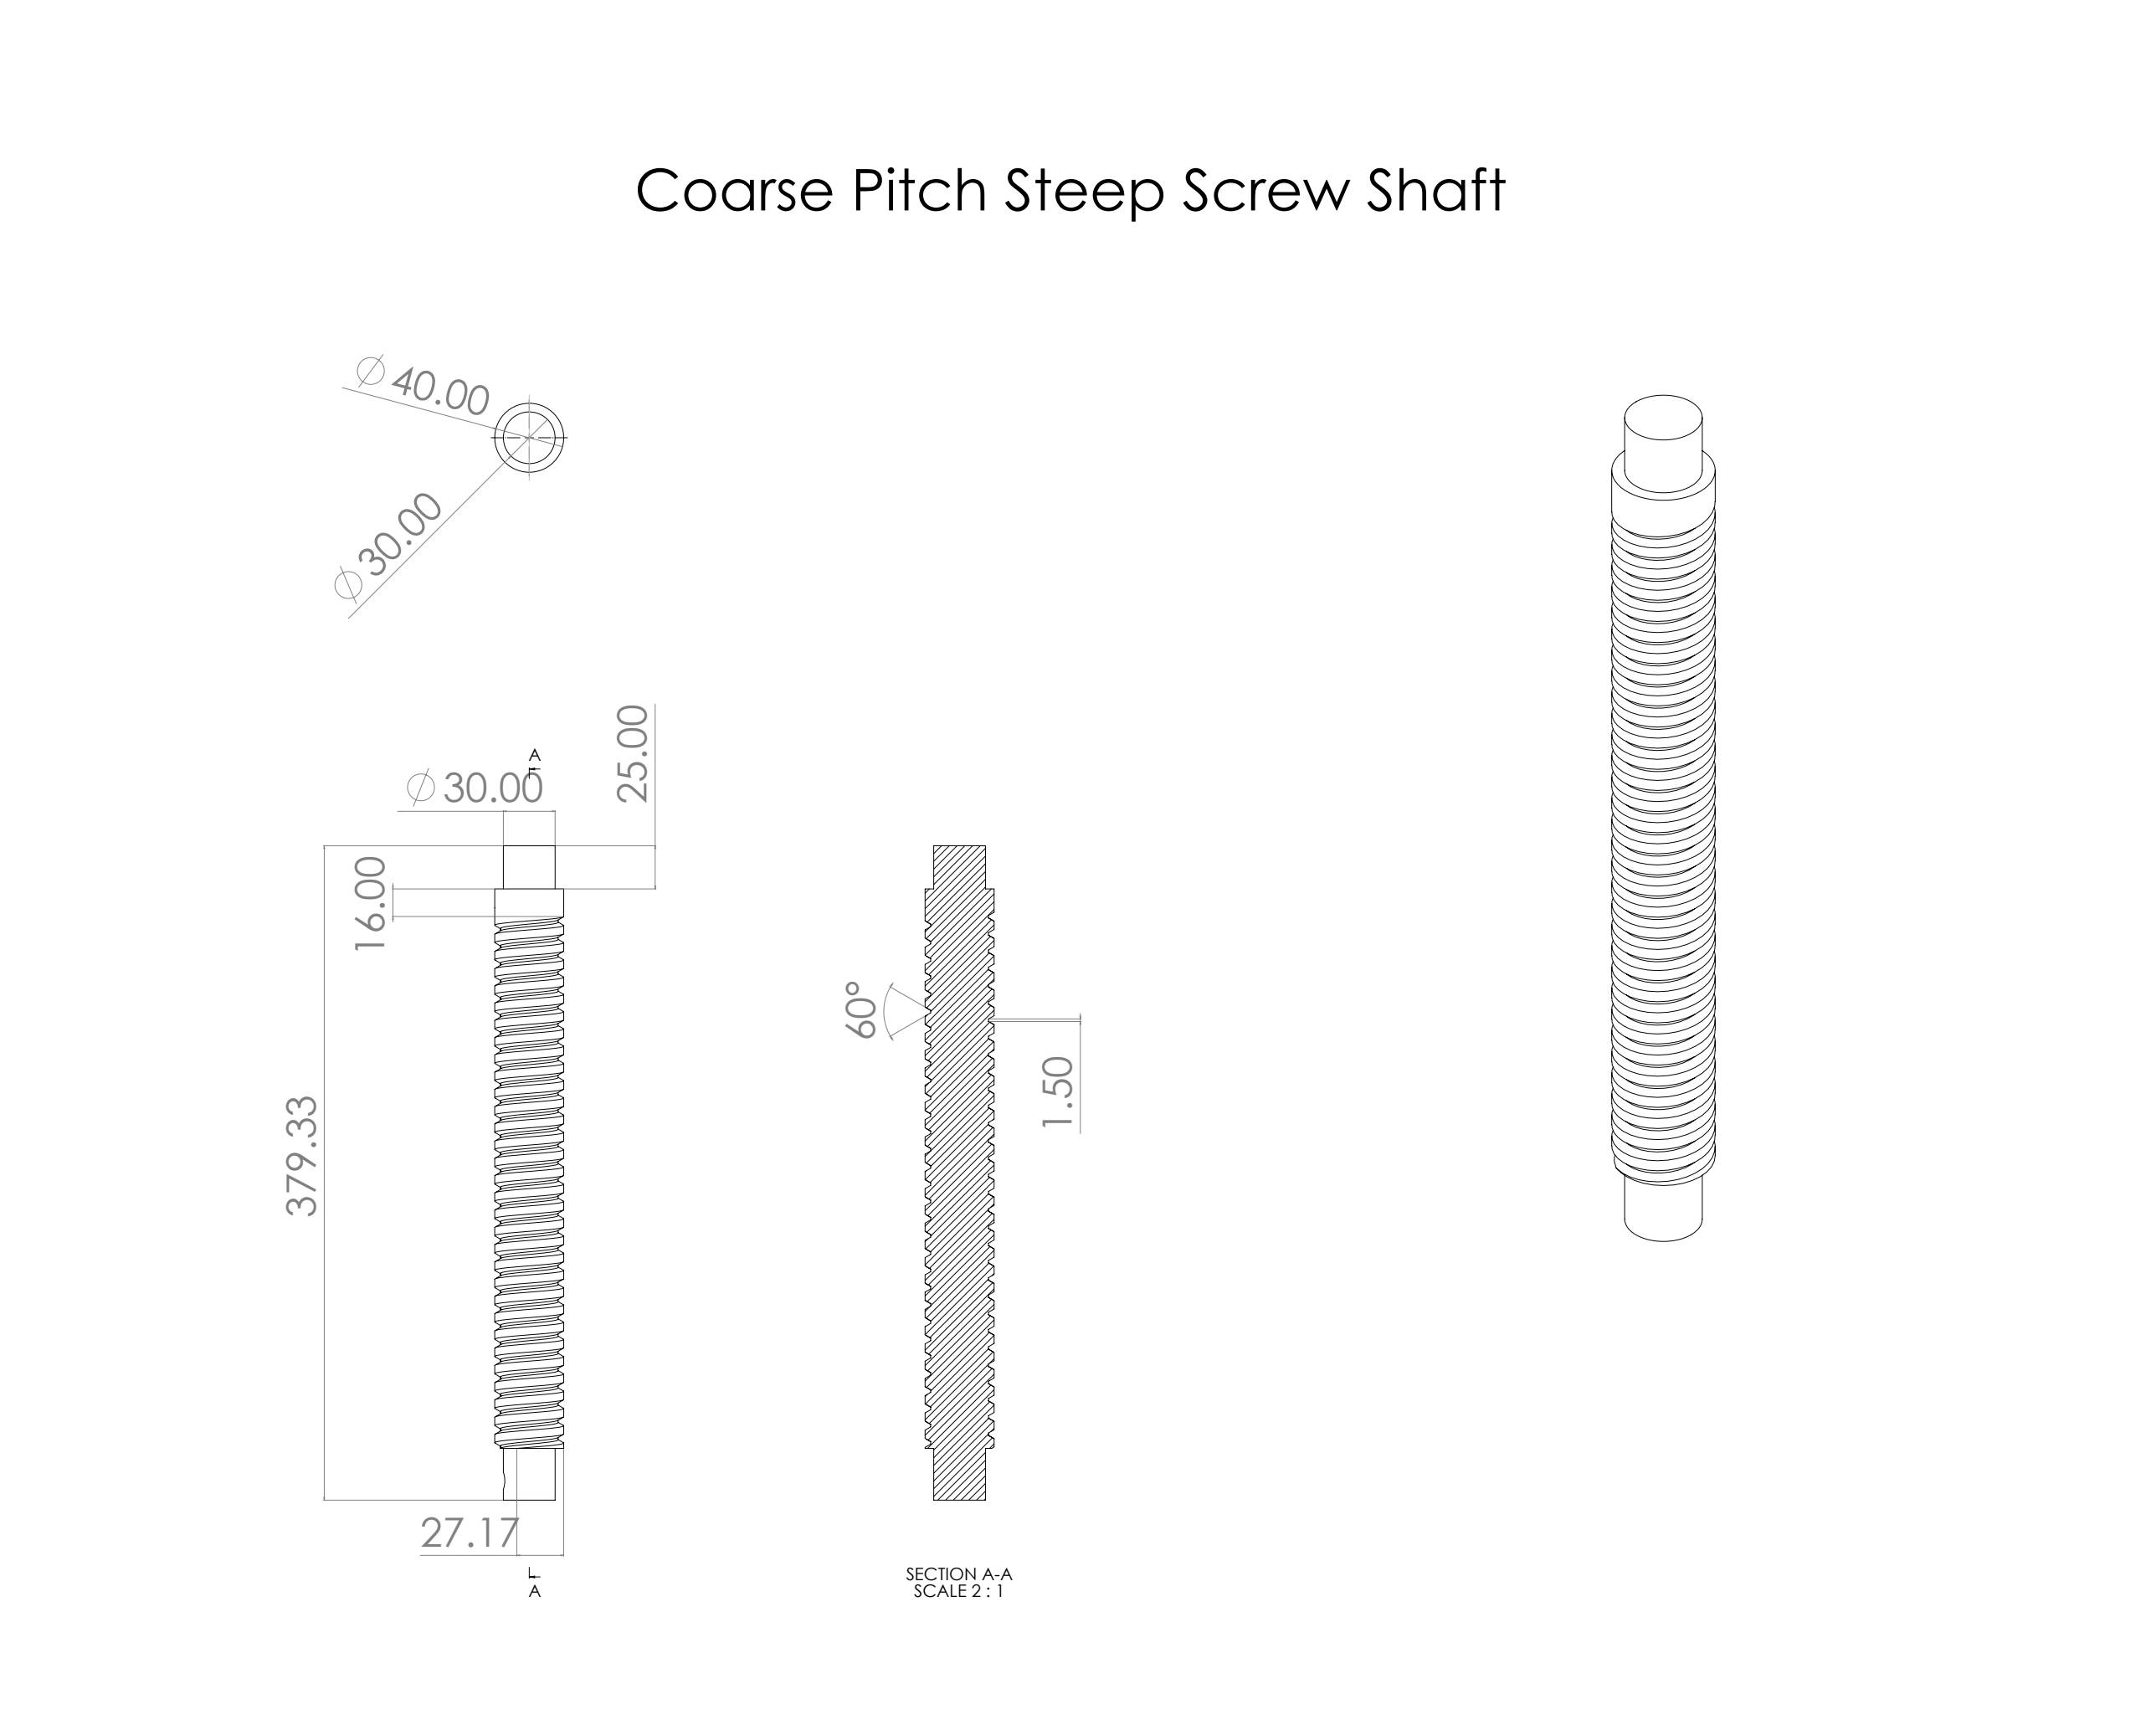
ISO-10303-21;
HEADER;
FILE_DESCRIPTION (('STEP AP214'),
    '1' );
FILE_NAME ('Coarse Pitch Steep Screw Shaft.step',
    '2026-10-24T00:28:05',
    ( '' ),
    ( '' ),
    'SwSTEP 2.0',
    'SolidWorks 2025',
    '' );
FILE_SCHEMA (( 'AUTOMOTIVE_DESIGN' ));
ENDSEC;

DATA;
#1=CARTESIAN_POINT ( 'NONE',  ( -40.53162694259543031, 272.6198905683720568, -11.84573899990672707 ) ) ;
#2=CARTESIAN_POINT ( 'NONE',  ( -13.20868407381886200, 380.9948905683720568, -6.410867750099233042 ) ) ;
#6=CARTESIAN_POINT ( 'NONE',  ( -10.20829729246297646, 267.6198905765655809, -7.653668647301794969 ) ) ;
#7=CARTESIAN_POINT ( 'NONE',  ( -42.88789093042844058, 432.9323905683720000, -9.489475012073736337 ) ) ;
#10=CARTESIAN_POINT ( 'NONE',  ( -47.16347859291445133, 436.6198905601784759, -7.653668647301793193 ) ) ;
#15=CARTESIAN_POINT ( 'NONE',  ( -40.01497788969912506, 298.8073905601784759, 16.95518130045146776 ) ) ;
#17=CARTESIAN_POINT ( 'NONE',  ( -40.53162694259543741, 334.1198905683720568, -11.84573899990672707 ) ) ;
#18=CARTESIAN_POINT ( 'NONE',  ( -48.68588794268872277, 492.3073905765656946, 3.978247347593168115 ) ) ;
#19=CARTESIAN_POINT ( 'NONE',  ( -25.35362745456398059, 366.6823905683720000, 16.75240474999998952 ) ) ;
#20=CARTESIAN_POINT ( 'NONE',  ( -28.68588794268870856, 309.4948905765656377, -19.99999999999999289 ) ) ;
#21=CARTESIAN_POINT ( 'NONE',  ( -11.93348319268872437, 388.5573905683719431, 3.332260488124728859 ) ) ;
#22=CARTESIAN_POINT ( 'NONE',  ( -36.33955658999050087, 300.1198905765656377, -18.47759065022572855 ) ) ;
#24=CARTESIAN_POINT ( 'NONE',  ( -28.68588794268870146, 276.3698905683720000, 16.75240474999999307 ) ) ;
#27=CARTESIAN_POINT ( 'NONE',  ( -16.84014894278199392, 429.1198905683720000, 11.84573899990672530 ) ) ;
#29=CARTESIAN_POINT ( 'NONE',  ( -45.64106924314019409, 498.1823905601784759, 11.32908994701042538 ) ) ;
#31=CARTESIAN_POINT ( 'NONE',  ( -36.33955658999052218, 449.1198905601784759, 18.47759065022572500 ) ) ;
#33=CARTESIAN_POINT ( 'NONE',  ( -35.09675569278794427, 343.4948905683720000, -15.47720386886985544 ) ) ;
#34=CARTESIAN_POINT ( 'NONE',  ( -45.43829269268872650, 483.8698905683720568, 0.000000000000000000 ) ) ;
#36=CARTESIAN_POINT ( 'NONE',  ( -14.54375231895778597, 493.4948905601784759, -14.14213562373094746 ) ) ;
#37=CARTESIAN_POINT ( 'NONE',  ( -11.93348319268871371, 298.8698905683720000, -2.051577885510841163E-15 ) ) ;
#43=ORIENTED_EDGE ( 'NONE', *, *, #17610, .F. ) ;
#44=CYLINDRICAL_SURFACE ( 'NONE', #20879, 19.99999999999999645 ) ;
#46=CARTESIAN_POINT ( 'NONE',  ( -38.17536295476245556, 396.9323905683721136, 14.20200298773971781 ) ) ;
#47=CARTESIAN_POINT ( 'NONE',  ( -42.82802356641967378, 478.4948905601784759, 14.14213562373094923 ) ) ;
#50=CARTESIAN_POINT ( 'NONE',  ( -35.09675569278795848, 415.7448905683720000, 15.47720386886985366 ) ) ;
#52=CARTESIAN_POINT ( 'NONE',  ( -44.16309181155858710, 453.2448905683720000, -6.410867750099231266 ) ) ;
#54=( BOUNDED_CURVE ( )  B_SPLINE_CURVE ( 2, ( #11189, #17470, #6102, #14134, #19307, #19518, #7828, #9666, #17890, #9247, #17790, #20831, #12824, #19413, #5894, #9562, #16180 ),
 .UNSPECIFIED., .F., .T. ) 
 B_SPLINE_CURVE_WITH_KNOTS ( ( 3, 2, 2, 2, 2, 2, 2, 2, 3 ),
 ( 0.5937500000000002220, 0.5957031250000002220, 0.5976562500000002220, 0.5996093750000002220, 0.6015625000000002220, 0.6035156250000002220, 0.6054687500000002220, 0.6074218750000002220, 0.6093750000000002220 ),
 .UNSPECIFIED. ) 
 CURVE ( )  GEOMETRIC_REPRESENTATION_ITEM ( )  RATIONAL_B_SPLINE_CURVE ( ( 0.9999999999999977796, 0.9807852804032326510, 1.000000000000000000, 0.9807852804032304306, 1.000000000000000000, 0.9807852804032304306, 1.000000000000000000, 0.9807852804032304306, 1.000000000000000000, 0.9807852804032304306, 1.000000000000000000, 0.9807852804032304306, 1.000000000000000000, 0.9807852804032304306, 1.000000000000000000, 0.9807852804032282101, 1.000000000000002220 ) ) 
 REPRESENTATION_ITEM ( '' )  );
#56=DIRECTION ( 'NONE',  ( -1.191790137725560488E-16, 1.000000000000000000, -0.000000000000000000 ) ) ;
#57=CARTESIAN_POINT ( 'NONE',  ( -40.01497788969913927, 393.5573905765656377, 16.95518130045146776 ) ) ;
#58=CYLINDRICAL_SURFACE ( 'NONE', #7896, 15.00000000000000000 ) ;
#61=CARTESIAN_POINT ( 'NONE',  ( -47.16347859291445843, 491.3698905765655809, -7.653668647301793193 ) ) ;
#62=CARTESIAN_POINT ( 'NONE',  ( -11.93348319268873858, 500.3698905683720000, -2.051577885510841163E-15 ) ) ;
#65=DIRECTION ( 'NONE',  ( -1.191790137725560488E-16, 1.000000000000000000, -0.000000000000000000 ) ) ;
#67=CARTESIAN_POINT ( 'NONE',  ( -48.68588794268872277, 467.2448905601784759, 0.000000000000000000 ) ) ;
#69=CARTESIAN_POINT ( 'NONE',  ( -11.93348319268872615, 400.3698905683720000, -2.051577885510841163E-15 ) ) ;
#71=CARTESIAN_POINT ( 'NONE',  ( -22.27502019258946930, 222.2448905683720568, -15.47720386886985544 ) ) ;
#72=CARTESIAN_POINT ( 'NONE',  ( -22.27502019258947641, 356.9948905683720000, 15.47720386886985189 ) ) ;
#75=CARTESIAN_POINT ( 'NONE',  ( -44.16309181155859420, 533.2448905683719431, -6.410867750099231266 ) ) ;
#76=ORIENTED_EDGE ( 'NONE', *, *, #1697, .T. ) ;
#77=CARTESIAN_POINT ( 'NONE',  ( -11.93348319268873148, 450.3698905683720000, -2.051577885510841163E-15 ) ) ;
#78=CARTESIAN_POINT ( 'NONE',  ( -11.93348319268874036, 519.1823905683719431, -3.332260488124732856 ) ) ;
#81=CARTESIAN_POINT ( 'NONE',  ( -36.33955658999052218, 429.1198905601784759, 18.47759065022572500 ) ) ;
#82=CARTESIAN_POINT ( 'NONE',  ( -45.43829269268872650, 493.8698905683720568, 0.000000000000000000 ) ) ;
#84=CARTESIAN_POINT ( 'NONE',  ( -13.20868407381887799, 499.4948905683720568, -6.410867750099233042 ) ) ;
#86=CARTESIAN_POINT ( 'NONE',  ( -40.01497788969914637, 440.4323905765656377, -16.95518130045146421 ) ) ;
#88=CARTESIAN_POINT ( 'NONE',  ( -8.685887942688530927, 247.3073905765656093, -3.978247347592740013 ) ) ;
#93=CARTESIAN_POINT ( 'NONE',  ( -28.68588794268870856, 292.8698905683720568, -16.75240474999999307 ) ) ;
#95=CARTESIAN_POINT ( 'NONE',  ( -14.54375231895775400, 260.9948905601784759, 14.14213562373094568 ) ) ;
#98=CARTESIAN_POINT ( 'NONE',  ( -16.84014894278200458, 509.1198905683720568, 11.84573899990672530 ) ) ;
#99=CARTESIAN_POINT ( 'NONE',  ( -32.66413529028187668, 369.4323905601784190, 19.99999999999999289 ) ) ;
#102=CARTESIAN_POINT ( 'NONE',  ( -14.48388495494900852, 469.4323905683720568, 9.489475012073732785 ) ) ;
#103=CARTESIAN_POINT ( 'NONE',  ( -42.88789093042842637, 274.8073905683720000, 9.489475012073736337 ) ) ;
#108=CARTESIAN_POINT ( 'NONE',  ( -10.20829729246297291, 237.6198905765656377, -7.653668647301794969 ) ) ;
#109=CARTESIAN_POINT ( 'NONE',  ( -28.68588794268870501, 309.7448905601785327, 19.99999999999999289 ) ) ;
#110=CARTESIAN_POINT ( 'NONE',  ( -48.68588794268872988, 537.2448905601785327, 0.000000000000000000 ) ) ;
#112=CARTESIAN_POINT ( 'NONE',  ( -44.16309181155856578, 273.2448905683720568, -6.410867750099231266 ) ) ;
#114=CARTESIAN_POINT ( 'NONE',  ( -11.93348319268872260, 350.6823905683720000, -3.332260488124732856 ) ) ;
#115=EDGE_CURVE ( 'NONE', #339, #18802, #16604, .T. ) ;
#118=CARTESIAN_POINT ( 'NONE',  ( -19.19641293061498999, 427.3073905683720568, 14.20200298773971426 ) ) ;
#119=CARTESIAN_POINT ( 'NONE',  ( -14.54375231895778420, 510.9948905601784190, 14.14213562373094568 ) ) ;
#121=CARTESIAN_POINT ( 'NONE',  ( -14.54375231895777354, 420.9948905601784759, 14.14213562373094568 ) ) ;
#125=ORIENTED_EDGE ( 'NONE', *, *, #1712, .T. ) ;
#126=VERTEX_POINT ( 'NONE', #20705 ) ;
#127=CARTESIAN_POINT ( 'NONE',  ( -45.43829269268873361, 525.3698905683720568, 0.000000000000000000 ) ) ;
#128=CARTESIAN_POINT ( 'NONE',  ( -36.33955658999050087, 305.3698905601784759, -18.47759065022572855 ) ) ;
#131=CARTESIAN_POINT ( 'NONE',  ( -35.09675569278794427, 343.4948905683720000, -15.47720386886985544 ) ) ;
#133=CARTESIAN_POINT ( 'NONE',  ( -45.64106924314020119, 481.0573905765656377, -11.32908994701042715 ) ) ;
#134=CARTESIAN_POINT ( 'NONE',  ( -38.17536295476245556, 362.3073905683719431, -14.20200298773971426 ) ) ;
#135=VECTOR ( 'NONE', #18235, 1000.000000000000000 ) ;
#136=CARTESIAN_POINT ( 'NONE',  ( -14.48388495494899963, 377.9323905683720000, 9.489475012073731008 ) ) ;
#137=CARTESIAN_POINT ( 'NONE',  ( -14.54375231895775933, 305.7448905765656377, 14.14213562373094568 ) ) ;
#139=CARTESIAN_POINT ( 'NONE',  ( -32.01814843081343298, 271.6823905683720000, -16.75240474999999307 ) ) ;
#140=CARTESIAN_POINT ( 'NONE',  ( -24.70764059509555821, 440.0573905601785327, 19.99999999999998934 ) ) ;
#141=CARTESIAN_POINT ( 'NONE',  ( -28.68588794268871922, 427.8698905683720568, 16.75240474999999307 ) ) ;
#143=CARTESIAN_POINT ( 'NONE',  ( -48.68588794268881514, 497.5573905601784190, 3.978247347592954952 ) ) ;
#148=CARTESIAN_POINT ( 'NONE',  ( -13.20868407381885845, 340.9948905683720000, -6.410867750099233042 ) ) ;
#149=CARTESIAN_POINT ( 'NONE',  ( -32.01814843081346140, 486.0573905683721136, 16.75240474999999307 ) ) ;
#152=CARTESIAN_POINT ( 'NONE',  ( -28.68588794268872633, 489.7448905601784759, 19.99999999999999289 ) ) ;
#153=CARTESIAN_POINT ( 'NONE',  ( -40.53162694259543031, 312.6198905683720000, -11.84573899990672707 ) ) ;
#159=CARTESIAN_POINT ( 'NONE',  ( -42.88789093042844058, 394.4323905683720000, -9.489475012073734561 ) ) ;
#160=CARTESIAN_POINT ( 'NONE',  ( -14.54375231895777709, 445.7448905765656377, 14.14213562373094568 ) ) ;
#162=CARTESIAN_POINT ( 'NONE',  ( -22.27502019258948351, 416.9948905683720000, 15.47720386886985189 ) ) ;
#163=CARTESIAN_POINT ( 'NONE',  ( -38.17536295476243424, 256.9323905683720568, 14.20200298773971781 ) ) ;
#164=CARTESIAN_POINT ( 'NONE',  ( -38.17536295476246266, 442.3073905683721136, -14.20200298773971426 ) ) ;
#166=CARTESIAN_POINT ( 'NONE',  ( -48.68588794268873698, 573.2448905601785327, 0.000000000000000000 ) ) ;
#167=CARTESIAN_POINT ( 'NONE',  ( -10.20829729246298534, 356.3698905765655809, 7.653668647301790529 ) ) ;
#169=CARTESIAN_POINT ( 'NONE',  ( -14.54375231895777354, 388.2448905765655809, -14.14213562373094746 ) ) ;
#170=CARTESIAN_POINT ( 'NONE',  ( -32.66413529028187668, 429.8073905765656946, -19.99999999999999289 ) ) ;
#172=CARTESIAN_POINT ( 'NONE',  ( -22.27502019258949417, 498.4948905683720568, 15.47720386886985189 ) ) ;
#175=CARTESIAN_POINT ( 'NONE',  ( -40.01497788969915348, 465.6823905601785896, -16.95518130045146421 ) ) ;
#176=CARTESIAN_POINT ( 'NONE',  ( -14.54375231895777354, 420.9948905601784759, 14.14213562373094568 ) ) ;
#177=CARTESIAN_POINT ( 'NONE',  ( -11.93348319268872615, 400.6823905683720568, -3.332260488124732856 ) ) ;
#178=CARTESIAN_POINT ( 'NONE',  ( -47.16347859291445843, 471.3698905765656377, -7.653668647301793193 ) ) ;
#180=CARTESIAN_POINT ( 'NONE',  ( -42.88789093042841927, 236.3073905683720284, 9.489475012073736337 ) ) ;
#181=CARTESIAN_POINT ( 'NONE',  ( -35.09675569278795138, 365.7448905683720568, 15.47720386886985366 ) ) ;
#183=CARTESIAN_POINT ( 'NONE',  ( -16.84014894278200813, 527.6198905683719431, 11.84573899990672530 ) ) ;
#185=CARTESIAN_POINT ( 'NONE',  ( -35.09675569278795848, 447.2448905683720000, 15.47720386886985366 ) ) ;
#186=( BOUNDED_CURVE ( )  B_SPLINE_CURVE ( 2, ( #15683, #18905, #9166, #8954, #869, #19445, #2803, #4526, #19338, #8177, #16322, #1390, #12644, #11113, #16106, #17715, #7966, #3227, #12748, #9388, #20969, #19235, #11001, #14702, #1604, #16006, #4629, #6032, #9702, #21278, #1189, #19652, #11223, #18032, #12856, #14808, #9803, #4832, #1496, #17820, #3012, #6451, #7759, #4419, #17612, #2913, #9493, #16426, #14385, #6138, #1283, #7861, #14489, #21070, #6244, #9596, #16213, #8072, #12959, #19548, #14595, #13067, #11432, #21177, #6349, #4729, #11326, #17920, #3118, #15134, #11654, #3650, #13178, #3748, #8400, #11760, #18356, #8721, #18246, #1830, #8286, #19984, #15026, #16753, #98, #20097, #13397, #18136, #19875, #13290, #2139, #10231, #1940, #6557, #5050, #10021, #3438, #8506, #18566, #6670, #3330, #16531, #19763, #4947, #8608, #16958, #9912, #5164, #20768, #16855, #15231, #1717, #13612, #3545, #11969, #6776, #11547, #10336, #20198, #2039, #10132, #14915, #16646, #425, #315, #209, #6883, #13503, #5266, #5365, #11868, #18461, #6991, #10875, #2352, #10445, #631, #10552, #740, #12189, #5585, #7091, #5797, #13712, #20306, #17173, #18775, #8932, #17275, #12296, #15557, #5689, #9041, #529, #12403, #4292, #955, #17481, #2563, #15766, #15347, #3962, #7306, #7521, #19110, #13933, #20522, #9145, #18884, #2669, #4071, #10655, #14146, #2460, #8827, #20732, #18666, #5476, #12074, #15662, #7197, #848, #13819, #7413, #3856, #5906, #12515, #17067, #2250, #15445, #14039, #18994, #20621, #20410, #4178, #10767, #17382, #21258, #1063, #15874, #16082, #16189, #2989, #18007, #17898, #19213, #1163, #4500, #6326, #4606, #4810, #20842, #11404, #1261, #21154, #7838, #11089, #11198, #9366, #7938, #14466, #4705, #21048, #6114, #17799, #6216, #1367, #7629, #15981, #19314, #3093, #9572, #4396, #13040, #12832, #10978, #14256, #6014, #9675, #9257, #12623, #2886, #17694, #20944, #11301, #17588, #2780, #19421, #7735, #16299, #1472, #14365, #8048, #9470, #12725, #14569, #12940, #19526, #14680, #6424, #19630, #3201, #8878, #8376, #18328, #19739, #20465, #11629, #4923, #9887, #19851, #9993, #77, #14890, #6644, #5242, #13477, #10105, #6534, #10497, #14999, #5139, #185, #5028, #6753, #3518, #9779, #290, #13876, #21366, #18113, #2297, #11520, #13371, #16727, #20070, #15496, #18223, #13265, #3416, #11842, #17118, #1807, #682, #16617, #12244, #7248, #5635, #6859, #19961, #16404, #11738, #1915, #8483, #15106, #18438, #1581, #3625, #3309, #8152, #14780, #16511, #13151, #1690, #8261, #12491, #1034, #12597, #2644, #17455, #9230, #7813, #16062, #12700, #9120, #12805, #10954, #14542, #17564, #6193, #17774, #20919, #12078, #2861, #16165, #19397, #1341, #14443, #4581, #5478, #19189, #20704, #15850, #21024, #4368, #1139, #14229, #9332, #14339, #6086, #19081, #7914, #18967, #15742, #4149, #4264, #7598, #5878, #20817, #5987, #929, #1239, #19291, #4477, #10741, #10851, #11172, #11060, #17355, #2967, #2755, #17668, #9546, #9445, #15953, #2537, #7495, #14118, #7712, #11494, #18091, #8456, #17979, #1556, #8023, #19933, #13346, #3178, #3493, #3067, #1449, #17875, #19608, #13015, #1889, #9972, #16487, #6302, #4784, #9758, #11381, #1669, #18303, #6402, #12913, #16381, #8126, #14759, #8238, #10079, #21343, #19714, #16273, #19503, #4682, #8348, #16700, #9651, #4897, #21128, #3393, #14972, #14655, #5111, #3286, #11711, #6511, #11275, #21236, #13127, #16591, #9860, #14868, #46, #1781, #6618, #13239, #19829, #5004, #11605, #18195, #159, #6730, #10183, #10609, #2089, #16804, #370, #10288, #482, #11919, #13880, #6833, #5532, #13449, #20040, #16909, #5319, #8670, #17014, #12025, #15294, #5425, #8781, #267, #12138, #4015, #687, #17227, #2301, #15501, #2409, #18513, #3700, #7253, #7045, #8563, #8885, #18410, #15081, #5217, #13665, #6939, #11816, #3599, #1995, #15185, #13563, #20252, #20151, #18618, #20471, #2196, #18724, #3804, #5640, #10395, #3912, #10502, #12248, #15397, #578, #7147, #13770, #18831, #20358, #17123, #12673, #798, #12779, #17435, #4345, #4558, #20573, #11145, #1010, #20895, #7576, #10825, #10928, #9098, #7686, #14202, #5740, #7466, #902, #17750, #19268, #17538, #15924, #7364, #15611, #15826, #2729, #6169, #9309, #20678, #4448, #13991, #19372, #2619, #20792, #5958, #8989, #5853, #9199, #17330, #7787, #1217, #12458, #12352, #10710, #18939, #11034, #12573, #19057, #1115, #19167, #14315, #4124, #15718, #4240, #2837, #6063, #2513, #14097, #17643, #9419, #16039, #14419, #21001, #19798, #8322, #17953, #12988, #14629, #4978, #2941, #16137, #8101, #6276, #11577, #18168, #1320, #16565, #19580, #11251, #17848, #7891, #13214, #19686, #1640, #19904, #6591, #3044, #3365, #13100, #3259, #9520, #7997, #9945, #1750, #4760, #14945, #131, #14519, #6704, #21102, #14841, #12890, #19480, #13321, #14731, #11686, #21312, #5085, #4660, #9627, #16246, #1423, #11356, #21214, #6379, #16354, #3151, #9732, #1531, #6484, #4871, #11466, #18064, #9835, #16458, #8213, #17, #5397, #10163, #20334, #15269, #3574, #20126, #20441, #10476, #17097, #3887, #10053, #12106, #20227, #15375, #348, #8856, #18385, #5506, #10261, #18700, #13537, #7227, #8538, #6912, #2277, #3678, #11789, #15477, #239, #13850, #5615, #15161, #16781, #18277, #3465, #6808, #16677, #663, #1863, #8435, #15057, #13425, #12001, #553, #5293, #20017, #5193, #7122, #13748, #1967, #11896, #18489, #16882, #18592, #2066, #3778, #8641, #452, #7018, #13641, #10366, #16991, #2171, #8755, #14394, #4216, #2706, #10798, #14069, #7552, #12325, #10904, #17414, #8964, #10686, #4098, #14177, #9176, #4321, #10579, #18913, #879, #6042, #20767, #770, #16015, #2596, #7335, #18806, #17202, #20877, #7768, #15587, #15801, #12223, #15903, #7662, #3988, #2381, #988, #13968, #14290, #12651, #20551, #4428, #7443, #5717, #17305, #2488, #1094, #5935, #9071, #5824, #15692, #20654, #17621, #12550, #19144, #12434, #19030, #19245, #11012, #17515, #2812, #9396, #9287, #1197, #20978, #18040, #19347, #4535, #7976, #17828, #1400, #8081, #3126, #18145, #9501, #16115, #11121, #16223, #9922, #3022, #1292, #4738, #6146, #9812, #5558, #2921, #19772, #11335, #3340, #12967, #14925, #16541, #4957, #14603, #14498, #21081, #17726, #16435, #1506, #12758, #21186, #6253, #7869, #11557, #17929, #21287, #12864, #1726, #6357, #19454, #4637, #19557, #9711, #11231, #8298, #9604, #3236, #16331, #14711, #6460, #13076, #19662, #4841, #11440, #1614, #8187, #14817, #6568, #13188, #8833, #5484, #13298, #8729, #1947, #19884, #11768, #20104, #18675, #3657, #15034, #3863, #1841, #11664, #19993, #18363, #8619, #15243, #20207, #11977, #10345, #2148, #4740, #16225, #12969, #3024, #11558, #1616, #8188, #18255, #1402, #3342, #14818, #6255, #9923, #14606, #19456, #4864, #9813, #3446, #16542, #4639, #21188, #11337, #6462, #13078, #16117, #9713, #16333, #9606, #6679, #13299, #19665, #19885, #6359, #11442, #18043, #1727, #3237, #16436, #6569, #13189, #19773, #5061, #11665, #15143, #11981, #7207, #16760, #6787, #3554, #8837, #5172, #432, #2151, #6999, #538, #8732, #5596, #13725, #10143, #5487, #20209, #10348, #12200, #18470, #11769, #1948, #5274, #16865, #6892, #325, #13512, #12086, #20315, #16971, #13405, #17076, #15245, #18787, #13621, #10456, #641, #19994, #16656, #7104, #20421, #2259, #10030, #18678, #15457, #1842, #2048, #8516, #20105, #3866, #8622, #5375, #3658, #18575, #3758, #15357, #11878, #13829, #8410, #18364, #15035, #10241, #218, #4081, #859, #7423, #20532, #20855, #10886, #17493, #6129, #10667, #12635, #2684, #2363, #6025, #17286, #10561, #1177, #19121, #15673, #7645, #17184, #7748, #12414, #15780, #968, #12737, #14050, #5807, #12305, #2793, #17601, #20633, #14377, #7316 ),
 .UNSPECIFIED., .F., .T. ) 
 B_SPLINE_CURVE_WITH_KNOTS ( ( 3, 2, 2, 2, 2, 2, 2, 2, 2, 2, 2, 2, 2, 2, 2, 2, 2, 2, 2, 2, 2, 2, 2, 2, 2, 2, 2, 2, 2, 2, 2, 2, 2, 2, 2, 2, 2, 2, 2, 2, 2, 2, 2, 2, 2, 2, 2, 2, 2, 2, 2, 2, 2, 2, 2, 2, 2, 2, 2, 2, 2, 2, 2, 2, 2, 2, 2, 2, 2, 2, 2, 2, 2, 2, 2, 2, 2, 2, 2, 2, 2, 2, 2, 2, 2, 2, 2, 2, 2, 2, 2, 2, 2, 2, 2, 2, 2, 2, 2, 2, 2, 2, 2, 2, 2, 2, 2, 2, 2, 2, 2, 2, 2, 2, 2, 2, 2, 2, 2, 2, 2, 2, 2, 2, 2, 2, 2, 2, 2, 2, 2, 2, 2, 2, 2, 2, 2, 2, 2, 2, 2, 2, 2, 2, 2, 2, 2, 2, 2, 2, 2, 2, 2, 2, 2, 2, 2, 2, 2, 2, 2, 2, 2, 2, 2, 2, 2, 2, 2, 2, 2, 2, 2, 2, 2, 2, 2, 2, 2, 2, 2, 2, 2, 2, 2, 2, 2, 2, 2, 2, 2, 2, 2, 2, 2, 2, 2, 2, 2, 2, 2, 2, 2, 2, 2, 2, 2, 2, 2, 2, 2, 2, 2, 2, 2, 2, 2, 2, 2, 2, 2, 2, 2, 2, 2, 2, 2, 2, 2, 2, 2, 2, 2, 2, 2, 2, 2, 2, 2, 2, 2, 2, 2, 2, 2, 2, 2, 2, 2, 2, 2, 2, 2, 2, 2, 2, 2, 2, 2, 2, 2, 2, 2, 2, 2, 2, 2, 2, 2, 2, 2, 2, 2, 2, 2, 2, 2, 2, 2, 2, 2, 2, 2, 2, 2, 2, 2, 2, 2, 2, 2, 2, 2, 2, 2, 2, 2, 2, 2, 2, 2, 2, 2, 2, 2, 2, 2, 2, 2, 2, 2, 2, 2, 2, 2, 2, 2, 2, 2, 2, 2, 2, 2, 2, 2, 2, 2, 2, 2, 2, 2, 2, 2, 2, 2, 2, 2, 2, 2, 2, 2, 2, 2, 2, 2, 2, 2, 2, 2, 2, 2, 2, 2, 2, 2, 2, 2, 2, 2, 2, 2, 2, 2, 2, 2, 2, 2, 2, 2, 2, 2, 2, 2, 2, 2, 2, 2, 2, 2, 2, 2, 2, 2, 2, 2, 2, 2, 2, 2, 2, 2, 2, 2, 2, 2, 2, 2, 2, 2, 2, 2, 2, 2, 2, 2, 2, 2, 2, 2, 2, 2, 2, 2, 2, 2, 2, 2, 2, 2, 2, 2, 2, 2, 2, 2, 2, 2, 2, 2, 2, 2, 2, 2, 2, 2, 2, 2, 2, 2, 2, 2, 2, 2, 2, 2, 2, 2, 2, 2, 2, 2, 2, 2, 2, 2, 2, 2, 2, 2, 2, 2, 2, 2, 2, 2, 2, 2, 2, 2, 2, 2, 2, 2, 2, 2, 2, 2, 2, 2, 2, 2, 2, 2, 2, 2, 2, 2, 2, 2, 2, 2, 2, 2, 2, 2, 2, 2, 2, 2, 3 ),
 ( 0.000000000000000000, 0.001953125000000000000, 0.003906250000000000000, 0.005859374999999999133, 0.007812500000000000000, 0.009765625000000000000, 0.01171874999999999827, 0.01367187500000000000, 0.01562500000000000000, 0.01757812500000000000, 0.01953125000000000000, 0.02148437500000000000, 0.02343749999999999653, 0.02539062500000000000, 0.02734375000000000000, 0.02929687500000000000, 0.03125000000000000000, 0.03320312500000000000, 0.03515625000000000000, 0.03710937500000000000, 0.03906250000000000000, 0.04101562500000000000, 0.04296875000000000000, 0.04492187500000000000, 0.04687499999999999306, 0.04882812500000000000, 0.05078125000000000000, 0.05273437500000000000, 0.05468750000000000000, 0.05664062500000000000, 0.05859375000000000000, 0.06054687500000000000, 0.06250000000000000000, 0.06445312500000000000, 0.06640625000000000000, 0.06835937500000000000, 0.07031250000000000000, 0.07226562500000000000, 0.07421875000000000000, 0.07617187500000000000, 0.07812500000000000000, 0.08007812500000000000, 0.08203125000000000000, 0.08398437500000000000, 0.08593750000000000000, 0.08789062500000000000, 0.08984375000000000000, 0.09179687500000000000, 0.09374999999999998612, 0.09570312500000000000, 0.09765625000000000000, 0.09960937500000000000, 0.1015625000000000000, 0.1035156250000000000, 0.1054687500000000000, 0.1074218750000000000, 0.1093750000000000000, 0.1113281250000000000, 0.1132812500000000000, 0.1152343750000000000, 0.1171875000000000000, 0.1191406250000000000, 0.1210937500000000000, 0.1230468750000000000, 0.1250000000000000000, 0.1269531250000000000, 0.1289062500000000000, 0.1308593750000000000, 0.1328125000000000000, 0.1347656250000000000, 0.1367187500000000000, 0.1386718750000000000, 0.1406250000000000000, 0.1425781250000000000, 0.1445312500000000000, 0.1464843750000000000, 0.1484375000000000000, 0.1503906250000000000, 0.1523437500000000000, 0.1542968750000000000, 0.1562500000000000000, 0.1582031250000000000, 0.1601562500000000000, 0.1621093750000000000, 0.1640625000000000000, 0.1660156250000000000, 0.1679687500000000000, 0.1699218750000000000, 0.1718750000000000000, 0.1738281250000000000, 0.1757812500000000000, 0.1777343750000000000, 0.1796875000000000000, 0.1816406250000000000, 0.1835937500000000000, 0.1855468750000000000, 0.1874999999999999722, 0.1894531250000000000, 0.1914062500000000000, 0.1933593750000000000, 0.1953125000000000000, 0.1972656250000000000, 0.1992187500000000000, 0.2011718750000000000, 0.2031250000000000000, 0.2050781250000000000, 0.2070312500000000000, 0.2089843750000000000, 0.2109375000000000000, 0.2128906250000000000, 0.2148437500000000000, 0.2167968750000000000, 0.2187500000000000000, 0.2207031250000000000, 0.2226562500000000000, 0.2246093750000000000, 0.2265625000000000000, 0.2285156250000000000, 0.2304687500000000000, 0.2324218750000000000, 0.2343750000000000000, 0.2363281250000000000, 0.2382812500000000000, 0.2402343750000000000, 0.2421875000000000000, 0.2441406250000000000, 0.2460937500000000000, 0.2480468750000000000, 0.2500000000000000000, 0.2519531250000000000, 0.2539062500000000000, 0.2558593750000000000, 0.2578125000000000000, 0.2597656250000000000, 0.2617187500000000000, 0.2636718750000000000, 0.2656250000000000000, 0.2675781250000000000, 0.2695312500000000000, 0.2714843750000000000, 0.2734375000000000000, 0.2753906250000000000, 0.2773437500000000000, 0.2792968750000000000, 0.2812500000000000000, 0.2832031250000000000, 0.2851562500000000000, 0.2871093750000000000, 0.2890625000000000000, 0.2910156250000000000, 0.2929687500000000000, 0.2949218750000000000, 0.2968750000000000000, 0.2988281250000000000, 0.3007812500000000000, 0.3027343750000000000, 0.3046875000000000000, 0.3066406250000000000, 0.3085937500000000000, 0.3105468750000000000, 0.3125000000000000000, 0.3144531249999999445, 0.3164062500000000000, 0.3183593750000000000, 0.3203125000000000000, 0.3222656250000000000, 0.3242187500000000000, 0.3261718750000000000, 0.3281250000000000000, 0.3300781250000000000, 0.3320312500000000000, 0.3339843750000000000, 0.3359375000000000000, 0.3378906250000000000, 0.3398437500000000000, 0.3417968750000000000, 0.3437500000000000000, 0.3457031250000000000, 0.3476562500000000000, 0.3496093750000000000, 0.3515625000000000000, 0.3535156250000000000, 0.3554687500000000000, 0.3574218750000000000, 0.3593750000000000000, 0.3613281250000000000, 0.3632812500000000000, 0.3652343750000000000, 0.3671875000000000000, 0.3691406250000000000, 0.3710937500000000000, 0.3730468750000000000, 0.3749999999999999445, 0.3769531250000000000, 0.3789062500000000000, 0.3808593750000000000, 0.3828125000000000000, 0.3847656250000000000, 0.3867187500000000000, 0.3886718750000000000, 0.3906250000000000000, 0.3925781250000000000, 0.3945312500000000000, 0.3964843750000000000, 0.3984375000000000000, 0.4003906250000000000, 0.4023437500000000000, 0.4042968750000000000, 0.4062500000000000000, 0.4082031250000000000, 0.4101562500000000000, 0.4121093750000000000, 0.4140625000000000000, 0.4160156250000000000, 0.4179687500000000000, 0.4199218750000000000, 0.4218750000000000000, 0.4238281250000000000, 0.4257812500000000000, 0.4277343750000000000, 0.4296875000000000000, 0.4316406250000000000, 0.4335937500000000000, 0.4355468750000000555, 0.4375000000000000000, 0.4394531250000000000, 0.4414062500000000000, 0.4433593750000000000, 0.4453125000000000000, 0.4472656250000000000, 0.4492187500000000000, 0.4511718750000000000, 0.4531250000000000000, 0.4550781250000000000, 0.4570312500000000000, 0.4589843750000000000, 0.4609375000000000000, 0.4628906250000000000, 0.4648437500000000000, 0.4667968750000000000, 0.4687500000000000000, 0.4707031250000000000, 0.4726562500000000000, 0.4746093750000000000, 0.4765625000000000000, 0.4785156250000000000, 0.4804687500000000000, 0.4824218750000000000, 0.4843750000000000000, 0.4863281250000000000, 0.4882812500000000000, 0.4902343750000000000, 0.4921875000000000000, 0.4941406250000000000, 0.4960937500000000000, 0.4980468750000000000, 0.5000000000000000000, 0.5019531250000000000, 0.5039062500000000000, 0.5058593750000000000, 0.5078125000000000000, 0.5097656250000000000, 0.5117187500000000000, 0.5136718750000000000, 0.5156250000000000000, 0.5175781250000000000, 0.5195312500000000000, 0.5214843750000000000, 0.5234375000000000000, 0.5253906250000000000, 0.5273437500000000000, 0.5292968750000000000, 0.5312500000000000000, 0.5332031250000000000, 0.5351562500000000000, 0.5371093750000000000, 0.5390625000000000000, 0.5410156250000000000, 0.5429687500000000000, 0.5449218750000000000, 0.5468750000000000000, 0.5488281250000000000, 0.5507812500000000000, 0.5527343750000000000, 0.5546875000000000000, 0.5566406250000000000, 0.5585937500000000000, 0.5605468750000001110, 0.5625000000000000000, 0.5644531250000000000, 0.5664062500000000000, 0.5683593750000000000, 0.5703125000000000000, 0.5722656250000000000, 0.5742187500000000000, 0.5761718750000000000, 0.5781250000000000000, 0.5800781250000000000, 0.5820312500000000000, 0.5839843750000000000, 0.5859375000000000000, 0.5878906250000000000, 0.5898437500000000000, 0.5917968750000000000, 0.5937500000000000000, 0.5957031250000000000, 0.5976562500000000000, 0.5996093750000000000, 0.6015625000000000000, 0.6035156250000000000, 0.6054687500000000000, 0.6074218750000000000, 0.6093750000000000000, 0.6113281250000000000, 0.6132812500000000000, 0.6152343750000000000, 0.6171875000000000000, 0.6191406250000000000, 0.6210937500000000000, 0.6230468750000000000, 0.6250000000000000000, 0.6269531250000000000, 0.6289062499999998890, 0.6308593750000000000, 0.6328125000000000000, 0.6347656250000000000, 0.6367187500000000000, 0.6386718750000000000, 0.6406250000000000000, 0.6425781250000000000, 0.6445312500000000000, 0.6464843750000000000, 0.6484375000000000000, 0.6503906250000000000, 0.6523437500000000000, 0.6542968750000000000, 0.6562500000000000000, 0.6582031250000000000, 0.6601562500000000000, 0.6621093750000000000, 0.6640625000000000000, 0.6660156250000000000, 0.6679687500000000000, 0.6699218750000000000, 0.6718750000000000000, 0.6738281250000000000, 0.6757812500000000000, 0.6777343750000000000, 0.6796875000000000000, 0.6816406250000001110, 0.6835937500000000000, 0.6855468750000000000, 0.6875000000000000000, 0.6894531250000000000, 0.6914062500000000000, 0.6933593750000000000, 0.6953125000000000000, 0.6972656250000000000, 0.6992187500000000000, 0.7011718750000000000, 0.7031250000000000000, 0.7050781250000000000, 0.7070312500000000000, 0.7089843750000000000, 0.7109375000000000000, 0.7128906250000000000, 0.7148437500000000000, 0.7167968750000000000, 0.7187500000000000000, 0.7207031250000000000, 0.7226562500000000000, 0.7246093750000000000, 0.7265625000000000000, 0.7285156250000000000, 0.7304687500000000000, 0.7324218750000000000, 0.7343750000000000000, 0.7363281250000000000, 0.7382812500000000000, 0.7402343750000000000, 0.7421875000000000000, 0.7441406250000000000, 0.7460937500000000000, 0.7480468750000000000, 0.7499999999999998890, 0.7519531250000000000, 0.7539062500000000000, 0.7558593750000000000, 0.7578125000000000000, 0.7597656250000000000, 0.7617187500000000000, 0.7636718750000000000, 0.7656250000000000000, 0.7675781250000000000, 0.7695312500000000000, 0.7714843750000000000, 0.7734375000000000000, 0.7753906250000000000, 0.7773437500000000000, 0.7792968750000000000, 0.7812500000000000000, 0.7832031250000000000, 0.7851562500000000000, 0.7871093750000000000, 0.7890625000000000000, 0.7910156250000000000, 0.7929687500000000000, 0.7949218750000000000, 0.7968750000000000000, 0.7988281250000000000, 0.8007812500000000000, 0.8027343750000000000, 0.8046875000000000000, 0.8066406250000000000, 0.8085937500000000000, 0.8105468750000000000, 0.8125000000000000000, 0.8144531250000000000, 0.8164062500000000000, 0.8183593749999998890, 0.8203125000000000000, 0.8222656250000000000, 0.8242187500000000000, 0.8261718750000000000, 0.8281250000000000000, 0.8300781250000000000, 0.8320312500000000000, 0.8339843750000000000, 0.8359375000000000000, 0.8378906250000000000, 0.8398437500000000000, 0.8417968750000000000, 0.8437500000000000000, 0.8457031250000000000, 0.8476562500000000000, 0.8496093750000000000, 0.8515625000000000000, 0.8535156250000000000, 0.8554687500000000000, 0.8574218750000000000, 0.8593750000000000000, 0.8613281250000000000, 0.8632812500000000000, 0.8652343750000000000, 0.8671875000000000000, 0.8691406250000000000, 0.8710937500000001110, 0.8730468750000000000, 0.8750000000000000000, 0.8769531250000000000, 0.8789062500000000000, 0.8808593750000000000, 0.8828125000000000000, 0.8847656250000000000, 0.8867187500000000000, 0.8886718750000000000, 0.8906250000000000000, 0.8925781250000000000, 0.8945312500000000000, 0.8964843750000000000, 0.8984375000000000000, 0.9003906250000000000, 0.9023437500000000000, 0.9042968750000000000, 0.9062500000000000000, 0.9082031250000000000, 0.9101562500000000000, 0.9121093750000000000, 0.9140625000000000000, 0.9160156250000000000, 0.9179687500000000000, 0.9199218750000000000, 0.9218750000000000000, 0.9238281250000000000, 0.9257812500000000000, 0.9277343750000000000, 0.9296875000000000000, 0.9316406250000000000, 0.9335937500000000000, 0.9355468750000000000, 0.9375000000000000000, 0.9394531249999998890, 0.9414062500000000000, 0.9433593750000000000, 0.9453125000000000000, 0.9472656250000000000, 0.9492187500000000000, 0.9511718750000000000, 0.9531250000000000000, 0.9550781250000000000, 0.9570312500000000000, 0.9589843750000000000, 0.9609375000000000000, 0.9628906250000000000, 0.9648437500000000000, 0.9667968750000000000, 0.9687500000000000000, 0.9707031250000000000, 0.9726562500000000000, 0.9733142789544542151 ),
 .UNSPECIFIED. ) 
 CURVE ( )  GEOMETRIC_REPRESENTATION_ITEM ( )  RATIONAL_B_SPLINE_CURVE ( ( 1.000000000000000000, 0.9807852804032304306, 1.000000000000000000, 0.9807852804032304306, 1.000000000000000000, 0.9807852804032304306, 1.000000000000000000, 0.9807852804032304306, 1.000000000000000000, 0.9807852804032304306, 1.000000000000000000, 0.9807852804032304306, 1.000000000000000000, 0.9807852804032304306, 1.000000000000000000, 0.9807852804032304306, 1.000000000000000000, 0.9807852804032304306, 1.000000000000000000, 0.9807852804032304306, 1.000000000000000000, 0.9807852804032304306, 1.000000000000000000, 0.9807852804032304306, 1.000000000000000000, 0.9807852804032304306, 1.000000000000000000, 0.9807852804032304306, 1.000000000000000000, 0.9807852804032304306, 1.000000000000000000, 0.9807852804032304306, 1.000000000000000000, 0.9807852804032304306, 1.000000000000000000, 0.9807852804032304306, 1.000000000000000000, 0.9807852804032304306, 1.000000000000000000, 0.9807852804032304306, 1.000000000000000000, 0.9807852804032304306, 1.000000000000000000, 0.9807852804032304306, 1.000000000000000000, 0.9807852804032304306, 1.000000000000000000, 0.9807852804032304306, 1.000000000000000000, 0.9807852804032304306, 1.000000000000000000, 0.9807852804032304306, 1.000000000000000000, 0.9807852804032304306, 1.000000000000000000, 0.9807852804032304306, 1.000000000000000000, 0.9807852804032304306, 1.000000000000000000, 0.9807852804032304306, 1.000000000000000000, 0.9807852804032304306, 1.000000000000000000, 0.9807852804032304306, 1.000000000000000000, 0.9807852804032304306, 1.000000000000000000, 0.9807852804032304306, 1.000000000000000000, 0.9807852804032304306, 1.000000000000000000, 0.9807852804032304306, 1.000000000000000000, 0.9807852804032304306, 1.000000000000000000, 0.9807852804032304306, 1.000000000000000000, 0.9807852804032304306, 1.000000000000000000, 0.9807852804032304306, 1.000000000000000000, 0.9807852804032304306, 1.000000000000000000, 0.9807852804032304306, 1.000000000000000000, 0.9807852804032304306, 1.000000000000000000, 0.9807852804032304306, 1.000000000000000000, 0.9807852804032304306, 1.000000000000000000, 0.9807852804032304306, 1.000000000000000000, 0.9807852804032304306, 1.000000000000000000, 0.9807852804032304306, 1.000000000000000000, 0.9807852804032304306, 1.000000000000000000, 0.9807852804032304306, 1.000000000000000000, 0.9807852804032304306, 1.000000000000000000, 0.9807852804032304306, 1.000000000000000000, 0.9807852804032304306, 1.000000000000000000, 0.9807852804032304306, 1.000000000000000000, 0.9807852804032304306, 1.000000000000000000, 0.9807852804032304306, 1.000000000000000000, 0.9807852804032304306, 1.000000000000000000, 0.9807852804032304306, 1.000000000000000000, 0.9807852804032304306, 1.000000000000000000, 0.9807852804032304306, 1.000000000000000000, 0.9807852804032304306, 1.000000000000000000, 0.9807852804032304306, 1.000000000000000000, 0.9807852804032304306, 1.000000000000000000, 0.9807852804032304306, 1.000000000000000000, 0.9807852804032304306, 1.000000000000000000, 0.9807852804032304306, 1.000000000000000000, 0.9807852804032304306, 1.000000000000000000, 0.9807852804032304306, 1.000000000000000000, 0.9807852804032304306, 1.000000000000000000, 0.9807852804032304306, 1.000000000000000000, 0.9807852804032304306, 1.000000000000000000, 0.9807852804032304306, 1.000000000000000000, 0.9807852804032304306, 1.000000000000000000, 0.9807852804032304306, 1.000000000000000000, 0.9807852804032304306, 1.000000000000000000, 0.9807852804032304306, 1.000000000000000000, 0.9807852804032304306, 1.000000000000000000, 0.9807852804032304306, 1.000000000000000000, 0.9807852804032304306, 1.000000000000000000, 0.9807852804032304306, 1.000000000000000000, 0.9807852804032304306, 1.000000000000000000, 0.9807852804032304306, 1.000000000000000000, 0.9807852804032304306, 1.000000000000000000, 0.9807852804032304306, 1.000000000000000000, 0.9807852804032304306, 1.000000000000000000, 0.9807852804032304306, 1.000000000000000000, 0.9807852804032304306, 1.000000000000000000, 0.9807852804032304306, 1.000000000000000000, 0.9807852804032304306, 1.000000000000000000, 0.9807852804032304306, 1.000000000000000000, 0.9807852804032304306, 1.000000000000000000, 0.9807852804032304306, 1.000000000000000000, 0.9807852804032304306, 1.000000000000000000, 0.9807852804032304306, 1.000000000000000000, 0.9807852804032304306, 1.000000000000000000, 0.9807852804032304306, 1.000000000000000000, 0.9807852804032304306, 1.000000000000000000, 0.9807852804032304306, 1.000000000000000000, 0.9807852804032304306, 1.000000000000000000, 0.9807852804032304306, 1.000000000000000000, 0.9807852804032304306, 1.000000000000000000, 0.9807852804032304306, 1.000000000000000000, 0.9807852804032304306, 1.000000000000000000, 0.9807852804032304306, 1.000000000000000000, 0.9807852804032304306, 1.000000000000000000, 0.9807852804032304306, 1.000000000000000000, 0.9807852804032304306, 1.000000000000000000, 0.9807852804032304306, 1.000000000000000000, 0.9807852804032304306, 1.000000000000000000, 0.9807852804032304306, 1.000000000000000000, 0.9807852804032304306, 1.000000000000000000, 0.9807852804032304306, 1.000000000000000000, 0.9807852804032304306, 1.000000000000000000, 0.9807852804032304306, 1.000000000000000000, 0.9807852804032304306, 1.000000000000000000, 0.9807852804032304306, 1.000000000000000000, 0.9807852804032304306, 1.000000000000000000, 0.9807852804032304306, 1.000000000000000000, 0.9807852804032304306, 1.000000000000000000, 0.9807852804032304306, 1.000000000000000000, 0.9807852804032304306, 1.000000000000000000, 0.9807852804032304306, 1.000000000000000000, 0.9807852804032304306, 1.000000000000000000, 0.9807852804032304306, 1.000000000000000000, 0.9807852804032304306, 1.000000000000000000, 0.9807852804032304306, 1.000000000000000000, 0.9807852804032304306, 1.000000000000000000, 0.9807852804032304306, 1.000000000000000000, 0.9807852804032304306, 1.000000000000000000, 0.9807852804032304306, 1.000000000000000000, 0.9807852804032304306, 1.000000000000000000, 0.9807852804032304306, 1.000000000000000000, 0.9807852804032304306, 1.000000000000000000, 0.9807852804032304306, 1.000000000000000000, 0.9807852804032304306, 1.000000000000000000, 0.9807852804032304306, 1.000000000000000000, 0.9807852804032304306, 1.000000000000000000, 0.9807852804032304306, 1.000000000000000000, 0.9807852804032304306, 1.000000000000000000, 0.9807852804032304306, 1.000000000000000000, 0.9807852804032304306, 1.000000000000000000, 0.9807852804032304306, 1.000000000000000000, 0.9807852804032304306, 1.000000000000000000, 0.9807852804032304306, 1.000000000000000000, 0.9807852804032304306, 1.000000000000000000, 0.9807852804032304306, 1.000000000000000000, 0.9807852804032304306, 1.000000000000000000, 0.9807852804032304306, 1.000000000000000000, 0.9807852804032304306, 1.000000000000000000, 0.9807852804032304306, 1.000000000000000000, 0.9807852804032304306, 1.000000000000000000, 0.9807852804032304306, 1.000000000000000000, 0.9807852804032304306, 1.000000000000000000, 0.9807852804032304306, 1.000000000000000000, 0.9807852804032304306, 1.000000000000000000, 0.9807852804032304306, 1.000000000000000000, 0.9807852804032304306, 1.000000000000000000, 0.9807852804032304306, 1.000000000000000000, 0.9807852804032304306, 1.000000000000000000, 0.9807852804032304306, 1.000000000000000000, 0.9807852804032304306, 1.000000000000000000, 0.9807852804032304306, 1.000000000000000000, 0.9807852804032304306, 1.000000000000000000, 0.9807852804032304306, 1.000000000000000000, 0.9807852804032304306, 1.000000000000000000, 0.9807852804032304306, 1.000000000000000000, 0.9807852804032304306, 1.000000000000000000, 0.9807852804032304306, 1.000000000000000000, 0.9807852804032304306, 1.000000000000000000, 0.9807852804032304306, 1.000000000000000000, 0.9807852804032304306, 1.000000000000000000, 0.9807852804032304306, 1.000000000000000000, 0.9807852804032304306, 1.000000000000000000, 0.9807852804032304306, 1.000000000000000000, 0.9807852804032304306, 1.000000000000000000, 0.9807852804032304306, 1.000000000000000000, 0.9807852804032304306, 1.000000000000000000, 0.9807852804032304306, 1.000000000000000000, 0.9807852804032304306, 1.000000000000000000, 0.9807852804032304306, 1.000000000000000000, 0.9807852804032304306, 1.000000000000000000, 0.9807852804032304306, 1.000000000000000000, 0.9807852804032304306, 1.000000000000000000, 0.9807852804032304306, 1.000000000000000000, 0.9807852804032304306, 1.000000000000000000, 0.9807852804032304306, 1.000000000000000000, 0.9807852804032304306, 1.000000000000000000, 0.9807852804032304306, 1.000000000000000000, 0.9807852804032304306, 1.000000000000000000, 0.9807852804032304306, 1.000000000000000000, 0.9807852804032304306, 1.000000000000000000, 0.9807852804032304306, 1.000000000000000000, 0.9807852804032304306, 1.000000000000000000, 0.9807852804032304306, 1.000000000000000000, 0.9807852804032304306, 1.000000000000000000, 0.9807852804032304306, 1.000000000000000000, 0.9807852804032304306, 1.000000000000000000, 0.9807852804032304306, 1.000000000000000000, 0.9807852804032304306, 1.000000000000000000, 0.9807852804032304306, 1.000000000000000000, 0.9807852804032304306, 1.000000000000000000, 0.9807852804032304306, 1.000000000000000000, 0.9807852804032304306, 1.000000000000000000, 0.9807852804032304306, 1.000000000000000000, 0.9807852804032304306, 1.000000000000000000, 0.9807852804032304306, 1.000000000000000000, 0.9807852804032304306, 1.000000000000000000, 0.9807852804032304306, 1.000000000000000000, 0.9807852804032304306, 1.000000000000000000, 0.9807852804032304306, 1.000000000000000000, 0.9807852804032304306, 1.000000000000000000, 0.9807852804032304306, 1.000000000000000000, 0.9807852804032304306, 1.000000000000000000, 0.9807852804032304306, 1.000000000000000000, 0.9807852804032304306, 1.000000000000000000, 0.9807852804032304306, 1.000000000000000000, 0.9807852804032304306, 1.000000000000000000, 0.9807852804032304306, 1.000000000000000000, 0.9807852804032304306, 1.000000000000000000, 0.9807852804032304306, 1.000000000000000000, 0.9807852804032304306, 1.000000000000000000, 0.9807852804032304306, 1.000000000000000000, 0.9807852804032304306, 1.000000000000000000, 0.9807852804032304306, 1.000000000000000000, 0.9807852804032304306, 1.000000000000000000, 0.9807852804032304306, 1.000000000000000000, 0.9807852804032304306, 1.000000000000000000, 0.9807852804032304306, 1.000000000000000000, 0.9807852804032304306, 1.000000000000000000, 0.9807852804032304306, 1.000000000000000000, 0.9807852804032304306, 1.000000000000000000, 0.9807852804032304306, 1.000000000000000000, 0.9807852804032304306, 1.000000000000000000, 0.9807852804032304306, 1.000000000000000000, 0.9807852804032304306, 1.000000000000000000, 0.9807852804032304306, 1.000000000000000000, 0.9807852804032304306, 1.000000000000000000, 0.9807852804032304306, 1.000000000000000000, 0.9807852804032304306, 1.000000000000000000, 0.9807852804032304306, 1.000000000000000000, 0.9807852804032304306, 1.000000000000000000, 0.9807852804032304306, 1.000000000000000000, 0.9807852804032304306, 1.000000000000000000, 0.9807852804032304306, 1.000000000000000000, 0.9807852804032304306, 1.000000000000000000, 0.9807852804032304306, 1.000000000000000000, 0.9807852804032304306, 1.000000000000000000, 0.9807852804032304306, 1.000000000000000000, 0.9807852804032304306, 1.000000000000000000, 0.9807852804032304306, 1.000000000000000000, 0.9807852804032304306, 1.000000000000000000, 0.9807852804032304306, 1.000000000000000000, 0.9807852804032304306, 1.000000000000000000, 0.9807852804032304306, 1.000000000000000000, 0.9807852804032304306, 1.000000000000000000, 0.9807852804032304306, 1.000000000000000000, 0.9807852804032304306, 1.000000000000000000, 0.9807852804032304306, 1.000000000000000000, 0.9807852804032304306, 1.000000000000000000, 0.9807852804032304306, 1.000000000000000000, 0.9807852804032304306, 1.000000000000000000, 0.9807852804032304306, 1.000000000000000000, 0.9807852804032304306, 1.000000000000000000, 0.9807852804032304306, 1.000000000000000000, 0.9807852804032304306, 1.000000000000000000, 0.9807852804032304306, 1.000000000000000000, 0.9807852804032304306, 1.000000000000000000, 0.9807852804032304306, 1.000000000000000000, 0.9807852804032304306, 1.000000000000000000, 0.9807852804032304306, 1.000000000000000000, 0.9807852804032304306, 1.000000000000000000, 0.9807852804032304306, 1.000000000000000000, 0.9807852804032304306, 1.000000000000000000, 0.9807852804032304306, 1.000000000000000000, 0.9807852804032304306, 1.000000000000000000, 0.9807852804032304306, 1.000000000000000000, 0.9807852804032304306, 1.000000000000000000, 0.9807852804032304306, 1.000000000000000000, 0.9807852804032304306, 1.000000000000000000, 0.9807852804032304306, 1.000000000000000000, 0.9807852804032304306, 1.000000000000000000, 0.9807852804032304306, 1.000000000000000000, 0.9807852804032304306, 1.000000000000000000, 0.9807852804032304306, 1.000000000000000000, 0.9807852804032304306, 1.000000000000000000, 0.9807852804032304306, 1.000000000000000000, 0.9807852804032304306, 1.000000000000000000, 0.9807852804032304306, 1.000000000000000000, 0.9807852804032304306, 1.000000000000000000, 0.9807852804032304306, 1.000000000000000000, 0.9807852804032304306, 1.000000000000000000, 0.9807852804032304306, 1.000000000000000000, 0.9807852804032304306, 1.000000000000000000, 0.9807852804032304306, 1.000000000000000000, 0.9807852804032304306, 1.000000000000000000, 0.9807852804032304306, 1.000000000000000000, 0.9807852804032304306, 1.000000000000000000, 0.9807852804032304306, 1.000000000000000000, 0.9807852804032304306, 1.000000000000000000, 0.9807852804032304306, 1.000000000000000000, 0.9807852804032304306, 1.000000000000000000, 0.9807852804032304306, 1.000000000000000000, 0.9807852804032304306, 1.000000000000000000, 0.9807852804032304306, 1.000000000000000000, 0.9807852804032304306, 1.000000000000000000, 0.9807852804032304306, 1.000000000000000000, 0.9807852804032304306, 1.000000000000000000, 0.9807852804032304306, 1.000000000000000000, 0.9807852804032304306, 1.000000000000000000, 0.9807852804032304306, 1.000000000000000000, 0.9807852804032304306, 1.000000000000000000, 0.9807852804032304306, 1.000000000000000000, 0.9807852804032304306, 1.000000000000000000, 0.9807852804032304306, 1.000000000000000000, 0.9807852804032304306, 1.000000000000000000, 0.9807852804032304306, 1.000000000000000000, 0.9807852804032304306, 1.000000000000000000, 0.9807852804032304306, 1.000000000000000000, 0.9807852804032304306, 1.000000000000000000, 0.9807852804032304306, 1.000000000000000000, 0.9807852804032304306, 1.000000000000000000, 0.9807852804032304306, 1.000000000000000000, 0.9807852804032304306, 1.000000000000000000, 0.9807852804032304306, 1.000000000000000000, 0.9807852804032304306, 1.000000000000000000, 0.9807852804032304306, 1.000000000000000000, 0.9807852804032304306, 1.000000000000000000, 0.9807852804032304306, 1.000000000000000000, 0.9807852804032304306, 1.000000000000000000, 0.9807852804032304306, 1.000000000000000000, 0.9807852804032304306, 1.000000000000000000, 0.9807852804032304306, 1.000000000000000000, 0.9807852804032304306, 1.000000000000000000, 0.9807852804032304306, 1.000000000000000000, 0.9807852804032304306, 1.000000000000000000, 0.9807852804032304306, 1.000000000000000000, 0.9807852804032304306, 1.000000000000000000, 0.9807852804032304306, 1.000000000000000000, 0.9807852804032304306, 1.000000000000000000, 0.9807852804032304306, 1.000000000000000000, 0.9807852804032304306, 1.000000000000000000, 0.9807852804032304306, 1.000000000000000000, 0.9807852804032304306, 1.000000000000000000, 0.9807852804032304306, 1.000000000000000000, 0.9807852804032304306, 1.000000000000000000, 0.9807852804032304306, 1.000000000000000000, 0.9807852804032304306, 1.000000000000000000, 0.9807852804032304306, 1.000000000000000000, 0.9807852804032304306, 1.000000000000000000, 0.9807852804032304306, 1.000000000000000000, 0.9807852804032304306, 1.000000000000000000, 0.9807852804032304306, 1.000000000000000000, 0.9807852804032304306, 1.000000000000000000, 0.9807852804032304306, 1.000000000000000000, 0.9807852804032304306, 1.000000000000000000, 0.9807852804032304306, 1.000000000000000000, 0.9807852804032304306, 1.000000000000000000, 0.9807852804032304306, 1.000000000000000000, 0.9807852804032304306, 1.000000000000000000, 0.9807852804032304306, 1.000000000000000000, 0.9807852804032304306, 1.000000000000000000, 0.9807852804032304306, 1.000000000000000000, 0.9807852804032304306, 1.000000000000000000, 0.9807852804032304306, 1.000000000000000000, 0.9807852804032304306, 1.000000000000000000, 0.9807852804032304306, 1.000000000000000000, 0.9807852804032304306, 1.000000000000000000, 0.9807852804032304306, 1.000000000000000000, 0.9807852804032304306, 1.000000000000000000, 0.9807852804032304306, 1.000000000000000000, 0.9807852804032304306, 1.000000000000000000, 0.9807852804032304306, 1.000000000000000000, 0.9807852804032304306, 1.000000000000000000, 0.9807852804032304306, 1.000000000000000000, 0.9807852804032304306, 1.000000000000000000, 0.9807852804032304306, 1.000000000000000000, 0.9807852804032304306, 1.000000000000000000, 0.9807852804032304306, 1.000000000000000000, 0.9807852804032304306, 1.000000000000000000, 0.9807852804032304306, 1.000000000000000000, 0.9807852804032304306, 1.000000000000000000, 0.9807852804032304306, 1.000000000000000000, 0.9807852804032304306, 1.000000000000000000, 0.9807852804032304306, 1.000000000000000000, 0.9807852804032304306, 1.000000000000000000, 0.9807852804032304306, 1.000000000000000000, 0.9807852804032304306, 1.000000000000000000, 0.9807852804032304306, 1.000000000000000000, 0.9807852804032304306, 1.000000000000000000, 0.9807852804032304306, 1.000000000000000000, 0.9807852804032304306, 1.000000000000000000, 0.9807852804032304306, 1.000000000000000000, 0.9807852804032304306, 1.000000000000000000, 0.9807852804032304306, 1.000000000000000000, 0.9807852804032304306, 1.000000000000000000, 0.9807852804032304306, 1.000000000000000000, 0.9807852804032304306, 1.000000000000000000, 0.9807852804032304306, 1.000000000000000000, 0.9807852804032304306, 1.000000000000000000, 0.9807852804032304306, 1.000000000000000000, 0.9807852804032304306, 1.000000000000000000, 0.9807852804032304306, 1.000000000000000000, 0.9807852804032304306, 1.000000000000000000, 0.9807852804032304306, 1.000000000000000000, 0.9807852804032304306, 1.000000000000000000, 0.9807852804032304306, 1.000000000000000000, 0.9807852804032304306, 1.000000000000000000, 0.9807852804032304306, 1.000000000000000000, 0.9807852804032304306, 1.000000000000000000, 0.9807852804032304306, 1.000000000000000000, 0.9807852804032304306, 1.000000000000000000, 0.9807852804032304306, 1.000000000000000000, 0.9807852804032304306, 1.000000000000000000, 0.9807852804032304306, 1.000000000000000000, 0.9807852804032304306, 1.000000000000000000, 0.9807852804032304306, 1.000000000000000000, 0.9807852804032304306, 1.000000000000000000, 0.9807852804032304306, 1.000000000000000000, 0.9807852804032304306, 1.000000000000000000, 0.9807852804032304306, 1.000000000000000000, 0.9807852804032304306, 1.000000000000000000, 0.9807852804032304306, 1.000000000000000000, 0.9807852804032304306, 1.000000000000000000, 0.9807852804032304306, 1.000000000000000000, 0.9807852804032304306, 1.000000000000000000, 0.9807852804032304306, 1.000000000000000000, 0.9807852804032304306, 1.000000000000000000, 0.9807852804032304306, 1.000000000000000000, 0.9807852804032304306, 1.000000000000000000, 0.9807852804032304306, 1.000000000000000000, 0.9807852804032304306, 1.000000000000000000, 0.9807852804032304306, 1.000000000000000000, 0.9807852804032304306, 1.000000000000000000, 0.9807852804032304306, 1.000000000000000000, 0.9807852804032304306, 1.000000000000000000, 0.9807852804032304306, 1.000000000000000000, 0.9807852804032304306, 1.000000000000000000, 0.9807852804032304306, 1.000000000000000000, 0.9807852804032304306, 1.000000000000000000, 0.9807852804032304306, 1.000000000000000000, 0.9807852804032304306, 1.000000000000000000, 0.9807852804032304306, 1.000000000000000000, 0.9807852804032304306, 1.000000000000000000, 0.9807852804032304306, 1.000000000000000000, 0.9807852804032304306, 1.000000000000000000, 0.9807852804032304306, 1.000000000000000000, 0.9807852804032304306, 1.000000000000000000, 0.9807852804032304306, 1.000000000000000000, 0.9807852804032304306, 1.000000000000000000, 0.9807852804032304306, 1.000000000000000000, 0.9807852804032304306, 1.000000000000000000, 0.9807852804032304306, 1.000000000000000000, 0.9807852804032304306, 1.000000000000000000, 0.9807852804032304306, 1.000000000000000000, 0.9807852804032304306, 1.000000000000000000, 0.9807852804032304306, 1.000000000000000000, 0.9807852804032304306, 1.000000000000000000, 0.9807852804032304306, 1.000000000000000000, 0.9807852804032304306, 1.000000000000000000, 0.9807852804032304306, 1.000000000000000000, 0.9807852804032304306, 1.000000000000000000, 0.9807852804032304306, 1.000000000000000000, 0.9807852804032304306, 1.000000000000000000, 0.9807852804032304306, 1.000000000000000000, 0.9807852804032304306, 1.000000000000000000, 0.9807852804032304306, 1.000000000000000000, 0.9807852804032304306, 1.000000000000000000, 0.9807852804032304306, 1.000000000000000000, 0.9807852804032304306, 1.000000000000000000, 0.9807852804032304306, 1.000000000000000000, 0.9807852804032304306, 1.000000000000000000, 0.9807852804032304306, 1.000000000000000000, 0.9807852804032304306, 1.000000000000000000, 0.9807852804032304306, 1.000000000000000000, 0.9807852804032304306, 1.000000000000000000, 0.9807852804032304306, 1.000000000000000000, 0.9807852804032304306, 1.000000000000000000, 0.9807852804032304306, 1.000000000000000000, 0.9807852804032304306, 1.000000000000000000, 0.9807852804032304306, 1.000000000000000000, 0.9807852804032304306, 1.000000000000000000, 0.9807852804032304306, 1.000000000000000000, 0.9807852804032304306, 1.000000000000000000, 0.9807852804032304306, 1.000000000000000000, 0.9807852804032304306, 1.000000000000000000, 0.9807852804032304306, 1.000000000000000000, 0.9807852804032304306, 1.000000000000000000, 0.9807852804032304306, 1.000000000000000000, 0.9807852804032304306, 1.000000000000000000, 0.9807852804032304306, 1.000000000000000000, 0.9807852804032304306, 1.000000000000000000, 0.9807852804032304306, 1.000000000000000000, 0.9807852804032304306, 1.000000000000000000, 0.9807852804032304306, 1.000000000000000000, 0.9807852804032304306, 1.000000000000000000, 0.9807852804032304306, 1.000000000000000000, 0.9807852804032304306, 1.000000000000000000, 0.9807852804032304306, 1.000000000000000000, 0.9935263529746467537, 0.9914147894652987070 ) ) 
 REPRESENTATION_ITEM ( '' )  );
#187=CARTESIAN_POINT ( 'NONE',  ( -35.09675569278796559, 521.9948905683720568, -15.47720386886985544 ) ) ;
#189=CARTESIAN_POINT ( 'NONE',  ( -28.68588794268874054, 573.2448905601785327, 0.000000000000000000 ) ) ;
#190=CARTESIAN_POINT ( 'NONE',  ( -45.43829269268871940, 484.1823905683720000, 3.332260488124734632 ) ) ;
#192=CARTESIAN_POINT ( 'NONE',  ( -22.27502019258949417, 496.9948905683720568, 15.47720386886985189 ) ) ;
#194=CARTESIAN_POINT ( 'NONE',  ( -28.68588794268871922, 414.4948905765656377, 19.99999999999999289 ) ) ;
#196=CARTESIAN_POINT ( 'NONE',  ( -28.68588794268870856, 329.7448905601784759, 19.99999999999999289 ) ) ;
#201=CARTESIAN_POINT ( 'NONE',  ( -43.20715004130836689, 201.8397834041948613, -3.766744768033091884 ) ) ;
#202=CARTESIAN_POINT ( 'NONE',  ( -19.19641293061497933, 291.9323905683720568, -14.20200298773971603 ) ) ;
#203=CARTESIAN_POINT ( 'NONE',  ( -36.33955658999053639, 529.1198905601785327, 18.47759065022572500 ) ) ;
#205=CARTESIAN_POINT ( 'NONE',  ( -8.685887942688710339, 262.2448905601784759, -2.449293598294705724E-15 ) ) ;
#207=CARTESIAN_POINT ( 'NONE',  ( -13.20868407381885135, 280.9948905683720000, -6.410867750099233042 ) ) ;
#208=CARTESIAN_POINT ( 'NONE',  ( -28.68588794268873698, 534.7448905601785327, -19.99999999999999289 ) ) ;
#209=CARTESIAN_POINT ( 'NONE',  ( -42.88789093042844769, 496.3073905683721136, 9.489475012073734561 ) ) ;
#213=CARTESIAN_POINT ( 'NONE',  ( -28.68588794268872988, 462.8698905683720000, -16.75240474999999307 ) ) ;
#215=CARTESIAN_POINT ( 'NONE',  ( -14.48388495494898720, 267.9323905683720568, 9.489475012073732785 ) ) ;
#217=CARTESIAN_POINT ( 'NONE',  ( -8.685887942688742314, 573.2448905601785327, 2.449293598294706119E-15 ) ) ;
#218=CARTESIAN_POINT ( 'NONE',  ( -38.17536295476244135, 233.8073905683720284, -14.20200298773971426 ) ) ;
#220=CARTESIAN_POINT ( 'NONE',  ( -48.68588794268869435, 251.6823905765656093, -3.978247347593158345 ) ) ;
#221=CARTESIAN_POINT ( 'NONE',  ( -21.03221929538690205, 310.3698905601784759, 18.47759065022572500 ) ) ;
#222=CARTESIAN_POINT ( 'NONE',  ( -28.68588794268870146, 234.7448905601785043, -19.99999999999999289 ) ) ;
#223=CARTESIAN_POINT ( 'NONE',  ( -8.685887942688726326, 412.2448905601784759, -2.449293598294705724E-15 ) ) ;
#224=CARTESIAN_POINT ( 'NONE',  ( -11.93348319268870839, 258.8698905683720000, -2.051577885510841163E-15 ) ) ;
#225=CARTESIAN_POINT ( 'NONE',  ( -40.53162694259543741, 354.1198905683720568, -11.84573899990672707 ) ) ;
#226=CARTESIAN_POINT ( 'NONE',  ( -48.68588794268865882, 506.9323905601784759, -3.978247347593317773 ) ) ;
#228=CARTESIAN_POINT ( 'NONE',  ( -25.35362745456398770, 416.6823905683720568, 16.75240474999998952 ) ) ;
#231=CARTESIAN_POINT ( 'NONE',  ( -36.33955658999051508, 415.3698905601784759, -18.47759065022572855 ) ) ;
#232=VERTEX_POINT ( 'NONE', #18752 ) ;
#233=ORIENTED_EDGE ( 'NONE', *, *, #12800, .T. ) ;
#235=CARTESIAN_POINT ( 'NONE',  ( -25.35362745456401257, 532.5573905683720568, -16.75240474999999307 ) ) ;
#236=CARTESIAN_POINT ( 'NONE',  ( -28.68588794268870856, 304.7448905601785327, -19.99999999999999289 ) ) ;
#237=CARTESIAN_POINT ( 'NONE',  ( -43.60140439023966508, 209.8858117899327169, -1.618481238659646326 ) ) ;
#238=ORIENTED_EDGE ( 'NONE', *, *, #8071, .F. ) ;
#239=CARTESIAN_POINT ( 'NONE',  ( -45.43829269268870519, 325.0573905683719431, -3.332260488124726638 ) ) ;
#240=ORIENTED_EDGE ( 'NONE', *, *, #13467, .F. ) ;
#241=CARTESIAN_POINT ( 'NONE',  ( -38.17536295476245556, 372.3073905683721136, -14.20200298773971426 ) ) ;
#242=CARTESIAN_POINT ( 'NONE',  ( -40.53162694259543741, 372.6198905683720000, -11.84573899990672707 ) ) ;
#244=CARTESIAN_POINT ( 'NONE',  ( -11.73070664223723902, 296.0573905765655809, 11.32908994701042005 ) ) ;
#246=CARTESIAN_POINT ( 'NONE',  ( -45.43829269268869808, 263.5573905683720000, -3.332260488124726638 ) ) ;
#247=CARTESIAN_POINT ( 'NONE',  ( -47.16347859291445133, 437.8698905601784759, 7.653668647301805628 ) ) ;
#248=EDGE_CURVE ( 'NONE', #20201, #15177, #9669, .T. ) ;
#249=CARTESIAN_POINT ( 'NONE',  ( -16.84014894278199392, 419.1198905683720000, 11.84573899990672530 ) ) ;
#252=LINE ( 'NONE', #16791, #13736 ) ;
#253=CARTESIAN_POINT ( 'NONE',  ( -24.70764059509557597, 514.4323905601785327, -19.99999999999999289 ) ) ;
#254=CARTESIAN_POINT ( 'NONE',  ( -28.68588794268874054, 573.2448905601785327, 0.000000000000000000 ) ) ;
#255=CARTESIAN_POINT ( 'NONE',  ( -17.35679799567829917, 450.6823905601784759, 16.95518130045146421 ) ) ;
#256=CARTESIAN_POINT ( 'NONE',  ( -11.93348319268871727, 320.0573905683720000, 3.332260488124728415 ) ) ;
#257=CARTESIAN_POINT ( 'NONE',  ( -42.88789093042844769, 492.9323905683720568, -9.489475012073736337 ) ) ;
#259=CARTESIAN_POINT ( 'NONE',  ( -40.01497788969914637, 458.8073905601784759, 16.95518130045146776 ) ) ;
#260=CARTESIAN_POINT ( 'NONE',  ( -16.84014894278198327, 300.1198905683720000, -11.84573899990672707 ) ) ;
#263=CARTESIAN_POINT ( 'NONE',  ( -48.68588794268870856, 341.9948905765656377, 0.000000000000000000 ) ) ;
#267=CARTESIAN_POINT ( 'NONE',  ( -35.09675569278795138, 387.2448905683720000, 15.47720386886985366 ) ) ;
#268=FACE_OUTER_BOUND ( 'NONE', #16614, .T. ) ;
#269=CARTESIAN_POINT ( 'NONE',  ( -28.68588794268871922, 416.3698905683720568, 16.75240474999999307 ) ) ;
#270=CARTESIAN_POINT ( 'NONE',  ( -45.43829269268869808, 255.3698905683720000, 0.000000000000000000 ) ) ;
#271=CARTESIAN_POINT ( 'NONE',  ( -35.09675569278795848, 425.7448905683720000, 15.47720386886985366 ) ) ;
#273=LINE ( 'NONE', #3605, #8631 ) ;
#274=CARTESIAN_POINT ( 'NONE',  ( -21.03221929538690915, 365.1198905765656377, 18.47759065022572500 ) ) ;
#277=CARTESIAN_POINT ( 'NONE',  ( -45.43829269268871229, 334.1823905683720000, 3.332260488124734632 ) ) ;
#279=CARTESIAN_POINT ( 'NONE',  ( -16.84014894278200458, 481.6198905683720000, -11.84573899990672707 ) ) ;
#282=CARTESIAN_POINT ( 'NONE',  ( -21.03221929538692692, 520.3698905601785327, 18.47759065022572500 ) ) ;
#283=CARTESIAN_POINT ( 'NONE',  ( -35.09675569278795848, 397.2448905683720568, 15.47720386886985366 ) ) ;
#284=CARTESIAN_POINT ( 'NONE',  ( -48.68588794268886488, 262.3073905765655240, 3.978247347592742678 ) ) ;
#285=CARTESIAN_POINT ( 'NONE',  ( -19.19641293061496512, 228.8073905683720284, 14.20200298773971426 ) ) ;
#286=CARTESIAN_POINT ( 'NONE',  ( -13.20868407381886200, 369.4948905683720568, -6.410867750099233042 ) ) ;
#288=CARTESIAN_POINT ( 'NONE',  ( -11.93348319268874214, 529.1823905683719431, -3.332260488124732856 ) ) ;
#290=CARTESIAN_POINT ( 'NONE',  ( -45.43829269268871940, 445.6823905683720000, 3.332260488124734632 ) ) ;
#291=CARTESIAN_POINT ( 'NONE',  ( -19.19641293061500065, 527.3073905683720568, 14.20200298773971426 ) ) ;
#293=CARTESIAN_POINT ( 'NONE',  ( -42.82802356641968089, 530.7448905765656946, -14.14213562373094746 ) ) ;
#294=CARTESIAN_POINT ( 'NONE',  ( -28.68588794268872988, 481.3698905683720568, -16.75240474999999307 ) ) ;
#295=ORIENTED_EDGE ( 'NONE', *, *, #7360, .T. ) ;
#296=CARTESIAN_POINT ( 'NONE',  ( -35.09675569278797269, 505.7448905683720000, 15.47720386886985366 ) ) ;
#298=CARTESIAN_POINT ( 'NONE',  ( -45.64106924314019409, 422.9323905765656377, 11.32908994701042715 ) ) ;
#301=CARTESIAN_POINT ( 'NONE',  ( -11.73070664223723547, 247.9323905765656377, -11.32908994701042538 ) ) ;
#302=CARTESIAN_POINT ( 'NONE',  ( -36.33955658999052218, 485.3698905601784759, -18.47759065022572855 ) ) ;
#306=CARTESIAN_POINT ( 'NONE',  ( -10.48919683876846420, 223.9102039777117170, -8.480601754011892979 ) ) ;
#307=CARTESIAN_POINT ( 'NONE',  ( -28.68588794268870146, 287.8698905683720568, 16.75240474999999307 ) ) ;
#308=LINE ( 'NONE', #5261, #20260 ) ;
#309=CARTESIAN_POINT ( 'NONE',  ( -42.82802356641965247, 278.4948905601785327, 14.14213562373094923 ) ) ;
#311=( BOUNDED_CURVE ( )  B_SPLINE_CURVE ( 2, ( #7202, #2045, #13619, #18362, #8409, #6891, #16759, #18573, #15242, #5273, #3755, #1946, #8514, #15141, #15354, #8617, #13511 ),
 .UNSPECIFIED., .F., .T. ) 
 B_SPLINE_CURVE_WITH_KNOTS ( ( 3, 2, 2, 2, 2, 2, 2, 2, 3 ),
 ( 0.6093750000000002220, 0.6113281250000002220, 0.6132812500000002220, 0.6152343750000002220, 0.6171875000000002220, 0.6191406250000002220, 0.6210937500000002220, 0.6230468750000002220, 0.6250000000000002220 ),
 .UNSPECIFIED. ) 
 CURVE ( )  GEOMETRIC_REPRESENTATION_ITEM ( )  RATIONAL_B_SPLINE_CURVE ( ( 0.9999999999999977796, 0.9807852804032326510, 1.000000000000000000, 0.9807852804032304306, 1.000000000000000000, 0.9807852804032304306, 1.000000000000000000, 0.9807852804032304306, 1.000000000000000000, 0.9807852804032304306, 1.000000000000000000, 0.9807852804032304306, 1.000000000000000000, 0.9807852804032304306, 1.000000000000000000, 0.9807852804032282101, 1.000000000000002220 ) ) 
 REPRESENTATION_ITEM ( '' )  );
#312=CARTESIAN_POINT ( 'NONE',  ( -42.88789093042842637, 294.4323905683720568, -9.489475012073736337 ) ) ;
#313=VERTEX_POINT ( 'NONE', #1450 ) ;
#314=CARTESIAN_POINT ( 'NONE',  ( -24.70764059509553690, 270.0573905601784759, 19.99999999999998934 ) ) ;
#315=CARTESIAN_POINT ( 'NONE',  ( -40.53162694259545162, 496.6198905683720000, 11.84573899990672885 ) ) ;
#316=ADVANCED_FACE ( 'NONE', ( #2968 ), #17876, .T. ) ;
#318=CARTESIAN_POINT ( 'NONE',  ( -38.17536295476246266, 466.9323905683720568, 14.20200298773971781 ) ) ;
#320=CARTESIAN_POINT ( 'NONE',  ( -11.93348319268871194, 268.5573905683720568, 3.332260488124728415 ) ) ;
#322=CARTESIAN_POINT ( 'NONE',  ( -48.68588794268873698, 573.2448905601785327, 0.000000000000000000 ) ) ;
#325=CARTESIAN_POINT ( 'NONE',  ( -45.43829269268869808, 245.3698905683720568, 0.000000000000000000 ) ) ;
#326=CARTESIAN_POINT ( 'NONE',  ( -32.66413529028186247, 239.8073905765656377, -19.99999999999999289 ) ) ;
#327=CARTESIAN_POINT ( 'NONE',  ( -17.35679799567828141, 310.6823905601784759, 16.95518130045146421 ) ) ;
#328=CARTESIAN_POINT ( 'NONE',  ( -45.64106924314017277, 226.3073905601784759, -11.32908994701042715 ) ) ;
#329=CARTESIAN_POINT ( 'NONE',  ( -11.93348319268871194, 268.5573905683720568, 3.332260488124728415 ) ) ;
#330=CARTESIAN_POINT ( 'NONE',  ( -32.01814843081344719, 367.5573905683721136, 16.75240474999999307 ) ) ;
#331=EDGE_CURVE ( 'NONE', #9067, #11943, #8433, .T. ) ;
#334=CARTESIAN_POINT ( 'NONE',  ( -42.88789093042844058, 412.9323905683720000, -9.489475012073736337 ) ) ;
#337=CARTESIAN_POINT ( 'NONE',  ( -10.20829729246299067, 402.8698905601784759, -7.653668647301794969 ) ) ;
#339=VERTEX_POINT ( 'NONE', #6303 ) ;
#343=CARTESIAN_POINT ( 'NONE',  ( -35.09675569278796559, 533.4948905683720568, -15.47720386886985544 ) ) ;
#345=CARTESIAN_POINT ( 'NONE',  ( -17.35679799567828852, 283.8073905601784190, -16.95518130045146421 ) ) ;
#348=CARTESIAN_POINT ( 'NONE',  ( -14.48388495494899431, 329.4323905683720568, 9.489475012073731008 ) ) ;
#349=VERTEX_POINT ( 'NONE', #11382 ) ;
#350=CARTESIAN_POINT ( 'NONE',  ( -28.68588794268871212, 366.3698905683720568, 16.75240474999999307 ) ) ;
#351=CARTESIAN_POINT ( 'NONE',  ( -19.19641293061498288, 360.4323905683720000, -14.20200298773971603 ) ) ;
#353=CARTESIAN_POINT ( 'NONE',  ( -28.68588794268870501, 294.4948905765656377, 19.99999999999999289 ) ) ;
#354=FACE_OUTER_BOUND ( 'NONE', #1771, .T. ) ;
#355=CARTESIAN_POINT ( 'NONE',  ( -19.19641293061496512, 257.3073905683720568, 14.20200298773971426 ) ) ;
#356=CARTESIAN_POINT ( 'NONE',  ( -8.685887942688868435, 466.6823905765656377, 3.978247347593479866 ) ) ;
#357=CARTESIAN_POINT ( 'NONE',  ( -45.43829269268871229, 415.0573905683721136, -3.332260488124726194 ) ) ;
#358=DIRECTION ( 'NONE',  ( -1.000000000000000000, 0.000000000000000000, 0.000000000000000000 ) ) ;
#360=CARTESIAN_POINT ( 'NONE',  ( -48.68588794268887199, 272.3073905765655809, 3.978247347592742678 ) ) ;
#361=CARTESIAN_POINT ( 'NONE',  ( -14.54375231895777176, 410.9948905601785327, 14.14213562373094568 ) ) ;
#362=CARTESIAN_POINT ( 'NONE',  ( -22.27502019258948351, 332.2448905683720568, -15.47720386886985544 ) ) ;
#363=CARTESIAN_POINT ( 'NONE',  ( -32.01814843081346140, 466.0573905683720000, 16.75240474999999307 ) ) ;
#365=CARTESIAN_POINT ( 'NONE',  ( -8.685887942688736985, 471.9323905601784759, 3.978247347593161010 ) ) ;
#366=CARTESIAN_POINT ( 'NONE',  ( -19.19641293061497578, 297.3073905683720568, 14.20200298773971426 ) ) ;
#368=VERTEX_POINT ( 'NONE', #4369 ) ;
#369=CARTESIAN_POINT ( 'NONE',  ( -10.20829729246298356, 341.6198905601784759, 7.653668647301790529 ) ) ;
#370=CARTESIAN_POINT ( 'NONE',  ( -25.35362745456399480, 392.5573905683720000, -16.75240474999999307 ) ) ;
#371=CARTESIAN_POINT ( 'NONE',  ( -11.73070664223725679, 446.0573905765656377, 11.32908994701042005 ) ) ;
#372=CARTESIAN_POINT ( 'NONE',  ( -42.88789093042844058, 432.9323905683720000, -9.489475012073736337 ) ) ;
#373=CARTESIAN_POINT ( 'NONE',  ( -16.84014894278197616, 251.6198905683720284, -11.84573899990672707 ) ) ;
#374=CARTESIAN_POINT ( 'NONE',  ( -35.09675569278795138, 421.9948905683720000, -15.47720386886985544 ) ) ;
#378=CARTESIAN_POINT ( 'NONE',  ( -48.68588794268870856, 361.9948905765655809, 0.000000000000000000 ) ) ;
#380=CARTESIAN_POINT ( 'NONE',  ( -8.685887942688742314, 573.2448905601785327, 2.449293598294706119E-15 ) ) ;
#381=CARTESIAN_POINT ( 'NONE',  ( -44.16309181155856578, 334.4948905683720568, 6.410867750099241924 ) ) ;
#382=DIRECTION ( 'NONE',  ( -1.191790137725560488E-16, 1.000000000000000000, -0.000000000000000000 ) ) ;
#383=CARTESIAN_POINT ( 'NONE',  ( -38.17536295476246266, 486.9323905683721136, 14.20200298773971781 ) ) ;
#384=ADVANCED_FACE ( 'NONE', ( #21025 ), #9547, .F. ) ;
#388=EDGE_CURVE ( 'NONE', #12297, #573, #12170, .T. ) ;
#391=CARTESIAN_POINT ( 'NONE',  ( -45.43829269268871229, 385.3698905683720568, 0.000000000000000000 ) ) ;
#394=CARTESIAN_POINT ( 'NONE',  ( -8.685887942688742314, 532.2448905601784190, -2.449293598294705724E-15 ) ) ;
#395=CARTESIAN_POINT ( 'NONE',  ( -11.93348319268872260, 368.8698905683720000, -2.051577885510841163E-15 ) ) ;
#397=CARTESIAN_POINT ( 'NONE',  ( -38.17536295476246977, 525.4323905683720568, 14.20200298773971781 ) ) ;
#398=ORIENTED_EDGE ( 'NONE', *, *, #15446, .F. ) ;
#400=CARTESIAN_POINT ( 'NONE',  ( -25.35362745456400191, 526.6823905683720568, 16.75240474999998952 ) ) ;
#401=EDGE_CURVE ( 'NONE', #17928, #21047, #11338, .T. ) ;
#403=CARTESIAN_POINT ( 'NONE',  ( -40.01497788969913927, 428.8073905601784759, 16.95518130045146776 ) ) ;
#404=CARTESIAN_POINT ( 'NONE',  ( -16.84014894278200103, 487.6198905683720000, 11.84573899990672530 ) ) ;
#406=CARTESIAN_POINT ( 'NONE',  ( -42.88789093042844769, 492.9323905683719431, -9.489475012073734561 ) ) ;
#408=VECTOR ( 'NONE', #5128, 1000.000000000000000 ) ;
#409=CARTESIAN_POINT ( 'NONE',  ( -21.03221929538693047, 418.8698905765655809, -18.47759065022572855 ) ) ;
#410=CARTESIAN_POINT ( 'NONE',  ( -11.73070664223726034, 476.0573905765656377, 11.32908994701042005 ) ) ;
#417=CARTESIAN_POINT ( 'NONE',  ( -32.01814843081344009, 293.1823905683720568, -16.75240474999999307 ) ) ;
#419=CARTESIAN_POINT ( 'NONE',  ( -25.35362745456400191, 452.5573905683720568, -16.75240474999999307 ) ) ;
#420=CARTESIAN_POINT ( 'NONE',  ( -40.01497788969913927, 413.5573905765656377, 16.95518130045146776 ) ) ;
#421=CARTESIAN_POINT ( 'NONE',  ( -25.35362745456398059, 272.5573905683721136, -16.75240474999999307 ) ) ;
#422=ORIENTED_EDGE ( 'NONE', *, *, #2699, .T. ) ;
#425=CARTESIAN_POINT ( 'NONE',  ( -38.17536295476246266, 496.9323905683720568, 14.20200298773971781 ) ) ;
#427=CARTESIAN_POINT ( 'NONE',  ( -22.27502019258948707, 458.4948905683720568, 15.47720386886985189 ) ) ;
#429=CARTESIAN_POINT ( 'NONE',  ( -13.20868407381884779, 258.2448905683720000, 6.410867750099229490 ) ) ;
#432=CARTESIAN_POINT ( 'NONE',  ( -13.20868407381884779, 250.9948905683720284, -6.410867750099233042 ) ) ;
#434=DIRECTION ( 'NONE',  ( -1.191790137725560488E-16, 1.000000000000000000, -0.000000000000000000 ) ) ;
#435=CARTESIAN_POINT ( 'NONE',  ( -11.93348319268871016, 259.1823905683720000, -3.332260488124732856 ) ) ;
#436=CARTESIAN_POINT ( 'NONE',  ( -22.27502019258948707, 362.2448905683720000, -15.47720386886985544 ) ) ;
#437=ADVANCED_FACE ( 'NONE', ( #268 ), #19715, .T. ) ;
#439=CARTESIAN_POINT ( 'NONE',  ( -25.35362745456398770, 406.6823905683720000, 16.75240474999998952 ) ) ;
#441=CARTESIAN_POINT ( 'NONE',  ( -36.33955658999053639, 509.1198905601784759, 18.47759065022572500 ) ) ;
#442=CARTESIAN_POINT ( 'NONE',  ( -45.64106924314019409, 416.3073905601784759, -11.32908994701042715 ) ) ;
#447=CARTESIAN_POINT ( 'NONE',  ( -32.01814843081346851, 527.5573905683720568, 16.75240474999999307 ) ) ;
#448=CARTESIAN_POINT ( 'NONE',  ( -42.82802356641965247, 295.9948905601784759, -14.14213562373094746 ) ) ;
#449=CARTESIAN_POINT ( 'NONE',  ( -47.16347859291443712, 321.3698905765656377, -7.653668647301793193 ) ) ;
#452=CARTESIAN_POINT ( 'NONE',  ( -44.16309181155855867, 315.9948905683720568, 6.410867750099241924 ) ) ;
#453=EDGE_CURVE ( 'NONE', #17091, #12371, #14396, .T. ) ;
#455=CARTESIAN_POINT ( 'NONE',  ( -11.93348319268872260, 339.1823905683720568, -3.332260488124732856 ) ) ;
#456=CARTESIAN_POINT ( 'NONE',  ( -25.35362745456399125, 371.0573905683719431, -16.75240474999999307 ) ) ;
#457=CARTESIAN_POINT ( 'NONE',  ( -36.33955658999050797, 293.8698905765656377, 18.47759065022572500 ) ) ;
#459=CARTESIAN_POINT ( 'NONE',  ( -40.53162694259543031, 272.6198905683720568, -11.84573899990672707 ) ) ;
#460=CARTESIAN_POINT ( 'NONE',  ( -28.68588794268872633, 464.4948905765656377, 19.99999999999999289 ) ) ;
#461=VECTOR ( 'NONE', #11102, 1000.000000000000000 ) ;
#462=CARTESIAN_POINT ( 'NONE',  ( -22.27502019258948351, 418.4948905683720000, 15.47720386886985189 ) ) ;
#465=CARTESIAN_POINT ( 'NONE',  ( -10.20829729246299600, 447.6198905765656377, -7.653668647301794969 ) ) ;
#467=CARTESIAN_POINT ( 'NONE',  ( -16.84014894278198327, 329.1198905683720568, 11.84573899990672530 ) ) ;
#468=CARTESIAN_POINT ( 'NONE',  ( -14.48388495494900852, 467.9323905683721136, 9.489475012073732785 ) ) ;
#470=CARTESIAN_POINT ( 'NONE',  ( -36.33955658999052218, 465.3698905601784759, -18.47759065022572855 ) ) ;
#471=CARTESIAN_POINT ( 'NONE',  ( -13.20868407381885135, 289.4948905683720000, -6.410867750099233042 ) ) ;
#474=CARTESIAN_POINT ( 'NONE',  ( -28.68588794268871212, 344.4948905765656377, 19.99999999999999289 ) ) ;
#477=CARTESIAN_POINT ( 'NONE',  ( -47.16347859291444422, 346.6198905601784190, -7.653668647301793193 ) ) ;
#480=CARTESIAN_POINT ( 'NONE',  ( -25.35362745456398414, 301.0573905683720568, -16.75240474999999307 ) ) ;
#482=CARTESIAN_POINT ( 'NONE',  ( -19.19641293061498644, 391.9323905683720568, -14.20200298773971603 ) ) ;
#484=CARTESIAN_POINT ( 'NONE',  ( -38.17536295476245556, 425.4323905683720000, 14.20200298773971781 ) ) ;
#485=CARTESIAN_POINT ( 'NONE',  ( -40.53162694259542320, 256.6198905683720568, 11.84573899990672885 ) ) ;
#486=CARTESIAN_POINT ( 'NONE',  ( -16.84014894278199392, 417.6198905683720000, 11.84573899990672530 ) ) ;
#488=CARTESIAN_POINT ( 'NONE',  ( -48.68588794268870856, 362.3073905765656377, 3.978247347593168115 ) ) ;
#489=LINE ( 'NONE', #7156, #6873 ) ;
#490=CARTESIAN_POINT ( 'NONE',  ( -19.19641293061497933, 320.4323905683720000, -14.20200298773971603 ) ) ;
#491=CARTESIAN_POINT ( 'NONE',  ( -14.48388495494901385, 481.3073905683720000, -9.489475012073736337 ) ) ;
#497=CARTESIAN_POINT ( 'NONE',  ( -44.16309181155857289, 395.9948905683720568, 6.410867750099241924 ) ) ;
#499=( BOUNDED_CURVE ( )  B_SPLINE_CURVE ( 2, ( #11343, #1515, #13084, #19671, #3244, #5381, #19892, #3874, #13412, #10462, #3766, #13307, #2053, #18372, #16664, #5070, #11672 ),
 .UNSPECIFIED., .F., .T. ) 
 B_SPLINE_CURVE_WITH_KNOTS ( ( 3, 2, 2, 2, 2, 2, 2, 2, 3 ),
 ( 0.7968750000000002220, 0.7988281250000002220, 0.8007812500000002220, 0.8027343750000002220, 0.8046875000000002220, 0.8066406250000002220, 0.8085937500000002220, 0.8105468750000002220, 0.8125000000000002220 ),
 .UNSPECIFIED. ) 
 CURVE ( )  GEOMETRIC_REPRESENTATION_ITEM ( )  RATIONAL_B_SPLINE_CURVE ( ( 0.9999999999999977796, 0.9807852804032326510, 1.000000000000000000, 0.9807852804032304306, 1.000000000000000000, 0.9807852804032304306, 1.000000000000000000, 0.9807852804032304306, 1.000000000000000000, 0.9807852804032304306, 1.000000000000000000, 0.9807852804032304306, 1.000000000000000000, 0.9807852804032304306, 1.000000000000000000, 0.9807852804032282101, 1.000000000000002220 ) ) 
 REPRESENTATION_ITEM ( '' )  );
#500=CARTESIAN_POINT ( 'NONE',  ( -17.35679799567831694, 533.8073905601784190, -16.95518130045146421 ) ) ;
#501=CARTESIAN_POINT ( 'NONE',  ( -28.68588794268871212, 346.3698905683720568, 16.75240474999999307 ) ) ;
#502=VERTEX_POINT ( 'NONE', #1782 ) ;
#503=CARTESIAN_POINT ( 'NONE',  ( -35.09675569278797269, 525.7448905683720568, 15.47720386886985366 ) ) ;
#505=CARTESIAN_POINT ( 'NONE',  ( -44.16309181155859420, 513.2448905683719431, -6.410867750099231266 ) ) ;
#506=ORIENTED_EDGE ( 'NONE', *, *, #5396, .F. ) ;
#507=CARTESIAN_POINT ( 'NONE',  ( -45.64106924314018698, 428.1823905601784190, 11.32908994701042538 ) ) ;
#508=CARTESIAN_POINT ( 'NONE',  ( -40.53162694259545162, 475.1198905683720000, 11.84573899990672885 ) ) ;
#510=CARTESIAN_POINT ( 'NONE',  ( -45.43829269268872650, 494.1823905683720000, 3.332260488124734632 ) ) ;
#511=CARTESIAN_POINT ( 'NONE',  ( -14.54375231895778242, 490.9948905601784759, 14.14213562373094568 ) ) ;
#513=CARTESIAN_POINT ( 'NONE',  ( -32.66413529028188378, 424.1823905765656377, 19.99999999999999289 ) ) ;
#515=CARTESIAN_POINT ( 'NONE',  ( -28.68588794268870501, 299.7448905601784759, 19.99999999999999289 ) ) ;
#516=CARTESIAN_POINT ( 'NONE',  ( -14.54375231895778064, 438.2448905765656377, -14.14213562373094746 ) ) ;
#520=EDGE_CURVE ( 'NONE', #232, #14361, #20193, .T. ) ;
#521=CARTESIAN_POINT ( 'NONE',  ( -42.88789093042842637, 294.4323905683720568, -9.489475012073736337 ) ) ;
#523=CARTESIAN_POINT ( 'NONE',  ( -48.68588794268871567, 437.2448905601785327, 0.000000000000000000 ) ) ;
#524=CARTESIAN_POINT ( 'NONE',  ( -38.17536295476246977, 453.8073905683720568, -14.20200298773971426 ) ) ;
#526=CARTESIAN_POINT ( 'NONE',  ( -11.93348319268871194, 270.6823905683719431, -3.332260488124732856 ) ) ;
#528=CARTESIAN_POINT ( 'NONE',  ( -48.68588794268886488, 267.5573905601783622, 3.978247347592742678 ) ) ;
#529=CARTESIAN_POINT ( 'NONE',  ( -32.01814843081345430, 487.5573905683720568, 16.75240474999999307 ) ) ;
#531=CARTESIAN_POINT ( 'NONE',  ( -22.27502019258949773, 462.2448905683720568, -15.47720386886985544 ) ) ;
#532=CARTESIAN_POINT ( 'NONE',  ( -28.68588794268874054, 573.2448905601785327, 0.000000000000000000 ) ) ;
#533=CARTESIAN_POINT ( 'NONE',  ( -40.53162694259542320, 252.6198905683720284, -11.84573899990672707 ) ) ;
#535=DIRECTION ( 'NONE',  ( -1.000000000000000000, 0.000000000000000000, 0.000000000000000000 ) ) ;
#536=CARTESIAN_POINT ( 'NONE',  ( -17.35679799567830628, 485.4323905765656946, 16.95518130045146421 ) ) ;
#537=CARTESIAN_POINT ( 'NONE',  ( -24.70764059509555111, 390.0573905601784759, 19.99999999999998934 ) ) ;
#538=CARTESIAN_POINT ( 'NONE',  ( -11.93348319268870661, 250.0573905683720000, 3.332260488124728859 ) ) ;
#539=CARTESIAN_POINT ( 'NONE',  ( -42.82802356641966668, 420.7448905765656377, -14.14213562373094746 ) ) ;
#540=CARTESIAN_POINT ( 'NONE',  ( -1.592577856902392952, 222.3338630624045607, -7.432224998792205994 ) ) ;
#541=CARTESIAN_POINT ( 'NONE',  ( -14.48388495494898365, 237.9323905683720000, 9.489475012073732785 ) ) ;
#542=CARTESIAN_POINT ( 'NONE',  ( -35.09675569278794427, 353.4948905683720000, -15.47720386886985544 ) ) ;
#544=CARTESIAN_POINT ( 'NONE',  ( -13.20868407381886378, 398.2448905683720568, 6.410867750099229490 ) ) ;
#545=CARTESIAN_POINT ( 'NONE',  ( -11.73070664223725501, 413.1823905601784190, -11.32908994701042715 ) ) ;
#550=CARTESIAN_POINT ( 'NONE',  ( -38.17536295476247687, 523.8073905683720568, -14.20200298773971426 ) ) ;
#551=CARTESIAN_POINT ( 'NONE',  ( -28.68588794268870146, 279.7448905601784759, 19.99999999999999289 ) ) ;
#552=CARTESIAN_POINT ( 'NONE',  ( -28.68588794268871212, 319.4948905765656377, -19.99999999999999289 ) ) ;
#553=CARTESIAN_POINT ( 'NONE',  ( -11.93348319268871549, 320.3698905683720568, -2.051577885510841163E-15 ) ) ;
#555=CARTESIAN_POINT ( 'NONE',  ( -40.53162694259543741, 352.6198905683720000, -11.84573899990672707 ) ) ;
#556=CARTESIAN_POINT ( 'NONE',  ( -22.27502019258947641, 356.9948905683720000, 15.47720386886985189 ) ) ;
#557=EDGE_CURVE ( 'NONE', #10903, #18972, #18791, .T. ) ;
#558=CARTESIAN_POINT ( 'NONE',  ( -36.33955658999050797, 273.8698905765656377, 18.47759065022572500 ) ) ;
#559=CARTESIAN_POINT ( 'NONE',  ( -48.68588794268873698, 573.2448905601785327, 0.000000000000000000 ) ) ;
#561=CARTESIAN_POINT ( 'NONE',  ( -40.53162694259542320, 262.6198905683720568, -11.84573899990672707 ) ) ;
#562=CARTESIAN_POINT ( 'NONE',  ( -43.20748696942036560, 201.8382954020867999, 3.765466433758052123 ) ) ;
#563=CARTESIAN_POINT ( 'NONE',  ( -13.20868407381886378, 409.7448905683720000, 6.410867750099229490 ) ) ;
#564=CARTESIAN_POINT ( 'NONE',  ( -48.68588794268854514, 336.9323905601784190, -3.978247347593583783 ) ) ;
#565=CARTESIAN_POINT ( 'NONE',  ( -36.33955658999050797, 355.3698905601784759, -18.47759065022572855 ) ) ;
#567=CARTESIAN_POINT ( 'NONE',  ( -44.16309181155856578, 324.7448905683720000, -6.410867750099231266 ) ) ;
#568=CARTESIAN_POINT ( 'NONE',  ( -11.93348319268873325, 459.1823905683720000, -3.332260488124732856 ) ) ;
#569=ORIENTED_EDGE ( 'NONE', *, *, #6635, .T. ) ;
#570=CARTESIAN_POINT ( 'NONE',  ( -45.64106924314020119, 468.1823905601785327, 11.32908994701042715 ) ) ;
#571=CARTESIAN_POINT ( 'NONE',  ( -22.27502019258947996, 290.7448905683720568, -15.47720386886985544 ) ) ;
#573=VERTEX_POINT ( 'NONE', #9099 ) ;
#575=CARTESIAN_POINT ( 'NONE',  ( -45.64106924314018698, 346.3073905601784759, -11.32908994701042715 ) ) ;
#576=CARTESIAN_POINT ( 'NONE',  ( -19.19641293061497933, 310.4323905683720568, -14.20200298773971603 ) ) ;
#578=CARTESIAN_POINT ( 'NONE',  ( -45.43829269268871229, 375.6823905683720000, 3.332260488124734632 ) ) ;
#580=CARTESIAN_POINT ( 'NONE',  ( -24.70764059509552979, 230.0573905601784759, 19.99999999999998934 ) ) ;
#582=CARTESIAN_POINT ( 'NONE',  ( -10.20829729246300666, 527.6198905765656946, -7.653668647301794969 ) ) ;
#583=CARTESIAN_POINT ( 'NONE',  ( -22.27502019258949062, 400.7448905683720568, -15.47720386886985544 ) ) ;
#584=CARTESIAN_POINT ( 'NONE',  ( -44.16309181155855867, 254.7448905683720284, -6.410867750099231266 ) ) ;
#585=CARTESIAN_POINT ( 'NONE',  ( -38.17536295476246266, 432.3073905683720000, -14.20200298773971426 ) ) ;
#587=CARTESIAN_POINT ( 'NONE',  ( -45.64106924314018698, 342.9323905765655809, 11.32908994701042715 ) ) ;
#589=CARTESIAN_POINT ( 'NONE',  ( -11.93348319268871727, 328.8698905683720000, -2.051577885510841163E-15 ) ) ;
#591=CARTESIAN_POINT ( 'NONE',  ( -44.16309181155857999, 485.9948905683720568, 6.410867750099241924 ) ) ;
#594=CARTESIAN_POINT ( 'NONE',  ( -28.68588794268869435, 224.4948905765656377, 19.99999999999999289 ) ) ;
#597=CARTESIAN_POINT ( 'NONE',  ( -32.01814843081344719, 387.5573905683719431, 16.75240474999999307 ) ) ;
#599=CARTESIAN_POINT ( 'NONE',  ( -40.01497788969915348, 518.8073905601785327, 16.95518130045146776 ) ) ;
#600=CARTESIAN_POINT ( 'NONE',  ( -11.93348319268872260, 339.1823905683720568, -3.332260488124732856 ) ) ;
#603=CARTESIAN_POINT ( 'NONE',  ( -11.93348319268873858, 508.5573905683720000, 3.332260488124728415 ) ) ;
#605=CARTESIAN_POINT ( 'NONE',  ( -43.23114467231988556, 223.9102039777116033, -8.415129624329841462 ) ) ;
#609=CARTESIAN_POINT ( 'NONE',  ( -45.43829269268871940, 473.5573905683720000, -3.332260488124726194 ) ) ;
#611=CARTESIAN_POINT ( 'NONE',  ( -28.68588794268872633, 486.3698905683720568, 16.75240474999999307 ) ) ;
#612=CARTESIAN_POINT ( 'NONE',  ( -24.70764059509553334, 244.8073905765656377, 19.99999999999998934 ) ) ;
#614=CARTESIAN_POINT ( 'NONE',  ( -21.03221929538691626, 415.1198905765656377, 18.47759065022572500 ) ) ;
#620=CARTESIAN_POINT ( 'NONE',  ( -32.66413529028185536, 259.8073905765655809, -19.99999999999999289 ) ) ;
#623=( BOUNDED_CURVE ( )  B_SPLINE_CURVE ( 2, ( #14337, #9648, #9329, #17771, #1236, #2749, #13124, #7910, #16269, #7808, #4893, #11168, #14440, #21020, #2962, #16160, #6190 ),
 .UNSPECIFIED., .F., .T. ) 
 B_SPLINE_CURVE_WITH_KNOTS ( ( 3, 2, 2, 2, 2, 2, 2, 2, 3 ),
 ( 0.03125000000000002776, 0.03320312500000007633, 0.03515625000000012490, 0.03710937500000016653, 0.03906250000000021511, 0.04101562500000026368, 0.04296875000000030531, 0.04492187500000035388, 0.04687500000000040246 ),
 .UNSPECIFIED. ) 
 CURVE ( )  GEOMETRIC_REPRESENTATION_ITEM ( )  RATIONAL_B_SPLINE_CURVE ( ( 0.9999999999999997780, 0.9807852804032306526, 1.000000000000000000, 0.9807852804032304306, 1.000000000000000000, 0.9807852804032304306, 1.000000000000000000, 0.9807852804032304306, 1.000000000000000000, 0.9807852804032304306, 1.000000000000000000, 0.9807852804032304306, 1.000000000000000000, 0.9807852804032304306, 1.000000000000000000, 0.9807852804032264338, 1.000000000000003997 ) ) 
 REPRESENTATION_ITEM ( '' )  );
#624=CARTESIAN_POINT ( 'NONE',  ( -25.35362745456398059, 272.5573905683721136, -16.75240474999999307 ) ) ;
#625=CARTESIAN_POINT ( 'NONE',  ( -24.70764059509555466, 404.8073905765656946, 19.99999999999998934 ) ) ;
#626=CARTESIAN_POINT ( 'NONE',  ( -32.01814843081346140, 453.1823905683720568, -16.75240474999999307 ) ) ;
#627=CARTESIAN_POINT ( 'NONE',  ( -45.64106924314018698, 401.0573905765655809, -11.32908994701042538 ) ) ;
#628=CARTESIAN_POINT ( 'NONE',  ( -22.27502019258947641, 262.2448905683720000, -15.47720386886985544 ) ) ;
#629=VERTEX_POINT ( 'NONE', #10503 ) ;
#630=CARTESIAN_POINT ( 'NONE',  ( -10.20829729246297646, 271.6198905601784759, 7.653668647301790529 ) ) ;
#631=CARTESIAN_POINT ( 'NONE',  ( -28.68588794268873343, 492.8698905683720568, -16.75240474999999307 ) ) ;
#634=CARTESIAN_POINT ( 'NONE',  ( -13.20868407381884779, 268.2448905683720568, 6.410867750099229490 ) ) ;
#635=EDGE_CURVE ( 'NONE', #15132, #11572, #2303, .T. ) ;
#638=CARTESIAN_POINT ( 'NONE',  ( -17.35679799567831338, 488.5573905765656377, -16.95518130045146421 ) ) ;
#640=CARTESIAN_POINT ( 'NONE',  ( -29.83144594096557967, 223.9102039777117170, -18.35382411513653267 ) ) ;
#641=CARTESIAN_POINT ( 'NONE',  ( -19.19641293061496867, 241.9323905683720000, -14.20200298773971603 ) ) ;
#642=CARTESIAN_POINT ( 'NONE',  ( -19.19641293061500420, 521.9323905683720568, -14.20200298773971603 ) ) ;
#643=CARTESIAN_POINT ( 'NONE',  ( -17.35679799567829207, 375.4323905765655809, 16.95518130045146421 ) ) ;
#644=CARTESIAN_POINT ( 'NONE',  ( -25.35362745456396638, 256.6823905683720000, 16.75240474999998952 ) ) ;
#645=CARTESIAN_POINT ( 'NONE',  ( -25.35362745456398770, 342.5573905683720568, -16.75240474999999307 ) ) ;
#646=EDGE_CURVE ( 'NONE', #8266, #13560, #21015, .T. ) ;
#650=CARTESIAN_POINT ( 'NONE',  ( -38.17536295476245556, 405.4323905683721136, 14.20200298773971781 ) ) ;
#652=CARTESIAN_POINT ( 'NONE',  ( -11.73070664223725146, 411.3073905601784759, 11.32908994701042005 ) ) ;
#654=ORIENTED_EDGE ( 'NONE', *, *, #11731, .T. ) ;
#658=CARTESIAN_POINT ( 'NONE',  ( -35.09675569278795848, 503.4948905683720568, -15.47720386886985544 ) ) ;
#659=CARTESIAN_POINT ( 'NONE',  ( -10.20829729246297646, 291.6198905601784759, 7.653668647301790529 ) ) ;
#660=CARTESIAN_POINT ( 'NONE',  ( -43.68588794268869435, 210.1437886375728965, 2.161863591991830530E-19 ) ) ;
#662=EDGE_CURVE ( 'NONE', #19239, #10847, #8186, .T. ) ;
#663=CARTESIAN_POINT ( 'NONE',  ( -22.27502019258948351, 322.2448905683720000, -15.47720386886985544 ) ) ;
#664=CARTESIAN_POINT ( 'NONE',  ( -44.16309181155857289, 343.2448905683720000, -6.410867750099231266 ) ) ;
#665=CARTESIAN_POINT ( 'NONE',  ( -42.88789093042843348, 364.8073905683720568, 9.489475012073734561 ) ) ;
#666=CARTESIAN_POINT ( 'NONE',  ( -48.68588794268870146, 292.3073905765656377, 3.978247347593168115 ) ) ;
#667=CARTESIAN_POINT ( 'NONE',  ( -24.70764059509557597, 499.1823905765655809, -19.99999999999999289 ) ) ;
#668=CARTESIAN_POINT ( 'NONE',  ( -11.93348319268870661, 248.8698905683720000, -2.051577885510841163E-15 ) ) ;
#670=CARTESIAN_POINT ( 'NONE',  ( -14.48388495494900496, 409.4323905683720000, 9.489475012073732785 ) ) ;
#672=CARTESIAN_POINT ( 'NONE',  ( -40.01497788969913927, 335.6823905601785327, -16.95518130045146421 ) ) ;
#675=CARTESIAN_POINT ( 'NONE',  ( -44.16309181155857289, 334.7448905683720568, -6.410867750099231266 ) ) ;
#676=CARTESIAN_POINT ( 'NONE',  ( -38.17536295476246266, 455.4323905683720000, 14.20200298773971781 ) ) ;
#677=ORIENTED_EDGE ( 'NONE', *, *, #8682, .F. ) ;
#678=CARTESIAN_POINT ( 'NONE',  ( -28.68588794268872633, 469.7448905601784759, 19.99999999999999289 ) ) ;
#679=CARTESIAN_POINT ( 'NONE',  ( -35.09675569278793716, 281.9948905683720000, -15.47720386886985544 ) ) ;
#681=CARTESIAN_POINT ( 'NONE',  ( -45.64106924314017988, 338.1823905601784759, 11.32908994701042538 ) ) ;
#682=CARTESIAN_POINT ( 'NONE',  ( -11.93348319268872970, 440.6823905683721136, -3.332260488124732856 ) ) ;
#683=VERTEX_POINT ( 'NONE', #12675 ) ;
#685=CARTESIAN_POINT ( 'NONE',  ( -22.27502019258947996, 290.7448905683720568, -15.47720386886985544 ) ) ;
#687=CARTESIAN_POINT ( 'NONE',  ( -42.88789093042843348, 386.3073905683720000, 9.489475012073734561 ) ) ;
#688=CARTESIAN_POINT ( 'NONE',  ( -21.03221929538692336, 374.1198905601785327, -18.47759065022572855 ) ) ;
#689=CARTESIAN_POINT ( 'NONE',  ( -11.73070664223726922, 517.9323905765655809, -11.32908994701042715 ) ) ;
#690=CARTESIAN_POINT ( 'NONE',  ( -11.93348319268872615, 398.5573905683720568, 3.332260488124728415 ) ) ;
#691=CARTESIAN_POINT ( 'NONE',  ( -11.93348319268870839, 240.0573905683720000, 3.332260488124728415 ) ) ;
#692=CARTESIAN_POINT ( 'NONE',  ( -25.35362745456398770, 426.6823905683720568, 16.75240474999998952 ) ) ;
#693=CARTESIAN_POINT ( 'NONE',  ( -14.54375231895776466, 345.7448905765655809, 14.14213562373094568 ) ) ;
#695=CARTESIAN_POINT ( 'NONE',  ( -25.35362745456397704, 316.6823905683720000, 16.75240474999998952 ) ) ;
#696=DIRECTION ( 'NONE',  ( 1.000000000000000000, 0.000000000000000000, 0.000000000000000000 ) ) ;
#697=CARTESIAN_POINT ( 'NONE',  ( -45.43829269268872650, 485.3698905683720568, 0.000000000000000000 ) ) ;
#699=DIRECTION ( 'NONE',  ( -1.191790137725560488E-16, 1.000000000000000000, -0.000000000000000000 ) ) ;
#701=ADVANCED_FACE ( 'NONE', ( #5959 ), #6064, .T. ) ;
#702=CARTESIAN_POINT ( 'NONE',  ( -22.27502019258947996, 378.4948905683720000, 15.47720386886985189 ) ) ;
#704=CARTESIAN_POINT ( 'NONE',  ( -48.68588794268872988, 517.5573905601784190, 3.978247347593168115 ) ) ;
#705=CARTESIAN_POINT ( 'NONE',  ( -32.01814843081344719, 336.0573905683721136, 16.75240474999999307 ) ) ;
#707=CARTESIAN_POINT ( 'NONE',  ( -28.68588794268873343, 511.3698905683720000, -16.75240474999999307 ) ) ;
#709=CARTESIAN_POINT ( 'NONE',  ( -42.53266943217990104, 223.9102039777116602, -9.520562566242684710 ) ) ;
#712=CARTESIAN_POINT ( 'NONE',  ( -45.64106924314020119, 521.0573905765656946, -11.32908994701042538 ) ) ;
#713=CARTESIAN_POINT ( 'NONE',  ( -25.35362745456399480, 466.6823905683720000, 16.75240474999998952 ) ) ;
#715=CARTESIAN_POINT ( 'NONE',  ( -11.93348319268873503, 478.5573905683721136, 3.332260488124728859 ) ) ;
#716=CARTESIAN_POINT ( 'NONE',  ( -28.68588794268869790, 249.7448905601784475, 19.99999999999999289 ) ) ;
#719=CARTESIAN_POINT ( 'NONE',  ( -48.68588794268871567, 402.3073905765655809, 3.978247347593168115 ) ) ;
#720=CARTESIAN_POINT ( 'NONE',  ( -11.73070664223724258, 297.9323905765655809, -11.32908994701042538 ) ) ;
#724=AXIS2_PLACEMENT_3D ( 'NONE', #8934, #10982, #3964 ) ;
#725=CARTESIAN_POINT ( 'NONE',  ( -45.64106924314016567, 261.0573905765656377, -11.32908994701042538 ) ) ;
#726=CARTESIAN_POINT ( 'NONE',  ( -14.54375231895775222, 240.9948905601784759, 14.14213562373094568 ) ) ;
#729=CARTESIAN_POINT ( 'NONE',  ( -28.68588794268870501, 282.8698905683720568, -16.75240474999999307 ) ) ;
#731=CARTESIAN_POINT ( 'NONE',  ( -40.01497788969912506, 255.6823905601785043, -16.95518130045146421 ) ) ;
#732=CARTESIAN_POINT ( 'NONE',  ( -21.03221929538691626, 405.1198905765656377, 18.47759065022572500 ) ) ;
#734=CARTESIAN_POINT ( 'NONE',  ( -16.84014894278200103, 451.6198905683720568, -11.84573899990672707 ) ) ;
#735=CARTESIAN_POINT ( 'NONE',  ( -24.70764059509555466, 329.1823905765656377, -19.99999999999999289 ) ) ;
#736=CARTESIAN_POINT ( 'NONE',  ( -14.48388495494898720, 261.3073905683720568, -9.489475012073736337 ) ) ;
#737=ORIENTED_EDGE ( 'NONE', *, *, #646, .T. ) ;
#738=CARTESIAN_POINT ( 'NONE',  ( -14.54375231895775755, 248.2448905765656377, -14.14213562373094746 ) ) ;
#740=CARTESIAN_POINT ( 'NONE',  ( -22.27502019258950128, 492.2448905683720000, -15.47720386886985544 ) ) ;
#745=CARTESIAN_POINT ( 'NONE',  ( -38.17536295476244135, 242.3073905683720284, -14.20200298773971426 ) ) ;
#746=ORIENTED_EDGE ( 'NONE', *, *, #17623, .T. ) ;
#747=CARTESIAN_POINT ( 'NONE',  ( -48.68588794268873698, 573.2448905601785327, 0.000000000000000000 ) ) ;
#748=CARTESIAN_POINT ( 'NONE',  ( -11.73070664223725856, 456.0573905765655809, 11.32908994701042005 ) ) ;
#749=CARTESIAN_POINT ( 'NONE',  ( -48.68588794268870146, 327.2448905601785327, 0.000000000000000000 ) ) ;
#752=( BOUNDED_CURVE ( )  B_SPLINE_CURVE ( 2, ( #12930, #11188, #17789, #4383, #17577, #16290, #7615, #7827, #20932, #11078, #9665, #14457, #2981, #9461, #1357, #7929, #14560 ),
 .UNSPECIFIED., .F., .T. ) 
 B_SPLINE_CURVE_WITH_KNOTS ( ( 3, 2, 2, 2, 2, 2, 2, 2, 3 ),
 ( 0.8750000000000002220, 0.8769531250000002220, 0.8789062500000002220, 0.8808593750000002220, 0.8828125000000002220, 0.8847656250000002220, 0.8867187500000002220, 0.8886718750000002220, 0.8906250000000002220 ),
 .UNSPECIFIED. ) 
 CURVE ( )  GEOMETRIC_REPRESENTATION_ITEM ( )  RATIONAL_B_SPLINE_CURVE ( ( 0.9999999999999977796, 0.9807852804032326510, 1.000000000000000000, 0.9807852804032304306, 1.000000000000000000, 0.9807852804032304306, 1.000000000000000000, 0.9807852804032304306, 1.000000000000000000, 0.9807852804032304306, 1.000000000000000000, 0.9807852804032304306, 1.000000000000000000, 0.9807852804032304306, 1.000000000000000000, 0.9807852804032282101, 1.000000000000002220 ) ) 
 REPRESENTATION_ITEM ( '' )  );
#753=CARTESIAN_POINT ( 'NONE',  ( -13.20868407381887799, 519.7448905683720568, 6.410867750099229490 ) ) ;
#755=CARTESIAN_POINT ( 'NONE',  ( -38.17536295476243424, 255.4323905683720284, 14.20200298773971781 ) ) ;
#756=CARTESIAN_POINT ( 'NONE',  ( -44.16309181155856578, 335.9948905683720000, 6.410867750099241924 ) ) ;
#757=CARTESIAN_POINT ( 'NONE',  ( -42.82802356641965247, 318.4948905601784759, 14.14213562373094923 ) ) ;
#758=AXIS2_PLACEMENT_3D ( 'NONE', #6274, #19685, #17847 ) ;
#759=CARTESIAN_POINT ( 'NONE',  ( -28.68588794268870501, 304.4948905765656377, 19.99999999999999289 ) ) ;
#760=CARTESIAN_POINT ( 'NONE',  ( -14.48388495494900496, 399.8073905683720568, -9.489475012073736337 ) ) ;
#761=CARTESIAN_POINT ( 'NONE',  ( -48.68588794268887199, 322.3073905765654672, 3.978247347592742678 ) ) ;
#762=CARTESIAN_POINT ( 'NONE',  ( -40.01497788969913216, 388.8073905601784759, 16.95518130045146776 ) ) ;
#767=CARTESIAN_POINT ( 'NONE',  ( -40.53162694259545162, 504.1198905683720568, -11.84573899990672707 ) ) ;
#770=CARTESIAN_POINT ( 'NONE',  ( -32.01814843081344009, 307.5573905683719431, 16.75240474999999307 ) ) ;
#773=CARTESIAN_POINT ( 'NONE',  ( -45.43829269268870519, 344.1823905683719431, 3.332260488124734632 ) ) ;
#776=CARTESIAN_POINT ( 'NONE',  ( -40.53162694259543741, 345.1198905683720568, 11.84573899990672885 ) ) ;
#778=CARTESIAN_POINT ( 'NONE',  ( -24.70764059509555111, 279.1823905765656377, -19.99999999999999289 ) ) ;
#780=CARTESIAN_POINT ( 'NONE',  ( -25.35362745456397704, 251.0573905683720000, -16.75240474999999307 ) ) ;
#781=CARTESIAN_POINT ( 'NONE',  ( -36.33955658999052929, 463.8698905765656377, 18.47759065022572500 ) ) ;
#782=CARTESIAN_POINT ( 'NONE',  ( -25.35362745456399480, 402.5573905683720000, -16.75240474999999307 ) ) ;
#784=CARTESIAN_POINT ( 'NONE',  ( -8.685887942688632180, 352.5573905601784759, -3.978247347592952732 ) ) ;
#786=CARTESIAN_POINT ( 'NONE',  ( -28.68588794268873343, 509.4948905765655809, -19.99999999999999289 ) ) ;
#787=ADVANCED_FACE ( 'NONE', ( #19771 ), #9521, .T. ) ;
#788=CARTESIAN_POINT ( 'NONE',  ( -44.16309181155857999, 454.4948905683720568, 6.410867750099241924 ) ) ;
#789=ORIENTED_EDGE ( 'NONE', *, *, #4805, .T. ) ;
#791=CARTESIAN_POINT ( 'NONE',  ( -32.66413529028188378, 449.4323905601785327, 19.99999999999999289 ) ) ;
#792=CARTESIAN_POINT ( 'NONE',  ( -22.27502019258946930, 286.9948905683720000, 15.47720386886985189 ) ) ;
#797=CARTESIAN_POINT ( 'NONE',  ( -38.17536295476244135, 305.4323905683720000, 14.20200298773971781 ) ) ;
#798=CARTESIAN_POINT ( 'NONE',  ( -35.09675569278794427, 373.4948905683720568, -15.47720386886985544 ) ) ;
#799=CARTESIAN_POINT ( 'NONE',  ( -36.33955658999050797, 375.3698905601784759, -18.47759065022572855 ) ) ;
#800=CARTESIAN_POINT ( 'NONE',  ( -10.20829729246300488, 516.3698905765656946, 7.653668647301790529 ) ) ;
#801=CARTESIAN_POINT ( 'NONE',  ( -25.35362745456399836, 411.0573905683720568, -16.75240474999999307 ) ) ;
#802=CARTESIAN_POINT ( 'NONE',  ( -11.93348319268870839, 240.6823905683720284, -3.332260488124732856 ) ) ;
#804=CARTESIAN_POINT ( 'NONE',  ( -32.01814843081344719, 411.6823905683720000, -16.75240474999999307 ) ) ;
#805=CARTESIAN_POINT ( 'NONE',  ( -47.16347859291444422, 351.3698905765655809, -7.653668647301793193 ) ) ;
#807=CARTESIAN_POINT ( 'NONE',  ( -16.84014894278197971, 297.6198905683720000, 11.84573899990672530 ) ) ;
#808=CARTESIAN_POINT ( 'NONE',  ( 0.000000000000000000, 0.000000000000000000, 0.000000000000000000 ) ) ;
#809=CARTESIAN_POINT ( 'NONE',  ( -11.93348319268873325, 460.0573905683720568, 3.332260488124728415 ) ) ;
#810=CARTESIAN_POINT ( 'NONE',  ( -28.68588794268874054, 573.2448905601785327, 0.000000000000000000 ) ) ;
#812=CARTESIAN_POINT ( 'NONE',  ( -14.54375231895775045, 225.7448905765656093, 14.14213562373094568 ) ) ;
#813=CARTESIAN_POINT ( 'NONE',  ( -32.01814843081344719, 367.5573905683721136, 16.75240474999999307 ) ) ;
#816=CARTESIAN_POINT ( 'NONE',  ( -42.82802356641968089, 535.9948905601785327, -14.14213562373094746 ) ) ;
#817=CARTESIAN_POINT ( 'NONE',  ( -16.84014894278198327, 337.6198905683720000, 11.84573899990672530 ) ) ;
#819=CARTESIAN_POINT ( 'NONE',  ( -44.16309181155859420, 513.2448905683719431, -6.410867750099231266 ) ) ;
#821=CARTESIAN_POINT ( 'NONE',  ( -42.82802356641965957, 355.9948905601784759, -14.14213562373094746 ) ) ;
#822=CARTESIAN_POINT ( 'NONE',  ( -45.30451366577094063, 223.9102039777116033, -2.213613569785925606 ) ) ;
#825=CARTESIAN_POINT ( 'NONE',  ( -8.685887942688422569, 517.3073905765655809, -3.978247347592394068 ) ) ;
#826=CARTESIAN_POINT ( 'NONE',  ( -25.35362745456400191, 461.0573905683721136, -16.75240474999999307 ) ) ;
#828=CARTESIAN_POINT ( 'NONE',  ( -35.09675569278796559, 465.7448905683720568, 15.47720386886985366 ) ) ;
#829=CARTESIAN_POINT ( 'NONE',  ( -21.03221929538689849, 245.1198905765656377, 18.47759065022572500 ) ) ;
#831=CARTESIAN_POINT ( 'NONE',  ( -36.33955658999051508, 410.1198905765656377, -18.47759065022572855 ) ) ;
#833=DIRECTION ( 'NONE',  ( -1.000000000000000000, 0.000000000000000000, 0.000000000000000000 ) ) ;
#837=CARTESIAN_POINT ( 'NONE',  ( -48.68588794268869435, 261.9948905765655809, 0.000000000000000000 ) ) ;
#838=CARTESIAN_POINT ( 'NONE',  ( -24.70764059509553334, 240.0573905601785043, 19.99999999999998934 ) ) ;
#841=CARTESIAN_POINT ( 'NONE',  ( -42.88789093042842637, 284.4323905683720000, -9.489475012073736337 ) ) ;
#842=CARTESIAN_POINT ( 'NONE',  ( -28.68588794268872633, 452.8698905683720000, -16.75240474999999307 ) ) ;
#843=CARTESIAN_POINT ( 'NONE',  ( -28.68588794268871212, 329.4948905765656377, -19.99999999999999289 ) ) ;
#844=CARTESIAN_POINT ( 'NONE',  ( -45.43829269268869098, 265.0573905683720568, -3.332260488124726194 ) ) ;
#846=LINE ( 'NONE', #7519, #3923 ) ;
#848=CARTESIAN_POINT ( 'NONE',  ( -19.19641293061499354, 478.8073905683720568, 14.20200298773971426 ) ) ;
#850=ORIENTED_EDGE ( 'NONE', *, *, #4862, .F. ) ;
#852=CARTESIAN_POINT ( 'NONE',  ( -22.27502019258946220, 236.9948905683720284, 15.47720386886985189 ) ) ;
#853=ORIENTED_EDGE ( 'NONE', *, *, #17633, .T. ) ;
#856=CARTESIAN_POINT ( 'NONE',  ( -10.20829729246299777, 466.3698905765656377, 7.653668647301790529 ) ) ;
#859=CARTESIAN_POINT ( 'NONE',  ( -32.01814843081343298, 233.1823905683720284, -16.75240474999999307 ) ) ;
#860=CARTESIAN_POINT ( 'NONE',  ( -13.20868407381887977, 520.9948905683720568, -6.410867750099233042 ) ) ;
#863=CARTESIAN_POINT ( 'NONE',  ( -13.20868407381884779, 239.4948905683720284, -6.410867750099233042 ) ) ;
#864=CARTESIAN_POINT ( 'NONE',  ( -11.93348319268871727, 330.3698905683720000, -2.051577885510841163E-15 ) ) ;
#867=EDGE_CURVE ( 'NONE', #17801, #4217, #13526, .T. ) ;
#868=CARTESIAN_POINT ( 'NONE',  ( -32.01814843081345430, 391.6823905683720568, -16.75240474999999307 ) ) ;
#869=CARTESIAN_POINT ( 'NONE',  ( -40.53162694259545873, 534.1198905683720568, -11.84573899990672707 ) ) ;
#870=CARTESIAN_POINT ( 'NONE',  ( -42.82802356641965957, 385.9948905601784759, -14.14213562373094746 ) ) ;
#875=CARTESIAN_POINT ( 'NONE',  ( -22.27502019258949417, 508.4948905683720568, 15.47720386886985189 ) ) ;
#876=CARTESIAN_POINT ( 'NONE',  ( -48.68588794268879383, 292.3073905765656377, 3.978247347592954952 ) ) ;
#879=CARTESIAN_POINT ( 'NONE',  ( -22.27502019258946930, 308.4948905683720568, 15.47720386886985189 ) ) ;
#881=CARTESIAN_POINT ( 'NONE',  ( -38.17536295476244845, 335.4323905683720000, 14.20200298773971781 ) ) ;
#882=CARTESIAN_POINT ( 'NONE',  ( -19.19641293061497578, 337.3073905683720568, 14.20200298773971426 ) ) ;
#883=CARTESIAN_POINT ( 'NONE',  ( -8.685887942688712116, 276.6823905765655809, 3.978247347593161010 ) ) ;
#885=CARTESIAN_POINT ( 'NONE',  ( -11.93348319268870661, 238.5573905683720284, 3.332260488124728859 ) ) ;
#886=CARTESIAN_POINT ( 'NONE',  ( -43.52298375438361688, 200.6544955639567149, 2.225641045960682796 ) ) ;
#888=CARTESIAN_POINT ( 'NONE',  ( -45.43829269268871229, 395.0573905683719431, -3.332260488124726194 ) ) ;
#891=CARTESIAN_POINT ( 'NONE',  ( -14.54375231895778775, 508.2448905765656377, -14.14213562373094746 ) ) ;
#892=CARTESIAN_POINT ( 'NONE',  ( -35.09675569278795848, 435.7448905683720000, 15.47720386886985366 ) ) ;
#894=CARTESIAN_POINT ( 'NONE',  ( -17.35679799567830983, 443.8073905601784759, -16.95518130045146421 ) ) ;
#896=LINE ( 'NONE', #14196, #5632 ) ;
#900=CARTESIAN_POINT ( 'NONE',  ( -28.68588794268870856, 329.7448905601784759, 19.99999999999999289 ) ) ;
#901=CARTESIAN_POINT ( 'NONE',  ( -11.93348319268871549, 299.1823905683720000, -3.332260488124732856 ) ) ;
#902=CARTESIAN_POINT ( 'NONE',  ( -25.35362745456398059, 368.1823905683721136, 16.75240474999998952 ) ) ;
#903=CARTESIAN_POINT ( 'NONE',  ( -8.685887942688724550, 372.2448905601784759, -2.449293598294705724E-15 ) ) ;
#904=CARTESIAN_POINT ( 'NONE',  ( -11.73070664223726745, 526.0573905765656946, 11.32908994701042005 ) ) ;
#905=CARTESIAN_POINT ( 'NONE',  ( -16.84014894278199392, 407.6198905683720568, 11.84573899990672530 ) ) ;
#906=CARTESIAN_POINT ( 'NONE',  ( -13.20868407381884602, 230.9948905683720284, -6.410867750099233042 ) ) ;
#908=CARTESIAN_POINT ( 'NONE',  ( -25.35362745456399836, 411.0573905683720568, -16.75240474999999307 ) ) ;
#911=CARTESIAN_POINT ( 'NONE',  ( -36.33955658999050797, 340.1198905765655809, -18.47759065022572855 ) ) ;
#913=CARTESIAN_POINT ( 'NONE',  ( -44.16309181155855867, 314.4948905683720000, 6.410867750099241924 ) ) ;
#915=CARTESIAN_POINT ( 'NONE',  ( -32.01814843081346140, 467.5573905683721136, 16.75240474999999307 ) ) ;
#916=CARTESIAN_POINT ( 'NONE',  ( -24.70764059509556532, 514.8073905765656946, 19.99999999999998934 ) ) ;
#919=ADVANCED_FACE ( 'NONE', ( #6784 ), #8728, .T. ) ;
#920=CARTESIAN_POINT ( 'NONE',  ( -35.09675569278795138, 367.2448905683720000, 15.47720386886985366 ) ) ;
#921=CARTESIAN_POINT ( 'NONE',  ( -47.16347859291445843, 506.6198905601784190, -7.653668647301793193 ) ) ;
#922=CARTESIAN_POINT ( 'NONE',  ( -45.43829269268870519, 344.1823905683719431, 3.332260488124734632 ) ) ;
#923=EDGE_CURVE ( 'NONE', #13560, #11943, #3445, .T. ) ;
#926=CARTESIAN_POINT ( 'NONE',  ( -45.43829269268872650, 503.8698905683720568, 0.000000000000000000 ) ) ;
#929=CARTESIAN_POINT ( 'NONE',  ( -13.20868407381886556, 419.7448905683720000, 6.410867750099229490 ) ) ;
#930=CARTESIAN_POINT ( 'NONE',  ( -47.16347859291443712, 291.3698905765655809, -7.653668647301793193 ) ) ;
#932=CARTESIAN_POINT ( 'NONE',  ( -44.16309181155858710, 473.2448905683720568, -6.410867750099231266 ) ) ;
#934=CARTESIAN_POINT ( 'NONE',  ( -14.48388495494901029, 467.9323905683721136, 9.489475012073731008 ) ) ;
#935=CARTESIAN_POINT ( 'NONE',  ( -45.64106924314016567, 242.9323905765656377, 11.32908994701042538 ) ) ;
#936=CARTESIAN_POINT ( 'NONE',  ( -24.70764059509555821, 404.8073905765656377, 19.99999999999998934 ) ) ;
#938=CARTESIAN_POINT ( 'NONE',  ( -28.68588794268871567, 369.4948905765656377, -19.99999999999999289 ) ) ;
#943=CARTESIAN_POINT ( 'NONE',  ( -8.685887942688799157, 241.9323905601784475, 3.978247347593374172 ) ) ;
#944=CARTESIAN_POINT ( 'NONE',  ( -35.86044580198795018, 223.9104597372275123, 18.66884633871304899 ) ) ;
#945=CARTESIAN_POINT ( 'NONE',  ( -16.84014894278197971, 281.6198905683720000, -11.84573899990672707 ) ) ;
#946=CARTESIAN_POINT ( 'NONE',  ( -28.68588794268870146, 244.7448905601785043, -19.99999999999999289 ) ) ;
#949=CARTESIAN_POINT ( 'NONE',  ( -40.53162694259544452, 434.1198905683720000, -11.84573899990672707 ) ) ;
#951=CARTESIAN_POINT ( 'NONE',  ( -13.20868407381884779, 250.9948905683720284, -6.410867750099233042 ) ) ;
#955=CARTESIAN_POINT ( 'NONE',  ( -40.53162694259545162, 486.6198905683720000, 11.84573899990672885 ) ) ;
#960=CARTESIAN_POINT ( 'NONE',  ( -14.48388495494898542, 239.8073905683720284, -9.489475012073736337 ) ) ;
#964=CARTESIAN_POINT ( 'NONE',  ( -17.35679799567830628, 465.4323905765656946, 16.95518130045146421 ) ) ;
#966=CARTESIAN_POINT ( 'NONE',  ( -8.685887942688713892, 286.9948905765656377, -2.449293598294705724E-15 ) ) ;
#967=CARTESIAN_POINT ( 'NONE',  ( -26.23092855549762348, 223.9102039777116318, -18.75754572640088114 ) ) ;
#968=CARTESIAN_POINT ( 'NONE',  ( -42.88789093042841927, 226.3073905683720000, 9.489475012073734561 ) ) ;
#969=CARTESIAN_POINT ( 'NONE',  ( -25.35362745456400901, 512.5573905683719431, -16.75240474999999307 ) ) ;
#971=CARTESIAN_POINT ( 'NONE',  ( -40.53162694259542320, 255.1198905683720284, 11.84573899990672885 ) ) ;
#972=CARTESIAN_POINT ( 'NONE',  ( -35.09675569278795138, 337.2448905683720568, 15.47720386886985366 ) ) ;
#974=CARTESIAN_POINT ( 'NONE',  ( -28.68588794268872633, 469.7448905601784759, 19.99999999999999289 ) ) ;
#975=CARTESIAN_POINT ( 'NONE',  ( -48.68588794268870856, 357.2448905601784759, 0.000000000000000000 ) ) ;
#978=CARTESIAN_POINT ( 'NONE',  ( -40.53162694259544452, 392.6198905683720568, -11.84573899990672707 ) ) ;
#980=CARTESIAN_POINT ( 'NONE',  ( -45.64106924314018698, 378.1823905601785327, 11.32908994701042715 ) ) ;
#982=CARTESIAN_POINT ( 'NONE',  ( -8.685887942688726326, 402.2448905601784759, -2.449293598294705724E-15 ) ) ;
#985=CARTESIAN_POINT ( 'NONE',  ( -19.19641293061499709, 498.8073905683720000, 14.20200298773971426 ) ) ;
#986=CARTESIAN_POINT ( 'NONE',  ( -28.68588794268870501, 294.4948905765656377, 19.99999999999999289 ) ) ;
#988=CARTESIAN_POINT ( 'NONE',  ( -28.68588794268870856, 302.8698905683720000, -16.75240474999999307 ) ) ;
#990=CARTESIAN_POINT ( 'NONE',  ( -45.43829269268870519, 333.5573905683720568, -3.332260488124726194 ) ) ;
#991=CARTESIAN_POINT ( 'NONE',  ( -25.35362745456398059, 346.6823905683720568, 16.75240474999998952 ) ) ;
#992=EDGE_CURVE ( 'NONE', #17870, #16862, #20206, .T. ) ;
#993=CARTESIAN_POINT ( 'NONE',  ( -24.70764059509553690, 274.8073905765656377, 19.99999999999998934 ) ) ;
#994=CARTESIAN_POINT ( 'NONE',  ( -32.66413529028188378, 499.8073905765655809, -19.99999999999999289 ) ) ;
#995=CARTESIAN_POINT ( 'NONE',  ( -14.48388495494898365, 247.9323905683720568, 9.489475012073731008 ) ) ;
#996=CARTESIAN_POINT ( 'NONE',  ( -11.93348319268872615, 400.0573905683720568, 3.332260488124728415 ) ) ;
#999=CARTESIAN_POINT ( 'NONE',  ( -42.82802356641964536, 245.9948905601784759, -14.14213562373094746 ) ) ;
#1001=CARTESIAN_POINT ( 'NONE',  ( -40.53162694259545162, 452.6198905683720568, -11.84573899990672707 ) ) ;
#1003=CARTESIAN_POINT ( 'NONE',  ( -36.33955658999051508, 445.3698905601785327, -18.47759065022572855 ) ) ;
#1004=ORIENTED_EDGE ( 'NONE', *, *, #18546, .F. ) ;
#1008=DIRECTION ( 'NONE',  ( -1.000000000000000000, 0.000000000000000000, 0.000000000000000000 ) ) ;
#1009=CARTESIAN_POINT ( 'NONE',  ( -48.68588794268870146, 317.2448905601784759, 0.000000000000000000 ) ) ;
#1010=CARTESIAN_POINT ( 'NONE',  ( -14.48388495494900141, 371.3073905683721136, -9.489475012073734561 ) ) ;
#1012=CARTESIAN_POINT ( 'NONE',  ( -45.64106924314020119, 521.0573905765656946, -11.32908994701042715 ) ) ;
#1013=CARTESIAN_POINT ( 'NONE',  ( -45.43829269268871940, 413.8698905683720568, 0.000000000000000000 ) ) ;
#1014=CARTESIAN_POINT ( 'NONE',  ( -28.68588794268869790, 237.8698905683720568, 16.75240474999999307 ) ) ;
#1015=CARTESIAN_POINT ( 'NONE',  ( -35.09675569278795138, 401.9948905683720568, -15.47720386886985544 ) ) ;
#1018=CARTESIAN_POINT ( 'NONE',  ( -48.68588794268870856, 342.3073905765656946, 3.978247347593168115 ) ) ;
#1020=CARTESIAN_POINT ( 'NONE',  ( -44.16309181155856578, 313.2448905683720000, -6.410867750099231266 ) ) ;
#1021=CARTESIAN_POINT ( 'NONE',  ( -25.35362745456400191, 452.5573905683720568, -16.75240474999999307 ) ) ;
#1025=CARTESIAN_POINT ( 'NONE',  ( -42.88789093042843348, 366.3073905683720000, 9.489475012073736337 ) ) ;
#1026=CARTESIAN_POINT ( 'NONE',  ( -44.16309181155857999, 494.4948905683720568, 6.410867750099241924 ) ) ;
#1027=CARTESIAN_POINT ( 'NONE',  ( -36.33955658999052929, 515.3698905601784190, -18.47759065022572855 ) ) ;
#1028=CARTESIAN_POINT ( 'NONE',  ( -32.01814843081344009, 321.6823905683720568, -16.75240474999999307 ) ) ;
#1031=CARTESIAN_POINT ( 'NONE',  ( -16.84014894278200458, 497.6198905683720000, 11.84573899990672530 ) ) ;
#1034=CARTESIAN_POINT ( 'NONE',  ( -35.09675569278795138, 433.4948905683720568, -15.47720386886985544 ) ) ;
#1036=DIRECTION ( 'NONE',  ( -1.000000000000000000, 0.000000000000000000, 0.000000000000000000 ) ) ;
#1037=CARTESIAN_POINT ( 'NONE',  ( -40.53162694259545162, 465.1198905683720568, 11.84573899990672885 ) ) ;
#1039=CARTESIAN_POINT ( 'NONE',  ( -25.35362745456400191, 461.0573905683720568, -16.75240474999999307 ) ) ;
#1041=EDGE_CURVE ( 'NONE', #14194, #126, #311, .T. ) ;
#1042=CARTESIAN_POINT ( 'NONE',  ( -32.66413529028188378, 399.8073905765656377, -19.99999999999999289 ) ) ;
#1043=CARTESIAN_POINT ( 'NONE',  ( -8.685887942688706786, 226.9948905765656377, -2.449293598294705724E-15 ) ) ;
#1054=CARTESIAN_POINT ( 'NONE',  ( -32.66413529028186247, 245.0573905601785327, -19.99999999999999289 ) ) ;
#1056=CARTESIAN_POINT ( 'NONE',  ( -35.09675569278795848, 427.2448905683720568, 15.47720386886985366 ) ) ;
#1057=CARTESIAN_POINT ( 'NONE',  ( -40.53162694259542320, 246.6198905683720284, 11.84573899990672885 ) ) ;
#1058=ADVANCED_FACE ( 'NONE', ( #20418 ), #5694, .T. ) ;
#1060=ORIENTED_EDGE ( 'NONE', *, *, #18546, .T. ) ;
#1061=PLANE ( 'NONE',  #2719 ) ;
#1063=CARTESIAN_POINT ( 'NONE',  ( -35.09675569278795848, 473.4948905683720000, -15.47720386886985544 ) ) ;
#1065=CARTESIAN_POINT ( 'NONE',  ( -22.27502019258947286, 240.7448905683720000, -15.47720386886985544 ) ) ;
#1067=( BOUNDED_CURVE ( )  B_SPLINE_CURVE ( 2, ( #3378, #11261, #14956, #3054, #6603, #14530, #6390, #21225, #9531, #19491, #6716, #11478, #14853, #9957, #11588, #16149, #21114 ),
 .UNSPECIFIED., .F., .T. ) 
 B_SPLINE_CURVE_WITH_KNOTS ( ( 3, 2, 2, 2, 2, 2, 2, 2, 3 ),
 ( 0.7812500000000001110, 0.7832031250000001110, 0.7851562500000001110, 0.7871093750000001110, 0.7890625000000002220, 0.7910156250000002220, 0.7929687500000002220, 0.7949218750000002220, 0.7968750000000002220 ),
 .UNSPECIFIED. ) 
 CURVE ( )  GEOMETRIC_REPRESENTATION_ITEM ( )  RATIONAL_B_SPLINE_CURVE ( ( 0.9999999999999988898, 0.9807852804032315408, 1.000000000000000000, 0.9807852804032304306, 1.000000000000000000, 0.9807852804032304306, 1.000000000000000000, 0.9807852804032304306, 1.000000000000000000, 0.9807852804032304306, 1.000000000000000000, 0.9807852804032304306, 1.000000000000000000, 0.9807852804032304306, 1.000000000000000000, 0.9807852804032282101, 1.000000000000002220 ) ) 
 REPRESENTATION_ITEM ( '' )  );
#1068=CARTESIAN_POINT ( 'NONE',  ( -13.20868407381887799, 518.2448905683720568, 6.410867750099229490 ) ) ;
#1070=CARTESIAN_POINT ( 'NONE',  ( -42.82802356641967378, 460.7448905765655809, -14.14213562373094746 ) ) ;
#1072=CARTESIAN_POINT ( 'NONE',  ( -14.54375231895775755, 285.7448905765655809, 14.14213562373094568 ) ) ;
#1073=CARTESIAN_POINT ( 'NONE',  ( -40.01497788969915348, 455.6823905601785896, -16.95518130045146421 ) ) ;
#1076=CARTESIAN_POINT ( 'NONE',  ( -22.27502019258946220, 236.9948905683720284, 15.47720386886985189 ) ) ;
#1077=CARTESIAN_POINT ( 'NONE',  ( -35.09675569278795138, 347.2448905683720000, 15.47720386886985366 ) ) ;
#1079=AXIS2_PLACEMENT_3D ( 'NONE', #13026, #13357, #3610 ) ;
#1080=CARTESIAN_POINT ( 'NONE',  ( -17.35679799567828852, 360.6823905601785327, 16.95518130045146421 ) ) ;
#1081=CARTESIAN_POINT ( 'NONE',  ( -19.19641293061497933, 311.9323905683720568, -14.20200298773971603 ) ) ;
#1083=CARTESIAN_POINT ( 'NONE',  ( -28.68588794268871567, 376.3698905683720568, 16.75240474999999307 ) ) ;
#1087=CARTESIAN_POINT ( 'NONE',  ( -47.16347859291445133, 396.6198905601784759, -7.653668647301793193 ) ) ;
#1089=EDGE_LOOP ( 'NONE', ( #10164, #17428, #9305, #19905 ) ) ;
#1091=CARTESIAN_POINT ( 'NONE',  ( -13.20868407381887621, 499.7448905683720000, 6.410867750099229490 ) ) ;
#1092=CARTESIAN_POINT ( 'NONE',  ( -42.82802356641965247, 293.2448905765655809, 14.14213562373094923 ) ) ;
#1094=CARTESIAN_POINT ( 'NONE',  ( -13.20868407381885135, 299.7448905683720568, 6.410867750099229490 ) ) ;
#1096=CARTESIAN_POINT ( 'NONE',  ( -45.43829269268871229, 333.8698905683720000, 0.000000000000000000 ) ) ;
#1098=CARTESIAN_POINT ( 'NONE',  ( -24.70764059509555111, 259.1823905765656377, -19.99999999999999289 ) ) ;
#1099=CARTESIAN_POINT ( 'NONE',  ( -8.685887942688509611, 497.3073905765656377, -3.978247347592607230 ) ) ;
#1100=CARTESIAN_POINT ( 'NONE',  ( -19.19641293061496867, 240.4323905683720000, -14.20200298773971603 ) ) ;
#1101=CARTESIAN_POINT ( 'NONE',  ( -13.20868407381886556, 400.9948905683720568, -6.410867750099233042 ) ) ;
#1102=CARTESIAN_POINT ( 'NONE',  ( -24.70764059509555466, 334.4323905601785327, -19.99999999999999289 ) ) ;
#1103=CYLINDRICAL_SURFACE ( 'NONE', #12822, 19.99999999999999645 ) ;
#1105=CARTESIAN_POINT ( 'NONE',  ( -42.82802356641968089, 510.7448905765656946, -14.14213562373094746 ) ) ;
#1106=CARTESIAN_POINT ( 'NONE',  ( -25.35362745456399125, 436.6823905683720000, 16.75240474999998952 ) ) ;
#1107=VERTEX_POINT ( 'NONE', #10773 ) ;
#1108=CARTESIAN_POINT ( 'NONE',  ( -21.03221929538691981, 440.3698905601784759, 18.47759065022572500 ) ) ;
#1110=ORIENTED_EDGE ( 'NONE', *, *, #12732, .T. ) ;
#1114=CARTESIAN_POINT ( 'NONE',  ( -17.35679799567828852, 330.6823905601785327, 16.95518130045146421 ) ) ;
#1115=CARTESIAN_POINT ( 'NONE',  ( -22.27502019258947641, 358.4948905683720000, 15.47720386886985189 ) ) ;
#1117=CARTESIAN_POINT ( 'NONE',  ( -36.33955658999052218, 500.1198905765655809, -18.47759065022572855 ) ) ;
#1118=CARTESIAN_POINT ( 'NONE',  ( -45.43829269268870519, 384.1823905683720000, 3.332260488124734632 ) ) ;
#1119=CARTESIAN_POINT ( 'NONE',  ( -35.09675569278793006, 243.4948905683720284, -15.47720386886985544 ) ) ;
#1120=CARTESIAN_POINT ( 'NONE',  ( -28.68588794268871922, 401.3698905683720000, -16.75240474999999307 ) ) ;
#1122=CARTESIAN_POINT ( 'NONE',  ( -24.70764059509554755, 324.8073905765656946, 19.99999999999998934 ) ) ;
#1124=CARTESIAN_POINT ( 'NONE',  ( -28.68588794268870856, 301.3698905683720568, -16.75240474999999307 ) ) ;
#1125=CARTESIAN_POINT ( 'NONE',  ( -11.93348319268873148, 450.6823905683721136, -3.332260488124732856 ) ) ;
#1130=CARTESIAN_POINT ( 'NONE',  ( -38.17536295476245556, 363.8073905683720568, -14.20200298773971426 ) ) ;
#1131=CARTESIAN_POINT ( 'NONE',  ( -38.17536295476247687, 512.3073905683719431, -14.20200298773971426 ) ) ;
#1132=CARTESIAN_POINT ( 'NONE',  ( -21.03221929538692692, 500.3698905601785327, 18.47759065022572500 ) ) ;
#1133=CARTESIAN_POINT ( 'NONE',  ( -38.17536295476244135, 315.4323905683720000, 14.20200298773971781 ) ) ;
#1134=EDGE_CURVE ( 'NONE', #18572, #20528, #15669, .T. ) ;
#1139=CARTESIAN_POINT ( 'NONE',  ( -42.88789093042844058, 424.4323905683720568, -9.489475012073734561 ) ) ;
#1140=CARTESIAN_POINT ( 'NONE',  ( -24.70764059509553334, 234.8073905765656377, 19.99999999999998934 ) ) ;
#1142=CARTESIAN_POINT ( 'NONE',  ( -13.20868407381886911, 448.2448905683720000, 6.410867750099229490 ) ) ;
#1144=CARTESIAN_POINT ( 'NONE',  ( -28.68588794268872988, 461.3698905683720000, -16.75240474999999307 ) ) ;
#1147=CARTESIAN_POINT ( 'NONE',  ( -42.82802356641966668, 413.2448905765655809, 14.14213562373094923 ) ) ;
#1154=CARTESIAN_POINT ( 'NONE',  ( -45.11206863185022087, 223.9102039777116033, 6.767993150222416432 ) ) ;
#1156=CARTESIAN_POINT ( 'NONE',  ( -32.66413529028186247, 239.4323905601785043, 19.99999999999999289 ) ) ;
#1157=CYLINDRICAL_SURFACE ( 'NONE', #9190, 19.99999999999999645 ) ;
#1158=CARTESIAN_POINT ( 'NONE',  ( -13.20868407381886733, 420.9948905683720000, -6.410867750099233042 ) ) ;
#1159=CARTESIAN_POINT ( 'NONE',  ( -48.68588794268854514, 386.9323905601785327, -3.978247347593583783 ) ) ;
#1160=CARTESIAN_POINT ( 'NONE',  ( -13.20868407381884602, 249.7448905683720000, 6.410867750099229490 ) ) ;
#1163=CARTESIAN_POINT ( 'NONE',  ( -13.20868407381887444, 470.9948905683720000, -6.410867750099233042 ) ) ;
#1164=CARTESIAN_POINT ( 'NONE',  ( -8.685887942688708563, 236.9948905765656377, -2.449293598294705724E-15 ) ) ;
#1166=CARTESIAN_POINT ( 'NONE',  ( -17.35679799567830983, 525.4323905765656946, 16.95518130045146421 ) ) ;
#1167=CARTESIAN_POINT ( 'NONE',  ( -16.84014894278197616, 250.1198905683720284, -11.84573899990672707 ) ) ;
#1170=CARTESIAN_POINT ( 'NONE',  ( -11.93348319268874214, 528.8698905683719431, -2.051577885510841163E-15 ) ) ;
#1172=CARTESIAN_POINT ( 'NONE',  ( -8.685887942688733432, 456.9948905765656377, -2.449293598294705724E-15 ) ) ;
#1174=DIRECTION ( 'NONE',  ( -1.000000000000000000, 0.000000000000000000, 0.000000000000000000 ) ) ;
#1177=CARTESIAN_POINT ( 'NONE',  ( -19.19641293061496157, 228.8073905683720284, 14.20200298773971426 ) ) ;
#1180=CARTESIAN_POINT ( 'NONE',  ( -40.53162694259542320, 225.1198905683720000, 11.84573899990672885 ) ) ;
#1181=CARTESIAN_POINT ( 'NONE',  ( -32.01814843081344009, 317.5573905683720568, 16.75240474999999307 ) ) ;
#1187=CARTESIAN_POINT ( 'NONE',  ( -40.53162694259543031, 304.1198905683720000, -11.84573899990672707 ) ) ;
#1188=CARTESIAN_POINT ( 'NONE',  ( -25.35362745456399480, 381.0573905683719431, -16.75240474999999307 ) ) ;
#1189=CARTESIAN_POINT ( 'NONE',  ( -44.16309181155858710, 525.9948905683720568, 6.410867750099241924 ) ) ;
#1190=CARTESIAN_POINT ( 'NONE',  ( -21.03221929538692692, 394.1198905601784759, -18.47759065022572855 ) ) ;
#1191=CARTESIAN_POINT ( 'NONE',  ( -48.68588794268860198, 231.6823905765656377, -3.978247347593371508 ) ) ;
#1194=CARTESIAN_POINT ( 'NONE',  ( -38.17536295476246977, 493.8073905683720000, -14.20200298773971426 ) ) ;
#1195=CARTESIAN_POINT ( 'NONE',  ( -17.35679799567828141, 295.4323905765656377, 16.95518130045146421 ) ) ;
#1197=CARTESIAN_POINT ( 'NONE',  ( -42.88789093042842637, 294.4323905683720000, -9.489475012073734561 ) ) ;
#1198=CARTESIAN_POINT ( 'NONE',  ( -13.20868407381885667, 329.4948905683720568, -6.410867750099233042 ) ) ;
#1200=CARTESIAN_POINT ( 'NONE',  ( -28.68588794268870146, 264.4948905765656377, 19.99999999999999289 ) ) ;
#1201=CARTESIAN_POINT ( 'NONE',  ( -48.68588794268872277, 477.2448905601784759, 0.000000000000000000 ) ) ;
#1202=DIRECTION ( 'NONE',  ( -1.191790137725560488E-16, 1.000000000000000000, -0.000000000000000000 ) ) ;
#1203=CARTESIAN_POINT ( 'NONE',  ( -22.27502019258947996, 388.4948905683720000, 15.47720386886985189 ) ) ;
#1204=CARTESIAN_POINT ( 'NONE',  ( -21.03221929538691981, 334.1198905601784759, -18.47759065022572855 ) ) ;
#1207=CARTESIAN_POINT ( 'NONE',  ( -28.68588794268872633, 441.3698905683720000, -16.75240474999999307 ) ) ;
#1208=CYLINDRICAL_SURFACE ( 'NONE', #2725, 19.99999999999999645 ) ;
#1210=CARTESIAN_POINT ( 'NONE',  ( -17.35679799567830273, 440.6823905601785327, 16.95518130045146421 ) ) ;
#1213=VERTEX_POINT ( 'NONE', #2359 ) ;
#1215=CARTESIAN_POINT ( 'NONE',  ( -48.68588794268870146, 327.5573905601784759, 3.978247347593168115 ) ) ;
#1216=CARTESIAN_POINT ( 'NONE',  ( -32.66413529028186957, 379.8073905765656377, -19.99999999999999289 ) ) ;
#1217=CARTESIAN_POINT ( 'NONE',  ( -13.20868407381886023, 360.9948905683720568, -6.410867750099233042 ) ) ;
#1219=CARTESIAN_POINT ( 'NONE',  ( -42.82802356641968089, 513.2448905765656946, 14.14213562373094923 ) ) ;
#1220=CARTESIAN_POINT ( 'NONE',  ( -45.43829269268871229, 393.5573905683720568, -3.332260488124726194 ) ) ;
#1221=CARTESIAN_POINT ( 'NONE',  ( -40.53162694259542320, 226.6198905683720000, 11.84573899990672885 ) ) ;
#1222=CARTESIAN_POINT ( 'NONE',  ( -38.17536295476246266, 402.3073905683720000, -14.20200298773971426 ) ) ;
#1223=CARTESIAN_POINT ( 'NONE',  ( -45.64106924314018698, 332.9323905765655809, 11.32908994701042715 ) ) ;
#1224=CARTESIAN_POINT ( 'NONE',  ( -48.68588794268870146, 326.9323905601784759, -3.978247347593157901 ) ) ;
#1225=CARTESIAN_POINT ( 'NONE',  ( -40.53162694259543031, 302.6198905683720000, -11.84573899990672707 ) ) ;
#1226=CARTESIAN_POINT ( 'NONE',  ( -25.35362745456399125, 458.1823905683720000, 16.75240474999998952 ) ) ;
#1227=CARTESIAN_POINT ( 'NONE',  ( -45.64106924314020119, 512.9323905765656946, 11.32908994701042538 ) ) ;
#1230=CARTESIAN_POINT ( 'NONE',  ( -40.53162694259543741, 364.1198905683720000, -11.84573899990672707 ) ) ;
#1231=CARTESIAN_POINT ( 'NONE',  ( -35.09675569278796559, 495.7448905683720000, 15.47720386886985366 ) ) ;
#1232=CARTESIAN_POINT ( 'NONE',  ( -47.16347859291446554, 516.6198905601784190, -7.653668647301793193 ) ) ;
#1233=CARTESIAN_POINT ( 'NONE',  ( -42.88789093042842637, 314.8073905683721136, 9.489475012073736337 ) ) ;
#1235=VERTEX_POINT ( 'NONE', #4077 ) ;
#1236=CARTESIAN_POINT ( 'NONE',  ( -42.82802356641968089, 525.9948905601785327, -14.14213562373094746 ) ) ;
#1239=CARTESIAN_POINT ( 'NONE',  ( -14.48388495494900674, 419.4323905683720000, 9.489475012073731008 ) ) ;
#1240=CARTESIAN_POINT ( 'NONE',  ( -10.20829729246299067, 396.3698905765656377, 7.653668647301790529 ) ) ;
#1241=CARTESIAN_POINT ( 'NONE',  ( -25.35362745456400191, 441.0573905683720000, -16.75240474999999307 ) ) ;
#1243=CARTESIAN_POINT ( 'NONE',  ( -32.01814843081345430, 471.6823905683720568, -16.75240474999999307 ) ) ;
#1245=CARTESIAN_POINT ( 'NONE',  ( -11.73070664223724968, 376.0573905765656377, 11.32908994701042005 ) ) ;
#1246=CARTESIAN_POINT ( 'NONE',  ( -48.68588794268870146, 281.9948905765656377, 0.000000000000000000 ) ) ;
#1247=LINE ( 'NONE', #10965, #4397 ) ;
#1248=CARTESIAN_POINT ( 'NONE',  ( -11.73070664223726034, 437.9323905765655809, -11.32908994701042538 ) ) ;
#1249=CARTESIAN_POINT ( 'NONE',  ( -36.33955658999050087, 253.8698905765656093, 18.47759065022572500 ) ) ;
#1250=EDGE_CURVE ( 'NONE', #16993, #19049, #14045, .T. ) ;
#1252=CARTESIAN_POINT ( 'NONE',  ( -44.73859291656508219, 223.9102039777117454, 8.083073056675337043 ) ) ;
#1253=CARTESIAN_POINT ( 'NONE',  ( -19.19641293061498999, 431.9323905683719431, -14.20200298773971603 ) ) ;
#1254=CARTESIAN_POINT ( 'NONE',  ( -8.685887942688712116, 266.9948905765656377, -2.449293598294705724E-15 ) ) ;
#1255=CARTESIAN_POINT ( 'NONE',  ( -25.35362745456397704, 242.5573905683720000, -16.75240474999999307 ) ) ;
#1261=CARTESIAN_POINT ( 'NONE',  ( -19.19641293061499354, 468.8073905683719431, 14.20200298773971426 ) ) ;
#1262=CARTESIAN_POINT ( 'NONE',  ( -17.35679799567828496, 228.5573905765656093, -16.95518130045146421 ) ) ;
#1264=CARTESIAN_POINT ( 'NONE',  ( -43.63240530816144513, 209.9813655751484589, 1.306613905557859834 ) ) ;
#1265=CARTESIAN_POINT ( 'NONE',  ( -45.43829269268873361, 535.3698905683720568, 0.000000000000000000 ) ) ;
#1266=ORIENTED_EDGE ( 'NONE', *, *, #20112, .F. ) ;
#1267=CARTESIAN_POINT ( 'NONE',  ( -13.20868407381887977, 528.2448905683720568, 6.410867750099229490 ) ) ;
#1269=CARTESIAN_POINT ( 'NONE',  ( -28.68588794268872633, 449.4948905765655809, -19.99999999999999289 ) ) ;
#1272=CARTESIAN_POINT ( 'NONE',  ( -8.685887942688617969, 237.3073905765656377, -3.978247347592952732 ) ) ;
#1273=FACE_OUTER_BOUND ( 'NONE', #7868, .T. ) ;
#1276=CARTESIAN_POINT ( 'NONE',  ( -25.35362745456396283, 226.6823905683720284, 16.75240474999998952 ) ) ;
#1277=CARTESIAN_POINT ( 'NONE',  ( -14.48388495494899431, 311.3073905683720568, -9.489475012073736337 ) ) ;
#1280=CARTESIAN_POINT ( 'NONE',  ( -45.43829269268870519, 315.3698905683720568, 0.000000000000000000 ) ) ;
#1282=CARTESIAN_POINT ( 'NONE',  ( -32.01814843081344719, 381.6823905683719431, -16.75240474999999307 ) ) ;
#1283=CARTESIAN_POINT ( 'NONE',  ( -13.20868407381887799, 519.7448905683720568, 6.410867750099229490 ) ) ;
#1285=CARTESIAN_POINT ( 'NONE',  ( -45.64106924314018698, 368.1823905601785327, 11.32908994701042715 ) ) ;
#1289=CARTESIAN_POINT ( 'NONE',  ( -14.48388495494901029, 479.4323905683720568, 9.489475012073732785 ) ) ;
#1290=CARTESIAN_POINT ( 'NONE',  ( -11.93348319268871194, 288.8698905683720568, -2.051577885510841163E-15 ) ) ;
#1291=ORIENTED_EDGE ( 'NONE', *, *, #9300, .F. ) ;
#1292=CARTESIAN_POINT ( 'NONE',  ( -16.84014894278197971, 289.1198905683720568, 11.84573899990672530 ) ) ;
#1293=B_SPLINE_CURVE_WITH_KNOTS ( 'NONE', 3,
 ( #3535, #14801, #1710, #13493, #14908, #5044, #18239, #16636, #15017, #201, #11752, #16419, #10123, #16744, #1931, #6875, #20088, #18453, #3640, #10757 ),
 .UNSPECIFIED., .F., .F.,
 ( 4, 2, 2, 2, 2, 2, 2, 2, 2, 4 ),
 ( 1.977866534538390665E-18, 0.0009844208871748756206, 0.001968841774349749506, 0.002953262661524623609, 0.003937683548699496411, 0.004922104435874370514, 0.005906525323049244616, 0.006398735766636719398, 0.006890946210224195047, 0.007875367097399143743 ),
 .UNSPECIFIED. ) ;
#1294=CARTESIAN_POINT ( 'NONE',  ( -16.84014894278198327, 327.6198905683720000, 11.84573899990672530 ) ) ;
#1297=CARTESIAN_POINT ( 'NONE',  ( -11.73070664223723902, 267.9323905765656946, -11.32908994701042715 ) ) ;
#1298=CARTESIAN_POINT ( 'NONE',  ( -28.68588794268872988, 474.7448905601784759, -19.99999999999999289 ) ) ;
#1299=CARTESIAN_POINT ( 'NONE',  ( -32.01814843081343298, 231.6823905683720284, -16.75240474999999307 ) ) ;
#1302=CARTESIAN_POINT ( 'NONE',  ( -38.17536295476244845, 376.9323905683719431, 14.20200298773971781 ) ) ;
#1305=CYLINDRICAL_SURFACE ( 'NONE', #8884, 19.99999999999999645 ) ;
#1307=( BOUNDED_CURVE ( )  B_SPLINE_CURVE ( 2, ( #6046, #5723, #19249, #17312, #9077, #14076, #20659, #5830, #12439, #8862, #4431, #12556, #4326, #11015, #10909, #11340, #9504 ),
 .UNSPECIFIED., .F., .T. ) 
 B_SPLINE_CURVE_WITH_KNOTS ( ( 3, 2, 2, 2, 2, 2, 2, 2, 3 ),
 ( 0.4375000000000002220, 0.4394531250000002220, 0.4414062500000002220, 0.4433593750000002220, 0.4453125000000002220, 0.4472656250000002220, 0.4492187500000002220, 0.4511718750000002220, 0.4531250000000002220 ),
 .UNSPECIFIED. ) 
 CURVE ( )  GEOMETRIC_REPRESENTATION_ITEM ( )  RATIONAL_B_SPLINE_CURVE ( ( 0.9999999999999977796, 0.9807852804032326510, 1.000000000000000000, 0.9807852804032304306, 1.000000000000000000, 0.9807852804032304306, 1.000000000000000000, 0.9807852804032304306, 1.000000000000000000, 0.9807852804032304306, 1.000000000000000000, 0.9807852804032304306, 1.000000000000000000, 0.9807852804032304306, 1.000000000000000000, 0.9807852804032282101, 1.000000000000002220 ) ) 
 REPRESENTATION_ITEM ( '' )  );
#1309=CARTESIAN_POINT ( 'NONE',  ( -11.93348319268873148, 448.5573905683720000, 3.332260488124728415 ) ) ;
#1312=CARTESIAN_POINT ( 'NONE',  ( -45.64106924314019409, 436.3073905601784759, -11.32908994701042715 ) ) ;
#1315=ORIENTED_EDGE ( 'NONE', *, *, #18124, .T. ) ;
#1318=CARTESIAN_POINT ( 'NONE',  ( -40.01497788969913216, 325.6823905601785327, -16.95518130045146421 ) ) ;
#1319=CARTESIAN_POINT ( 'NONE',  ( -11.73070664223725679, 417.9323905765656377, -11.32908994701042538 ) ) ;
#1320=CARTESIAN_POINT ( 'NONE',  ( -11.93348319268872260, 350.0573905683720000, 3.332260488124728859 ) ) ;
#1321=CARTESIAN_POINT ( 'NONE',  ( -24.70764059509557953, 499.1823905765656377, -19.99999999999999289 ) ) ;
#1322=CARTESIAN_POINT ( 'NONE',  ( -22.27502019258949062, 380.7448905683720000, -15.47720386886985544 ) ) ;
#1324=CARTESIAN_POINT ( 'NONE',  ( -45.43829269268871229, 384.1823905683720568, 3.332260488124734632 ) ) ;
#1325=CARTESIAN_POINT ( 'NONE',  ( -32.66413529028186957, 324.1823905765655809, 19.99999999999999289 ) ) ;
#1326=CARTESIAN_POINT ( 'NONE',  ( -36.33955658999051508, 425.3698905601784759, -18.47759065022572855 ) ) ;
#1327=CARTESIAN_POINT ( 'NONE',  ( -22.27502019258946575, 276.9948905683720000, 15.47720386886985189 ) ) ;
#1328=CARTESIAN_POINT ( 'NONE',  ( -13.20868407381886733, 439.7448905683720000, 6.410867750099229490 ) ) ;
#1329=DIRECTION ( 'NONE',  ( -1.191790137725560488E-16, 1.000000000000000000, -0.000000000000000000 ) ) ;
#1330=CARTESIAN_POINT ( 'NONE',  ( -40.01497788969913216, 368.8073905601785327, 16.95518130045146776 ) ) ;
#1332=CARTESIAN_POINT ( 'NONE',  ( -45.43829269268871229, 345.3698905683720568, 0.000000000000000000 ) ) ;
#1333=CARTESIAN_POINT ( 'NONE',  ( -35.09675569278796559, 511.9948905683720000, -15.47720386886985544 ) ) ;
#1334=CARTESIAN_POINT ( 'NONE',  ( -24.70764059509557953, 504.4323905601785327, -19.99999999999999289 ) ) ;
#1335=CARTESIAN_POINT ( 'NONE',  ( -13.20868407381885667, 329.4948905683720568, -6.410867750099233042 ) ) ;
#1337=CARTESIAN_POINT ( 'NONE',  ( -45.64106924314016567, 258.1823905601784190, 11.32908994701042538 ) ) ;
#1341=CARTESIAN_POINT ( 'NONE',  ( -35.09675569278795848, 427.2448905683720568, 15.47720386886985366 ) ) ;
#1342=CARTESIAN_POINT ( 'NONE',  ( -36.33955658999050087, 233.8698905765656093, 18.47759065022572500 ) ) ;
#1343=( LENGTH_UNIT ( ) NAMED_UNIT ( * ) SI_UNIT ( .MILLI., .METRE. ) );
#1344=CARTESIAN_POINT ( 'NONE',  ( -44.16309181155857289, 434.4948905683720568, 6.410867750099241924 ) ) ;
#1346=CARTESIAN_POINT ( 'NONE',  ( -40.53162694259545162, 452.6198905683720568, -11.84573899990672707 ) ) ;
#1349=CARTESIAN_POINT ( 'NONE',  ( -11.73070664223725146, 377.9323905765656946, -11.32908994701042715 ) ) ;
#1350=CARTESIAN_POINT ( 'NONE',  ( -28.68588794268874054, 573.2448905601785327, 0.000000000000000000 ) ) ;
#1352=CARTESIAN_POINT ( 'NONE',  ( -28.68588794268872277, 429.4948905765655809, -19.99999999999999289 ) ) ;
#1354=CARTESIAN_POINT ( 'NONE',  ( -38.17536295476246977, 516.9323905683720568, 14.20200298773971781 ) ) ;
#1357=CARTESIAN_POINT ( 'NONE',  ( -10.20829729246297291, 252.8698905601785043, -7.653668647301794969 ) ) ;
#1359=CARTESIAN_POINT ( 'NONE',  ( -19.19641293061498999, 421.9323905683720000, -14.20200298773971603 ) ) ;
#1360=CARTESIAN_POINT ( 'NONE',  ( -14.54375231895775578, 265.7448905765656377, 14.14213562373094568 ) ) ;
#1361=CARTESIAN_POINT ( 'NONE',  ( -28.68588794268869790, 247.8698905683720000, 16.75240474999999307 ) ) ;
#1367=CARTESIAN_POINT ( 'NONE',  ( -44.16309181155858710, 464.7448905683720568, -6.410867750099231266 ) ) ;
#1368=CARTESIAN_POINT ( 'NONE',  ( -18.67112375231569743, 218.6607918971888864, -17.31197557216455252 ) ) ;
#1369=ADVANCED_FACE ( 'NONE', ( #4931 ), #11208, .T. ) ;
#1371=CARTESIAN_POINT ( 'NONE',  ( -43.31915179403467420, 208.9097650327693430, 3.305147470758841077 ) ) ;
#1372=CARTESIAN_POINT ( 'NONE',  ( -25.35362745456401257, 532.5573905683720568, -16.75240474999999307 ) ) ;
#1374=CARTESIAN_POINT ( 'NONE',  ( -45.43829269268873361, 523.8698905683720568, 0.000000000000000000 ) ) ;
#1376=CARTESIAN_POINT ( 'NONE',  ( -40.01497788969915348, 450.4323905765656946, -16.95518130045146421 ) ) ;
#1377=CARTESIAN_POINT ( 'NONE',  ( -24.70764059509554755, 350.0573905601785327, 19.99999999999998934 ) ) ;
#1378=CARTESIAN_POINT ( 'NONE',  ( -11.93348319268871904, 348.8698905683720568, -2.051577885510841163E-15 ) ) ;
#1380=DIRECTION ( 'NONE',  ( -1.191790137725560488E-16, 1.000000000000000000, -0.000000000000000000 ) ) ;
#1383=CARTESIAN_POINT ( 'NONE',  ( -24.73359481245773495, 223.9102039777117454, 19.67196200432813313 ) ) ;
#1384=CARTESIAN_POINT ( 'NONE',  ( -25.35362745456397704, 231.0573905683720568, -16.75240474999999307 ) ) ;
#1385=CARTESIAN_POINT ( 'NONE',  ( -28.68588794268870501, 307.8698905683720000, 16.75240474999999307 ) ) ;
#1386=CARTESIAN_POINT ( 'NONE',  ( -28.68588794268872633, 444.7448905601784759, -19.99999999999999289 ) ) ;
#1388=CARTESIAN_POINT ( 'NONE',  ( -42.88789093042842637, 316.3073905683720568, 9.489475012073736337 ) ) ;
#1389=CARTESIAN_POINT ( 'NONE',  ( -45.43829269268870519, 354.1823905683721136, 3.332260488124734632 ) ) ;
#1390=CARTESIAN_POINT ( 'NONE',  ( -19.19641293061500420, 531.9323905683720568, -14.20200298773971603 ) ) ;
#1391=CARTESIAN_POINT ( 'NONE',  ( -48.68588794268870856, 367.2448905601784759, 0.000000000000000000 ) ) ;
#1395=CARTESIAN_POINT ( 'NONE',  ( -44.16309181155857999, 495.9948905683720568, 6.410867750099241924 ) ) ;
#1397=CARTESIAN_POINT ( 'NONE',  ( -35.09675569278794427, 275.7448905683720568, 15.47720386886985366 ) ) ;
#1400=CARTESIAN_POINT ( 'NONE',  ( -22.27502019258947996, 292.2448905683720000, -15.47720386886985544 ) ) ;
#1401=CARTESIAN_POINT ( 'NONE',  ( -22.27502019258947286, 326.9948905683720000, 15.47720386886985189 ) ) ;
#1402=CARTESIAN_POINT ( 'NONE',  ( -42.88789093042841927, 264.4323905683720568, -9.489475012073734561 ) ) ;
#1403=CARTESIAN_POINT ( 'NONE',  ( -48.68588794268870146, 272.3073905765656377, 3.978247347593168115 ) ) ;
#1405=CARTESIAN_POINT ( 'NONE',  ( -45.43829269268869808, 234.1823905683720284, 3.332260488124734632 ) ) ;
#1406=CARTESIAN_POINT ( 'NONE',  ( -11.93348319268872260, 380.6823905683720568, -3.332260488124732856 ) ) ;
#1408=CIRCLE ( 'NONE', #8309, 15.00000000000000000 ) ;
#1409=CARTESIAN_POINT ( 'NONE',  ( -17.35679799567830628, 458.5573905765656946, -16.95518130045146421 ) ) ;
#1412=CARTESIAN_POINT ( 'NONE',  ( -45.43829269268871229, 414.1823905683720000, 3.332260488124734632 ) ) ;
#1415=AXIS2_PLACEMENT_3D ( 'NONE', #17806, #14791, #21161 ) ;
#1416=CARTESIAN_POINT ( 'NONE',  ( -48.68588794268871567, 417.5573905601784759, 3.978247347593168115 ) ) ;
#1420=CARTESIAN_POINT ( 'NONE',  ( -8.685887942688715668, 311.9323905601784759, 3.978247347593161010 ) ) ;
#1423=CARTESIAN_POINT ( 'NONE',  ( -19.19641293061497578, 338.8073905683720000, 14.20200298773971426 ) ) ;
#1426=CARTESIAN_POINT ( 'NONE',  ( -48.68588794268872988, 511.9948905765656377, 0.000000000000000000 ) ) ;
#1427=CARTESIAN_POINT ( 'NONE',  ( -38.17536295476244845, 375.4323905683720568, 14.20200298773971781 ) ) ;
#1428=CARTESIAN_POINT ( 'NONE',  ( -11.93348319268870483, 230.3698905683720284, -2.051577885510841163E-15 ) ) ;
#1429=CARTESIAN_POINT ( 'NONE',  ( -38.17536295476245556, 382.3073905683719431, -14.20200298773971426 ) ) ;
#1430=CARTESIAN_POINT ( 'NONE',  ( -8.685887942688717445, 327.3073905765656377, -3.978247347593165895 ) ) ;
#1432=CARTESIAN_POINT ( 'NONE',  ( -32.01814843081344009, 281.6823905683720000, -16.75240474999999307 ) ) ;
#1433=AXIS2_PLACEMENT_3D ( 'NONE', #11035, #7577, #6678 ) ;
#1434=( BOUNDED_CURVE ( )  B_SPLINE_CURVE ( 2, ( #15145, #20106, #16867, #15037, #20211, #327, #221, #13407, #109, #2049, #11771, #18576, #3344, #5376, #8623, #7000, #19996 ),
 .UNSPECIFIED., .F., .T. ) 
 B_SPLINE_CURVE_WITH_KNOTS ( ( 3, 2, 2, 2, 2, 2, 2, 2, 3 ),
 ( 0.7031250000000002220, 0.7050781250000002220, 0.7070312500000002220, 0.7089843750000002220, 0.7109375000000002220, 0.7128906250000002220, 0.7148437500000002220, 0.7167968750000002220, 0.7187500000000002220 ),
 .UNSPECIFIED. ) 
 CURVE ( )  GEOMETRIC_REPRESENTATION_ITEM ( )  RATIONAL_B_SPLINE_CURVE ( ( 0.9999999999999977796, 0.9807852804032326510, 1.000000000000000000, 0.9807852804032304306, 1.000000000000000000, 0.9807852804032304306, 1.000000000000000000, 0.9807852804032304306, 1.000000000000000000, 0.9807852804032304306, 1.000000000000000000, 0.9807852804032304306, 1.000000000000000000, 0.9807852804032304306, 1.000000000000000000, 0.9807852804032282101, 1.000000000000002220 ) ) 
 REPRESENTATION_ITEM ( '' )  );
#1435=CARTESIAN_POINT ( 'NONE',  ( -14.48388495494900496, 439.4323905683720000, 9.489475012073732785 ) ) ;
#1440=CARTESIAN_POINT ( 'NONE',  ( -38.17536295476245556, 353.8073905683720568, -14.20200298773971426 ) ) ;
#1441=CARTESIAN_POINT ( 'NONE',  ( -44.16309181155858710, 503.2448905683719431, -6.410867750099231266 ) ) ;
#1443=CARTESIAN_POINT ( 'NONE',  ( -45.64106924314020119, 478.1823905601784759, 11.32908994701042715 ) ) ;
#1444=CARTESIAN_POINT ( 'NONE',  ( -11.93348319268871727, 318.5573905683720000, 3.332260488124728415 ) ) ;
#1449=CARTESIAN_POINT ( 'NONE',  ( -11.93348319268872615, 410.3698905683720568, -2.051577885510841163E-15 ) ) ;
#1450=CARTESIAN_POINT ( 'NONE',  ( -48.68588794268871567, 397.2448905601784759, 0.000000000000000000 ) ) ;
#1452=CARTESIAN_POINT ( 'NONE',  ( -40.53162694259545162, 452.6198905683720568, -11.84573899990672707 ) ) ;
#1453=CARTESIAN_POINT ( 'NONE',  ( -28.68588794268872277, 446.3698905683720000, 16.75240474999999307 ) ) ;
#1455=CARTESIAN_POINT ( 'NONE',  ( -8.685887942688726326, 402.2448905601784759, -2.449293598294705724E-15 ) ) ;
#1456=CARTESIAN_POINT ( 'NONE',  ( -36.33955658999051508, 390.1198905765656377, -18.47759065022572855 ) ) ;
#1459=CARTESIAN_POINT ( 'NONE',  ( -8.685887942688642838, 427.3073905765655809, -3.978247347592952732 ) ) ;
#1460=CYLINDRICAL_SURFACE ( 'NONE', #1079, 19.99999999999999645 ) ;
#1461=AXIS2_PLACEMENT_3D ( 'NONE', #2129, #11857, #15336 ) ;
#1462=CARTESIAN_POINT ( 'NONE',  ( -42.88789093042844769, 494.4323905683720000, -9.489475012073736337 ) ) ;
#1465=CARTESIAN_POINT ( 'NONE',  ( -24.70764059509555466, 420.0573905601784190, 19.99999999999998934 ) ) ;
#1466=CARTESIAN_POINT ( 'NONE',  ( -45.43829269268871940, 405.3698905683720000, 0.000000000000000000 ) ) ;
#1467=CARTESIAN_POINT ( 'NONE',  ( -8.685887942688546914, 382.5573905601784190, -3.978247347592740013 ) ) ;
#1468=CARTESIAN_POINT ( 'NONE',  ( -13.20868407381884602, 239.7448905683720000, 6.410867750099229490 ) ) ;
#1469=ORIENTED_EDGE ( 'NONE', *, *, #331, .T. ) ;
#1472=CARTESIAN_POINT ( 'NONE',  ( -35.09675569278796559, 457.2448905683720568, 15.47720386886985366 ) ) ;
#1473=CARTESIAN_POINT ( 'NONE',  ( -8.685887942688706786, 226.6823905765656377, 3.978247347593161010 ) ) ;
#1475=CARTESIAN_POINT ( 'NONE',  ( -43.52342829599625418, 209.6345393943126396, 2.222589281884804979 ) ) ;
#1476=CARTESIAN_POINT ( 'NONE',  ( -32.01814843081343298, 221.6823905683720000, -16.75240474999999307 ) ) ;
#1477=ORIENTED_EDGE ( 'NONE', *, *, #4146, .F. ) ;
#1479=CARTESIAN_POINT ( 'NONE',  ( -13.20868407381887799, 509.4948905683720568, -6.410867750099233042 ) ) ;
#1481=CARTESIAN_POINT ( 'NONE',  ( -36.33955658999051508, 440.1198905765656377, -18.47759065022572855 ) ) ;
#1482=CARTESIAN_POINT ( 'NONE',  ( -48.68588794268843145, 361.6823905765655240, -3.978247347593797389 ) ) ;
#1486=CARTESIAN_POINT ( 'NONE',  ( -48.68588794268870146, 287.2448905601784759, 0.000000000000000000 ) ) ;
#1488=CARTESIAN_POINT ( 'NONE',  ( -32.77073113723689346, 223.9102039777117454, 19.64486615283885840 ) ) ;
#1489=CARTESIAN_POINT ( 'NONE',  ( -45.43829269268869808, 233.8698905683720284, 0.000000000000000000 ) ) ;
#1491=CARTESIAN_POINT ( 'NONE',  ( -19.19641293061498288, 321.9323905683720000, -14.20200298773971603 ) ) ;
#1493=CARTESIAN_POINT ( 'NONE',  ( -8.685887942688710339, 261.9323905601784759, 3.978247347593161010 ) ) ;
#1494=CARTESIAN_POINT ( 'NONE',  ( -24.70764059509555111, 380.0573905601785327, 19.99999999999998934 ) ) ;
#1495=CARTESIAN_POINT ( 'NONE',  ( -11.93348319268871727, 310.6823905683720568, -3.332260488124732856 ) ) ;
#1496=CARTESIAN_POINT ( 'NONE',  ( -35.09675569278796559, 523.4948905683720568, -15.47720386886985544 ) ) ;
#1498=CARTESIAN_POINT ( 'NONE',  ( -21.03221929538692336, 364.1198905601785327, -18.47759065022572855 ) ) ;
#1500=CARTESIAN_POINT ( 'NONE',  ( -8.685887942688706786, 226.9948905765656377, -2.449293598294705724E-15 ) ) ;
#1502=CARTESIAN_POINT ( 'NONE',  ( -25.35362745456399480, 478.1823905683720568, 16.75240474999998952 ) ) ;
#1504=CARTESIAN_POINT ( 'NONE',  ( -38.17536295476244845, 282.3073905683720568, -14.20200298773971426 ) ) ;
#1505=ORIENTED_EDGE ( 'NONE', *, *, #11334, .F. ) ;
#1506=CARTESIAN_POINT ( 'NONE',  ( -35.09675569278793716, 283.4948905683720000, -15.47720386886985544 ) ) ;
#1507=CARTESIAN_POINT ( 'NONE',  ( -45.43829269268869808, 314.1823905683720000, 3.332260488124734632 ) ) ;
#1509=CARTESIAN_POINT ( 'NONE',  ( -48.68588794268869435, 261.6823905765656377, -3.978247347593158345 ) ) ;
#1511=CARTESIAN_POINT ( 'NONE',  ( -19.19641293061496157, 227.3073905683720000, 14.20200298773971426 ) ) ;
#1513=CARTESIAN_POINT ( 'NONE',  ( -45.43829269268871229, 385.3698905683720568, 0.000000000000000000 ) ) ;
#1515=CARTESIAN_POINT ( 'NONE',  ( -8.685887942688887975, 281.9323905601784759, 3.978247347593586447 ) ) ;
#1519=CARTESIAN_POINT ( 'NONE',  ( -35.09675569278795848, 425.7448905683720000, 15.47720386886985366 ) ) ;
#1522=CARTESIAN_POINT ( 'NONE',  ( -17.35679799567829917, 430.6823905601785327, 16.95518130045146421 ) ) ;
#1528=CARTESIAN_POINT ( 'NONE',  ( -32.66413529028186957, 309.4323905601784759, 19.99999999999999289 ) ) ;
#1529=CARTESIAN_POINT ( 'NONE',  ( -42.82802356641964536, 205.1437886375728965, -5.000000000000001776 ) ) ;
#1531=CARTESIAN_POINT ( 'NONE',  ( -40.53162694259543741, 336.6198905683720000, 11.84573899990672885 ) ) ;
#1532=CARTESIAN_POINT ( 'NONE',  ( -21.03221929538692692, 505.1198905765656946, 18.47759065022572500 ) ) ;
#1533=CARTESIAN_POINT ( 'NONE',  ( -13.20868407381886023, 378.2448905683720000, 6.410867750099229490 ) ) ;
#1534=CARTESIAN_POINT ( 'NONE',  ( -48.68588794268870146, 311.9948905765655809, 0.000000000000000000 ) ) ;
#1535=CARTESIAN_POINT ( 'NONE',  ( -11.93348319268872437, 388.8698905683720000, -2.051577885510841163E-15 ) ) ;
#1536=CARTESIAN_POINT ( 'NONE',  ( -11.73070664223724080, 316.0573905765655240, 11.32908994701042005 ) ) ;
#1538=CARTESIAN_POINT ( 'NONE',  ( -38.17536295476244135, 285.4323905683720568, 14.20200298773971781 ) ) ;
#1540=CARTESIAN_POINT ( 'NONE',  ( -28.68588794268872277, 432.8698905683720568, -16.75240474999999307 ) ) ;
#1542=CARTESIAN_POINT ( 'NONE',  ( -11.73070664223726389, 501.3073905601784759, 11.32908994701042005 ) ) ;
#1545=CARTESIAN_POINT ( 'NONE',  ( -32.01814843081344719, 347.5573905683720568, 16.75240474999999307 ) ) ;
#1546=CARTESIAN_POINT ( 'NONE',  ( -22.27502019258950128, 490.7448905683720000, -15.47720386886985544 ) ) ;
#1548=CARTESIAN_POINT ( 'NONE',  ( -32.66413529028189089, 495.0573905601784759, -19.99999999999999289 ) ) ;
#1549=CARTESIAN_POINT ( 'NONE',  ( -22.27502019258946930, 306.9948905683720568, 15.47720386886985189 ) ) ;
#1551=CARTESIAN_POINT ( 'NONE',  ( -36.33955658999050087, 259.1198905601784759, 18.47759065022572500 ) ) ;
#1555=EDGE_CURVE ( 'NONE', #5796, #1687, #14959, .T. ) ;
#1556=CARTESIAN_POINT ( 'NONE',  ( -25.35362745456399836, 412.5573905683720000, -16.75240474999999307 ) ) ;
#1557=CARTESIAN_POINT ( 'NONE',  ( -17.35679799567830273, 480.6823905601784759, 16.95518130045146421 ) ) ;
#1559=CARTESIAN_POINT ( 'NONE',  ( -28.68588794268872277, 446.3698905683720000, 16.75240474999999307 ) ) ;
#1560=CARTESIAN_POINT ( 'NONE',  ( -32.01814843081344719, 441.6823905683721136, -16.75240474999999307 ) ) ;
#1561=( BOUNDED_CURVE ( )  B_SPLINE_CURVE ( 2, ( #10290, #7047, #19935, #5006, #5113, #5427, #9974, #18516, #16593, #3494, #10081, #16702, #1891, #8458, #15083, #11922, #3702 ),
 .UNSPECIFIED., .F., .T. ) 
 B_SPLINE_CURVE_WITH_KNOTS ( ( 3, 2, 2, 2, 2, 2, 2, 2, 3 ),
 ( 0.4531250000000002220, 0.4550781250000002220, 0.4570312500000002220, 0.4589843750000002220, 0.4609375000000002220, 0.4628906250000002220, 0.4648437500000002220, 0.4667968750000002220, 0.4687500000000002220 ),
 .UNSPECIFIED. ) 
 CURVE ( )  GEOMETRIC_REPRESENTATION_ITEM ( )  RATIONAL_B_SPLINE_CURVE ( ( 0.9999999999999977796, 0.9807852804032326510, 1.000000000000000000, 0.9807852804032304306, 1.000000000000000000, 0.9807852804032304306, 1.000000000000000000, 0.9807852804032304306, 1.000000000000000000, 0.9807852804032304306, 1.000000000000000000, 0.9807852804032304306, 1.000000000000000000, 0.9807852804032304306, 1.000000000000000000, 0.9807852804032282101, 1.000000000000002220 ) ) 
 REPRESENTATION_ITEM ( '' )  );
#1563=CARTESIAN_POINT ( 'NONE',  ( -48.68588794268870856, 381.9948905765655809, 0.000000000000000000 ) ) ;
#1565=CARTESIAN_POINT ( 'NONE',  ( -17.35679799567828496, 263.8073905601784759, -16.95518130045146421 ) ) ;
#1568=CARTESIAN_POINT ( 'NONE',  ( -44.16309181155857999, 495.9948905683720568, 6.410867750099241924 ) ) ;
#1575=CARTESIAN_POINT ( 'NONE',  ( -35.09675569278795138, 403.4948905683720000, -15.47720386886985544 ) ) ;
#1577=CARTESIAN_POINT ( 'NONE',  ( -38.17536295476243424, 236.9323905683720000, 14.20200298773971781 ) ) ;
#1578=ORIENTED_EDGE ( 'NONE', *, *, #8549, .F. ) ;
#1579=CARTESIAN_POINT ( 'NONE',  ( -40.01497788969913927, 423.5573905765656377, 16.95518130045146776 ) ) ;
#1581=CARTESIAN_POINT ( 'NONE',  ( -40.53162694259544452, 436.6198905683720000, 11.84573899990672885 ) ) ;
#1582=CARTESIAN_POINT ( 'NONE',  ( -48.68588794268869435, 221.9948905765656377, 0.000000000000000000 ) ) ;
#1586=CARTESIAN_POINT ( 'NONE',  ( -13.20868407381884424, 228.2448905683720568, 6.410867750099229490 ) ) ;
#1587=VERTEX_POINT ( 'NONE', #10747 ) ;
#1588=CARTESIAN_POINT ( 'NONE',  ( -42.88789093042844769, 502.9323905683720000, -9.489475012073734561 ) ) ;
#1590=CARTESIAN_POINT ( 'NONE',  ( -28.68588794268872633, 439.4948905765655809, -19.99999999999999289 ) ) ;
#1591=CARTESIAN_POINT ( 'NONE',  ( -17.35679799567828852, 298.5573905765656377, -16.95518130045146421 ) ) ;
#1592=CARTESIAN_POINT ( 'NONE',  ( -45.64106924314017277, 328.1823905601785327, 11.32908994701042538 ) ) ;
#1596=CARTESIAN_POINT ( 'NONE',  ( -27.94030887803372210, 223.9102039777117739, 20.05120499983352289 ) ) ;
#1597=CARTESIAN_POINT ( 'NONE',  ( -14.54375231895778420, 495.7448905765656377, 14.14213562373094568 ) ) ;
#1598=CARTESIAN_POINT ( 'NONE',  ( -45.43829269268870519, 325.3698905683720000, 0.000000000000000000 ) ) ;
#1599=CARTESIAN_POINT ( 'NONE',  ( -48.68588794268869435, 237.2448905601785043, 0.000000000000000000 ) ) ;
#1600=CARTESIAN_POINT ( 'NONE',  ( -11.73070664223723725, 263.1823905601784759, -11.32908994701042715 ) ) ;
#1602=CARTESIAN_POINT ( 'NONE',  ( -19.19641293061497578, 288.8073905683719431, 14.20200298773971426 ) ) ;
#1603=EDGE_CURVE ( 'NONE', #3040, #19138, #13575, .T. ) ;
#1604=CARTESIAN_POINT ( 'NONE',  ( -28.68588794268873343, 527.8698905683720568, 16.75240474999999307 ) ) ;
#1605=CARTESIAN_POINT ( 'NONE',  ( -14.54375231895776821, 370.9948905601784759, 14.14213562373094568 ) ) ;
#1607=CARTESIAN_POINT ( 'NONE',  ( -45.64106924314017277, 316.3073905601785327, -11.32908994701042538 ) ) ;
#1608=VERTEX_POINT ( 'NONE', #20824 ) ;
#1609=CARTESIAN_POINT ( 'NONE',  ( -13.20868407381887621, 490.9948905683720568, -6.410867750099233042 ) ) ;
#1611=CARTESIAN_POINT ( 'NONE',  ( -14.48388495494899075, 289.8073905683720000, -9.489475012073736337 ) ) ;
#1613=CARTESIAN_POINT ( 'NONE',  ( -40.01497788969911795, 228.8073905601784475, 16.95518130045146776 ) ) ;
#1614=CARTESIAN_POINT ( 'NONE',  ( -45.43829269268870519, 275.3698905683720000, 0.000000000000000000 ) ) ;
#1616=CARTESIAN_POINT ( 'NONE',  ( -45.43829269268869808, 265.3698905683720000, 0.000000000000000000 ) ) ;
#1617=CARTESIAN_POINT ( 'NONE',  ( -11.73070664223723547, 237.9323905765656093, -11.32908994701042715 ) ) ;
#1618=CARTESIAN_POINT ( 'NONE',  ( -45.64106924314019409, 476.3073905601785327, -11.32908994701042538 ) ) ;
#1619=CARTESIAN_POINT ( 'NONE',  ( -16.84014894278196905, 227.6198905683720000, 11.84573899990672530 ) ) ;
#1620=CARTESIAN_POINT ( 'NONE',  ( -16.84014894278197616, 267.6198905683720568, 11.84573899990672530 ) ) ;
#1621=CARTESIAN_POINT ( 'NONE',  ( -35.09675569278794427, 383.4948905683720000, -15.47720386886985544 ) ) ;
#1626=CARTESIAN_POINT ( 'NONE',  ( -8.685887942688712116, 266.9948905765656377, -2.449293598294705724E-15 ) ) ;
#1628=CARTESIAN_POINT ( 'NONE',  ( -42.88789093042844058, 414.8073905683720568, 9.489475012073736337 ) ) ;
#1630=CARTESIAN_POINT ( 'NONE',  ( -28.68588794268874054, 573.2448905601785327, 0.000000000000000000 ) ) ;
#1631=ORIENTED_EDGE ( 'NONE', *, *, #15630, .T. ) ;
#1632=CARTESIAN_POINT ( 'NONE',  ( -32.66413529028188378, 419.4323905601784190, 19.99999999999999289 ) ) ;
#1633=ORIENTED_EDGE ( 'NONE', *, *, #5512, .T. ) ;
#1637=CARTESIAN_POINT ( 'NONE',  ( -28.68588794268870501, 299.7448905601784759, 19.99999999999999289 ) ) ;
#1640=CARTESIAN_POINT ( 'NONE',  ( -32.01814843081344719, 347.5573905683720568, 16.75240474999999307 ) ) ;
#1642=CARTESIAN_POINT ( 'NONE',  ( -24.70764059509557953, 489.1823905765656377, -19.99999999999999289 ) ) ;
#1643=CARTESIAN_POINT ( 'NONE',  ( -22.27502019258948707, 370.7448905683720568, -15.47720386886985544 ) ) ;
#1644=CARTESIAN_POINT ( 'NONE',  ( -32.01814843081343298, 223.1823905683720000, -16.75240474999999307 ) ) ;
#1645=CARTESIAN_POINT ( 'NONE',  ( -32.01814843081344719, 396.0573905683720568, 16.75240474999999307 ) ) ;
#1647=CARTESIAN_POINT ( 'NONE',  ( -48.68588794268870146, 301.9948905765655809, 0.000000000000000000 ) ) ;
#1649=CARTESIAN_POINT ( 'NONE',  ( -16.84014894278197616, 277.6198905683720568, 11.84573899990672530 ) ) ;
#1651=CARTESIAN_POINT ( 'NONE',  ( -44.16309181155857289, 435.9948905683720568, 6.410867750099241924 ) ) ;
#1654=EDGE_CURVE ( 'NONE', #5794, #9671, #20601, .T. ) ;
#1655=CARTESIAN_POINT ( 'NONE',  ( -32.66413529028188378, 499.4323905601784759, 19.99999999999999289 ) ) ;
#1658=CARTESIAN_POINT ( 'NONE',  ( -10.20829729246299600, 451.6198905601784759, 7.653668647301790529 ) ) ;
#1659=CARTESIAN_POINT ( 'NONE',  ( -40.53162694259543741, 344.1198905683720568, -11.84573899990672707 ) ) ;
#1660=CARTESIAN_POINT ( 'NONE',  ( -38.17536295476246977, 482.3073905683720568, -14.20200298773971426 ) ) ;
#1662=CARTESIAN_POINT ( 'NONE',  ( -36.33955658999052929, 489.1198905601785327, 18.47759065022572500 ) ) ;
#1663=CARTESIAN_POINT ( 'NONE',  ( -16.84014894278197971, 307.6198905683720000, 11.84573899990672530 ) ) ;
#1664=ORIENTED_EDGE ( 'NONE', *, *, #10335, .F. ) ;
#1665=CARTESIAN_POINT ( 'NONE',  ( -42.82802356641965957, 343.2448905765656377, 14.14213562373094923 ) ) ;
#1667=ORIENTED_EDGE ( 'NONE', *, *, #5396, .T. ) ;
#1669=CARTESIAN_POINT ( 'NONE',  ( -38.17536295476245556, 406.9323905683719431, 14.20200298773971781 ) ) ;
#1671=CARTESIAN_POINT ( 'NONE',  ( -42.88789093042844058, 424.8073905683720000, 9.489475012073736337 ) ) ;
#1672=CARTESIAN_POINT ( 'NONE',  ( -22.27502019258949773, 440.7448905683720000, -15.47720386886985544 ) ) ;
#1673=CARTESIAN_POINT ( 'NONE',  ( -32.66413529028187668, 399.4323905601784759, 19.99999999999999289 ) ) ;
#1674=CARTESIAN_POINT ( 'NONE',  ( -17.35679799567829562, 375.4323905765656377, 16.95518130045146421 ) ) ;
#1678=CARTESIAN_POINT ( 'NONE',  ( -48.68588794268872277, 491.9948905765656377, 0.000000000000000000 ) ) ;
#1679=CARTESIAN_POINT ( 'NONE',  ( -28.68588794268873343, 492.8698905683720568, -16.75240474999999307 ) ) ;
#1681=DIRECTION ( 'NONE',  ( -1.191790137725560488E-16, 1.000000000000000000, -0.000000000000000000 ) ) ;
#1683=CARTESIAN_POINT ( 'NONE',  ( -40.53162694259544452, 406.6198905683720568, 11.84573899990672885 ) ) ;
#1684=CARTESIAN_POINT ( 'NONE',  ( -11.73070664223726389, 467.9323905765655240, -11.32908994701042538 ) ) ;
#1685=CARTESIAN_POINT ( 'NONE',  ( -40.53162694259542320, 234.1198905683720000, -11.84573899990672707 ) ) ;
#1687=VERTEX_POINT ( 'NONE', #18757 ) ;
#1688=CARTESIAN_POINT ( 'NONE',  ( -21.03221929538691626, 425.1198905765656377, 18.47759065022572500 ) ) ;
#1690=CARTESIAN_POINT ( 'NONE',  ( -42.88789093042844058, 434.4323905683720568, -9.489475012073734561 ) ) ;
#1692=CARTESIAN_POINT ( 'NONE',  ( -22.27502019258950483, 520.7448905683720568, -15.47720386886985544 ) ) ;
#1695=CARTESIAN_POINT ( 'NONE',  ( -42.82802356641965247, 205.4732429224858095, 5.000000000000000888 ) ) ;
#1696=CARTESIAN_POINT ( 'NONE',  ( -35.09675569278796559, 533.4948905683720568, -15.47720386886985544 ) ) ;
#1697=EDGE_CURVE ( 'NONE', #18805, #19193, #17964, .T. ) ;
#1699=CARTESIAN_POINT ( 'NONE',  ( -22.27502019258950128, 500.7448905683720000, -15.47720386886985544 ) ) ;
#1702=CARTESIAN_POINT ( 'NONE',  ( -10.20829729246299600, 446.3698905765656377, 7.653668647301790529 ) ) ;
#1704=CARTESIAN_POINT ( 'NONE',  ( -24.70764059509554755, 330.0573905601785896, 19.99999999999998934 ) ) ;
#1710=CARTESIAN_POINT ( 'NONE',  ( -43.67481775055303928, 200.1767262095909246, -0.6600471188826696478 ) ) ;
#1711=CARTESIAN_POINT ( 'NONE',  ( -19.19641293061497578, 298.8073905683719431, 14.20200298773971426 ) ) ;
#1712=EDGE_CURVE ( 'NONE', #1687, #15268, #14346, .T. ) ;
#1714=CARTESIAN_POINT ( 'NONE',  ( -32.66413529028186247, 259.4323905601784759, 19.99999999999999289 ) ) ;
#1715=CARTESIAN_POINT ( 'NONE',  ( -17.35679799567829562, 415.4323905765656946, 16.95518130045146421 ) ) ;
#1716=CARTESIAN_POINT ( 'NONE',  ( -22.27502019258946930, 298.4948905683720568, 15.47720386886985189 ) ) ;
#1717=CARTESIAN_POINT ( 'NONE',  ( -11.93348319268873858, 500.6823905683720568, -3.332260488124732856 ) ) ;
#1718=CARTESIAN_POINT ( 'NONE',  ( -36.33955658999050797, 365.3698905601784759, -18.47759065022572855 ) ) ;
#1721=CARTESIAN_POINT ( 'NONE',  ( -32.01814843081346140, 463.1823905683720000, -16.75240474999999307 ) ) ;
#1723=CARTESIAN_POINT ( 'NONE',  ( -19.19641293061497223, 277.3073905683720000, 14.20200298773971426 ) ) ;
#1725=CARTESIAN_POINT ( 'NONE',  ( -48.68588794268869435, 227.2448905601785043, 0.000000000000000000 ) ) ;
#1726=CARTESIAN_POINT ( 'NONE',  ( -11.93348319268871194, 280.6823905683720000, -3.332260488124732856 ) ) ;
#1727=CARTESIAN_POINT ( 'NONE',  ( -44.16309181155855157, 255.9948905683720568, 6.410867750099241924 ) ) ;
#1728=CARTESIAN_POINT ( 'NONE',  ( -32.66413529028186247, 249.8073905765656662, -19.99999999999999289 ) ) ;
#1729=CARTESIAN_POINT ( 'NONE',  ( -14.54375231895777709, 418.2448905765655809, -14.14213562373094746 ) ) ;
#1730=CARTESIAN_POINT ( 'NONE',  ( -24.70764059509552979, 230.0573905601784759, 19.99999999999998934 ) ) ;
#1732=CARTESIAN_POINT ( 'NONE',  ( -32.01814843081343298, 261.6823905683720568, -16.75240474999999307 ) ) ;
#1733=CARTESIAN_POINT ( 'NONE',  ( -11.93348319268872260, 370.0573905683719431, 3.332260488124728415 ) ) ;
#1738=CARTESIAN_POINT ( 'NONE',  ( -28.68588794268872277, 421.3698905683720568, -16.75240474999999307 ) ) ;
#1740=ORIENTED_EDGE ( 'NONE', *, *, #8071, .T. ) ;
#1741=CARTESIAN_POINT ( 'NONE',  ( -48.68588794268871567, 427.2448905601784759, 0.000000000000000000 ) ) ;
#1744=ORIENTED_EDGE ( 'NONE', *, *, #18262, .T. ) ;
#1746=CARTESIAN_POINT ( 'NONE',  ( -21.03221929538690915, 355.1198905765656377, 18.47759065022572500 ) ) ;
#1747=CARTESIAN_POINT ( 'NONE',  ( -14.54375231895775933, 310.9948905601784759, 14.14213562373094568 ) ) ;
#1750=CARTESIAN_POINT ( 'NONE',  ( -42.88789093042843348, 344.4323905683719431, -9.489475012073734561 ) ) ;
#1753=CARTESIAN_POINT ( 'NONE',  ( -45.64106924314020119, 482.9323905765656377, 11.32908994701042715 ) ) ;
#1754=CARTESIAN_POINT ( 'NONE',  ( -11.93348319268872260, 368.5573905683720568, 3.332260488124728415 ) ) ;
#1755=CARTESIAN_POINT ( 'NONE',  ( -44.16309181155857999, 393.2448905683720568, -6.410867750099231266 ) ) ;
#1756=VECTOR ( 'NONE', #4073, 1000.000000000000000 ) ;
#1757=CARTESIAN_POINT ( 'NONE',  ( -48.68588794268870146, 302.3073905765655809, 3.978247347593168115 ) ) ;
#1759=EDGE_CURVE ( 'NONE', #5272, #15608, #7604, .T. ) ;
#1760=CARTESIAN_POINT ( 'NONE',  ( -38.17536295476244135, 295.4323905683720000, 14.20200298773971781 ) ) ;
#1761=CARTESIAN_POINT ( 'NONE',  ( -10.20829729246299422, 441.6198905601784759, 7.653668647301790529 ) ) ;
#1763=CARTESIAN_POINT ( 'NONE',  ( -25.35362745456398770, 428.1823905683720000, 16.75240474999998952 ) ) ;
#1765=CARTESIAN_POINT ( 'NONE',  ( -47.16347859291445843, 497.8698905601784759, 7.653668647301805628 ) ) ;
#1766=FACE_OUTER_BOUND ( 'NONE', #2668, .T. ) ;
#1769=CARTESIAN_POINT ( 'NONE',  ( -13.20868407381885667, 349.7448905683720568, 6.410867750099229490 ) ) ;
#1770=CARTESIAN_POINT ( 'NONE',  ( -38.17536295476246266, 485.4323905683720000, 14.20200298773971781 ) ) ;
#1771=EDGE_LOOP ( 'NONE', ( #6459, #8341, #11486, #9330 ) ) ;
#1772=CARTESIAN_POINT ( 'NONE',  ( -8.685887942688735208, 482.2448905601784759, -2.449293598294705724E-15 ) ) ;
#1773=CARTESIAN_POINT ( 'NONE',  ( -19.19641293061497578, 307.3073905683720000, 14.20200298773971426 ) ) ;
#1781=CARTESIAN_POINT ( 'NONE',  ( -40.53162694259544452, 396.6198905683720568, 11.84573899990672885 ) ) ;
#1782=CARTESIAN_POINT ( 'NONE',  ( -8.685887942688726326, 386.9948905765655809, -2.449293598294705724E-15 ) ) ;
#1783=CARTESIAN_POINT ( 'NONE',  ( -42.88789093042844058, 414.8073905683720568, 9.489475012073736337 ) ) ;
#1784=CARTESIAN_POINT ( 'NONE',  ( -16.84014894278197616, 259.1198905683720568, 11.84573899990672530 ) ) ;
#1785=AXIS2_PLACEMENT_3D ( 'NONE', #13720, #18253, #535 ) ;
#1786=CARTESIAN_POINT ( 'NONE',  ( -13.20868407381886733, 438.2448905683720000, 6.410867750099229490 ) ) ;
#1789=CARTESIAN_POINT ( 'NONE',  ( -45.64106924314018698, 371.0573905765656377, -11.32908994701042715 ) ) ;
#1791=CARTESIAN_POINT ( 'NONE',  ( -21.03221929538692692, 388.8698905765656377, -18.47759065022572855 ) ) ;
#1794=CARTESIAN_POINT ( 'NONE',  ( -13.20868407381887799, 500.9948905683721136, -6.410867750099233042 ) ) ;
#1797=CARTESIAN_POINT ( 'NONE',  ( -8.685887942688580665, 462.5573905601784759, -3.978247347592792860 ) ) ;
#1800=CARTESIAN_POINT ( 'NONE',  ( -14.48388495494900496, 409.4323905683720000, 9.489475012073732785 ) ) ;
#1802=CARTESIAN_POINT ( 'NONE',  ( -28.68588794268870146, 232.8698905683720284, -16.75240474999999307 ) ) ;
#1803=CARTESIAN_POINT ( 'NONE',  ( -25.35362745456399125, 371.0573905683720000, -16.75240474999999307 ) ) ;
#1805=CARTESIAN_POINT ( 'NONE',  ( -28.68588794268873698, 521.3698905683720568, -16.75240474999999307 ) ) ;
#1807=CARTESIAN_POINT ( 'NONE',  ( -13.20868407381887089, 440.9948905683720568, -6.410867750099233042 ) ) ;
#1808=CARTESIAN_POINT ( 'NONE',  ( -44.16309181155858710, 524.4948905683719431, 6.410867750099241924 ) ) ;
#1811=CARTESIAN_POINT ( 'NONE',  ( -24.70764059509555466, 430.0573905601785327, 19.99999999999998934 ) ) ;
#1812=CARTESIAN_POINT ( 'NONE',  ( -32.01814843081346140, 491.6823905683720000, -16.75240474999999307 ) ) ;
#1815=CARTESIAN_POINT ( 'NONE',  ( -19.19641293061499709, 497.3073905683721136, 14.20200298773971426 ) ) ;
#1817=CARTESIAN_POINT ( 'NONE',  ( -17.35679799567829917, 425.4323905765656377, 16.95518130045146421 ) ) ;
#1818=CARTESIAN_POINT ( 'NONE',  ( -32.66413529028186247, 299.8073905765656377, -19.99999999999999289 ) ) ;
#1819=CARTESIAN_POINT ( 'NONE',  ( -32.66413529028186247, 329.4323905601784759, 19.99999999999999289 ) ) ;
#1822=CARTESIAN_POINT ( 'NONE',  ( -36.33955658999052929, 493.8698905765655809, 18.47759065022572500 ) ) ;
#1823=CARTESIAN_POINT ( 'NONE',  ( -11.93348319268871371, 290.6823905683721136, -3.332260488124732856 ) ) ;
#1824=CARTESIAN_POINT ( 'NONE',  ( -28.68588794268870146, 234.7448905601785043, -19.99999999999999289 ) ) ;
#1825=CARTESIAN_POINT ( 'NONE',  ( -24.70764059509555111, 264.4323905601784759, -19.99999999999999289 ) ) ;
#1828=CARTESIAN_POINT ( 'NONE',  ( -45.43829269268869808, 285.0573905683720000, -3.332260488124726194 ) ) ;
#1829=CARTESIAN_POINT ( 'NONE',  ( -8.685887942688442109, 532.5573905601785327, -3.978247347592446914 ) ) ;
#1830=CARTESIAN_POINT ( 'NONE',  ( -11.93348319268873858, 510.6823905683719431, -3.332260488124732856 ) ) ;
#1833=CARTESIAN_POINT ( 'NONE',  ( -25.35362745456400191, 462.5573905683720000, -16.75240474999999307 ) ) ;
#1835=CARTESIAN_POINT ( 'NONE',  ( -25.35362745456396993, 266.6823905683720568, 16.75240474999998952 ) ) ;
#1841=CARTESIAN_POINT ( 'NONE',  ( -11.93348319268871016, 270.0573905683719431, 3.332260488124728859 ) ) ;
#1842=CARTESIAN_POINT ( 'NONE',  ( -16.84014894278197261, 239.1198905683720284, 11.84573899990672530 ) ) ;
#1843=CARTESIAN_POINT ( 'NONE',  ( -40.01497788969912506, 250.4323905765656093, -16.95518130045146421 ) ) ;
#1845=CARTESIAN_POINT ( 'NONE',  ( -32.66413529028186247, 225.0573905601784759, -19.99999999999999289 ) ) ;
#1847=CARTESIAN_POINT ( 'NONE',  ( -35.09675569278793006, 261.9948905683720000, -15.47720386886985544 ) ) ;
#1848=CARTESIAN_POINT ( 'NONE',  ( -38.17536295476244845, 356.9323905683720000, 14.20200298773971781 ) ) ;
#1849=DIRECTION ( 'NONE',  ( -1.191790137725560488E-16, 1.000000000000000000, -0.000000000000000000 ) ) ;
#1852=CARTESIAN_POINT ( 'NONE',  ( -13.20868407381886733, 419.4948905683720000, -6.410867750099233042 ) ) ;
#1853=CARTESIAN_POINT ( 'NONE',  ( -42.82802356641965957, 340.7448905765655809, -14.14213562373094746 ) ) ;
#1855=CARTESIAN_POINT ( 'NONE',  ( -14.54375231895777176, 410.9948905601785327, 14.14213562373094568 ) ) ;
#1859=CARTESIAN_POINT ( 'NONE',  ( -19.19641293061500065, 528.8073905683719431, 14.20200298773971426 ) ) ;
#1860=CARTESIAN_POINT ( 'NONE',  ( -21.03221929538691626, 314.1198905601784759, -18.47759065022572855 ) ) ;
#1863=CARTESIAN_POINT ( 'NONE',  ( -19.19641293061497933, 321.9323905683720568, -14.20200298773971603 ) ) ;
#1865=CARTESIAN_POINT ( 'NONE',  ( -14.48388495494900141, 369.8073905683720000, -9.489475012073736337 ) ) ;
#1867=CARTESIAN_POINT ( 'NONE',  ( -14.48388495494899963, 359.8073905683720000, -9.489475012073734561 ) ) ;
#1868=CARTESIAN_POINT ( 'NONE',  ( -48.68588794268870146, 311.6823905765656377, -3.978247347593158345 ) ) ;
#1870=CARTESIAN_POINT ( 'NONE',  ( -19.19641293061497223, 270.4323905683720000, -14.20200298773971603 ) ) ;
#1871=CARTESIAN_POINT ( 'NONE',  ( -36.33955658999052218, 439.1198905601784759, 18.47759065022572500 ) ) ;
#1872=CARTESIAN_POINT ( 'NONE',  ( -44.16309181155857289, 425.9948905683720568, 6.410867750099241924 ) ) ;
#1879=CARTESIAN_POINT ( 'NONE',  ( -35.09675569278793716, 323.4948905683720000, -15.47720386886985544 ) ) ;
#1880=CARTESIAN_POINT ( 'NONE',  ( -11.93348319268873503, 478.5573905683721136, 3.332260488124728415 ) ) ;
#1882=CARTESIAN_POINT ( 'NONE',  ( -8.685887942688738761, 491.9323905601785327, 3.978247347593161010 ) ) ;
#1883=CARTESIAN_POINT ( 'NONE',  ( -38.17536295476244845, 302.3073905683720568, -14.20200298773971426 ) ) ;
#1885=CARTESIAN_POINT ( 'NONE',  ( -11.73070664223724613, 341.3073905601785327, 11.32908994701042005 ) ) ;
#1889=CARTESIAN_POINT ( 'NONE',  ( -16.84014894278199392, 409.1198905683720000, 11.84573899990672530 ) ) ;
#1890=CARTESIAN_POINT ( 'NONE',  ( -45.64106924314018698, 442.9323905765656377, 11.32908994701042538 ) ) ;
#1891=CARTESIAN_POINT ( 'NONE',  ( -42.82802356641965957, 383.2448905765656377, 14.14213562373094923 ) ) ;
#1892=CARTESIAN_POINT ( 'NONE',  ( -13.20868407381886911, 429.4948905683720568, -6.410867750099233042 ) ) ;
#1893=CARTESIAN_POINT ( 'NONE',  ( -42.88789093042841927, 264.4323905683720568, -9.489475012073736337 ) ) ;
#1894=CARTESIAN_POINT ( 'NONE',  ( -13.20868407381886733, 428.2448905683720568, 6.410867750099229490 ) ) ;
#1897=CARTESIAN_POINT ( 'NONE',  ( -40.01497788969913927, 360.4323905765656946, -16.95518130045146421 ) ) ;
#1900=CARTESIAN_POINT ( 'NONE',  ( -40.53162694259543741, 332.6198905683720000, -11.84573899990672707 ) ) ;
#1901=CARTESIAN_POINT ( 'NONE',  ( -11.73070664223726567, 487.9323905765656377, -11.32908994701042538 ) ) ;
#1903=CARTESIAN_POINT ( 'NONE',  ( -19.19641293061499354, 488.8073905683720568, 14.20200298773971426 ) ) ;
#1908=CARTESIAN_POINT ( 'NONE',  ( -16.84014894278199037, 399.1198905683720000, 11.84573899990672530 ) ) ;
#1909=CARTESIAN_POINT ( 'NONE',  ( -40.01497788969915348, 470.4323905765656377, -16.95518130045146421 ) ) ;
#1910=CARTESIAN_POINT ( 'NONE',  ( -45.43829269268869098, 235.0573905683720568, -3.332260488124726194 ) ) ;
#1911=CARTESIAN_POINT ( 'NONE',  ( -16.84014894278199037, 360.1198905683720000, -11.84573899990672707 ) ) ;
#1913=CARTESIAN_POINT ( 'NONE',  ( -35.09675569278797269, 515.7448905683720568, 15.47720386886985366 ) ) ;
#1914=ORIENTED_EDGE ( 'NONE', *, *, #2617, .T. ) ;
#1915=CARTESIAN_POINT ( 'NONE',  ( -28.68588794268872277, 437.8698905683720568, 16.75240474999999307 ) ) ;
#1916=CARTESIAN_POINT ( 'NONE',  ( -40.53162694259545873, 515.1198905683720568, 11.84573899990672885 ) ) ;
#1919=CARTESIAN_POINT ( 'NONE',  ( -45.43829269268872650, 483.8698905683720568, 0.000000000000000000 ) ) ;
#1921=CARTESIAN_POINT ( 'NONE',  ( -25.35362745456399836, 506.6823905683720568, 16.75240474999998952 ) ) ;
#1924=CARTESIAN_POINT ( 'NONE',  ( -8.685887942688729879, 426.9948905765656377, -2.449293598294705724E-15 ) ) ;
#1927=CARTESIAN_POINT ( 'NONE',  ( -48.68588794268871567, 441.9948905765656377, 0.000000000000000000 ) ) ;
#1931=CARTESIAN_POINT ( 'NONE',  ( -42.91921849944091605, 203.5275734399367025, -4.734433616062221795 ) ) ;
#1932=CARTESIAN_POINT ( 'NONE',  ( -40.53162694259543031, 306.6198905683720000, 11.84573899990672885 ) ) ;
#1933=EDGE_CURVE ( 'NONE', #18296, #313, #17169, .T. ) ;
#1935=CARTESIAN_POINT ( 'NONE',  ( -40.01497788969912506, 265.6823905601784759, -16.95518130045146421 ) ) ;
#1936=CARTESIAN_POINT ( 'NONE',  ( -8.685887942688818697, 416.6823905765656377, 3.978247347593374172 ) ) ;
#1937=CARTESIAN_POINT ( 'NONE',  ( -38.17536295476244135, 296.9323905683720000, 14.20200298773971781 ) ) ;
#1939=CARTESIAN_POINT ( 'NONE',  ( -11.73070664223723547, 271.3073905601784759, 11.32908994701042005 ) ) ;
#1940=CARTESIAN_POINT ( 'NONE',  ( -40.53162694259545873, 506.6198905683721136, 11.84573899990672885 ) ) ;
#1942=CARTESIAN_POINT ( 'NONE',  ( -11.93348319268873325, 460.0573905683720568, 3.332260488124728415 ) ) ;
#1943=CARTESIAN_POINT ( 'NONE',  ( -14.54375231895777532, 408.2448905765655809, -14.14213562373094746 ) ) ;
#1944=CARTESIAN_POINT ( 'NONE',  ( -19.19641293061497578, 270.4323905683720000, -14.20200298773971603 ) ) ;
#1946=CARTESIAN_POINT ( 'NONE',  ( -40.01497788969913216, 333.5573905765655809, 16.95518130045146776 ) ) ;
#1947=CARTESIAN_POINT ( 'NONE',  ( -25.35362745456398059, 272.5573905683720568, -16.75240474999999307 ) ) ;
#1948=CARTESIAN_POINT ( 'NONE',  ( -40.53162694259542320, 246.6198905683720284, 11.84573899990672885 ) ) ;
#1949=CARTESIAN_POINT ( 'NONE',  ( -47.16347859291443001, 251.3698905765656093, -7.653668647301793193 ) ) ;
#1950=CARTESIAN_POINT ( 'NONE',  ( -48.68588794268871567, 421.9948905765656377, 0.000000000000000000 ) ) ;
#1951=CARTESIAN_POINT ( 'NONE',  ( -48.68588794268869435, 227.2448905601785043, 0.000000000000000000 ) ) ;
#1952=CARTESIAN_POINT ( 'NONE',  ( -14.48388495494898542, 257.9323905683720568, 9.489475012073732785 ) ) ;
#1953=CARTESIAN_POINT ( 'NONE',  ( -16.84014894278198682, 349.1198905683720568, 11.84573899990672530 ) ) ;
#1954=CARTESIAN_POINT ( 'NONE',  ( -24.70764059509557597, 504.4323905601785327, -19.99999999999999289 ) ) ;
#1956=CARTESIAN_POINT ( 'NONE',  ( -35.09675569278795848, 395.7448905683720568, 15.47720386886985366 ) ) ;
#1959=CARTESIAN_POINT ( 'NONE',  ( -48.68588794268871567, 397.5573905601785327, 3.978247347593168115 ) ) ;
#1960=ORIENTED_EDGE ( 'NONE', *, *, #10517, .T. ) ;
#1962=ORIENTED_EDGE ( 'NONE', *, *, #18558, .T. ) ;
#1963=CARTESIAN_POINT ( 'NONE',  ( -40.53162694259545873, 526.6198905683720568, 11.84573899990672885 ) ) ;
#1964=CARTESIAN_POINT ( 'NONE',  ( -40.01497788969913216, 295.6823905601784190, -16.95518130045146421 ) ) ;
#1967=CARTESIAN_POINT ( 'NONE',  ( -22.27502019258947286, 318.4948905683720000, 15.47720386886985189 ) ) ;
#1968=CARTESIAN_POINT ( 'NONE',  ( -28.68588794268871567, 361.3698905683720568, -16.75240474999999307 ) ) ;
#1969=EDGE_CURVE ( 'NONE', #629, #9649, #273, .T. ) ;
#1970=CARTESIAN_POINT ( 'NONE',  ( -45.43829269268871229, 373.5573905683720568, -3.332260488124726638 ) ) ;
#1973=CARTESIAN_POINT ( 'NONE',  ( -17.35679799567828496, 295.4323905765655809, 16.95518130045146421 ) ) ;
#1974=CARTESIAN_POINT ( 'NONE',  ( -31.26501780185373391, 205.1437886375728965, 0.000000000000000000 ) ) ;
#1975=CARTESIAN_POINT ( 'NONE',  ( -13.20868407381884779, 258.2448905683720000, 6.410867750099229490 ) ) ;
#1976=DIRECTION ( 'NONE',  ( -1.191790137725560488E-16, 1.000000000000000000, -0.000000000000000000 ) ) ;
#1977=CARTESIAN_POINT ( 'NONE',  ( -28.68588794268871922, 417.8698905683720568, 16.75240474999999307 ) ) ;
#1980=CARTESIAN_POINT ( 'NONE',  ( -8.685887942688724550, 382.2448905601784759, -2.449293598294705724E-15 ) ) ;
#1983=CARTESIAN_POINT ( 'NONE',  ( -32.01814843081344719, 337.5573905683720000, 16.75240474999999307 ) ) ;
#1984=CARTESIAN_POINT ( 'NONE',  ( -45.43829269268871940, 464.1823905683720568, 3.332260488124734632 ) ) ;
#1986=CARTESIAN_POINT ( 'NONE',  ( -28.68588794268872988, 474.7448905601784759, -19.99999999999999289 ) ) ;
#1987=CARTESIAN_POINT ( 'NONE',  ( -11.93348319268871549, 298.5573905683720000, 3.332260488124728415 ) ) ;
#1989=CARTESIAN_POINT ( 'NONE',  ( -32.66413529028186957, 344.1823905765656377, 19.99999999999999289 ) ) ;
#1992=CARTESIAN_POINT ( 'NONE',  ( -14.54375231895776821, 343.4948905601785327, -14.14213562373094746 ) ) ;
#1995=CARTESIAN_POINT ( 'NONE',  ( -11.93348319268872260, 380.6823905683720568, -3.332260488124732856 ) ) ;
#1997=CARTESIAN_POINT ( 'NONE',  ( -45.43829269268871229, 423.5573905683720000, -3.332260488124726194 ) ) ;
#1998=CARTESIAN_POINT ( 'NONE',  ( -19.19641293061496867, 258.8073905683720000, 14.20200298773971426 ) ) ;
#1999=CARTESIAN_POINT ( 'NONE',  ( -22.27502019258948351, 426.9948905683720568, 15.47720386886985189 ) ) ;
#2002=CARTESIAN_POINT ( 'NONE',  ( -42.82802356641965957, 363.2448905765656377, 14.14213562373094923 ) ) ;
#2004=LINE ( 'NONE', #380, #19948 ) ;
#2005=CARTESIAN_POINT ( 'NONE',  ( -13.20868407381885667, 329.4948905683720568, -6.410867750099233042 ) ) ;
#2007=CARTESIAN_POINT ( 'NONE',  ( -32.01814843081346140, 483.1823905683720000, -16.75240474999999307 ) ) ;
#2008=VECTOR ( 'NONE', #1202, 1000.000000000000000 ) ;
#2009=CARTESIAN_POINT ( 'NONE',  ( -8.685887942688729879, 442.2448905601785327, -2.449293598294705724E-15 ) ) ;
#2010=CARTESIAN_POINT ( 'NONE',  ( -21.03221929538691626, 304.1198905601785327, -18.47759065022572855 ) ) ;
#2012=CARTESIAN_POINT ( 'NONE',  ( -35.09675569278795138, 393.4948905683720000, -15.47720386886985544 ) ) ;
#2013=CARTESIAN_POINT ( 'NONE',  ( -48.68588794268872277, 471.9948905765656377, 0.000000000000000000 ) ) ;
#2014=CARTESIAN_POINT ( 'NONE',  ( -36.33955658999052929, 525.3698905601784190, -18.47759065022572855 ) ) ;
#2015=CARTESIAN_POINT ( 'NONE',  ( -25.35362745456398059, 366.6823905683720000, 16.75240474999998952 ) ) ;
#2017=CARTESIAN_POINT ( 'NONE',  ( -19.19641293061500065, 527.3073905683720568, 14.20200298773971426 ) ) ;
#2019=CARTESIAN_POINT ( 'NONE',  ( -11.93348319268874036, 518.5573905683720568, 3.332260488124728415 ) ) ;
#2021=CARTESIAN_POINT ( 'NONE',  ( -42.82802356641964536, 205.1437886375728965, 5.000000000000001776 ) ) ;
#2022=CARTESIAN_POINT ( 'NONE',  ( -11.93348319268873503, 479.1823905683721136, -3.332260488124732856 ) ) ;
#2023=ORIENTED_EDGE ( 'NONE', *, *, #10335, .T. ) ;
#2024=CARTESIAN_POINT ( 'NONE',  ( -11.93348319268873681, 488.5573905683720568, 3.332260488124728859 ) ) ;
#2025=CARTESIAN_POINT ( 'NONE',  ( -8.685887942688736985, 492.2448905601785327, -2.449293598294705724E-15 ) ) ;
#2027=CARTESIAN_POINT ( 'NONE',  ( -45.64106924314019409, 421.0573905765655809, -11.32908994701042715 ) ) ;
#2029=CARTESIAN_POINT ( 'NONE',  ( -28.68588794268872633, 439.4948905765655809, -19.99999999999999289 ) ) ;
#2032=CARTESIAN_POINT ( 'NONE',  ( -21.03221929538692692, 495.1198905765656377, 18.47759065022572500 ) ) ;
#2033=CARTESIAN_POINT ( 'NONE',  ( -32.01814843081344009, 303.1823905683720000, -16.75240474999999307 ) ) ;
#2035=CARTESIAN_POINT ( 'NONE',  ( -14.48388495494900674, 449.4323905683720568, 9.489475012073732785 ) ) ;
#2038=CARTESIAN_POINT ( 'NONE',  ( -48.68588794268872988, 536.9323905601785327, -3.978247347593157901 ) ) ;
#2039=CARTESIAN_POINT ( 'NONE',  ( -25.35362745456399836, 498.1823905683720568, 16.75240474999998952 ) ) ;
#2040=ORIENTED_EDGE ( 'NONE', *, *, #13784, .T. ) ;
#2041=CARTESIAN_POINT ( 'NONE',  ( -45.43829269268871940, 465.0573905683720000, -3.332260488124726194 ) ) ;
#2043=CARTESIAN_POINT ( 'NONE',  ( -28.68588794268870146, 266.3698905683720000, 16.75240474999999307 ) ) ;
#2045=CARTESIAN_POINT ( 'NONE',  ( -8.685887942688898633, 336.6823905765656377, 3.978247347593586447 ) ) ;
#2047=CARTESIAN_POINT ( 'NONE',  ( -24.70764059509555111, 309.1823905765656377, -19.99999999999999289 ) ) ;
#2048=CARTESIAN_POINT ( 'NONE',  ( -19.19641293061496512, 238.8073905683720284, 14.20200298773971426 ) ) ;
#2049=CARTESIAN_POINT ( 'NONE',  ( -32.66413529028186247, 309.4323905601785327, 19.99999999999999289 ) ) ;
#2050=FACE_OUTER_BOUND ( 'NONE', #14540, .T. ) ;
#2051=CARTESIAN_POINT ( 'NONE',  ( -42.88789093042841927, 262.9323905683720568, -9.489475012073736337 ) ) ;
#2052=CARTESIAN_POINT ( 'NONE',  ( -42.88789093042843348, 366.3073905683720000, 9.489475012073736337 ) ) ;
#2053=CARTESIAN_POINT ( 'NONE',  ( -42.82802356641965247, 278.4948905601785327, 14.14213562373094923 ) ) ;
#2055=EDGE_CURVE ( 'NONE', #10338, #15635, #16707, .T. ) ;
#2056=CARTESIAN_POINT ( 'NONE',  ( -28.68588794268871922, 406.3698905683720000, 16.75240474999999307 ) ) ;
#2057=CARTESIAN_POINT ( 'NONE',  ( -47.16347859291445843, 507.8698905601785327, 7.653668647301805628 ) ) ;
#2058=CARTESIAN_POINT ( 'NONE',  ( -32.66413529028188378, 399.4323905601784759, 19.99999999999999289 ) ) ;
#2059=EDGE_LOOP ( 'NONE', ( #17770, #21021, #12429, #7123 ) ) ;
#2061=ORIENTED_EDGE ( 'NONE', *, *, #13941, .T. ) ;
#2062=CARTESIAN_POINT ( 'NONE',  ( -14.48388495494901740, 521.3073905683720568, -9.489475012073736337 ) ) ;
#2064=CARTESIAN_POINT ( 'NONE',  ( -8.685887942688712116, 282.2448905601784759, -2.449293598294705724E-15 ) ) ;
#2066=CARTESIAN_POINT ( 'NONE',  ( -38.17536295476244135, 316.9323905683719431, 14.20200298773971781 ) ) ;
#2068=CARTESIAN_POINT ( 'NONE',  ( -35.09675569278795138, 365.7448905683720568, 15.47720386886985366 ) ) ;
#2069=CARTESIAN_POINT ( 'NONE',  ( -13.20868407381886200, 369.4948905683720568, -6.410867750099233042 ) ) ;
#2070=CARTESIAN_POINT ( 'NONE',  ( -8.685887942688717445, 306.9948905765655809, -2.449293598294705724E-15 ) ) ;
#2072=CARTESIAN_POINT ( 'NONE',  ( -25.35362745456396638, 256.6823905683720000, 16.75240474999998952 ) ) ;
#2073=CARTESIAN_POINT ( 'NONE',  ( -43.67482055103364047, 200.1767183643994770, 0.6599055232175832231 ) ) ;
#2074=CARTESIAN_POINT ( 'NONE',  ( -40.53162694259544452, 426.6198905683720000, 11.84573899990672885 ) ) ;
#2076=CARTESIAN_POINT ( 'NONE',  ( -48.68588794268861619, 356.9323905601784190, -3.978247347593371508 ) ) ;
#2077=CARTESIAN_POINT ( 'NONE',  ( -42.82802356641965247, 273.2448905765656377, 14.14213562373094923 ) ) ;
#2078=PRODUCT_DEFINITION_CONTEXT ( 'detailed design', #15254, 'design' ) ;
#2079=CARTESIAN_POINT ( 'NONE',  ( -10.20829729246299067, 411.6198905601784759, 7.653668647301790529 ) ) ;
#2080=CARTESIAN_POINT ( 'NONE',  ( -44.16309181155856578, 335.9948905683720000, 6.410867750099241924 ) ) ;
#2081=CARTESIAN_POINT ( 'NONE',  ( -13.20868407381887444, 469.4948905683720000, -6.410867750099233042 ) ) ;
#2082=VERTEX_POINT ( 'NONE', #11927 ) ;
#2083=CARTESIAN_POINT ( 'NONE',  ( -14.54375231895778242, 463.4948905601785327, -14.14213562373094746 ) ) ;
#2084=CARTESIAN_POINT ( 'NONE',  ( -42.88789093042842637, 282.9323905683721136, -9.489475012073736337 ) ) ;
#2085=CARTESIAN_POINT ( 'NONE',  ( -14.54375231895776466, 340.9948905601784759, 14.14213562373094568 ) ) ;
#2087=LINE ( 'NONE', #16698, #11544 ) ;
#2088=CARTESIAN_POINT ( 'NONE',  ( -14.54375231895776466, 340.9948905601784759, 14.14213562373094568 ) ) ;
#2089=CARTESIAN_POINT ( 'NONE',  ( -32.01814843081344719, 393.1823905683721136, -16.75240474999999307 ) ) ;
#2090=CARTESIAN_POINT ( 'NONE',  ( -11.73070664223723014, 231.3073905601784475, 11.32908994701042005 ) ) ;
#2091=CARTESIAN_POINT ( 'NONE',  ( -28.68588794268874054, 573.2448905601785327, 0.000000000000000000 ) ) ;
#2092=CARTESIAN_POINT ( 'NONE',  ( -32.01814843081345430, 421.6823905683720568, -16.75240474999999307 ) ) ;
#2093=CARTESIAN_POINT ( 'NONE',  ( -19.19641293061497578, 261.9323905683720568, -14.20200298773971603 ) ) ;
#2096=CARTESIAN_POINT ( 'NONE',  ( -44.16309181155857999, 433.2448905683720000, -6.410867750099231266 ) ) ;
#2098=EDGE_CURVE ( 'NONE', #2934, #3515, #9978, .T. ) ;
#2099=CARTESIAN_POINT ( 'NONE',  ( -47.16347859291444422, 362.6198905765656377, 7.653668647301805628 ) ) ;
#2100=CARTESIAN_POINT ( 'NONE',  ( -14.54375231895775933, 273.4948905601785327, -14.14213562373094746 ) ) ;
#2101=CARTESIAN_POINT ( 'NONE',  ( -14.48388495494899431, 319.8073905683720568, -9.489475012073734561 ) ) ;
#2103=CARTESIAN_POINT ( 'NONE',  ( -25.35362745456399480, 478.1823905683720568, 16.75240474999998952 ) ) ;
#2107=CARTESIAN_POINT ( 'NONE',  ( -21.03221929538689494, 225.1198905765656093, 18.47759065022572500 ) ) ;
#2109=CARTESIAN_POINT ( 'NONE',  ( -16.84014894278199037, 389.1198905683720568, 11.84573899990672530 ) ) ;
#2112=CARTESIAN_POINT ( 'NONE',  ( -8.685887942688742314, 522.5573905601785327, -3.978247347593165895 ) ) ;
#2113=CARTESIAN_POINT ( 'NONE',  ( -38.17536295476244845, 355.4323905683720568, 14.20200298773971781 ) ) ;
#2115=CARTESIAN_POINT ( 'NONE',  ( -44.16309181155858710, 524.4948905683719431, 6.410867750099241924 ) ) ;
#2117=CARTESIAN_POINT ( 'NONE',  ( -17.35679799567829917, 353.8073905601784759, -16.95518130045146421 ) ) ;
#2118=CARTESIAN_POINT ( 'NONE',  ( -45.43829269268872650, 514.1823905683719431, 3.332260488124734632 ) ) ;
#2120=CARTESIAN_POINT ( 'NONE',  ( -32.01814843081346140, 476.0573905683720000, 16.75240474999999307 ) ) ;
#2122=CARTESIAN_POINT ( 'NONE',  ( -45.43829269268872650, 483.5573905683720000, -3.332260488124726638 ) ) ;
#2123=CARTESIAN_POINT ( 'NONE',  ( -24.70764059509556176, 490.0573905601784190, 19.99999999999998934 ) ) ;
#2124=CARTESIAN_POINT ( 'NONE',  ( -8.685887942688728103, 416.6823905765656377, 3.978247347593161010 ) ) ;
#2125=AXIS2_PLACEMENT_3D ( 'NONE', #18739, #699, #7268 ) ;
#2127=CARTESIAN_POINT ( 'NONE',  ( -8.685887942688980345, 301.9323905601784190, 3.978247347593800054 ) ) ;
#2128=CARTESIAN_POINT ( 'NONE',  ( -48.68588794268873698, 573.2448905601785327, 0.000000000000000000 ) ) ;
#2129=CARTESIAN_POINT ( 'NONE',  ( -28.68588794268873698, 548.2448905601784190, 0.000000000000000000 ) ) ;
#2131=( BOUNDED_CURVE ( )  B_SPLINE_CURVE ( 2, ( #17586, #8930, #12188, #18992, #5904, #9364, #19108, #2458, #15872, #15555, #15979, #14037, #17380, #2561, #9038, #15764, #17479 ),
 .UNSPECIFIED., .F., .T. ) 
 B_SPLINE_CURVE_WITH_KNOTS ( ( 3, 2, 2, 2, 2, 2, 2, 2, 3 ),
 ( 0.1562500000000001388, 0.1582031250000001388, 0.1601562500000001388, 0.1621093750000001388, 0.1640625000000001665, 0.1660156250000001665, 0.1679687500000001665, 0.1699218750000001665, 0.1718750000000001665 ),
 .UNSPECIFIED. ) 
 CURVE ( )  GEOMETRIC_REPRESENTATION_ITEM ( )  RATIONAL_B_SPLINE_CURVE ( ( 0.9999999999999986677, 0.9807852804032317628, 1.000000000000000000, 0.9807852804032304306, 1.000000000000000000, 0.9807852804032304306, 1.000000000000000000, 0.9807852804032304306, 1.000000000000000000, 0.9807852804032304306, 1.000000000000000000, 0.9807852804032304306, 1.000000000000000000, 0.9807852804032304306, 1.000000000000000000, 0.9807852804032287652, 1.000000000000001554 ) ) 
 REPRESENTATION_ITEM ( '' )  );
#2132=CARTESIAN_POINT ( 'NONE',  ( -13.20868407381885312, 300.9948905683720568, -6.410867750099233042 ) ) ;
#2134=CARTESIAN_POINT ( 'NONE',  ( -35.09675569278795848, 447.2448905683720000, 15.47720386886985366 ) ) ;
#2135=LINE ( 'NONE', #2245, #16838 ) ;
#2136=CARTESIAN_POINT ( 'NONE',  ( -45.43829269268869098, 265.6823905683720568, 3.332260488124734632 ) ) ;
#2138=CARTESIAN_POINT ( 'NONE',  ( -47.16347859291443001, 267.8698905601784759, 7.653668647301805628 ) ) ;
#2139=CARTESIAN_POINT ( 'NONE',  ( -35.09675569278797269, 507.2448905683719431, 15.47720386886985366 ) ) ;
#2140=EDGE_CURVE ( 'NONE', #3989, #15664, #6840, .T. ) ;
#2142=CARTESIAN_POINT ( 'NONE',  ( -14.48388495494901029, 461.3073905683720568, -9.489475012073736337 ) ) ;
#2144=DIRECTION ( 'NONE',  ( -1.000000000000000000, 0.000000000000000000, 0.000000000000000000 ) ) ;
#2145=CARTESIAN_POINT ( 'NONE',  ( -44.16309181155855867, 253.2448905683720284, -6.410867750099231266 ) ) ;
#2148=CARTESIAN_POINT ( 'NONE',  ( -35.09675569278793716, 267.2448905683720568, 15.47720386886985366 ) ) ;
#2149=CARTESIAN_POINT ( 'NONE',  ( -10.20829729246299955, 477.6198905765656377, -7.653668647301794969 ) ) ;
#2151=CARTESIAN_POINT ( 'NONE',  ( -11.93348319268870661, 250.6823905683720568, -3.332260488124732856 ) ) ;
#2155=CARTESIAN_POINT ( 'NONE',  ( -19.19641293061497223, 250.4323905683720284, -14.20200298773971603 ) ) ;
#2157=CARTESIAN_POINT ( 'NONE',  ( -42.88789093042843348, 356.3073905683720000, 9.489475012073736337 ) ) ;
#2160=CARTESIAN_POINT ( 'NONE',  ( -42.88789093042844058, 402.9323905683720000, -9.489475012073736337 ) ) ;
#2161=CARTESIAN_POINT ( 'NONE',  ( -48.68588794268870856, 341.9948905765656377, 0.000000000000000000 ) ) ;
#2163=CARTESIAN_POINT ( 'NONE',  ( -8.685887942688726326, 401.9323905601784190, 3.978247347593161010 ) ) ;
#2165=CARTESIAN_POINT ( 'NONE',  ( -17.35679799567829562, 348.5573905765655809, -16.95518130045146421 ) ) ;
#2168=CARTESIAN_POINT ( 'NONE',  ( -35.09675569278797269, 527.2448905683719431, 15.47720386886985366 ) ) ;
#2169=CARTESIAN_POINT ( 'NONE',  ( -32.66413529028186957, 289.4323905601784759, 19.99999999999999289 ) ) ;
#2171=CARTESIAN_POINT ( 'NONE',  ( -42.88789093042842637, 314.4323905683719431, -9.489475012073734561 ) ) ;
#2172=CARTESIAN_POINT ( 'NONE',  ( -13.20868407381885667, 338.2448905683720568, 6.410867750099229490 ) ) ;
#2173=CARTESIAN_POINT ( 'NONE',  ( -13.20868407381886023, 368.2448905683720000, 6.410867750099229490 ) ) ;
#2174=ADVANCED_FACE ( 'NONE', ( #11454 ), #1208, .T. ) ;
#2175=CARTESIAN_POINT ( 'NONE',  ( -48.68588794268870146, 291.6823905765656377, -3.978247347593158345 ) ) ;
#2177=CARTESIAN_POINT ( 'NONE',  ( -44.16309181155855867, 263.2448905683720000, -6.410867750099231266 ) ) ;
#2180=CARTESIAN_POINT ( 'NONE',  ( -11.93348319268872615, 410.3698905683720568, -2.051577885510841163E-15 ) ) ;
#2182=CARTESIAN_POINT ( 'NONE',  ( -21.03221929538693402, 448.8698905765656377, -18.47759065022572855 ) ) ;
#2185=CARTESIAN_POINT ( 'NONE',  ( -11.93348319268871727, 320.6823905683720000, -3.332260488124732856 ) ) ;
#2186=CARTESIAN_POINT ( 'NONE',  ( -45.43829269268872650, 463.8698905683720000, 0.000000000000000000 ) ) ;
#2187=EDGE_LOOP ( 'NONE', ( #11092, #20552, #125, #11975 ) ) ;
#2188=CARTESIAN_POINT ( 'NONE',  ( -36.33955658999052929, 469.1198905601784759, 18.47759065022572500 ) ) ;
#2189=CARTESIAN_POINT ( 'NONE',  ( -19.19641293061497578, 280.4323905683720568, -14.20200298773971603 ) ) ;
#2194=CIRCLE ( 'NONE', #7691, 15.00000000000000355 ) ;
#2195=CARTESIAN_POINT ( 'NONE',  ( -14.48388495494899253, 299.8073905683720000, -9.489475012073736337 ) ) ;
#2196=CARTESIAN_POINT ( 'NONE',  ( -22.27502019258947996, 378.4948905683720000, 15.47720386886985189 ) ) ;
#2197=CARTESIAN_POINT ( 'NONE',  ( -40.01497788969913216, 295.6823905601784190, -16.95518130045146421 ) ) ;
#2198=CARTESIAN_POINT ( 'NONE',  ( -42.82802356641968089, 520.7448905765656946, -14.14213562373094746 ) ) ;
#2199=CARTESIAN_POINT ( 'NONE',  ( -40.53162694259544452, 412.6198905683720568, -11.84573899990672707 ) ) ;
#2200=CARTESIAN_POINT ( 'NONE',  ( -28.68588794268870501, 262.8698905683720000, -16.75240474999999307 ) ) ;
#2201=CARTESIAN_POINT ( 'NONE',  ( -11.93348319268872970, 429.1823905683720568, -3.332260488124732856 ) ) ;
#2202=CARTESIAN_POINT ( 'NONE',  ( -45.64106924314018698, 372.9323905765655809, 11.32908994701042715 ) ) ;
#2204=CARTESIAN_POINT ( 'NONE',  ( -14.48388495494899253, 317.9323905683719431, 9.489475012073731008 ) ) ;
#2205=CARTESIAN_POINT ( 'NONE',  ( -35.09675569278795848, 473.4948905683720000, -15.47720386886985544 ) ) ;
#2212=CARTESIAN_POINT ( 'NONE',  ( -19.19641293061498999, 381.9323905683720568, -14.20200298773971603 ) ) ;
#2215=CARTESIAN_POINT ( 'NONE',  ( -14.54375231895778597, 520.9948905601784190, 14.14213562373094568 ) ) ;
#2216=CARTESIAN_POINT ( 'NONE',  ( -13.20868407381885845, 339.4948905683720568, -6.410867750099233042 ) ) ;
#2219=CARTESIAN_POINT ( 'NONE',  ( -11.93348319268874214, 528.8698905683719431, -2.051577885510841163E-15 ) ) ;
#2220=ORIENTED_EDGE ( 'NONE', *, *, #18687, .F. ) ;
#2221=CARTESIAN_POINT ( 'NONE',  ( -11.73070664223724968, 353.1823905601784759, -11.32908994701042715 ) ) ;
#2223=CARTESIAN_POINT ( 'NONE',  ( -48.68588794268870146, 317.2448905601784759, 0.000000000000000000 ) ) ;
#2224=CARTESIAN_POINT ( 'NONE',  ( -28.68588794268870856, 289.4948905765656377, -19.99999999999999289 ) ) ;
#2225=CARTESIAN_POINT ( 'NONE',  ( -28.68588794268873343, 494.7448905601785327, -19.99999999999999289 ) ) ;
#2226=CARTESIAN_POINT ( 'NONE',  ( -25.35362745456400546, 481.0573905683720568, -16.75240474999999307 ) ) ;
#2228=CARTESIAN_POINT ( 'NONE',  ( -13.20868407381887444, 479.4948905683720000, -6.410867750099233042 ) ) ;
#2229=CARTESIAN_POINT ( 'NONE',  ( -28.68588794268869790, 244.4948905765655809, 19.99999999999999289 ) ) ;
#2232=CARTESIAN_POINT ( 'NONE',  ( -17.35679799567829917, 415.4323905765656377, 16.95518130045146421 ) ) ;
#2233=CARTESIAN_POINT ( 'NONE',  ( -36.33955658999052929, 473.8698905765656377, 18.47759065022572500 ) ) ;
#2239=CARTESIAN_POINT ( 'NONE',  ( -48.68588794268871567, 431.9948905765656377, 0.000000000000000000 ) ) ;
#2241=CARTESIAN_POINT ( 'NONE',  ( -28.68588794268870501, 272.8698905683720000, -16.75240474999999307 ) ) ;
#2242=CARTESIAN_POINT ( 'NONE',  ( -21.03221929538689849, 250.3698905601785043, 18.47759065022572500 ) ) ;
#2243=CARTESIAN_POINT ( 'NONE',  ( -40.01497788969913216, 363.5573905765655809, 16.95518130045146776 ) ) ;
#2244=CARTESIAN_POINT ( 'NONE',  ( -16.84014894278199748, 439.1198905683720568, 11.84573899990672530 ) ) ;
#2245=CARTESIAN_POINT ( 'NONE',  ( -48.68588794268873698, 573.2448905601785327, 0.000000000000000000 ) ) ;
#2246=CARTESIAN_POINT ( 'NONE',  ( -32.01814843081343298, 267.5573905683720000, 16.75240474999999307 ) ) ;
#2249=CARTESIAN_POINT ( 'NONE',  ( -42.82802356641968089, 535.9948905601785327, -14.14213562373094746 ) ) ;
#2250=CARTESIAN_POINT ( 'NONE',  ( -40.53162694259545162, 476.6198905683720000, 11.84573899990672885 ) ) ;
#2252=CARTESIAN_POINT ( 'NONE',  ( -28.68588794268874054, 573.2448905601785327, 0.000000000000000000 ) ) ;
#2253=CARTESIAN_POINT ( 'NONE',  ( -19.19641293061497223, 267.3073905683720568, 14.20200298773971426 ) ) ;
#2256=CARTESIAN_POINT ( 'NONE',  ( -21.03221929538692336, 475.1198905765656377, 18.47759065022572500 ) ) ;
#2257=CARTESIAN_POINT ( 'NONE',  ( -45.64106924314017988, 388.1823905601784759, 11.32908994701042538 ) ) ;
#2258=B_SPLINE_CURVE_WITH_KNOTS ( 'NONE', 3,
 ( #5767, #10523, #7786, #9013, #8906, #709, #605, #12374, #18853, #12778, #18639, #19371, #822, #17642, #13904, #11143 ),
 .UNSPECIFIED., .F., .F.,
 ( 4, 2, 2, 2, 2, 2, 2, 4 ),
 ( 0.000000000000000000, 0.001981573912372597106, 0.003963147824745194212, 0.007926295649490388423, 0.009907869561862979457, 0.01188944347423557223, 0.01387101738660816673, 0.01585259129898075950 ),
 .UNSPECIFIED. ) ;
#2259=CARTESIAN_POINT ( 'NONE',  ( -11.93348319268870661, 240.3698905683720568, -2.051577885510841163E-15 ) ) ;
#2260=( BOUNDED_CURVE ( )  B_SPLINE_CURVE ( 2, ( #11395, #8040, #14672, #18106, #6524, #21251, #282, #18212, #8253, #14882, #14989, #16608, #19731, #4913, #9771, #16397, #11619 ),
 .UNSPECIFIED., .F., .T. ) 
 B_SPLINE_CURVE_WITH_KNOTS ( ( 3, 2, 2, 2, 2, 2, 2, 2, 3 ),
 ( 0.04687500000000040246, 0.04882812500000036082, 0.05078125000000031919, 0.05273437500000027062, 0.05468750000000022898, 0.05664062500000018735, 0.05859375000000013878, 0.06054687500000009714, 0.06250000000000005551 ),
 .UNSPECIFIED. ) 
 CURVE ( )  GEOMETRIC_REPRESENTATION_ITEM ( )  RATIONAL_B_SPLINE_CURVE ( ( 0.9999999999999960032, 0.9807852804032344274, 1.000000000000000000, 0.9807852804032304306, 1.000000000000000000, 0.9807852804032304306, 1.000000000000000000, 0.9807852804032304306, 1.000000000000000000, 0.9807852804032304306, 1.000000000000000000, 0.9807852804032304306, 1.000000000000000000, 0.9807852804032304306, 1.000000000000000000, 0.9807852804032298755, 1.000000000000000444 ) ) 
 REPRESENTATION_ITEM ( '' )  );
#2261=CARTESIAN_POINT ( 'NONE',  ( -28.68588794268871567, 374.4948905765656377, 19.99999999999999289 ) ) ;
#2262=CARTESIAN_POINT ( 'NONE',  ( -42.88789093042841927, 242.9323905683720284, -9.489475012073736337 ) ) ;
#2263=CARTESIAN_POINT ( 'NONE',  ( -40.53162694259543741, 356.6198905683720000, 11.84573899990672885 ) ) ;
#2266=CARTESIAN_POINT ( 'NONE',  ( -45.43829269268871229, 394.1823905683720000, 3.332260488124734632 ) ) ;
#2268=CARTESIAN_POINT ( 'NONE',  ( -40.01497788969914637, 405.6823905601784759, -16.95518130045146421 ) ) ;
#2270=CARTESIAN_POINT ( 'NONE',  ( -28.68588794268874054, 573.2448905601785327, 0.000000000000000000 ) ) ;
#2273=CARTESIAN_POINT ( 'NONE',  ( -44.16309181155857999, 505.9948905683720000, 6.410867750099241924 ) ) ;
#2274=CARTESIAN_POINT ( 'NONE',  ( -8.685887942688713892, 292.2448905601784759, -2.449293598294705724E-15 ) ) ;
#2277=CARTESIAN_POINT ( 'NONE',  ( -42.88789093042842637, 326.3073905683720568, 9.489475012073734561 ) ) ;
#2278=CARTESIAN_POINT ( 'NONE',  ( -44.16309181155857289, 353.2448905683720000, -6.410867750099231266 ) ) ;
#2279=CARTESIAN_POINT ( 'NONE',  ( -44.16309181155856578, 374.4948905683720000, 6.410867750099241924 ) ) ;
#2281=CARTESIAN_POINT ( 'NONE',  ( -47.16347859291443712, 282.6198905765656377, 7.653668647301805628 ) ) ;
#2283=CARTESIAN_POINT ( 'NONE',  ( -32.01814843081343298, 251.6823905683720568, -16.75240474999999307 ) ) ;
#2285=CARTESIAN_POINT ( 'NONE',  ( -40.53162694259544452, 424.1198905683720000, -11.84573899990672707 ) ) ;
#2286=CARTESIAN_POINT ( 'NONE',  ( -48.68588794268870856, 337.2448905601784759, 0.000000000000000000 ) ) ;
#2287=CARTESIAN_POINT ( 'NONE',  ( -14.54375231895778064, 448.2448905765656377, -14.14213562373094746 ) ) ;
#2290=CARTESIAN_POINT ( 'NONE',  ( -45.43829269268870519, 325.3698905683720000, 0.000000000000000000 ) ) ;
#2291=CARTESIAN_POINT ( 'NONE',  ( -25.35362745456399480, 466.6823905683720000, 16.75240474999998952 ) ) ;
#2293=CARTESIAN_POINT ( 'NONE',  ( -48.68588794268872277, 467.2448905601784759, 0.000000000000000000 ) ) ;
#2294=CARTESIAN_POINT ( 'NONE',  ( -14.48388495494898898, 287.9323905683720000, 9.489475012073732785 ) ) ;
#2297=CARTESIAN_POINT ( 'NONE',  ( -42.88789093042844058, 444.4323905683720000, -9.489475012073734561 ) ) ;
#2299=DIRECTION ( 'NONE',  ( -1.191790137725560488E-16, 1.000000000000000000, -0.000000000000000000 ) ) ;
#2300=CARTESIAN_POINT ( 'NONE',  ( -28.68588794268870856, 291.3698905683720568, -16.75240474999999307 ) ) ;
#2301=CARTESIAN_POINT ( 'NONE',  ( -45.43829269268871229, 385.6823905683720000, 3.332260488124734632 ) ) ;
#2303=LINE ( 'NONE', #3805, #2804 ) ;
#2304=CARTESIAN_POINT ( 'NONE',  ( -21.03221929538694468, 518.8698905765655809, -18.47759065022572855 ) ) ;
#2305=CARTESIAN_POINT ( 'NONE',  ( -42.88789093042844058, 402.9323905683720000, -9.489475012073736337 ) ) ;
#2306=CARTESIAN_POINT ( 'NONE',  ( -44.16309181155855157, 245.9948905683720284, 6.410867750099241924 ) ) ;
#2307=CARTESIAN_POINT ( 'NONE',  ( -44.16309181155857289, 434.4948905683720568, 6.410867750099241924 ) ) ;
#2310=CARTESIAN_POINT ( 'NONE',  ( -17.35679799567829562, 338.5573905765655809, -16.95518130045146421 ) ) ;
#2312=CARTESIAN_POINT ( 'NONE',  ( -19.19641293061497578, 317.3073905683720000, 14.20200298773971426 ) ) ;
#2314=CARTESIAN_POINT ( 'NONE',  ( -16.84014894278200458, 471.6198905683720000, -11.84573899990672707 ) ) ;
#2319=CARTESIAN_POINT ( 'NONE',  ( -32.01814843081345430, 393.1823905683721136, -16.75240474999999307 ) ) ;
#2321=CARTESIAN_POINT ( 'NONE',  ( -21.03221929538694468, 524.1198905601785327, -18.47759065022572855 ) ) ;
#2322=CARTESIAN_POINT ( 'NONE',  ( -38.17536295476245556, 342.3073905683721136, -14.20200298773971426 ) ) ;
#2325=CARTESIAN_POINT ( 'NONE',  ( -45.43829269268872650, 514.1823905683719431, 3.332260488124734632 ) ) ;
#2327=CARTESIAN_POINT ( 'NONE',  ( -32.66413529028186247, 314.1823905765655809, 19.99999999999999289 ) ) ;
#2329=CYLINDRICAL_SURFACE ( 'NONE', #16267, 19.99999999999999645 ) ;
#2330=CARTESIAN_POINT ( 'NONE',  ( -42.88789093042844769, 462.9323905683720568, -9.489475012073736337 ) ) ;
#2332=CARTESIAN_POINT ( 'NONE',  ( -32.01814843081345430, 496.0573905683720000, 16.75240474999999307 ) ) ;
#2333=CARTESIAN_POINT ( 'NONE',  ( -32.66413529028185536, 244.1823905765656093, 19.99999999999999289 ) ) ;
#2335=CARTESIAN_POINT ( 'NONE',  ( -11.73070664223725146, 406.0573905765655240, 11.32908994701042005 ) ) ;
#2338=CARTESIAN_POINT ( 'NONE',  ( -48.68588794268872988, 531.9948905765656946, 0.000000000000000000 ) ) ;
#2339=CARTESIAN_POINT ( 'NONE',  ( -45.64106924314019409, 482.9323905765656377, 11.32908994701042538 ) ) ;
#2343=CARTESIAN_POINT ( 'NONE',  ( -19.19641293061497578, 271.9323905683720568, -14.20200298773971603 ) ) ;
#2344=CARTESIAN_POINT ( 'NONE',  ( -47.16347859291443001, 257.8698905601785327, 7.653668647301805628 ) ) ;
#2346=CARTESIAN_POINT ( 'NONE',  ( -35.09675569278795848, 453.4948905683720568, -15.47720386886985544 ) ) ;
#2347=CARTESIAN_POINT ( 'NONE',  ( -40.01497788969913927, 330.4323905765655809, -16.95518130045146421 ) ) ;
#2348=CARTESIAN_POINT ( 'NONE',  ( -28.68588794268870501, 272.8698905683720000, -16.75240474999999307 ) ) ;
#2349=ADVANCED_FACE ( 'NONE', ( #12979 ), #20992, .T. ) ;
#2351=EDGE_LOOP ( 'NONE', ( #17827, #14649, #19605, #7935 ) ) ;
#2352=CARTESIAN_POINT ( 'NONE',  ( -35.09675569278795848, 493.4948905683720568, -15.47720386886985544 ) ) ;
#2356=CARTESIAN_POINT ( 'NONE',  ( -47.16347859291444422, 366.6198905601784759, -7.653668647301793193 ) ) ;
#2357=CARTESIAN_POINT ( 'NONE',  ( -38.17536295476243424, 235.4323905683720284, 14.20200298773971781 ) ) ;
#2359=CARTESIAN_POINT ( 'NONE',  ( -43.68588794268873698, 573.2448905601785327, 0.000000000000000000 ) ) ;
#2360=CARTESIAN_POINT ( 'NONE',  ( -21.03221929538693757, 478.8698905765656377, -18.47759065022572855 ) ) ;
#2361=CARTESIAN_POINT ( 'NONE',  ( -36.33955658999051508, 389.1198905601784759, 18.47759065022572500 ) ) ;
#2363=CARTESIAN_POINT ( 'NONE',  ( -11.93348319268870661, 230.0573905683720568, 3.332260488124728859 ) ) ;
#2365=CARTESIAN_POINT ( 'NONE',  ( -42.88789093042845479, 526.3073905683720568, 9.489475012073736337 ) ) ;
#2367=CARTESIAN_POINT ( 'NONE',  ( -44.16309181155855867, 253.2448905683720284, -6.410867750099231266 ) ) ;
#2368=CARTESIAN_POINT ( 'NONE',  ( -38.17536295476244845, 346.9323905683720568, 14.20200298773971781 ) ) ;
#2369=CARTESIAN_POINT ( 'NONE',  ( -36.33955658999052929, 469.1198905601784759, 18.47759065022572500 ) ) ;
#2370=CARTESIAN_POINT ( 'NONE',  ( -14.48388495494900496, 397.9323905683719431, 9.489475012073732785 ) ) ;
#2372=CARTESIAN_POINT ( 'NONE',  ( -32.66413529028187668, 379.4323905601785327, 19.99999999999999289 ) ) ;
#2374=ORIENTED_EDGE ( 'NONE', *, *, #11940, .T. ) ;
#2375=DIRECTION ( 'NONE',  ( 0.000000000000000000, 0.000000000000000000, 1.000000000000000000 ) ) ;
#2378=CARTESIAN_POINT ( 'NONE',  ( -11.93348319268873858, 500.3698905683720000, -2.051577885510841163E-15 ) ) ;
#2379=CARTESIAN_POINT ( 'NONE',  ( -48.68588794268870146, 297.2448905601784759, 0.000000000000000000 ) ) ;
#2380=EDGE_LOOP ( 'NONE', ( #1962, #16194, #18482, #2961 ) ) ;
#2381=CARTESIAN_POINT ( 'NONE',  ( -32.01814843081344009, 303.1823905683720568, -16.75240474999999307 ) ) ;
#2383=CARTESIAN_POINT ( 'NONE',  ( -16.84014894278199037, 350.1198905683720568, -11.84573899990672707 ) ) ;
#2384=CARTESIAN_POINT ( 'NONE',  ( -32.01814843081344719, 346.0573905683721136, 16.75240474999999307 ) ) ;
#2385=CARTESIAN_POINT ( 'NONE',  ( -45.64106924314017988, 281.0573905765656377, -11.32908994701042715 ) ) ;
#2387=CARTESIAN_POINT ( 'NONE',  ( -45.43829269268869808, 253.5573905683720000, -3.332260488124726638 ) ) ;
#2388=CARTESIAN_POINT ( 'NONE',  ( -24.70764059509556176, 464.8073905765656377, 19.99999999999998934 ) ) ;
#2390=CARTESIAN_POINT ( 'NONE',  ( -14.48388495494900496, 391.3073905683720000, -9.489475012073736337 ) ) ;
#2393=CARTESIAN_POINT ( 'NONE',  ( -42.82802356641965957, 355.9948905601784759, -14.14213562373094746 ) ) ;
#2395=CARTESIAN_POINT ( 'NONE',  ( -19.19641293061497578, 308.8073905683721136, 14.20200298773971426 ) ) ;
#2396=CARTESIAN_POINT ( 'NONE',  ( -14.48388495494901385, 469.8073905683719431, -9.489475012073736337 ) ) ;
#2398=CARTESIAN_POINT ( 'NONE',  ( -24.70764059509557597, 474.4323905601785327, -19.99999999999999289 ) ) ;
#2399=CARTESIAN_POINT ( 'NONE',  ( -11.93348319268871371, 288.5573905683720000, 3.332260488124728415 ) ) ;
#2400=EDGE_CURVE ( 'NONE', #13902, #14194, #12740, .T. ) ;
#2402=CARTESIAN_POINT ( 'NONE',  ( -8.685887942688724550, 376.9948905765655809, -2.449293598294705724E-15 ) ) ;
#2406=CARTESIAN_POINT ( 'NONE',  ( -10.20829729246298356, 342.8698905601785327, -7.653668647301794969 ) ) ;
#2407=CARTESIAN_POINT ( 'NONE',  ( -28.68588794268870856, 301.3698905683720568, -16.75240474999999307 ) ) ;
#2409=CARTESIAN_POINT ( 'NONE',  ( -45.43829269268871229, 385.0573905683720000, -3.332260488124726638 ) ) ;
#2411=EDGE_CURVE ( 'NONE', #629, #2934, #19362, .T. ) ;
#2412=CARTESIAN_POINT ( 'NONE',  ( -24.70764059509556887, 514.8073905765656946, 19.99999999999998934 ) ) ;
#2413=CARTESIAN_POINT ( 'NONE',  ( -13.20868407381886556, 409.4948905683720000, -6.410867750099233042 ) ) ;
#2414=CARTESIAN_POINT ( 'NONE',  ( -19.19641293061496867, 238.8073905683720000, 14.20200298773971426 ) ) ;
#2415=CARTESIAN_POINT ( 'NONE',  ( -42.88789093042844058, 414.8073905683720000, 9.489475012073734561 ) ) ;
#2416=CARTESIAN_POINT ( 'NONE',  ( -28.68588794268871212, 339.4948905765656377, -19.99999999999999289 ) ) ;
#2418=CARTESIAN_POINT ( 'NONE',  ( -16.84014894278198327, 300.1198905683720000, -11.84573899990672707 ) ) ;
#2419=DIRECTION ( 'NONE',  ( 0.000000000000000000, 0.000000000000000000, 1.000000000000000000 ) ) ;
#2420=CARTESIAN_POINT ( 'NONE',  ( -11.93348319268873503, 470.3698905683720568, -2.051577885510841163E-15 ) ) ;
#2421=CARTESIAN_POINT ( 'NONE',  ( -11.73070664223726567, 516.0573905765655809, 11.32908994701042005 ) ) ;
#2424=CARTESIAN_POINT ( 'NONE',  ( -19.19641293061498288, 368.8073905683720000, 14.20200298773971426 ) ) ;
#2426=CARTESIAN_POINT ( 'NONE',  ( -28.68588794268873343, 529.7448905601785327, 19.99999999999999289 ) ) ;
#2427=CARTESIAN_POINT ( 'NONE',  ( -45.43829269268870519, 343.5573905683720000, -3.332260488124726194 ) ) ;
#2429=ORIENTED_EDGE ( 'NONE', *, *, #331, .F. ) ;
#2430=CARTESIAN_POINT ( 'NONE',  ( -28.68588794268873343, 501.3698905683721136, -16.75240474999999307 ) ) ;
#2433=CARTESIAN_POINT ( 'NONE',  ( -45.64106924314017988, 381.0573905765656377, -11.32908994701042538 ) ) ;
#2435=CARTESIAN_POINT ( 'NONE',  ( -8.685887942688625074, 287.3073905765656377, -3.978247347592952732 ) ) ;
#2437=CARTESIAN_POINT ( 'NONE',  ( -14.48388495494900852, 457.9323905683720568, 9.489475012073732785 ) ) ;
#2439=CARTESIAN_POINT ( 'NONE',  ( -25.35362745456399480, 476.6823905683720000, 16.75240474999998952 ) ) ;
#2441=CARTESIAN_POINT ( 'NONE',  ( -8.685887942688726326, 406.6823905765656377, 3.978247347593161010 ) ) ;
#2443=CARTESIAN_POINT ( 'NONE',  ( -28.68588794268874054, 573.2448905601785327, 0.000000000000000000 ) ) ;
#2444=FACE_OUTER_BOUND ( 'NONE', #15870, .T. ) ;
#2445=CARTESIAN_POINT ( 'NONE',  ( -28.68588794268874054, 573.2448905601785327, 0.000000000000000000 ) ) ;
#2451=CARTESIAN_POINT ( 'NONE',  ( -45.43829269268869808, 285.6823905683720000, 3.332260488124734632 ) ) ;
#2452=CARTESIAN_POINT ( 'NONE',  ( -48.68588794268871567, 401.9948905765656377, 0.000000000000000000 ) ) ;
#2453=CARTESIAN_POINT ( 'NONE',  ( -44.16309181155857289, 445.9948905683720568, 6.410867750099241924 ) ) ;
#2454=LINE ( 'NONE', #18989, #5756 ) ;
#2455=CARTESIAN_POINT ( 'NONE',  ( -13.20868407381884779, 279.7448905683720568, 6.410867750099229490 ) ) ;
#2457=EDGE_LOOP ( 'NONE', ( #14566, #789, #6059, #11333 ) ) ;
#2458=CARTESIAN_POINT ( 'NONE',  ( -32.66413529028188378, 479.8073905765656377, -19.99999999999999289 ) ) ;
#2460=CARTESIAN_POINT ( 'NONE',  ( -14.48388495494901029, 481.3073905683720000, -9.489475012073734561 ) ) ;
#2463=CARTESIAN_POINT ( 'NONE',  ( -11.73070664223724968, 363.1823905601784759, -11.32908994701042538 ) ) ;
#2464=CARTESIAN_POINT ( 'NONE',  ( -13.20868407381884602, 238.2448905683720000, 6.410867750099229490 ) ) ;
#2467=CARTESIAN_POINT ( 'NONE',  ( -11.73070664223725856, 466.0573905765656946, 11.32908994701042005 ) ) ;
#2471=CARTESIAN_POINT ( 'NONE',  ( -11.93348319268874036, 520.6823905683719431, -3.332260488124732856 ) ) ;
#2472=CARTESIAN_POINT ( 'NONE',  ( -14.54375231895776821, 375.7448905765656377, 14.14213562373094568 ) ) ;
#2473=CARTESIAN_POINT ( 'NONE',  ( -16.84014894278197261, 247.6198905683720284, 11.84573899990672530 ) ) ;
#2474=CARTESIAN_POINT ( 'NONE',  ( -25.35362745456397704, 338.1823905683720000, 16.75240474999998952 ) ) ;
#2475=CARTESIAN_POINT ( 'NONE',  ( -8.685887942688742314, 573.2448905601785327, 2.449293598294706119E-15 ) ) ;
#2476=CARTESIAN_POINT ( 'NONE',  ( -24.70764059509554045, 304.8073905765655809, 19.99999999999998934 ) ) ;
#2477=CARTESIAN_POINT ( 'NONE',  ( -42.88789093042843348, 382.9323905683720568, -9.489475012073736337 ) ) ;
#2478=CARTESIAN_POINT ( 'NONE',  ( -11.73070664223724258, 326.0573905765656377, 11.32908994701042005 ) ) ;
#2480=CARTESIAN_POINT ( 'NONE',  ( -45.64106924314018698, 388.1823905601784759, 11.32908994701042715 ) ) ;
#2485=CARTESIAN_POINT ( 'NONE',  ( -40.53162694259545873, 506.6198905683721136, 11.84573899990672885 ) ) ;
#2486=CARTESIAN_POINT ( 'NONE',  ( -40.01497788969912506, 293.5573905765655809, 16.95518130045146776 ) ) ;
#2488=CARTESIAN_POINT ( 'NONE',  ( -11.93348319268871371, 300.0573905683720568, 3.332260488124728859 ) ) ;
#2491=ORIENTED_EDGE ( 'NONE', *, *, #5373, .T. ) ;
#2492=CARTESIAN_POINT ( 'NONE',  ( -44.16309181155856578, 344.4948905683720000, 6.410867750099241924 ) ) ;
#2493=CARTESIAN_POINT ( 'NONE',  ( -19.19641293061497933, 340.4323905683720568, -14.20200298773971603 ) ) ;
#2494=CARTESIAN_POINT ( 'NONE',  ( -21.03221929538691626, 288.8698905765656377, -18.47759065022572855 ) ) ;
#2495=LINE ( 'NONE', #2711, #8951 ) ;
#2496=CARTESIAN_POINT ( 'NONE',  ( -22.27502019258946220, 246.9948905683720284, 15.47720386886985189 ) ) ;
#2497=CARTESIAN_POINT ( 'NONE',  ( -47.16347859291445843, 462.6198905765655809, 7.653668647301805628 ) ) ;
#2498=CARTESIAN_POINT ( 'NONE',  ( -38.17536295476245556, 396.9323905683721136, 14.20200298773971781 ) ) ;
#2500=CARTESIAN_POINT ( 'NONE',  ( -11.73070664223726034, 447.9323905765656946, -11.32908994701042538 ) ) ;
#2502=CARTESIAN_POINT ( 'NONE',  ( -25.35362745456400191, 441.0573905683720000, -16.75240474999999307 ) ) ;
#2505=CARTESIAN_POINT ( 'NONE',  ( -45.64106924314019409, 448.1823905601785327, 11.32908994701042715 ) ) ;
#2511=CARTESIAN_POINT ( 'NONE',  ( -36.33955658999050087, 325.3698905601784759, -18.47759065022572855 ) ) ;
#2512=CARTESIAN_POINT ( 'NONE',  ( -45.43829269268869808, 304.1823905683720568, 3.332260488124734632 ) ) ;
#2513=CARTESIAN_POINT ( 'NONE',  ( -44.16309181155856578, 355.9948905683720000, 6.410867750099241924 ) ) ;
#2515=CARTESIAN_POINT ( 'NONE',  ( -11.73070664223727100, 527.9323905765655809, -11.32908994701042715 ) ) ;
#2516=CARTESIAN_POINT ( 'NONE',  ( -19.19641293061498999, 400.4323905683720568, -14.20200298773971603 ) ) ;
#2517=CARTESIAN_POINT ( 'NONE',  ( -14.48388495494898365, 231.3073905683720000, -9.489475012073736337 ) ) ;
#2519=CARTESIAN_POINT ( 'NONE',  ( -38.17536295476245556, 405.4323905683721136, 14.20200298773971781 ) ) ;
#2521=CARTESIAN_POINT ( 'NONE',  ( -48.68588794268870856, 341.6823905765656946, -3.978247347593158345 ) ) ;
#2522=CARTESIAN_POINT ( 'NONE',  ( -28.68588794268871212, 324.7448905601784759, -19.99999999999999289 ) ) ;
#2523=CARTESIAN_POINT ( 'NONE',  ( -16.84014894278198327, 310.1198905683720000, -11.84573899990672707 ) ) ;
#2524=CARTESIAN_POINT ( 'NONE',  ( -38.17536295476246977, 463.8073905683720000, -14.20200298773971426 ) ) ;
#2525=CARTESIAN_POINT ( 'NONE',  ( -40.01497788969915348, 513.5573905765656946, 16.95518130045146776 ) ) ;
#2528=DIRECTION ( 'NONE',  ( -1.191790137725560488E-16, 1.000000000000000000, -0.000000000000000000 ) ) ;
#2529=CARTESIAN_POINT ( 'NONE',  ( -42.88789093042843348, 364.4323905683720568, -9.489475012073736337 ) ) ;
#2531=CARTESIAN_POINT ( 'NONE',  ( -17.35679799567830983, 500.6823905601785327, 16.95518130045146421 ) ) ;
#2532=CARTESIAN_POINT ( 'NONE',  ( -35.09675569278794427, 341.9948905683720000, -15.47720386886985544 ) ) ;
#2534=CARTESIAN_POINT ( 'NONE',  ( -32.01814843081346851, 511.6823905683720000, -16.75240474999999307 ) ) ;
#2537=CARTESIAN_POINT ( 'NONE',  ( -45.43829269268871940, 415.0573905683721136, -3.332260488124726638 ) ) ;
#2540=CARTESIAN_POINT ( 'NONE',  ( -45.43829269268871940, 464.1823905683720568, 3.332260488124734632 ) ) ;
#2542=CARTESIAN_POINT ( 'NONE',  ( -13.20868407381887266, 459.4948905683720568, -6.410867750099233042 ) ) ;
#2543=CARTESIAN_POINT ( 'NONE',  ( -48.68588794268869435, 241.9948905765656377, 0.000000000000000000 ) ) ;
#2545=CARTESIAN_POINT ( 'NONE',  ( -17.35679799567829562, 395.4323905765655809, 16.95518130045146421 ) ) ;
#2547=CARTESIAN_POINT ( 'NONE',  ( -48.68588794268870856, 371.9948905765655809, 0.000000000000000000 ) ) ;
#2553=CARTESIAN_POINT ( 'NONE',  ( -48.68588794268869435, 237.2448905601785043, 0.000000000000000000 ) ) ;
#2555=CARTESIAN_POINT ( 'NONE',  ( -19.19641293061497223, 278.8073905683720000, 14.20200298773971426 ) ) ;
#2557=CARTESIAN_POINT ( 'NONE',  ( -13.20868407381886911, 430.9948905683720568, -6.410867750099233042 ) ) ;
#2558=CARTESIAN_POINT ( 'NONE',  ( -10.20829729246299067, 397.6198905765655809, -7.653668647301794969 ) ) ;
#2559=CARTESIAN_POINT ( 'NONE',  ( -11.93348319268871194, 280.0573905683720568, 3.332260488124728415 ) ) ;
#2561=CARTESIAN_POINT ( 'NONE',  ( -11.73070664223726389, 477.9323905765656946, -11.32908994701042538 ) ) ;
#2563=CARTESIAN_POINT ( 'NONE',  ( -44.16309181155857999, 485.9948905683720568, 6.410867750099241924 ) ) ;
#2567=CARTESIAN_POINT ( 'NONE',  ( -17.35679799567829562, 363.8073905601784759, -16.95518130045146421 ) ) ;
#2568=CARTESIAN_POINT ( 'NONE',  ( -45.43829269268869098, 233.5573905683720568, -3.332260488124726194 ) ) ;
#2570=( BOUNDED_CURVE ( )  B_SPLINE_CURVE ( 2, ( #14302, #15914, #11134, #19358, #1105, #15704, #9509, #20561, #786, #6053, #19256, #11022, #891, #17632, #12340, #14407, #20989 ),
 .UNSPECIFIED., .F., .T. ) 
 B_SPLINE_CURVE_WITH_KNOTS ( ( 3, 2, 2, 2, 2, 2, 2, 2, 3 ),
 ( 0.06250000000000005551, 0.06445312500000009714, 0.06640625000000015266, 0.06835937500000019429, 0.07031250000000024980, 0.07226562500000029143, 0.07421875000000033307, 0.07617187500000038858, 0.07812500000000043021 ),
 .UNSPECIFIED. ) 
 CURVE ( )  GEOMETRIC_REPRESENTATION_ITEM ( )  RATIONAL_B_SPLINE_CURVE ( ( 0.9999999999999994449, 0.9807852804032309857, 1.000000000000000000, 0.9807852804032304306, 1.000000000000000000, 0.9807852804032304306, 1.000000000000000000, 0.9807852804032304306, 1.000000000000000000, 0.9807852804032304306, 1.000000000000000000, 0.9807852804032304306, 1.000000000000000000, 0.9807852804032304306, 1.000000000000000000, 0.9807852804032262117, 1.000000000000004219 ) ) 
 REPRESENTATION_ITEM ( '' )  );
#2571=CARTESIAN_POINT ( 'NONE',  ( -40.53162694259545873, 522.6198905683720568, -11.84573899990672707 ) ) ;
#2573=CARTESIAN_POINT ( 'NONE',  ( -8.685887942688736985, 466.6823905765656946, 3.978247347593161010 ) ) ;
#2575=CARTESIAN_POINT ( 'NONE',  ( -36.33955658999050797, 283.8698905765656377, 18.47759065022572500 ) ) ;
#2576=CARTESIAN_POINT ( 'NONE',  ( -42.82802356641967378, 455.9948905601784759, -14.14213562373094746 ) ) ;
#2579=CARTESIAN_POINT ( 'NONE',  ( -28.68588794268873698, 522.8698905683719431, -16.75240474999999307 ) ) ;
#2582=CARTESIAN_POINT ( 'NONE',  ( -11.93348319268870839, 248.5573905683719715, 3.332260488124728415 ) ) ;
#2583=CARTESIAN_POINT ( 'NONE',  ( -44.16309181155856578, 345.9948905683720000, 6.410867750099241924 ) ) ;
#2584=DIRECTION ( 'NONE',  ( -1.191790137725560488E-16, 1.000000000000000000, -0.000000000000000000 ) ) ;
#2585=CARTESIAN_POINT ( 'NONE',  ( -40.01497788969912506, 303.5573905765656377, 16.95518130045146776 ) ) ;
#2586=CARTESIAN_POINT ( 'NONE',  ( -13.20868407381886378, 389.4948905683720000, -6.410867750099233042 ) ) ;
#2588=CARTESIAN_POINT ( 'NONE',  ( -21.03221929538691271, 380.3698905601784759, 18.47759065022572500 ) ) ;
#2591=ORIENTED_EDGE ( 'NONE', *, *, #21349, .F. ) ;
#2593=CARTESIAN_POINT ( 'NONE',  ( -14.48388495494901562, 499.4323905683720000, 9.489475012073732785 ) ) ;
#2594=CARTESIAN_POINT ( 'NONE',  ( -28.68588794268874054, 573.2448905601785327, 0.000000000000000000 ) ) ;
#2596=CARTESIAN_POINT ( 'NONE',  ( -38.17536295476244135, 306.9323905683719431, 14.20200298773971781 ) ) ;
#2598=CARTESIAN_POINT ( 'NONE',  ( -22.27502019258948707, 350.7448905683720568, -15.47720386886985544 ) ) ;
#2599=CARTESIAN_POINT ( 'NONE',  ( -35.09675569278794427, 341.9948905683720000, -15.47720386886985544 ) ) ;
#2600=CARTESIAN_POINT ( 'NONE',  ( -10.20829729246297646, 286.3698905765655809, 7.653668647301790529 ) ) ;
#2601=CYLINDRICAL_SURFACE ( 'NONE', #3439, 19.99999999999999645 ) ;
#2602=CARTESIAN_POINT ( 'NONE',  ( -11.93348319268870661, 238.8698905683720568, -2.051577885510841163E-15 ) ) ;
#2603=CARTESIAN_POINT ( 'NONE',  ( -21.03221929538690560, 224.1198905601785043, -18.47759065022572855 ) ) ;
#2604=CARTESIAN_POINT ( 'NONE',  ( -22.27502019258949062, 392.2448905683720568, -15.47720386886985544 ) ) ;
#2608=CARTESIAN_POINT ( 'NONE',  ( -11.93348319268873148, 449.1823905683720000, -3.332260488124732856 ) ) ;
#2610=CARTESIAN_POINT ( 'NONE',  ( -45.64106924314019409, 438.1823905601784190, 11.32908994701042715 ) ) ;
#2613=VERTEX_POINT ( 'NONE', #7542 ) ;
#2616=CARTESIAN_POINT ( 'NONE',  ( -45.64106924314017988, 316.3073905601784759, -11.32908994701042715 ) ) ;
#2617=EDGE_CURVE ( 'NONE', #2082, #10139, #12035, .T. ) ;
#2618=ADVANCED_FACE ( 'NONE', ( #20756 ), #9061, .F. ) ;
#2619=CARTESIAN_POINT ( 'NONE',  ( -35.09675569278794427, 363.4948905683720568, -15.47720386886985544 ) ) ;
#2621=CARTESIAN_POINT ( 'NONE',  ( -48.68588794268872988, 521.6823905765656946, -3.978247347593158345 ) ) ;
#2622=CARTESIAN_POINT ( 'NONE',  ( -32.01814843081345430, 401.6823905683720000, -16.75240474999999307 ) ) ;
#2623=CARTESIAN_POINT ( 'NONE',  ( -11.93348319268870661, 250.3698905683720000, -2.051577885510841163E-15 ) ) ;
#2624=CARTESIAN_POINT ( 'NONE',  ( -25.35362745456398414, 396.6823905683720000, 16.75240474999998952 ) ) ;
#2625=B_SPLINE_CURVE_WITH_KNOTS ( 'NONE', 3,
 ( #11318, #8168, #1488, #12738, #1596, #1383, #17913, #17603, #17708, #14800, #21384, #7853, #9380, #15998, #20960, #6131, #19330, #9486 ),
 .UNSPECIFIED., .F., .F.,
 ( 4, 2, 2, 2, 2, 2, 2, 2, 4 ),
 ( 0.1916473082429159536, 0.2301913947125514559, 0.2687354811821869305, 0.3072795676518224606, 0.3458236541214579907, 0.3843677405910934652, 0.4229118270607289398, 0.4614559135303645254, 0.5000000000000000000 ),
 .UNSPECIFIED. ) ;
#2626=CARTESIAN_POINT ( 'NONE',  ( -8.685887942688720997, 336.9948905765656377, -2.449293598294705724E-15 ) ) ;
#2627=CARTESIAN_POINT ( 'NONE',  ( -36.33955658999050087, 325.3698905601784759, -18.47759065022572855 ) ) ;
#2628=CARTESIAN_POINT ( 'NONE',  ( -32.01814843081344009, 316.0573905683720000, 16.75240474999999307 ) ) ;
#2630=CARTESIAN_POINT ( 'NONE',  ( -32.01814843081346140, 453.1823905683720568, -16.75240474999999307 ) ) ;
#2632=CARTESIAN_POINT ( 'NONE',  ( -48.68588794268872988, 511.9948905765656377, 0.000000000000000000 ) ) ;
#2635=CARTESIAN_POINT ( 'NONE',  ( -22.27502019258950128, 500.7448905683720000, -15.47720386886985544 ) ) ;
#2636=CARTESIAN_POINT ( 'NONE',  ( -17.35679799567830983, 510.6823905601785327, 16.95518130045146421 ) ) ;
#2637=CARTESIAN_POINT ( 'NONE',  ( -42.88789093042842637, 324.8073905683720000, 9.489475012073736337 ) ) ;
#2639=CARTESIAN_POINT ( 'NONE',  ( -45.43829269268872650, 513.5573905683719431, -3.332260488124726194 ) ) ;
#2640=VERTEX_POINT ( 'NONE', #15790 ) ;
#2644=CARTESIAN_POINT ( 'NONE',  ( -28.68588794268872277, 432.8698905683720568, -16.75240474999999307 ) ) ;
#2647=CARTESIAN_POINT ( 'NONE',  ( -38.17536295476246977, 472.3073905683720568, -14.20200298773971426 ) ) ;
#2649=CARTESIAN_POINT ( 'NONE',  ( -11.93348319268873325, 458.8698905683720000, -2.051577885510841163E-15 ) ) ;
#2651=CARTESIAN_POINT ( 'NONE',  ( -47.16347859291445133, 411.3698905765656377, -7.653668647301793193 ) ) ;
#2654=CARTESIAN_POINT ( 'NONE',  ( -8.685887942688642838, 437.3073905765655809, -3.978247347592952732 ) ) ;
#2655=CARTESIAN_POINT ( 'NONE',  ( -48.68588794268882936, 482.3073905765655240, 3.978247347592901217 ) ) ;
#2659=CARTESIAN_POINT ( 'NONE',  ( -42.82802356641964536, 248.4948905601784759, 14.14213562373094923 ) ) ;
#2661=CARTESIAN_POINT ( 'NONE',  ( -8.685887942688735208, 476.9948905765656377, -2.449293598294705724E-15 ) ) ;
#2662=CARTESIAN_POINT ( 'NONE',  ( -22.27502019258949417, 432.2448905683720000, -15.47720386886985544 ) ) ;
#2664=CARTESIAN_POINT ( 'NONE',  ( -14.48388495494898542, 259.4323905683720000, 9.489475012073732785 ) ) ;
#2665=ORIENTED_EDGE ( 'NONE', *, *, #635, .T. ) ;
#2667=FACE_OUTER_BOUND ( 'NONE', #17699, .T. ) ;
#2668=EDGE_LOOP ( 'NONE', ( #11517, #43, #4733, #6560 ) ) ;
#2669=CARTESIAN_POINT ( 'NONE',  ( -25.35362745456400546, 482.5573905683720000, -16.75240474999999307 ) ) ;
#2673=CARTESIAN_POINT ( 'NONE',  ( -14.54375231895778775, 525.7448905765655809, 14.14213562373094568 ) ) ;
#2674=CARTESIAN_POINT ( 'NONE',  ( -14.48388495494898365, 237.9323905683720000, 9.489475012073732785 ) ) ;
#2676=CARTESIAN_POINT ( 'NONE',  ( -14.48388495494901740, 519.8073905683719431, -9.489475012073734561 ) ) ;
#2679=CARTESIAN_POINT ( 'NONE',  ( -10.20829729246299777, 457.6198905765656377, -7.653668647301794969 ) ) ;
#2680=CARTESIAN_POINT ( 'NONE',  ( -48.68588794268887199, 347.5573905601784190, 3.978247347592742678 ) ) ;
#2683=CARTESIAN_POINT ( 'NONE',  ( -17.35679799567830628, 453.8073905601784759, -16.95518130045146421 ) ) ;
#2684=CARTESIAN_POINT ( 'NONE',  ( -11.93348319268870483, 230.3698905683720284, -2.051577885510841163E-15 ) ) ;
#2685=CARTESIAN_POINT ( 'NONE',  ( -32.01814843081346851, 507.5573905683720568, 16.75240474999999307 ) ) ;
#2687=CARTESIAN_POINT ( 'NONE',  ( -14.48388495494898365, 229.8073905683720000, -9.489475012073736337 ) ) ;
#2688=CARTESIAN_POINT ( 'NONE',  ( -40.53162694259543741, 336.6198905683720000, 11.84573899990672885 ) ) ;
#2691=CARTESIAN_POINT ( 'NONE',  ( -32.66413529028186247, 274.1823905765656377, 19.99999999999999289 ) ) ;
#2694=CARTESIAN_POINT ( 'NONE',  ( -19.19641293061498644, 377.3073905683720568, 14.20200298773971426 ) ) ;
#2695=CARTESIAN_POINT ( 'NONE',  ( -36.33955658999050797, 323.8698905765656377, 18.47759065022572500 ) ) ;
#2697=( BOUNDED_CURVE ( )  B_SPLINE_CURVE ( 2, ( #12849, #9696, #17711, #7959, #6134, #4725, #3007, #21274, #1386, #16209, #11107, #6446, #19333, #16421, #21173, #4828, #7857 ),
 .UNSPECIFIED., .F., .T. ) 
 B_SPLINE_CURVE_WITH_KNOTS ( ( 3, 2, 2, 2, 2, 2, 2, 2, 3 ),
 ( 0.2812500000000000555, 0.2832031250000000555, 0.2851562500000000555, 0.2871093750000000555, 0.2890625000000001110, 0.2910156250000001110, 0.2929687500000001110, 0.2949218750000001110, 0.2968750000000001110 ),
 .UNSPECIFIED. ) 
 CURVE ( )  GEOMETRIC_REPRESENTATION_ITEM ( )  RATIONAL_B_SPLINE_CURVE ( ( 0.9999999999999994449, 0.9807852804032309857, 1.000000000000000000, 0.9807852804032304306, 1.000000000000000000, 0.9807852804032304306, 1.000000000000000000, 0.9807852804032304306, 1.000000000000000000, 0.9807852804032304306, 1.000000000000000000, 0.9807852804032304306, 1.000000000000000000, 0.9807852804032304306, 1.000000000000000000, 0.9807852804032293204, 1.000000000000001110 ) ) 
 REPRESENTATION_ITEM ( '' )  );
#2698=CARTESIAN_POINT ( 'NONE',  ( -32.66413529028187668, 389.4323905601784759, 19.99999999999999289 ) ) ;
#2699=EDGE_CURVE ( 'NONE', #7041, #6110, #186, .T. ) ;
#2703=CARTESIAN_POINT ( 'NONE',  ( -32.01814843081346851, 513.1823905683720568, -16.75240474999999307 ) ) ;
#2705=ORIENTED_EDGE ( 'NONE', *, *, #13259, .F. ) ;
#2706=CARTESIAN_POINT ( 'NONE',  ( -32.01814843081344009, 313.1823905683720000, -16.75240474999999307 ) ) ;
#2707=ORIENTED_EDGE ( 'NONE', *, *, #19267, .F. ) ;
#2708=CARTESIAN_POINT ( 'NONE',  ( -11.93348319268871727, 328.8698905683720000, -2.051577885510841163E-15 ) ) ;
#2709=CARTESIAN_POINT ( 'NONE',  ( -42.88789093042843348, 354.8073905683720568, 9.489475012073734561 ) ) ;
#2710=CARTESIAN_POINT ( 'NONE',  ( -45.64106924314017988, 271.0573905765656946, -11.32908994701042715 ) ) ;
#2711=CARTESIAN_POINT ( 'NONE',  ( -48.68588794268873698, 573.2448905601785327, 0.000000000000000000 ) ) ;
#2712=CARTESIAN_POINT ( 'NONE',  ( -44.16309181155855867, 243.2448905683720000, -6.410867750099231266 ) ) ;
#2713=CARTESIAN_POINT ( 'NONE',  ( -40.01497788969912506, 225.6823905601784759, -16.95518130045146421 ) ) ;
#2714=CARTESIAN_POINT ( 'NONE',  ( -25.35362745456398414, 398.1823905683720568, 16.75240474999998952 ) ) ;
#2719=AXIS2_PLACEMENT_3D ( 'NONE', #7627, #20840, #6012 ) ;
#2720=CARTESIAN_POINT ( 'NONE',  ( -19.19641293061499354, 440.4323905683720000, -14.20200298773971603 ) ) ;
#2722=CARTESIAN_POINT ( 'NONE',  ( -14.54375231895777709, 450.9948905601784759, 14.14213562373094568 ) ) ;
#2725=AXIS2_PLACEMENT_3D ( 'NONE', #1630, #2826, #14619 ) ;
#2728=CARTESIAN_POINT ( 'NONE',  ( -11.73070664223724791, 333.1823905601784190, -11.32908994701042715 ) ) ;
#2729=CARTESIAN_POINT ( 'NONE',  ( -45.43829269268871229, 365.6823905683720568, 3.332260488124734632 ) ) ;
#2731=CARTESIAN_POINT ( 'NONE',  ( -11.73070664223726745, 497.9323905765655809, -11.32908994701042715 ) ) ;
#2732=CARTESIAN_POINT ( 'NONE',  ( -35.09675569278794427, 381.9948905683720568, -15.47720386886985544 ) ) ;
#2733=CARTESIAN_POINT ( 'NONE',  ( -40.53162694259542320, 244.1198905683720284, -11.84573899990672707 ) ) ;
#2734=CARTESIAN_POINT ( 'NONE',  ( -22.27502019258947996, 396.9948905683720568, 15.47720386886985189 ) ) ;
#2736=CARTESIAN_POINT ( 'NONE',  ( -21.03221929538690560, 335.1198905765655809, 18.47759065022572500 ) ) ;
#2738=CARTESIAN_POINT ( 'NONE',  ( -11.93348319268871549, 309.1823905683720000, -3.332260488124732856 ) ) ;
#2739=CARTESIAN_POINT ( 'NONE',  ( -40.53162694259545162, 454.1198905683720568, -11.84573899990672707 ) ) ;
#2740=CARTESIAN_POINT ( 'NONE',  ( -24.70764059509555821, 460.0573905601785327, 19.99999999999998934 ) ) ;
#2743=CARTESIAN_POINT ( 'NONE',  ( -14.48388495494899786, 359.4323905683719431, 9.489475012073732785 ) ) ;
#2744=CARTESIAN_POINT ( 'NONE',  ( -25.35362745456400901, 501.0573905683720568, -16.75240474999999307 ) ) ;
#2745=CARTESIAN_POINT ( 'NONE',  ( -8.685887942688740537, 512.5573905601785327, -3.978247347593165895 ) ) ;
#2746=CARTESIAN_POINT ( 'NONE',  ( -38.17536295476245556, 332.3073905683720000, -14.20200298773971426 ) ) ;
#2749=CARTESIAN_POINT ( 'NONE',  ( -40.01497788969916058, 525.6823905601785327, -16.95518130045146421 ) ) ;
#2752=EDGE_CURVE ( 'NONE', #349, #8848, #3971, .T. ) ;
#2755=CARTESIAN_POINT ( 'NONE',  ( -40.53162694259544452, 416.6198905683720000, 11.84573899990672885 ) ) ;
#2758=CARTESIAN_POINT ( 'NONE',  ( -40.53162694259545162, 472.6198905683720000, -11.84573899990672707 ) ) ;
#2760=CARTESIAN_POINT ( 'NONE',  ( -45.43829269268872650, 464.1823905683720000, 3.332260488124734632 ) ) ;
#2763=CARTESIAN_POINT ( 'NONE',  ( -10.20829729246299067, 397.6198905765655809, -7.653668647301794969 ) ) ;
#2765=DIRECTION ( 'NONE',  ( -1.191790137725560488E-16, 1.000000000000000000, -0.000000000000000000 ) ) ;
#2767=CARTESIAN_POINT ( 'NONE',  ( -10.20829729246297468, 256.3698905765656377, 7.653668647301790529 ) ) ;
#2771=CARTESIAN_POINT ( 'NONE',  ( -45.43280446313950449, 223.9102039777116602, 0.4287796227366179602 ) ) ;
#2772=CARTESIAN_POINT ( 'NONE',  ( -8.685887942688708563, 241.9323905601784475, 3.978247347593161010 ) ) ;
#2774=CARTESIAN_POINT ( 'NONE',  ( -45.43829269268871940, 425.3698905683720568, 0.000000000000000000 ) ) ;
#2776=CARTESIAN_POINT ( 'NONE',  ( -13.20868407381884779, 259.7448905683720000, 6.410867750099229490 ) ) ;
#2780=CARTESIAN_POINT ( 'NONE',  ( -22.27502019258948707, 458.4948905683720568, 15.47720386886985189 ) ) ;
#2781=CARTESIAN_POINT ( 'NONE',  ( -40.01497788969912506, 230.4323905765656377, -16.95518130045146421 ) ) ;
#2783=CARTESIAN_POINT ( 'NONE',  ( -10.20829729246298534, 362.8698905601784759, -7.653668647301794969 ) ) ;
#2784=CARTESIAN_POINT ( 'NONE',  ( -40.53162694259542320, 232.6198905683720000, -11.84573899990672707 ) ) ;
#2786=CARTESIAN_POINT ( 'NONE',  ( -19.19641293061500420, 520.4323905683719431, -14.20200298773971603 ) ) ;
#2787=DIRECTION ( 'NONE',  ( -1.000000000000000000, -0.000000000000000000, -0.000000000000000000 ) ) ;
#2788=CARTESIAN_POINT ( 'NONE',  ( -36.33955658999052929, 463.8698905765656377, 18.47759065022572500 ) ) ;
#2790=CARTESIAN_POINT ( 'NONE',  ( -17.35679799567828141, 285.4323905765656377, 16.95518130045146421 ) ) ;
#2793=CARTESIAN_POINT ( 'NONE',  ( -44.16309181155855867, 224.7448905683720568, -6.410867750099231266 ) ) ;
#2795=CARTESIAN_POINT ( 'NONE',  ( -11.93348319268870661, 229.1823905683720284, -3.332260488124732856 ) ) ;
#2796=CARTESIAN_POINT ( 'NONE',  ( -28.68588794268870856, 327.8698905683720000, 16.75240474999999307 ) ) ;
#2797=CARTESIAN_POINT ( 'NONE',  ( -8.685887942688717445, 322.2448905601784759, -2.449293598294705724E-15 ) ) ;
#2799=CARTESIAN_POINT ( 'NONE',  ( -45.43829269268869808, 315.6823905683720000, 3.332260488124734632 ) ) ;
#2800=CARTESIAN_POINT ( 'NONE',  ( -19.19641293061498644, 387.3073905683720000, 14.20200298773971426 ) ) ;
#2803=CARTESIAN_POINT ( 'NONE',  ( -35.09675569278796559, 533.4948905683720568, -15.47720386886985544 ) ) ;
#2804=VECTOR ( 'NONE', #17124, 1000.000000000000000 ) ;
#2805=CARTESIAN_POINT ( 'NONE',  ( -21.03221929538692692, 384.1198905601784759, -18.47759065022572855 ) ) ;
#2809=CARTESIAN_POINT ( 'NONE',  ( -22.27502019258950128, 492.2448905683720000, -15.47720386886985544 ) ) ;
#2811=EDGE_LOOP ( 'NONE', ( #2591, #8808, #16191, #16987 ) ) ;
#2812=CARTESIAN_POINT ( 'NONE',  ( -45.43829269268870519, 295.3698905683720568, 0.000000000000000000 ) ) ;
#2814=CARTESIAN_POINT ( 'NONE',  ( -22.27502019258948351, 330.7448905683720568, -15.47720386886985544 ) ) ;
#2815=MECHANICAL_DESIGN_GEOMETRIC_PRESENTATION_REPRESENTATION('',(#9005),#17309);
#2816=CARTESIAN_POINT ( 'NONE',  ( -10.20829729246297646, 266.3698905765656377, 7.653668647301790529 ) ) ;
#2817=CYLINDRICAL_SURFACE ( 'NONE', #13121, 19.99999999999999645 ) ;
#2819=CARTESIAN_POINT ( 'NONE',  ( -14.48388495494900141, 389.4323905683720568, 9.489475012073732785 ) ) ;
#2821=CARTESIAN_POINT ( 'NONE',  ( -48.68588794268871567, 447.2448905601785327, 0.000000000000000000 ) ) ;
#2822=FACE_OUTER_BOUND ( 'NONE', #16266, .T. ) ;
#2823=( BOUNDED_CURVE ( )  B_SPLINE_CURVE ( 2, ( #17250, #20815, #15741, #9014, #14016, #15529, #19080, #18966, #10953, #2327, #12596, #4263, #15847, #5768, #15952, #5665, #14228 ),
 .UNSPECIFIED., .F., .T. ) 
 B_SPLINE_CURVE_WITH_KNOTS ( ( 3, 2, 2, 2, 2, 2, 2, 2, 3 ),
 ( 0.6718750000000002220, 0.6738281250000002220, 0.6757812500000002220, 0.6777343750000002220, 0.6796875000000002220, 0.6816406250000002220, 0.6835937500000002220, 0.6855468750000002220, 0.6875000000000002220 ),
 .UNSPECIFIED. ) 
 CURVE ( )  GEOMETRIC_REPRESENTATION_ITEM ( )  RATIONAL_B_SPLINE_CURVE ( ( 0.9999999999999977796, 0.9807852804032326510, 1.000000000000000000, 0.9807852804032304306, 1.000000000000000000, 0.9807852804032304306, 1.000000000000000000, 0.9807852804032304306, 1.000000000000000000, 0.9807852804032304306, 1.000000000000000000, 0.9807852804032304306, 1.000000000000000000, 0.9807852804032304306, 1.000000000000000000, 0.9807852804032282101, 1.000000000000002220 ) ) 
 REPRESENTATION_ITEM ( '' )  );
#2825=CARTESIAN_POINT ( 'NONE',  ( -45.43829269268871229, 443.5573905683720000, -3.332260488124726194 ) ) ;
#2826=DIRECTION ( 'NONE',  ( -1.191790137725560488E-16, 1.000000000000000000, -0.000000000000000000 ) ) ;
#2827=ORIENTED_EDGE ( 'NONE', *, *, #10142, .F. ) ;
#2828=CARTESIAN_POINT ( 'NONE',  ( -40.01497788969913927, 448.8073905601785327, 16.95518130045146776 ) ) ;
#2831=ORIENTED_EDGE ( 'NONE', *, *, #1697, .F. ) ;
#2834=CARTESIAN_POINT ( 'NONE',  ( -14.54375231895776110, 320.9948905601784759, 14.14213562373094568 ) ) ;
#2837=CARTESIAN_POINT ( 'NONE',  ( -40.53162694259543741, 356.6198905683720000, 11.84573899990672885 ) ) ;
#2838=DIRECTION ( 'NONE',  ( 1.191790137725560488E-16, -1.000000000000000000, 0.000000000000000000 ) ) ;
#2839=CARTESIAN_POINT ( 'NONE',  ( -40.01497788969916058, 510.4323905765656946, -16.95518130045146421 ) ) ;
#2840=CARTESIAN_POINT ( 'NONE',  ( -16.84014894278199392, 380.1198905683720568, -11.84573899990672707 ) ) ;
#2842=CARTESIAN_POINT ( 'NONE',  ( -44.16309181155857289, 414.4948905683720000, 6.410867750099241924 ) ) ;
#2843=CARTESIAN_POINT ( 'NONE',  ( -47.16347859291444422, 332.6198905765656377, 7.653668647301805628 ) ) ;
#2844=CARTESIAN_POINT ( 'NONE',  ( -10.20829729246298001, 322.8698905601784759, -7.653668647301794969 ) ) ;
#2845=CARTESIAN_POINT ( 'NONE',  ( -14.48388495494899253, 299.8073905683719431, -9.489475012073734561 ) ) ;
#2846=CARTESIAN_POINT ( 'NONE',  ( -19.19641293061498999, 458.8073905683720000, 14.20200298773971426 ) ) ;
#2848=CARTESIAN_POINT ( 'NONE',  ( -8.685887942688733432, 462.2448905601784759, -2.449293598294705724E-15 ) ) ;
#2852=CARTESIAN_POINT ( 'NONE',  ( -44.16309181155856578, 375.9948905683720568, 6.410867750099241924 ) ) ;
#2853=CARTESIAN_POINT ( 'NONE',  ( -38.17536295476246977, 505.4323905683720568, 14.20200298773971781 ) ) ;
#2854=CARTESIAN_POINT ( 'NONE',  ( -8.685887942688738761, 502.2448905601784190, -2.449293598294705724E-15 ) ) ;
#2855=CARTESIAN_POINT ( 'NONE',  ( -14.48388495494899431, 319.8073905683720568, -9.489475012073736337 ) ) ;
#2857=CARTESIAN_POINT ( 'NONE',  ( -48.68588794268869435, 257.2448905601784759, 0.000000000000000000 ) ) ;
#2861=CARTESIAN_POINT ( 'NONE',  ( -25.35362745456398770, 428.1823905683720568, 16.75240474999998952 ) ) ;
#2862=DIRECTION ( 'NONE',  ( -1.000000000000000000, 0.000000000000000000, 0.000000000000000000 ) ) ;
#2864=CARTESIAN_POINT ( 'NONE',  ( -22.27502019258948707, 446.9948905683720000, 15.47720386886985189 ) ) ;
#2866=CARTESIAN_POINT ( 'NONE',  ( -13.20868407381887089, 458.2448905683720568, 6.410867750099229490 ) ) ;
#2868=CARTESIAN_POINT ( 'NONE',  ( -36.33955658999051508, 415.3698905601784759, -18.47759065022572855 ) ) ;
#2869=CARTESIAN_POINT ( 'NONE',  ( -47.16347859291444422, 382.6198905765655809, 7.653668647301805628 ) ) ;
#2871=CARTESIAN_POINT ( 'NONE',  ( -13.68588794268869790, 223.9102039777116602, 1.836970198721029589E-15 ) ) ;
#2872=CARTESIAN_POINT ( 'NONE',  ( -28.68588794268874054, 573.2448905601785327, 0.000000000000000000 ) ) ;
#2874=CARTESIAN_POINT ( 'NONE',  ( -48.68588794268870856, 337.2448905601784759, 0.000000000000000000 ) ) ;
#2876=DIRECTION ( 'NONE',  ( -1.191790137725560488E-16, 1.000000000000000000, -0.000000000000000000 ) ) ;
#2878=AXIS2_PLACEMENT_3D ( 'NONE', #12735, #19327, #1174 ) ;
#2879=CARTESIAN_POINT ( 'NONE',  ( -19.19641293061498999, 418.8073905683720568, 14.20200298773971426 ) ) ;
#2881=CARTESIAN_POINT ( 'NONE',  ( -25.35362745456396638, 258.1823905683720000, 16.75240474999998952 ) ) ;
#2883=ORIENTED_EDGE ( 'NONE', *, *, #19354, .T. ) ;
#2886=CARTESIAN_POINT ( 'NONE',  ( -11.93348319268873325, 460.0573905683720568, 3.332260488124728859 ) ) ;
#2887=CARTESIAN_POINT ( 'NONE',  ( -14.54375231895775400, 228.2448905765656093, -14.14213562373094746 ) ) ;
#2888=ADVANCED_FACE ( 'NONE', ( #1273 ), #16417, .T. ) ;
#2891=CARTESIAN_POINT ( 'NONE',  ( -42.91697296918459870, 206.7606908932681336, 4.742769269235595608 ) ) ;
#2892=CARTESIAN_POINT ( 'NONE',  ( -44.16309181155859420, 534.7448905683720568, -6.410867750099231266 ) ) ;
#2893=EDGE_CURVE ( 'NONE', #18972, #18441, #14274, .T. ) ;
#2894=AXIS2_PLACEMENT_3D ( 'NONE', #13804, #5570, #20084 ) ;
#2899=CARTESIAN_POINT ( 'NONE',  ( -8.685887942688735208, 456.6823905765655809, 3.978247347593161010 ) ) ;
#2901=DIRECTION ( 'NONE',  ( -1.000000000000000000, 0.000000000000000000, 0.000000000000000000 ) ) ;
#2902=CARTESIAN_POINT ( 'NONE',  ( -42.82802356641964536, 240.7448905765656093, -14.14213562373094746 ) ) ;
#2903=CARTESIAN_POINT ( 'NONE',  ( -28.68588794268870146, 289.7448905601784759, 19.99999999999999289 ) ) ;
#2904=CARTESIAN_POINT ( 'NONE',  ( -38.17536295476244135, 222.3073905683720284, -14.20200298773971426 ) ) ;
#2905=CARTESIAN_POINT ( 'NONE',  ( -42.88789093042842637, 316.3073905683720568, 9.489475012073736337 ) ) ;
#2909=CARTESIAN_POINT ( 'NONE',  ( -21.03221929538691271, 380.3698905601784759, 18.47759065022572500 ) ) ;
#2911=CARTESIAN_POINT ( 'NONE',  ( -45.43829269268869808, 315.0573905683720000, -3.332260488124726194 ) ) ;
#2912=CARTESIAN_POINT ( 'NONE',  ( -35.09675569278795138, 375.7448905683720000, 15.47720386886985366 ) ) ;
#2913=CARTESIAN_POINT ( 'NONE',  ( -14.48388495494901740, 521.3073905683720568, -9.489475012073734561 ) ) ;
#2914=CARTESIAN_POINT ( 'NONE',  ( -11.73070664223724791, 361.3073905601785327, 11.32908994701042005 ) ) ;
#2916=ORIENTED_EDGE ( 'NONE', *, *, #20244, .F. ) ;
#2917=CARTESIAN_POINT ( 'NONE',  ( -19.19641293061499354, 488.8073905683720568, 14.20200298773971426 ) ) ;
#2919=CARTESIAN_POINT ( 'NONE',  ( -45.43829269268870519, 283.8698905683720568, 0.000000000000000000 ) ) ;
#2920=ORIENTED_EDGE ( 'NONE', *, *, #17887, .F. ) ;
#2921=CARTESIAN_POINT ( 'NONE',  ( -32.01814843081344009, 287.5573905683720000, 16.75240474999999307 ) ) ;
#2922=CARTESIAN_POINT ( 'NONE',  ( -13.20868407381885490, 328.2448905683720000, 6.410867750099229490 ) ) ;
#2923=CARTESIAN_POINT ( 'NONE',  ( -11.73070664223723725, 257.9323905765655809, -11.32908994701042715 ) ) ;
#2924=CARTESIAN_POINT ( 'NONE',  ( -40.01497788969915348, 475.6823905601784190, -16.95518130045146421 ) ) ;
#2925=CARTESIAN_POINT ( 'NONE',  ( -13.20868407381884424, 228.2448905683720568, 6.410867750099229490 ) ) ;
#2926=CARTESIAN_POINT ( 'NONE',  ( -25.35362745456398059, 368.1823905683721136, 16.75240474999998952 ) ) ;
#2929=CARTESIAN_POINT ( 'NONE',  ( -8.685887942688708563, 252.2448905601784475, -2.449293598294705724E-15 ) ) ;
#2930=CARTESIAN_POINT ( 'NONE',  ( -22.27502019258948707, 436.9948905683720568, 15.47720386886985189 ) ) ;
#2933=CARTESIAN_POINT ( 'NONE',  ( -32.66413529028188378, 445.0573905601784759, -19.99999999999999289 ) ) ;
#2934=VERTEX_POINT ( 'NONE', #16203 ) ;
#2937=CARTESIAN_POINT ( 'NONE',  ( -28.68588794268871212, 354.4948905765656377, 19.99999999999999289 ) ) ;
#2938=CARTESIAN_POINT ( 'NONE',  ( -45.64106924314017988, 328.1823905601784759, 11.32908994701042715 ) ) ;
#2941=CARTESIAN_POINT ( 'NONE',  ( -19.19641293061498288, 351.9323905683720568, -14.20200298773971603 ) ) ;
#2943=CARTESIAN_POINT ( 'NONE',  ( -28.68588794268873343, 509.4948905765655809, -19.99999999999999289 ) ) ;
#2944=CARTESIAN_POINT ( 'NONE',  ( -28.68588794268871567, 386.3698905683720568, 16.75240474999999307 ) ) ;
#2945=CARTESIAN_POINT ( 'NONE',  ( -42.88789093042841927, 226.3073905683720000, 9.489475012073736337 ) ) ;
#2946=CARTESIAN_POINT ( 'NONE',  ( -22.27502019258949062, 390.7448905683720000, -15.47720386886985544 ) ) ;
#2947=CARTESIAN_POINT ( 'NONE',  ( -21.03221929538691981, 318.8698905765656377, -18.47759065022572855 ) ) ;
#2948=CARTESIAN_POINT ( 'NONE',  ( -42.82802356641966668, 425.9948905601784759, -14.14213562373094746 ) ) ;
#2949=CARTESIAN_POINT ( 'NONE',  ( -13.20868407381885135, 279.4948905683720000, -6.410867750099233042 ) ) ;
#2950=( BOUNDED_CURVE ( )  B_SPLINE_CURVE ( 2, ( #16937, #8379, #7070, #15003, #293, #13591, #15212, #18332, #3522, #6756, #13374, #10210, #10109, #13690, #3834, #18541, #20282 ),
 .UNSPECIFIED., .F., .T. ) 
 B_SPLINE_CURVE_WITH_KNOTS ( ( 3, 2, 2, 2, 2, 2, 2, 2, 3 ),
 ( 0.000000000000000000, 0.001953125000000046838, 0.003906250000000093675, 0.005859375000000140513, 0.007812500000000187350, 0.009765625000000234188, 0.01171875000000028103, 0.01367187500000032786, 0.01562500000000037470 ),
 .UNSPECIFIED. ) 
 CURVE ( )  GEOMETRIC_REPRESENTATION_ITEM ( )  RATIONAL_B_SPLINE_CURVE ( ( 1.000000000000000000, 0.9807852804032304306, 1.000000000000000000, 0.9807852804032304306, 1.000000000000000000, 0.9807852804032304306, 1.000000000000000000, 0.9807852804032304306, 1.000000000000000000, 0.9807852804032304306, 1.000000000000000000, 0.9807852804032304306, 1.000000000000000000, 0.9807852804032304306, 1.000000000000000000, 0.9807852804032267668, 1.000000000000003775 ) ) 
 REPRESENTATION_ITEM ( '' )  );
#2951=CARTESIAN_POINT ( 'NONE',  ( -38.17536295476245556, 436.9323905683720568, 14.20200298773971781 ) ) ;
#2956=ADVANCED_FACE ( 'NONE', ( #7852 ), #6232, .F. ) ;
#2957=CARTESIAN_POINT ( 'NONE',  ( -40.53162694259543741, 354.1198905683720568, -11.84573899990672707 ) ) ;
#2958=CARTESIAN_POINT ( 'NONE',  ( -45.43829269268871940, 503.5573905683720000, -3.332260488124726194 ) ) ;
#2959=CARTESIAN_POINT ( 'NONE',  ( -40.01497788969915348, 505.6823905601784759, -16.95518130045146421 ) ) ;
#2960=CARTESIAN_POINT ( 'NONE',  ( -32.01814843081344009, 316.0573905683720000, 16.75240474999999307 ) ) ;
#2961=ORIENTED_EDGE ( 'NONE', *, *, #7094, .F. ) ;
#2962=CARTESIAN_POINT ( 'NONE',  ( -10.20829729246300488, 522.8698905601785327, -7.653668647301794969 ) ) ;
#2967=CARTESIAN_POINT ( 'NONE',  ( -38.17536295476245556, 416.9323905683720568, 14.20200298773971781 ) ) ;
#2968=FACE_OUTER_BOUND ( 'NONE', #21263, .T. ) ;
#2970=CARTESIAN_POINT ( 'NONE',  ( -40.53162694259544452, 435.1198905683720000, 11.84573899990672885 ) ) ;
#2972=CARTESIAN_POINT ( 'NONE',  ( -32.01814843081345430, 476.0573905683720000, 16.75240474999999307 ) ) ;
#2975=CARTESIAN_POINT ( 'NONE',  ( -8.685887942688724550, 387.3073905765656377, -3.978247347593165895 ) ) ;
#2981=CARTESIAN_POINT ( 'NONE',  ( -14.54375231895775755, 253.4948905601784759, -14.14213562373094746 ) ) ;
#2982=LINE ( 'NONE', #11079, #9368 ) ;
#2983=CARTESIAN_POINT ( 'NONE',  ( -32.01814843081345430, 427.5573905683720000, 16.75240474999999307 ) ) ;
#2985=CARTESIAN_POINT ( 'NONE',  ( -38.17536295476243424, 246.9323905683720284, 14.20200298773971781 ) ) ;
#2987=CARTESIAN_POINT ( 'NONE',  ( -8.685887942688820473, 426.6823905765655809, 3.978247347593374172 ) ) ;
#2989=CARTESIAN_POINT ( 'NONE',  ( -22.27502019258949773, 472.2448905683720568, -15.47720386886985544 ) ) ;
#2990=CARTESIAN_POINT ( 'NONE',  ( -28.68588794268869790, 219.4948905765656377, -19.99999999999999289 ) ) ;
#2991=VERTEX_POINT ( 'NONE', #19435 ) ;
#2992=LINE ( 'NONE', #7941, #3820 ) ;
#2993=CARTESIAN_POINT ( 'NONE',  ( -13.20868407381888154, 530.9948905683720568, -6.410867750099233042 ) ) ;
#2994=ORIENTED_EDGE ( 'NONE', *, *, #19444, .T. ) ;
#2995=CARTESIAN_POINT ( 'NONE',  ( -42.88789093042845479, 522.9323905683720568, -9.489475012073734561 ) ) ;
#2998=CARTESIAN_POINT ( 'NONE',  ( -32.66413529028188378, 444.1823905765655809, 19.99999999999999289 ) ) ;
#2999=CARTESIAN_POINT ( 'NONE',  ( -48.68588794268870856, 347.2448905601784759, 0.000000000000000000 ) ) ;
#3000=DIRECTION ( 'NONE',  ( -1.191790137725560488E-16, 1.000000000000000000, -0.000000000000000000 ) ) ;
#3005=CARTESIAN_POINT ( 'NONE',  ( -45.43829269268869098, 234.1823905683720284, 3.332260488124734632 ) ) ;
#3006=CARTESIAN_POINT ( 'NONE',  ( -22.27502019258946930, 308.4948905683720568, 15.47720386886985189 ) ) ;
#3007=CARTESIAN_POINT ( 'NONE',  ( -36.33955658999051508, 445.3698905601785327, -18.47759065022572855 ) ) ;
#3008=CARTESIAN_POINT ( 'NONE',  ( -28.68588794268871567, 379.7448905601785327, 19.99999999999999289 ) ) ;
#3010=CARTESIAN_POINT ( 'NONE',  ( -14.48388495494899075, 299.4323905683720568, 9.489475012073732785 ) ) ;
#3011=CARTESIAN_POINT ( 'NONE',  ( -42.88789093042843348, 354.8073905683720568, 9.489475012073736337 ) ) ;
#3012=CARTESIAN_POINT ( 'NONE',  ( -28.68588794268873698, 522.8698905683719431, -16.75240474999999307 ) ) ;
#3013=CARTESIAN_POINT ( 'NONE',  ( -8.685887942688722774, 371.9323905601784759, 3.978247347593161010 ) ) ;
#3017=CARTESIAN_POINT ( 'NONE',  ( -25.35362745456399480, 488.1823905683720568, 16.75240474999998952 ) ) ;
#3019=CARTESIAN_POINT ( 'NONE',  ( -44.16309181155856578, 283.2448905683720568, -6.410867750099231266 ) ) ;
#3022=CARTESIAN_POINT ( 'NONE',  ( -14.48388495494898898, 289.4323905683720000, 9.489475012073731008 ) ) ;
#3023=CARTESIAN_POINT ( 'NONE',  ( -40.53162694259543031, 315.1198905683720568, 11.84573899990672885 ) ) ;
#3024=CARTESIAN_POINT ( 'NONE',  ( -44.16309181155855157, 265.9948905683720000, 6.410867750099241924 ) ) ;
#3026=CARTESIAN_POINT ( 'NONE',  ( -10.20829729246297646, 267.6198905765655809, -7.653668647301794969 ) ) ;
#3027=CARTESIAN_POINT ( 'NONE',  ( -28.68588794268874054, 573.2448905601785327, 0.000000000000000000 ) ) ;
#3028=CARTESIAN_POINT ( 'NONE',  ( -44.16309181155855867, 233.2448905683720000, -6.410867750099231266 ) ) ;
#3029=CARTESIAN_POINT ( 'NONE',  ( -32.01814843081344719, 377.5573905683720568, 16.75240474999999307 ) ) ;
#3033=CARTESIAN_POINT ( 'NONE',  ( -45.64106924314017277, 271.0573905765656946, -11.32908994701042538 ) ) ;
#3034=CARTESIAN_POINT ( 'NONE',  ( -32.01814843081345430, 416.0573905683720568, 16.75240474999999307 ) ) ;
#3037=CARTESIAN_POINT ( 'NONE',  ( -21.03221929538691626, 430.3698905601784759, 18.47759065022572500 ) ) ;
#3039=ORIENTED_EDGE ( 'NONE', *, *, #17623, .F. ) ;
#3040=VERTEX_POINT ( 'NONE', #3322 ) ;
#3042=CARTESIAN_POINT ( 'NONE',  ( -10.20829729246298001, 312.8698905601784759, -7.653668647301794969 ) ) ;
#3044=CARTESIAN_POINT ( 'NONE',  ( -40.53162694259543741, 346.6198905683720000, 11.84573899990672885 ) ) ;
#3045=CARTESIAN_POINT ( 'NONE',  ( -11.73070664223726389, 496.0573905765656377, 11.32908994701042005 ) ) ;
#3046=CARTESIAN_POINT ( 'NONE',  ( -32.01814843081344719, 376.0573905683720000, 16.75240474999999307 ) ) ;
#3047=CARTESIAN_POINT ( 'NONE',  ( -22.27502019258945865, 228.4948905683720284, 15.47720386886985189 ) ) ;
#3048=CARTESIAN_POINT ( 'NONE',  ( -40.53162694259543741, 385.1198905683720568, 11.84573899990672885 ) ) ;
#3049=CARTESIAN_POINT ( 'NONE',  ( -17.35679799567828852, 315.4323905765656377, 16.95518130045146421 ) ) ;
#3050=FACE_OUTER_BOUND ( 'NONE', #2380, .T. ) ;
#3051=CARTESIAN_POINT ( 'NONE',  ( -45.43829269268870519, 283.8698905683720568, 0.000000000000000000 ) ) ;
#3053=CARTESIAN_POINT ( 'NONE',  ( -25.35362745456399125, 438.1823905683720000, 16.75240474999998952 ) ) ;
#3054=CARTESIAN_POINT ( 'NONE',  ( -45.64106924314017277, 286.3073905601785327, -11.32908994701042538 ) ) ;
#3056=CARTESIAN_POINT ( 'NONE',  ( -8.685887942688742314, 573.2448905601785327, 2.449293598294706119E-15 ) ) ;
#3057=CARTESIAN_POINT ( 'NONE',  ( -22.27502019258948707, 352.2448905683720000, -15.47720386886985544 ) ) ;
#3058=CARTESIAN_POINT ( 'NONE',  ( -16.84014894278200813, 500.1198905683720000, -11.84573899990672707 ) ) ;
#3059=CARTESIAN_POINT ( 'NONE',  ( -42.82802356641967378, 485.9948905601784759, -14.14213562373094746 ) ) ;
#3060=CARTESIAN_POINT ( 'NONE',  ( -14.48388495494899431, 327.9323905683720568, 9.489475012073732785 ) ) ;
#3067=CARTESIAN_POINT ( 'NONE',  ( -11.93348319268872615, 410.6823905683720000, -3.332260488124732856 ) ) ;
#3068=CARTESIAN_POINT ( 'NONE',  ( -28.68588794268869790, 234.4948905765656377, 19.99999999999999289 ) ) ;
#3069=CARTESIAN_POINT ( 'NONE',  ( -48.68588794268873698, 573.2448905601785327, 0.000000000000000000 ) ) ;
#3070=CARTESIAN_POINT ( 'NONE',  ( -11.93348319268873148, 448.5573905683720000, 3.332260488124728415 ) ) ;
#3071=CARTESIAN_POINT ( 'NONE',  ( -13.20868407381887089, 449.4948905683720568, -6.410867750099233042 ) ) ;
#3073=CARTESIAN_POINT ( 'NONE',  ( -17.35679799567830273, 413.8073905601785327, -16.95518130045146421 ) ) ;
#3074=CARTESIAN_POINT ( 'NONE',  ( -24.70764059509555466, 384.8073905765655809, 19.99999999999998934 ) ) ;
#3075=DIRECTION ( 'NONE',  ( -1.000000000000000000, 0.000000000000000000, 0.000000000000000000 ) ) ;
#3076=CARTESIAN_POINT ( 'NONE',  ( -48.68588794268855224, 391.6823905765656377, -3.978247347593583783 ) ) ;
#3079=CARTESIAN_POINT ( 'NONE',  ( -32.01814843081346140, 497.5573905683720568, 16.75240474999999307 ) ) ;
#3082=CARTESIAN_POINT ( 'NONE',  ( -45.21523660720509952, 223.9102039777117454, 6.319766016702155653 ) ) ;
#3085=CARTESIAN_POINT ( 'NONE',  ( -38.17536295476245556, 406.9323905683719431, 14.20200298773971781 ) ) ;
#3086=DIRECTION ( 'NONE',  ( -1.000000000000000000, 0.000000000000000000, 0.000000000000000000 ) ) ;
#3087=CARTESIAN_POINT ( 'NONE',  ( -35.09675569278793006, 223.4948905683720284, -15.47720386886985544 ) ) ;
#3091=EDGE_LOOP ( 'NONE', ( #12081, #398, #11971, #422 ) ) ;
#3093=CARTESIAN_POINT ( 'NONE',  ( -35.09675569278795848, 463.4948905683720000, -15.47720386886985544 ) ) ;
#3094=CARTESIAN_POINT ( 'NONE',  ( -10.20829729246297113, 227.6198905765656093, -7.653668647301794969 ) ) ;
#3096=CARTESIAN_POINT ( 'NONE',  ( -43.68588794268870856, 210.1437886375728965, 0.3278592396120688091 ) ) ;
#3097=CARTESIAN_POINT ( 'NONE',  ( -19.19641293061500420, 531.9323905683720568, -14.20200298773971603 ) ) ;
#3099=CARTESIAN_POINT ( 'NONE',  ( -40.53162694259545873, 515.1198905683720568, 11.84573899990672885 ) ) ;
#3103=CARTESIAN_POINT ( 'NONE',  ( -47.16347859291445133, 441.3698905765656377, -7.653668647301793193 ) ) ;
#3105=CARTESIAN_POINT ( 'NONE',  ( -11.93348319268871904, 338.8698905683720000, -2.051577885510841163E-15 ) ) ;
#3106=CARTESIAN_POINT ( 'NONE',  ( -14.54375231895777887, 455.7448905765656377, 14.14213562373094568 ) ) ;
#3112=CARTESIAN_POINT ( 'NONE',  ( -44.16309181155855867, 325.9948905683720000, 6.410867750099241924 ) ) ;
#3115=CARTESIAN_POINT ( 'NONE',  ( -17.35679799567828141, 270.6823905601785327, 16.95518130045146421 ) ) ;
#3117=CARTESIAN_POINT ( 'NONE',  ( -40.53162694259543031, 306.6198905683720000, 11.84573899990672885 ) ) ;
#3118=CARTESIAN_POINT ( 'NONE',  ( -40.53162694259545873, 514.1198905683720568, -11.84573899990672707 ) ) ;
#3119=CARTESIAN_POINT ( 'NONE',  ( -28.68588794268871212, 369.7448905601785327, 19.99999999999999289 ) ) ;
#3120=CARTESIAN_POINT ( 'NONE',  ( -36.33955658999050087, 315.3698905601784759, -18.47759065022572855 ) ) ;
#3122=CARTESIAN_POINT ( 'NONE',  ( -42.88789093042844769, 486.3073905683721136, 9.489475012073736337 ) ) ;
#3124=CARTESIAN_POINT ( 'NONE',  ( -13.20868407381884779, 278.2448905683720568, 6.410867750099229490 ) ) ;
#3126=CARTESIAN_POINT ( 'NONE',  ( -16.84014894278198327, 291.6198905683720000, -11.84573899990672707 ) ) ;
#3127=CARTESIAN_POINT ( 'NONE',  ( -13.20868407381885490, 319.4948905683720000, -6.410867750099233042 ) ) ;
#3128=CARTESIAN_POINT ( 'NONE',  ( -8.685887942688710339, 256.9948905765655809, -2.449293598294705724E-15 ) ) ;
#3131=CARTESIAN_POINT ( 'NONE',  ( -40.53162694259542320, 235.1198905683720000, 11.84573899990672885 ) ) ;
#3132=CARTESIAN_POINT ( 'NONE',  ( -16.84014894278198682, 369.1198905683720000, 11.84573899990672530 ) ) ;
#3135=AXIS2_PLACEMENT_3D ( 'NONE', #14923, #15926, #7687 ) ;
#3139=CARTESIAN_POINT ( 'NONE',  ( -32.01814843081345430, 431.6823905683720000, -16.75240474999999307 ) ) ;
#3142=CARTESIAN_POINT ( 'NONE',  ( -47.16347859291445133, 427.8698905601784759, 7.653668647301805628 ) ) ;
#3145=ORIENTED_EDGE ( 'NONE', *, *, #6536, .T. ) ;
#3147=CARTESIAN_POINT ( 'NONE',  ( -48.68588794268870856, 351.9948905765656377, 0.000000000000000000 ) ) ;
#3148=CARTESIAN_POINT ( 'NONE',  ( -14.54375231895776288, 303.4948905601784759, -14.14213562373094746 ) ) ;
#3151=CARTESIAN_POINT ( 'NONE',  ( -35.09675569278795138, 337.2448905683720568, 15.47720386886985366 ) ) ;
#3154=CARTESIAN_POINT ( 'NONE',  ( -28.68588794268872988, 504.4948905765655809, 19.99999999999999289 ) ) ;
#3155=CARTESIAN_POINT ( 'NONE',  ( -38.17536295476244845, 385.4323905683720000, 14.20200298773971781 ) ) ;
#3156=CARTESIAN_POINT ( 'NONE',  ( -35.09675569278793716, 227.2448905683720568, 15.47720386886985366 ) ) ;
#3157=CARTESIAN_POINT ( 'NONE',  ( -14.48388495494900674, 389.8073905683721136, -9.489475012073734561 ) ) ;
#3159=CARTESIAN_POINT ( 'NONE',  ( -40.01497788969913927, 330.4323905765655809, -16.95518130045146421 ) ) ;
#3160=CARTESIAN_POINT ( 'NONE',  ( -45.64106924314018698, 426.3073905601784190, -11.32908994701042538 ) ) ;
#3161=CARTESIAN_POINT ( 'NONE',  ( -25.35362745456398414, 291.0573905683720568, -16.75240474999999307 ) ) ;
#3163=CARTESIAN_POINT ( 'NONE',  ( -22.27502019258948707, 438.4948905683720568, 15.47720386886985189 ) ) ;
#3165=CARTESIAN_POINT ( 'NONE',  ( -48.68588794268870856, 357.2448905601784759, 0.000000000000000000 ) ) ;
#3169=CARTESIAN_POINT ( 'NONE',  ( -11.93348319268872260, 340.6823905683720000, -3.332260488124732856 ) ) ;
#3170=CARTESIAN_POINT ( 'NONE',  ( -40.53162694259545162, 492.6198905683720000, -11.84573899990672707 ) ) ;
#3172=CARTESIAN_POINT ( 'NONE',  ( -28.68588794268872633, 479.7448905601784759, 19.99999999999999289 ) ) ;
#3173=CARTESIAN_POINT ( 'NONE',  ( -13.20868407381885312, 299.4948905683720568, -6.410867750099233042 ) ) ;
#3178=CARTESIAN_POINT ( 'NONE',  ( -14.48388495494900674, 411.3073905683720000, -9.489475012073734561 ) ) ;
#3179=DIRECTION ( 'NONE',  ( 0.000000000000000000, 0.000000000000000000, 1.000000000000000000 ) ) ;
#3181=CARTESIAN_POINT ( 'NONE',  ( -28.68588794268872633, 451.3698905683720000, -16.75240474999999307 ) ) ;
#3182=CARTESIAN_POINT ( 'NONE',  ( -42.88789093042844058, 442.9323905683720568, -9.489475012073734561 ) ) ;
#3184=CARTESIAN_POINT ( 'NONE',  ( -17.35679799567830273, 378.5573905765656946, -16.95518130045146421 ) ) ;
#3185=CARTESIAN_POINT ( 'NONE',  ( -48.68588794268870856, 361.9948905765655809, 0.000000000000000000 ) ) ;
#3186=DIRECTION ( 'NONE',  ( -1.000000000000000000, 0.000000000000000000, 0.000000000000000000 ) ) ;
#3188=CARTESIAN_POINT ( 'NONE',  ( -32.66413529028185536, 254.1823905765656377, 19.99999999999999289 ) ) ;
#3190=CARTESIAN_POINT ( 'NONE',  ( -45.43829269268872650, 495.3698905683720568, 0.000000000000000000 ) ) ;
#3195=CARTESIAN_POINT ( 'NONE',  ( -44.16309181155857289, 415.9948905683720000, 6.410867750099241924 ) ) ;
#3196=CARTESIAN_POINT ( 'NONE',  ( -36.33955658999052218, 470.1198905765656377, -18.47759065022572855 ) ) ;
#3197=CARTESIAN_POINT ( 'NONE',  ( -32.01814843081343298, 233.1823905683720284, -16.75240474999999307 ) ) ;
#3201=CARTESIAN_POINT ( 'NONE',  ( -38.17536295476246977, 453.8073905683720568, -14.20200298773971426 ) ) ;
#3203=CARTESIAN_POINT ( 'NONE',  ( -8.685887942688706786, 227.3073905765656093, -3.978247347593165895 ) ) ;
#3206=CARTESIAN_POINT ( 'NONE',  ( -38.17536295476246977, 526.9323905683719431, 14.20200298773971781 ) ) ;
#3207=ORIENTED_EDGE ( 'NONE', *, *, #20195, .F. ) ;
#3208=CARTESIAN_POINT ( 'NONE',  ( -14.48388495494901385, 507.9323905683720000, 9.489475012073731008 ) ) ;
#3211=CARTESIAN_POINT ( 'NONE',  ( -48.68588794268872277, 451.9948905765656377, 0.000000000000000000 ) ) ;
#3212=CARTESIAN_POINT ( 'NONE',  ( -24.70764059509555111, 299.1823905765656377, -19.99999999999999289 ) ) ;
#3214=CARTESIAN_POINT ( 'NONE',  ( -48.68588794268869435, 247.2448905601785043, 0.000000000000000000 ) ) ;
#3215=LINE ( 'NONE', #6231, #461 ) ;
#3220=CARTESIAN_POINT ( 'NONE',  ( -11.93348319268871727, 320.6823905683720000, -3.332260488124732856 ) ) ;
#3222=CARTESIAN_POINT ( 'NONE',  ( -14.54375231895775933, 273.4948905601785327, -14.14213562373094746 ) ) ;
#3224=CARTESIAN_POINT ( 'NONE',  ( -44.16309181155855867, 295.9948905683720000, 6.410867750099241924 ) ) ;
#3227=CARTESIAN_POINT ( 'NONE',  ( -11.93348319268874214, 530.0573905683720568, 3.332260488124728859 ) ) ;
#3229=CARTESIAN_POINT ( 'NONE',  ( -47.16347859291444422, 357.8698905601784759, 7.653668647301805628 ) ) ;
#3230=CARTESIAN_POINT ( 'NONE',  ( -11.73070664223723369, 227.9323905765656377, -11.32908994701042538 ) ) ;
#3232=CARTESIAN_POINT ( 'NONE',  ( -45.43829269268871940, 485.6823905683721136, 3.332260488124734632 ) ) ;
#3233=CARTESIAN_POINT ( 'NONE',  ( -25.35362745456398059, 281.0573905683720568, -16.75240474999999307 ) ) ;
#3234=ORIENTED_EDGE ( 'NONE', *, *, #8416, .F. ) ;
#3236=CARTESIAN_POINT ( 'NONE',  ( -28.68588794268870146, 277.8698905683720000, 16.75240474999999307 ) ) ;
#3237=CARTESIAN_POINT ( 'NONE',  ( -45.43829269268869808, 255.6823905683720000, 3.332260488124734632 ) ) ;
#3239=CARTESIAN_POINT ( 'NONE',  ( -8.685887942688708563, 246.9948905765656093, -2.449293598294705724E-15 ) ) ;
#3241=CARTESIAN_POINT ( 'NONE',  ( -44.16309181155855157, 234.4948905683720284, 6.410867750099241924 ) ) ;
#3243=CARTESIAN_POINT ( 'NONE',  ( -45.43829269268870519, 375.0573905683720000, -3.332260488124726194 ) ) ;
#3244=CARTESIAN_POINT ( 'NONE',  ( -14.54375231895775578, 280.9948905601785327, 14.14213562373094568 ) ) ;
#3245=CARTESIAN_POINT ( 'NONE',  ( -45.64106924314019409, 461.0573905765656377, -11.32908994701042538 ) ) ;
#3247=CARTESIAN_POINT ( 'NONE',  ( -14.48388495494900496, 427.9323905683720568, 9.489475012073732785 ) ) ;
#3250=CARTESIAN_POINT ( 'NONE',  ( -14.54375231895777887, 433.4948905601784759, -14.14213562373094746 ) ) ;
#3253=ORIENTED_EDGE ( 'NONE', *, *, #18866, .T. ) ;
#3256=CARTESIAN_POINT ( 'NONE',  ( -10.20829729246297823, 311.6198905601784759, 7.653668647301790529 ) ) ;
#3259=CARTESIAN_POINT ( 'NONE',  ( -45.43829269268871229, 345.6823905683720000, 3.332260488124734632 ) ) ;
#3260=CARTESIAN_POINT ( 'NONE',  ( -24.70764059509556532, 474.8073905765655809, 19.99999999999998934 ) ) ;
#3261=CARTESIAN_POINT ( 'NONE',  ( -13.20868407381885845, 358.2448905683720000, 6.410867750099229490 ) ) ;
#3262=CARTESIAN_POINT ( 'NONE',  ( -14.48388495494898187, 229.4323905683720000, 9.489475012073732785 ) ) ;
#3263=CARTESIAN_POINT ( 'NONE',  ( -45.43829269268871940, 393.8698905683720000, 0.000000000000000000 ) ) ;
#3264=( BOUNDED_CURVE ( )  B_SPLINE_CURVE ( 2, ( #17062, #5580, #20405, #627, #4170, #13928, #5685, #13708, #7516, #15341, #15761, #5900, #7192, #7086, #2558, #3852, #14140 ),
 .UNSPECIFIED., .F., .T. ) 
 B_SPLINE_CURVE_WITH_KNOTS ( ( 3, 2, 2, 2, 2, 2, 2, 2, 3 ),
 ( 0.4062500000000001665, 0.4082031250000001665, 0.4101562500000001665, 0.4121093750000001665, 0.4140625000000001665, 0.4160156250000001665, 0.4179687500000001665, 0.4199218750000001665, 0.4218750000000001665 ),
 .UNSPECIFIED. ) 
 CURVE ( )  GEOMETRIC_REPRESENTATION_ITEM ( )  RATIONAL_B_SPLINE_CURVE ( ( 0.9999999999999983347, 0.9807852804032320959, 1.000000000000000000, 0.9807852804032304306, 1.000000000000000000, 0.9807852804032304306, 1.000000000000000000, 0.9807852804032304306, 1.000000000000000000, 0.9807852804032304306, 1.000000000000000000, 0.9807852804032304306, 1.000000000000000000, 0.9807852804032304306, 1.000000000000000000, 0.9807852804032287652, 1.000000000000001554 ) ) 
 REPRESENTATION_ITEM ( '' )  );
#3265=CARTESIAN_POINT ( 'NONE',  ( -32.66413529028186957, 314.1823905765655809, 19.99999999999999289 ) ) ;
#3267=CARTESIAN_POINT ( 'NONE',  ( -38.17536295476244845, 292.3073905683720000, -14.20200298773971426 ) ) ;
#3269=CARTESIAN_POINT ( 'NONE',  ( -11.93348319268872970, 430.0573905683721136, 3.332260488124728415 ) ) ;
#3273=CARTESIAN_POINT ( 'NONE',  ( -45.43829269268873361, 533.8698905683720568, 0.000000000000000000 ) ) ;
#3275=CARTESIAN_POINT ( 'NONE',  ( -22.27502019258947286, 338.4948905683720568, 15.47720386886985189 ) ) ;
#3276=CARTESIAN_POINT ( 'NONE',  ( -32.01814843081346140, 481.6823905683720568, -16.75240474999999307 ) ) ;
#3279=CARTESIAN_POINT ( 'NONE',  ( -24.70764059509557953, 494.4323905601783622, -19.99999999999999289 ) ) ;
#3280=CARTESIAN_POINT ( 'NONE',  ( -45.43829269268870519, 303.8698905683720000, 0.000000000000000000 ) ) ;
#3282=EDGE_LOOP ( 'NONE', ( #21260, #654, #1914, #18858 ) ) ;
#3286=CARTESIAN_POINT ( 'NONE',  ( -13.20868407381886378, 399.7448905683720568, 6.410867750099229490 ) ) ;
#3288=FACE_OUTER_BOUND ( 'NONE', #18886, .T. ) ;
#3289=CARTESIAN_POINT ( 'NONE',  ( -25.35362745456399836, 431.0573905683720000, -16.75240474999999307 ) ) ;
#3290=CARTESIAN_POINT ( 'NONE',  ( -25.35362745456399125, 446.6823905683720568, 16.75240474999998952 ) ) ;
#3293=ADVANCED_FACE ( 'NONE', ( #5003 ), #44, .T. ) ;
#3294=CARTESIAN_POINT ( 'NONE',  ( -8.685887942688724550, 386.6823905765655809, 3.978247347593161010 ) ) ;
#3295=FACE_OUTER_BOUND ( 'NONE', #10572, .T. ) ;
#3299=CARTESIAN_POINT ( 'NONE',  ( -25.35362745456400901, 492.5573905683721136, -16.75240474999999307 ) ) ;
#3300=CARTESIAN_POINT ( 'NONE',  ( -8.685887942688717445, 312.2448905601784759, -2.449293598294705724E-15 ) ) ;
#3301=CARTESIAN_POINT ( 'NONE',  ( -8.685887942688733432, 462.2448905601784759, -2.449293598294705724E-15 ) ) ;
#3303=CARTESIAN_POINT ( 'NONE',  ( -16.84014894278199392, 401.6198905683720568, -11.84573899990672707 ) ) ;
#3305=CARTESIAN_POINT ( 'NONE',  ( -45.43829269268869098, 225.0573905683720568, -3.332260488124726194 ) ) ;
#3306=ORIENTED_EDGE ( 'NONE', *, *, #9439, .F. ) ;
#3307=DIRECTION ( 'NONE',  ( -1.000000000000000000, 0.000000000000000000, 0.000000000000000000 ) ) ;
#3309=CARTESIAN_POINT ( 'NONE',  ( -44.16309181155857289, 435.9948905683720568, 6.410867750099241924 ) ) ;
#3310=CARTESIAN_POINT ( 'NONE',  ( -40.53162694259545873, 525.1198905683720568, 11.84573899990672885 ) ) ;
#3313=CARTESIAN_POINT ( 'NONE',  ( -28.68588794268869435, 226.3698905683720284, 16.75240474999999307 ) ) ;
#3315=CARTESIAN_POINT ( 'NONE',  ( -11.93348319268873858, 508.5573905683720000, 3.332260488124728859 ) ) ;
#3317=CARTESIAN_POINT ( 'NONE',  ( -14.54375231895777532, 435.7448905765656377, 14.14213562373094568 ) ) ;
#3318=CARTESIAN_POINT ( 'NONE',  ( -11.73070664223724968, 357.9323905765656377, -11.32908994701042538 ) ) ;
#3319=CARTESIAN_POINT ( 'NONE',  ( -8.685887942688895080, 331.9323905601783622, 3.978247347593586447 ) ) ;
#3322=CARTESIAN_POINT ( 'NONE',  ( -8.685887942688708563, 246.9948905765656093, -2.449293598294705724E-15 ) ) ;
#3324=CARTESIAN_POINT ( 'NONE',  ( -14.48388495494898898, 289.4323905683720000, 9.489475012073732785 ) ) ;
#3326=CARTESIAN_POINT ( 'NONE',  ( -47.16347859291443712, 276.6198905601784759, -7.653668647301793193 ) ) ;
#3327=CARTESIAN_POINT ( 'NONE',  ( -18.66797547166049753, 223.9102039777116602, -17.31025331282116397 ) ) ;
#3328=CARTESIAN_POINT ( 'NONE',  ( -35.09675569278794427, 297.2448905683720000, 15.47720386886985366 ) ) ;
#3330=CARTESIAN_POINT ( 'NONE',  ( -40.53162694259545162, 504.1198905683720568, -11.84573899990672707 ) ) ;
#3331=CARTESIAN_POINT ( 'NONE',  ( -42.82802356641965957, 368.4948905601784759, 14.14213562373094923 ) ) ;
#3333=CARTESIAN_POINT ( 'NONE',  ( -32.66413529028186247, 315.0573905601784190, -19.99999999999999289 ) ) ;
#3335=CARTESIAN_POINT ( 'NONE',  ( -13.20868407381887444, 470.9948905683720000, -6.410867750099233042 ) ) ;
#3337=CARTESIAN_POINT ( 'NONE',  ( -45.43829269268869808, 284.1823905683720568, 3.332260488124734632 ) ) ;
#3340=CARTESIAN_POINT ( 'NONE',  ( -40.53162694259543031, 286.6198905683720000, 11.84573899990672885 ) ) ;
#3342=CARTESIAN_POINT ( 'NONE',  ( -40.53162694259542320, 264.1198905683720568, -11.84573899990672707 ) ) ;
#3343=CARTESIAN_POINT ( 'NONE',  ( -40.01497788969911795, 243.5573905765656377, 16.95518130045146776 ) ) ;
#3344=CARTESIAN_POINT ( 'NONE',  ( -42.82802356641965247, 308.4948905601784759, 14.14213562373094923 ) ) ;
#3345=CARTESIAN_POINT ( 'NONE',  ( -40.01497788969911795, 228.8073905601784759, 16.95518130045146776 ) ) ;
#3346=CARTESIAN_POINT ( 'NONE',  ( -8.685887942688710339, 256.9948905765655809, -2.449293598294705724E-15 ) ) ;
#3347=CARTESIAN_POINT ( 'NONE',  ( -44.16309181155855867, 263.2448905683720000, -6.410867750099231266 ) ) ;
#3348=CARTESIAN_POINT ( 'NONE',  ( -19.19641293061498644, 371.9323905683720568, -14.20200298773971603 ) ) ;
#3350=CARTESIAN_POINT ( 'NONE',  ( -48.68588794268872277, 461.9948905765656377, 0.000000000000000000 ) ) ;
#3355=CARTESIAN_POINT ( 'NONE',  ( -11.93348319268872793, 419.1823905683720000, -3.332260488124732856 ) ) ;
#3356=CARTESIAN_POINT ( 'NONE',  ( -48.68588794268854514, 341.6823905765656946, -3.978247347593583783 ) ) ;
#3358=CARTESIAN_POINT ( 'NONE',  ( -42.82802356641966668, 428.4948905601784759, 14.14213562373094923 ) ) ;
#3363=CARTESIAN_POINT ( 'NONE',  ( -45.64106924314017988, 296.3073905601784190, -11.32908994701042715 ) ) ;
#3365=CARTESIAN_POINT ( 'NONE',  ( -42.88789093042843348, 346.3073905683720568, 9.489475012073734561 ) ) ;
#3367=VERTEX_POINT ( 'NONE', #3908 ) ;
#3368=CARTESIAN_POINT ( 'NONE',  ( -32.66413529028189089, 484.1823905765656946, 19.99999999999999289 ) ) ;
#3369=CARTESIAN_POINT ( 'NONE',  ( -40.53162694259543741, 365.1198905683720000, 11.84573899990672885 ) ) ;
#3371=CARTESIAN_POINT ( 'NONE',  ( -32.01814843081344719, 381.6823905683719431, -16.75240474999999307 ) ) ;
#3373=CARTESIAN_POINT ( 'NONE',  ( -45.64106924314017988, 312.9323905765655809, 11.32908994701042715 ) ) ;
#3374=CARTESIAN_POINT ( 'NONE',  ( -40.01497788969914637, 425.6823905601784759, -16.95518130045146421 ) ) ;
#3375=CARTESIAN_POINT ( 'NONE',  ( -44.16309181155856578, 293.2448905683720000, -6.410867750099231266 ) ) ;
#3377=CARTESIAN_POINT ( 'NONE',  ( -35.09675569278795138, 433.4948905683720568, -15.47720386886985544 ) ) ;
#3378=CARTESIAN_POINT ( 'NONE',  ( -48.68588794268870146, 287.2448905601784759, 0.000000000000000000 ) ) ;
#3379=CARTESIAN_POINT ( 'NONE',  ( -8.685887942688399477, 512.5573905601783053, -3.978247347592341221 ) ) ;
#3380=DIRECTION ( 'NONE',  ( -1.000000000000000000, 0.000000000000000000, 0.000000000000000000 ) ) ;
#3383=CARTESIAN_POINT ( 'NONE',  ( -28.68588794268871212, 342.8698905683720000, -16.75240474999999307 ) ) ;
#3384=CARTESIAN_POINT ( 'NONE',  ( -16.84014894278200458, 490.1198905683720000, -11.84573899990672707 ) ) ;
#3386=CARTESIAN_POINT ( 'NONE',  ( -10.20829729246300133, 492.8698905601784759, -7.653668647301794969 ) ) ;
#3387=CARTESIAN_POINT ( 'NONE',  ( -38.17536295476244845, 312.3073905683720000, -14.20200298773971426 ) ) ;
#3393=CARTESIAN_POINT ( 'NONE',  ( -13.20868407381886556, 400.9948905683720568, -6.410867750099233042 ) ) ;
#3394=CARTESIAN_POINT ( 'NONE',  ( -28.68588794268872277, 444.4948905765655809, 19.99999999999999289 ) ) ;
#3395=CARTESIAN_POINT ( 'NONE',  ( -35.09675569278795138, 421.9948905683720000, -15.47720386886985544 ) ) ;
#3396=CARTESIAN_POINT ( 'NONE',  ( -45.43829269268872650, 453.8698905683720000, 0.000000000000000000 ) ) ;
#3398=CARTESIAN_POINT ( 'NONE',  ( -47.16347859291444422, 361.3698905765655809, -7.653668647301793193 ) ) ;
#3401=CARTESIAN_POINT ( 'NONE',  ( -8.685887942688729879, 426.9948905765656377, -2.449293598294705724E-15 ) ) ;
#3402=CARTESIAN_POINT ( 'NONE',  ( -24.70764059509557597, 489.1823905765656377, -19.99999999999999289 ) ) ;
#3403=CARTESIAN_POINT ( 'NONE',  ( -42.88789093042844769, 504.4323905683721136, -9.489475012073736337 ) ) ;
#3406=CARTESIAN_POINT ( 'NONE',  ( -36.33955658999052218, 419.1198905601784759, 18.47759065022572500 ) ) ;
#3407=CARTESIAN_POINT ( 'NONE',  ( -35.09675569278795848, 417.2448905683720568, 15.47720386886985366 ) ) ;
#3408=EDGE_CURVE ( 'NONE', #19361, #13635, #2087, .T. ) ;
#3409=CARTESIAN_POINT ( 'NONE',  ( -16.84014894278196905, 229.1198905683720000, 11.84573899990672530 ) ) ;
#3410=CARTESIAN_POINT ( 'NONE',  ( -13.20868407381886023, 359.4948905683720000, -6.410867750099233042 ) ) ;
#3414=CARTESIAN_POINT ( 'NONE',  ( -14.48388495494901740, 519.8073905683720568, -9.489475012073736337 ) ) ;
#3416=CARTESIAN_POINT ( 'NONE',  ( -19.19641293061499354, 441.9323905683720568, -14.20200298773971603 ) ) ;
#3417=CARTESIAN_POINT ( 'NONE',  ( -22.27502019258949417, 516.9948905683720568, 15.47720386886985189 ) ) ;
#3419=FACE_OUTER_BOUND ( 'NONE', #13096, .T. ) ;
#3420=CARTESIAN_POINT ( 'NONE',  ( -11.93348319268873681, 488.5573905683720568, 3.332260488124728415 ) ) ;
#3422=CARTESIAN_POINT ( 'NONE',  ( -14.48388495494901562, 509.8073905683720000, -9.489475012073734561 ) ) ;
#3424=CARTESIAN_POINT ( 'NONE',  ( -24.70764059509555821, 414.8073905765656946, 19.99999999999998934 ) ) ;
#3425=CARTESIAN_POINT ( 'NONE',  ( -48.68588794268870146, 301.9948905765655809, 0.000000000000000000 ) ) ;
#3426=CARTESIAN_POINT ( 'NONE',  ( -17.35679799567828496, 330.6823905601785896, 16.95518130045146421 ) ) ;
#3427=DIRECTION ( 'NONE',  ( -1.191790137725560488E-16, 1.000000000000000000, -0.000000000000000000 ) ) ;
#3432=CARTESIAN_POINT ( 'NONE',  ( -32.01814843081344009, 297.5573905683720000, 16.75240474999999307 ) ) ;
#3433=DIRECTION ( 'NONE',  ( -1.191790137725560488E-16, 1.000000000000000000, -0.000000000000000000 ) ) ;
#3434=CARTESIAN_POINT ( 'NONE',  ( -48.68588794268869435, 267.5573905601784759, 3.978247347593168115 ) ) ;
#3435=CARTESIAN_POINT ( 'NONE',  ( -45.64106924314018698, 412.9323905765655809, 11.32908994701042538 ) ) ;
#3436=CARTESIAN_POINT ( 'NONE',  ( -13.20868407381884957, 289.7448905683720568, 6.410867750099229490 ) ) ;
#3438=CARTESIAN_POINT ( 'NONE',  ( -45.43829269268872650, 505.3698905683721136, 0.000000000000000000 ) ) ;
#3439=AXIS2_PLACEMENT_3D ( 'NONE', #17420, #15482, #19038 ) ;
#3441=CARTESIAN_POINT ( 'NONE',  ( -14.48388495494901385, 471.3073905683720568, -9.489475012073736337 ) ) ;
#3443=CARTESIAN_POINT ( 'NONE',  ( -40.53162694259542320, 265.1198905683720568, 11.84573899990672885 ) ) ;
#3445=LINE ( 'NONE', #322, #5917 ) ;
#3446=CARTESIAN_POINT ( 'NONE',  ( -16.84014894278197971, 261.6198905683720568, -11.84573899990672707 ) ) ;
#3447=CARTESIAN_POINT ( 'NONE',  ( -48.68588794268869435, 252.3073905765655809, 3.978247347593168115 ) ) ;
#3449=CARTESIAN_POINT ( 'NONE',  ( -45.64106924314017277, 228.1823905601784759, 11.32908994701042715 ) ) ;
#3450=CARTESIAN_POINT ( 'NONE',  ( -11.73070664223723725, 257.9323905765656377, -11.32908994701042538 ) ) ;
#3451=CARTESIAN_POINT ( 'NONE',  ( -25.35362745456396993, 266.6823905683720568, 16.75240474999998952 ) ) ;
#3452=CARTESIAN_POINT ( 'NONE',  ( -35.09675569278795138, 357.2448905683720000, 15.47720386886985366 ) ) ;
#3455=CARTESIAN_POINT ( 'NONE',  ( -44.16309181155857289, 424.4948905683720568, 6.410867750099241924 ) ) ;
#3458=CARTESIAN_POINT ( 'NONE',  ( -47.16347859291445133, 397.8698905601784759, 7.653668647301805628 ) ) ;
#3461=ORIENTED_EDGE ( 'NONE', *, *, #6048, .T. ) ;
#3462=CARTESIAN_POINT ( 'NONE',  ( -25.35362745456400191, 528.1823905683719431, 16.75240474999998952 ) ) ;
#3463=CARTESIAN_POINT ( 'NONE',  ( -8.685887942688715668, 301.9323905601784190, 3.978247347593161010 ) ) ;
#3465=CARTESIAN_POINT ( 'NONE',  ( -32.01814843081344009, 323.1823905683720000, -16.75240474999999307 ) ) ;
#3467=CARTESIAN_POINT ( 'NONE',  ( -32.66413529028189089, 489.8073905765656377, -19.99999999999999289 ) ) ;
#3468=CARTESIAN_POINT ( 'NONE',  ( -19.19641293061498288, 357.3073905683720568, 14.20200298773971426 ) ) ;
#3469=CARTESIAN_POINT ( 'NONE',  ( -35.09675569278794427, 361.9948905683720568, -15.47720386886985544 ) ) ;
#3472=CARTESIAN_POINT ( 'NONE',  ( -24.70764059509555466, 299.1823905765656377, -19.99999999999999289 ) ) ;
#3474=CARTESIAN_POINT ( 'NONE',  ( -45.43829269268870519, 273.5573905683720000, -3.332260488124726638 ) ) ;
#3476=CARTESIAN_POINT ( 'NONE',  ( -45.43829269268871940, 425.3698905683720568, 0.000000000000000000 ) ) ;
#3477=DIRECTION ( 'NONE',  ( -1.191790137725560488E-16, 1.000000000000000000, -0.000000000000000000 ) ) ;
#3478=CARTESIAN_POINT ( 'NONE',  ( -36.33955658999052929, 515.3698905601784190, -18.47759065022572855 ) ) ;
#3480=DIRECTION ( 'NONE',  ( -1.000000000000000000, 0.000000000000000000, 0.000000000000000000 ) ) ;
#3481=CARTESIAN_POINT ( 'NONE',  ( -38.17536295476244135, 326.9323905683720568, 14.20200298773971781 ) ) ;
#3482=CARTESIAN_POINT ( 'NONE',  ( -44.16309181155858710, 483.2448905683720000, -6.410867750099231266 ) ) ;
#3483=ORIENTED_EDGE ( 'NONE', *, *, #11940, .F. ) ;
#3484=CARTESIAN_POINT ( 'NONE',  ( -8.685887942688736985, 481.9323905601784759, 3.978247347593161010 ) ) ;
#3485=CARTESIAN_POINT ( 'NONE',  ( -42.88789093042842637, 304.8073905683720000, 9.489475012073736337 ) ) ;
#3486=ADVANCED_FACE ( 'NONE', ( #10499 ), #20149, .T. ) ;
#3490=CARTESIAN_POINT ( 'NONE',  ( -11.73070664223724613, 346.0573905765656377, 11.32908994701042005 ) ) ;
#3491=ORIENTED_EDGE ( 'NONE', *, *, #4797, .F. ) ;
#3493=CARTESIAN_POINT ( 'NONE',  ( -13.20868407381886556, 410.9948905683720000, -6.410867750099233042 ) ) ;
#3494=CARTESIAN_POINT ( 'NONE',  ( -32.66413529028186957, 384.1823905765656377, 19.99999999999999289 ) ) ;
#3495=CARTESIAN_POINT ( 'NONE',  ( -44.16309181155857289, 414.4948905683720000, 6.410867750099241924 ) ) ;
#3496=CARTESIAN_POINT ( 'NONE',  ( -11.93348319268871016, 260.6823905683720000, -3.332260488124732856 ) ) ;
#3497=CARTESIAN_POINT ( 'NONE',  ( -13.20868407381886911, 448.2448905683720000, 6.410867750099229490 ) ) ;
#3501=CARTESIAN_POINT ( 'NONE',  ( -48.68588794268870856, 371.6823905765656377, -3.978247347593158345 ) ) ;
#3503=CARTESIAN_POINT ( 'NONE',  ( -8.685887942688532704, 262.5573905601784190, -3.978247347592740013 ) ) ;
#3504=CARTESIAN_POINT ( 'NONE',  ( -11.93348319268871727, 328.5573905683720568, 3.332260488124728859 ) ) ;
#3506=CARTESIAN_POINT ( 'NONE',  ( -45.43829269268871940, 505.0573905683721136, -3.332260488124726194 ) ) ;
#3508=CARTESIAN_POINT ( 'NONE',  ( -36.33955658999052218, 465.3698905601784759, -18.47759065022572855 ) ) ;
#3509=CARTESIAN_POINT ( 'NONE',  ( -48.68588794268873698, 573.2448905601785327, 0.000000000000000000 ) ) ;
#3510=CARTESIAN_POINT ( 'NONE',  ( -22.27502019258947996, 398.4948905683720000, 15.47720386886985189 ) ) ;
#3512=( BOUNDED_CURVE ( )  B_SPLINE_CURVE ( 2, ( #1201, #17730, #6257, #1618, #9715, #2924, #13192, #7979, #1298, #7771, #7872, #16336, #14501, #12971, #6361, #8191, #21084 ),
 .UNSPECIFIED., .F., .T. ) 
 B_SPLINE_CURVE_WITH_KNOTS ( ( 3, 2, 2, 2, 2, 2, 2, 2, 3 ),
 ( 0.1875000000000001665, 0.1894531250000001665, 0.1914062500000001665, 0.1933593750000001665, 0.1953125000000001665, 0.1972656250000001665, 0.1992187500000001665, 0.2011718750000001665, 0.2031250000000001665 ),
 .UNSPECIFIED. ) 
 CURVE ( )  GEOMETRIC_REPRESENTATION_ITEM ( )  RATIONAL_B_SPLINE_CURVE ( ( 0.9999999999999983347, 0.9807852804032320959, 1.000000000000000000, 0.9807852804032304306, 1.000000000000000000, 0.9807852804032304306, 1.000000000000000000, 0.9807852804032304306, 1.000000000000000000, 0.9807852804032304306, 1.000000000000000000, 0.9807852804032304306, 1.000000000000000000, 0.9807852804032304306, 1.000000000000000000, 0.9807852804032287652, 1.000000000000001554 ) ) 
 REPRESENTATION_ITEM ( '' )  );
#3513=CARTESIAN_POINT ( 'NONE',  ( -20.29730442470228624, 222.0357903062241860, -14.50085278421890322 ) ) ;
#3514=CARTESIAN_POINT ( 'NONE',  ( -22.27502019258948707, 370.7448905683720568, -15.47720386886985544 ) ) ;
#3515=VERTEX_POINT ( 'NONE', #15498 ) ;
#3516=CARTESIAN_POINT ( 'NONE',  ( -32.01814843081346851, 516.0573905683720568, 16.75240474999999307 ) ) ;
#3518=CARTESIAN_POINT ( 'NONE',  ( -42.88789093042844058, 446.3073905683720568, 9.489475012073734561 ) ) ;
#3519=CARTESIAN_POINT ( 'NONE',  ( -32.01814843081346851, 521.6823905683720568, -16.75240474999999307 ) ) ;
#3522=CARTESIAN_POINT ( 'NONE',  ( -28.68588794268873698, 529.4948905765655809, -19.99999999999999289 ) ) ;
#3523=CARTESIAN_POINT ( 'NONE',  ( -44.16309181155857999, 484.4948905683720000, 6.410867750099241924 ) ) ;
#3526=CARTESIAN_POINT ( 'NONE',  ( -48.68588794268872277, 487.2448905601784759, 0.000000000000000000 ) ) ;
#3527=CARTESIAN_POINT ( 'NONE',  ( -40.01497788969914637, 430.4323905765655809, -16.95518130045146421 ) ) ;
#3531=CARTESIAN_POINT ( 'NONE',  ( -48.68588794268872277, 471.9948905765656377, 0.000000000000000000 ) ) ;
#3535=CARTESIAN_POINT ( 'NONE',  ( -43.68588794268869435, 200.1437886375728965, -2.037320803886357560E-15 ) ) ;
#3536=CARTESIAN_POINT ( 'NONE',  ( -22.27502019258946930, 288.4948905683720000, 15.47720386886985189 ) ) ;
#3537=CARTESIAN_POINT ( 'NONE',  ( -21.03221929538690915, 234.1198905601784475, -18.47759065022572855 ) ) ;
#3538=CARTESIAN_POINT ( 'NONE',  ( -14.54375231895775578, 270.9948905601784759, 14.14213562373094568 ) ) ;
#3541=CARTESIAN_POINT ( 'NONE',  ( -11.93348319268871016, 280.3698905683720000, -2.051577885510841163E-15 ) ) ;
#3545=CARTESIAN_POINT ( 'NONE',  ( -11.93348319268873858, 500.0573905683720568, 3.332260488124728859 ) ) ;
#3547=ADVANCED_FACE ( 'NONE', ( #17120 ), #20248, .T. ) ;
#3549=CARTESIAN_POINT ( 'NONE',  ( -11.93348319268873325, 460.6823905683720568, -3.332260488124732856 ) ) ;
#3550=CARTESIAN_POINT ( 'NONE',  ( -38.17536295476243424, 265.4323905683720568, 14.20200298773971781 ) ) ;
#3552=ORIENTED_EDGE ( 'NONE', *, *, #6959, .F. ) ;
#3554=CARTESIAN_POINT ( 'NONE',  ( -19.19641293061496867, 251.9323905683720284, -14.20200298773971603 ) ) ;
#3556=CARTESIAN_POINT ( 'NONE',  ( -45.64106924314017277, 252.9323905765656377, 11.32908994701042715 ) ) ;
#3558=CARTESIAN_POINT ( 'NONE',  ( -48.68588794268869435, 226.9323905601785043, -3.978247347593158345 ) ) ;
#3559=CARTESIAN_POINT ( 'NONE',  ( -13.20868407381884779, 258.2448905683720000, 6.410867750099229490 ) ) ;
#3560=CARTESIAN_POINT ( 'NONE',  ( -45.43829269268870519, 365.6823905683720568, 3.332260488124734632 ) ) ;
#3561=CARTESIAN_POINT ( 'NONE',  ( -8.685887942688742314, 573.2448905601785327, 2.449293598294706119E-15 ) ) ;
#3562=VECTOR ( 'NONE', #14190, 1000.000000000000000 ) ;
#3563=CARTESIAN_POINT ( 'NONE',  ( -44.16309181155857289, 404.4948905683720000, 6.410867750099241924 ) ) ;
#3564=CARTESIAN_POINT ( 'NONE',  ( -40.01497788969915348, 508.8073905601784190, 16.95518130045146776 ) ) ;
#3565=ORIENTED_EDGE ( 'NONE', *, *, #17674, .T. ) ;
#3566=CARTESIAN_POINT ( 'NONE',  ( -11.73070664223725146, 401.3073905601784759, 11.32908994701042005 ) ) ;
#3568=ORIENTED_EDGE ( 'NONE', *, *, #10003, .F. ) ;
#3570=CARTESIAN_POINT ( 'NONE',  ( -42.88789093042845479, 526.3073905683720568, 9.489475012073736337 ) ) ;
#3571=CARTESIAN_POINT ( 'NONE',  ( -21.03221929538691626, 294.1198905601785327, -18.47759065022572855 ) ) ;
#3572=CARTESIAN_POINT ( 'NONE',  ( -43.68588794268869435, 210.1437886375729533, -0.1639321870911867873 ) ) ;
#3574=CARTESIAN_POINT ( 'NONE',  ( -25.35362745456398770, 332.5573905683719431, -16.75240474999999307 ) ) ;
#3576=CARTESIAN_POINT ( 'NONE',  ( -32.01814843081344719, 371.6823905683720000, -16.75240474999999307 ) ) ;
#3577=CARTESIAN_POINT ( 'NONE',  ( -40.53162694259543741, 375.1198905683720000, 11.84573899990672885 ) ) ;
#3578=CARTESIAN_POINT ( 'NONE',  ( -36.33955658999050797, 303.8698905765656377, 18.47759065022572500 ) ) ;
#3580=CARTESIAN_POINT ( 'NONE',  ( -11.93348319268870839, 259.1823905683720568, -3.332260488124732856 ) ) ;
#3581=CARTESIAN_POINT ( 'NONE',  ( -42.82802356641966668, 438.4948905601784759, 14.14213562373094923 ) ) ;
#3582=CARTESIAN_POINT ( 'NONE',  ( -45.43829269268871229, 425.6823905683720568, 3.332260488124734632 ) ) ;
#3587=CARTESIAN_POINT ( 'NONE',  ( -17.35679799567829562, 410.6823905601784759, 16.95518130045146421 ) ) ;
#3588=CARTESIAN_POINT ( 'NONE',  ( -13.20868407381885490, 329.7448905683720568, 6.410867750099229490 ) ) ;
#3589=CARTESIAN_POINT ( 'NONE',  ( -11.93348319268873503, 479.1823905683721136, -3.332260488124732856 ) ) ;
#3591=CARTESIAN_POINT ( 'NONE',  ( -32.66413529028189089, 475.0573905601785327, -19.99999999999999289 ) ) ;
#3592=CARTESIAN_POINT ( 'NONE',  ( -42.88789093042842637, 302.9323905683720568, -9.489475012073736337 ) ) ;
#3596=CARTESIAN_POINT ( 'NONE',  ( -21.03221929538690915, 345.1198905765656377, 18.47759065022572500 ) ) ;
#3599=CARTESIAN_POINT ( 'NONE',  ( -13.20868407381886200, 380.9948905683720568, -6.410867750099233042 ) ) ;
#3600=CARTESIAN_POINT ( 'NONE',  ( -45.64106924314019409, 478.1823905601785327, 11.32908994701042538 ) ) ;
#3602=CARTESIAN_POINT ( 'NONE',  ( -14.48388495494900496, 427.9323905683720568, 9.489475012073732785 ) ) ;
#3603=CARTESIAN_POINT ( 'NONE',  ( -40.53162694259542320, 266.6198905683720568, 11.84573899990672885 ) ) ;
#3604=CARTESIAN_POINT ( 'NONE',  ( -40.53162694259544452, 435.1198905683720000, 11.84573899990672885 ) ) ;
#3605=CARTESIAN_POINT ( 'NONE',  ( -8.685887942688742314, 573.2448905601785327, 2.449293598294706119E-15 ) ) ;
#3606=CARTESIAN_POINT ( 'NONE',  ( -32.66413529028187668, 354.1823905765656377, 19.99999999999999289 ) ) ;
#3608=DIRECTION ( 'NONE',  ( -1.191790137725560488E-16, 1.000000000000000000, -0.000000000000000000 ) ) ;
#3609=CARTESIAN_POINT ( 'NONE',  ( -32.01814843081344009, 326.0573905683719431, 16.75240474999999307 ) ) ;
#3610=DIRECTION ( 'NONE',  ( -1.000000000000000000, 0.000000000000000000, 0.000000000000000000 ) ) ;
#3611=CARTESIAN_POINT ( 'NONE',  ( -19.19641293061499354, 468.8073905683720000, 14.20200298773971426 ) ) ;
#3613=CARTESIAN_POINT ( 'NONE',  ( -42.82802356641966668, 433.2448905765656377, 14.14213562373094923 ) ) ;
#3615=CARTESIAN_POINT ( 'NONE',  ( -40.01497788969913927, 418.8073905601785896, 16.95518130045146776 ) ) ;
#3616=CARTESIAN_POINT ( 'NONE',  ( -22.27502019258947996, 388.4948905683720000, 15.47720386886985189 ) ) ;
#3618=CARTESIAN_POINT ( 'NONE',  ( -21.03221929538693047, 530.3698905601784190, 18.47759065022572500 ) ) ;
#3619=CARTESIAN_POINT ( 'NONE',  ( -40.53162694259543741, 362.6198905683720000, -11.84573899990672707 ) ) ;
#3623=CARTESIAN_POINT ( 'NONE',  ( -45.43829269268872650, 524.1823905683720568, 3.332260488124734632 ) ) ;
#3625=CARTESIAN_POINT ( 'NONE',  ( -42.88789093042844058, 436.3073905683720568, 9.489475012073734561 ) ) ;
#3626=CARTESIAN_POINT ( 'NONE',  ( -14.48388495494901740, 527.9323905683719431, 9.489475012073732785 ) ) ;
#3629=CARTESIAN_POINT ( 'NONE',  ( -42.88789093042844769, 484.8073905683720000, 9.489475012073736337 ) ) ;
#3631=CARTESIAN_POINT ( 'NONE',  ( -13.20868407381887444, 488.2448905683720000, 6.410867750099229490 ) ) ;
#3633=CARTESIAN_POINT ( 'NONE',  ( -48.68588794268871567, 432.3073905765656946, 3.978247347593168115 ) ) ;
#3636=CARTESIAN_POINT ( 'NONE',  ( -42.82802356641966668, 440.7448905765656377, -14.14213562373094746 ) ) ;
#3639=CARTESIAN_POINT ( 'NONE',  ( -47.16347859291445133, 436.6198905601784759, -7.653668647301793193 ) ) ;
#3640=CARTESIAN_POINT ( 'NONE',  ( -42.82802356641963826, 204.8148611821455916, -5.000000000000001776 ) ) ;
#3641=( BOUNDED_CURVE ( )  B_SPLINE_CURVE ( 2, ( #10065, #14056, #3690, #18500, #6924, #13550, #9059, #10276, #5924, #2691, #17402, #12535, #2077, #15573, #20139, #360, #19129 ),
 .UNSPECIFIED., .F., .T. ) 
 B_SPLINE_CURVE_WITH_KNOTS ( ( 3, 2, 2, 2, 2, 2, 2, 2, 3 ),
 ( 0.7968750000000002220, 0.7988281250000002220, 0.8007812500000002220, 0.8027343750000002220, 0.8046875000000002220, 0.8066406250000002220, 0.8085937500000002220, 0.8105468750000002220, 0.8125000000000002220 ),
 .UNSPECIFIED. ) 
 CURVE ( )  GEOMETRIC_REPRESENTATION_ITEM ( )  RATIONAL_B_SPLINE_CURVE ( ( 0.9999999999999977796, 0.9807852804032326510, 1.000000000000000000, 0.9807852804032304306, 1.000000000000000000, 0.9807852804032304306, 1.000000000000000000, 0.9807852804032304306, 1.000000000000000000, 0.9807852804032304306, 1.000000000000000000, 0.9807852804032304306, 1.000000000000000000, 0.9807852804032304306, 1.000000000000000000, 0.9807852804032282101, 1.000000000000002220 ) ) 
 REPRESENTATION_ITEM ( '' )  );
#3642=CARTESIAN_POINT ( 'NONE',  ( -45.43829269268870519, 305.3698905683720568, 0.000000000000000000 ) ) ;
#3645=CARTESIAN_POINT ( 'NONE',  ( -38.17536295476246266, 456.9323905683720000, 14.20200298773971781 ) ) ;
#3646=CARTESIAN_POINT ( 'NONE',  ( -48.68588794268873698, 573.2448905601785327, 0.000000000000000000 ) ) ;
#3647=CARTESIAN_POINT ( 'NONE',  ( -25.35362745456398414, 292.5573905683720568, -16.75240474999999307 ) ) ;
#3649=CARTESIAN_POINT ( 'NONE',  ( -32.66413529028185536, 269.4323905601784759, 19.99999999999999289 ) ) ;
#3650=CARTESIAN_POINT ( 'NONE',  ( -32.01814843081346140, 513.1823905683721705, -16.75240474999999307 ) ) ;
#3652=CARTESIAN_POINT ( 'NONE',  ( -35.09675569278795848, 473.4948905683720000, -15.47720386886985544 ) ) ;
#3654=CARTESIAN_POINT ( 'NONE',  ( -25.35362745456398059, 261.0573905683720000, -16.75240474999999307 ) ) ;
#3655=ORIENTED_EDGE ( 'NONE', *, *, #12335, .F. ) ;
#3657=CARTESIAN_POINT ( 'NONE',  ( -13.20868407381884957, 270.9948905683720000, -6.410867750099233042 ) ) ;
#3658=CARTESIAN_POINT ( 'NONE',  ( -38.17536295476243424, 236.9323905683720000, 14.20200298773971781 ) ) ;
#3661=CARTESIAN_POINT ( 'NONE',  ( -35.09675569278793716, 265.7448905683720000, 15.47720386886985366 ) ) ;
#3662=CARTESIAN_POINT ( 'NONE',  ( -28.68588794268871212, 347.8698905683720568, 16.75240474999999307 ) ) ;
#3664=AXIS2_PLACEMENT_3D ( 'NONE', #7699, #2528, #16051 ) ;
#3665=CARTESIAN_POINT ( 'NONE',  ( -11.93348319268872615, 408.5573905683720568, 3.332260488124728415 ) ) ;
#3666=CARTESIAN_POINT ( 'NONE',  ( -8.685887942689081598, 511.9323905601784759, 3.978247347593985683 ) ) ;
#3668=CARTESIAN_POINT ( 'NONE',  ( -28.68588794268872277, 414.7448905601784759, -19.99999999999999289 ) ) ;
#3675=CARTESIAN_POINT ( 'NONE',  ( -42.88789093042845479, 534.4323905683720568, -9.489475012073736337 ) ) ;
#3676=CARTESIAN_POINT ( 'NONE',  ( -40.01497788969912506, 288.8073905601785327, 16.95518130045146776 ) ) ;
#3678=CARTESIAN_POINT ( 'NONE',  ( -44.16309181155855867, 325.9948905683720000, 6.410867750099241924 ) ) ;
#3680=CARTESIAN_POINT ( 'NONE',  ( -42.88789093042843348, 354.8073905683720568, 9.489475012073736337 ) ) ;
#3681=CARTESIAN_POINT ( 'NONE',  ( -22.27502019258947641, 366.9948905683720568, 15.47720386886985189 ) ) ;
#3683=CARTESIAN_POINT ( 'NONE',  ( -47.16347859291443712, 312.6198905765655809, 7.653668647301805628 ) ) ;
#3684=CARTESIAN_POINT ( 'NONE',  ( -42.88789093042841927, 262.9323905683720568, -9.489475012073734561 ) ) ;
#3685=CARTESIAN_POINT ( 'NONE',  ( -32.66413529028188378, 464.1823905765656377, 19.99999999999999289 ) ) ;
#3686=CARTESIAN_POINT ( 'NONE',  ( -14.48388495494900496, 421.3073905683720000, -9.489475012073736337 ) ) ;
#3688=LINE ( 'NONE', #5304, #6453 ) ;
#3689=CARTESIAN_POINT ( 'NONE',  ( -36.33955658999053639, 503.8698905765656377, 18.47759065022572500 ) ) ;
#3690=CARTESIAN_POINT ( 'NONE',  ( -10.20829729246297646, 276.3698905765656377, 7.653668647301790529 ) ) ;
#3691=CARTESIAN_POINT ( 'NONE',  ( -28.68588794268871212, 332.8698905683720000, -16.75240474999999307 ) ) ;
#3692=CARTESIAN_POINT ( 'NONE',  ( -19.19641293061499709, 470.4323905683719431, -14.20200298773971603 ) ) ;
#3694=CARTESIAN_POINT ( 'NONE',  ( -40.01497788969915348, 475.6823905601784190, -16.95518130045146421 ) ) ;
#3695=CARTESIAN_POINT ( 'NONE',  ( -45.43829269268869808, 293.5573905683720568, -3.332260488124726194 ) ) ;
#3696=VECTOR ( 'NONE', #19761, 1000.000000000000000 ) ;
#3700=CARTESIAN_POINT ( 'NONE',  ( -42.88789093042843348, 384.4323905683720568, -9.489475012073734561 ) ) ;
#3701=DIRECTION ( 'NONE',  ( -1.191790137725560488E-16, 1.000000000000000000, -0.000000000000000000 ) ) ;
#3702=CARTESIAN_POINT ( 'NONE',  ( -48.68588794268870856, 381.9948905765655809, 0.000000000000000000 ) ) ;
#3703=CARTESIAN_POINT ( 'NONE',  ( -28.68588794268872277, 431.3698905683720000, -16.75240474999999307 ) ) ;
#3704=CARTESIAN_POINT ( 'NONE',  ( -44.16309181155855157, 265.9948905683720000, 6.410867750099241924 ) ) ;
#3705=CARTESIAN_POINT ( 'NONE',  ( -13.20868407381886733, 419.4948905683720000, -6.410867750099233042 ) ) ;
#3707=CARTESIAN_POINT ( 'NONE',  ( -48.68588794268870856, 361.6823905765656946, -3.978247347593158345 ) ) ;
#3709=CARTESIAN_POINT ( 'NONE',  ( -25.35362745456398770, 321.0573905683720000, -16.75240474999999307 ) ) ;
#3710=CARTESIAN_POINT ( 'NONE',  ( -8.685887942688742314, 573.2448905601785327, 2.449293598294706119E-15 ) ) ;
#3711=CARTESIAN_POINT ( 'NONE',  ( -44.16309181155857999, 475.9948905683720000, 6.410867750099241924 ) ) ;
#3715=CARTESIAN_POINT ( 'NONE',  ( -42.82802356641965247, 305.9948905601784759, -14.14213562373094746 ) ) ;
#3718=CARTESIAN_POINT ( 'NONE',  ( -45.43829269268871940, 395.3698905683720000, 0.000000000000000000 ) ) ;
#3721=CARTESIAN_POINT ( 'NONE',  ( -14.54375231895778775, 530.9948905601784190, 14.14213562373094568 ) ) ;
#3722=CARTESIAN_POINT ( 'NONE',  ( -32.01814843081344719, 356.0573905683719431, 16.75240474999999307 ) ) ;
#3724=CARTESIAN_POINT ( 'NONE',  ( -14.48388495494901740, 527.9323905683719431, 9.489475012073732785 ) ) ;
#3726=CARTESIAN_POINT ( 'NONE',  ( -45.43829269268872650, 523.5573905683721705, -3.332260488124726194 ) ) ;
#3728=CARTESIAN_POINT ( 'NONE',  ( -17.35679799567831338, 493.8073905601785327, -16.95518130045146421 ) ) ;
#3729=CARTESIAN_POINT ( 'NONE',  ( -22.27502019258949062, 476.9948905683720000, 15.47720386886985189 ) ) ;
#3731=CARTESIAN_POINT ( 'NONE',  ( -28.68588794268873343, 491.3698905683720568, -16.75240474999999307 ) ) ;
#3733=CARTESIAN_POINT ( 'NONE',  ( -36.33955658999051508, 420.1198905765656377, -18.47759065022572855 ) ) ;
#3738=DIRECTION ( 'NONE',  ( -1.000000000000000000, 0.000000000000000000, 0.000000000000000000 ) ) ;
#3740=CARTESIAN_POINT ( 'NONE',  ( -38.17536295476244845, 303.8073905683720000, -14.20200298773971426 ) ) ;
#3743=CARTESIAN_POINT ( 'NONE',  ( -40.53162694259545162, 454.1198905683720568, -11.84573899990672707 ) ) ;
#3745=CARTESIAN_POINT ( 'NONE',  ( -14.48388495494898720, 279.4323905683720568, 9.489475012073732785 ) ) ;
#3748=CARTESIAN_POINT ( 'NONE',  ( -25.35362745456400901, 512.5573905683720568, -16.75240474999999307 ) ) ;
#3751=CARTESIAN_POINT ( 'NONE',  ( -16.84014894278199748, 459.1198905683720568, 11.84573899990672530 ) ) ;
#3753=CARTESIAN_POINT ( 'NONE',  ( -11.93348319268871016, 259.1823905683720000, -3.332260488124732856 ) ) ;
#3755=CARTESIAN_POINT ( 'NONE',  ( -36.33955658999051508, 333.8698905765656377, 18.47759065022572500 ) ) ;
#3757=CARTESIAN_POINT ( 'NONE',  ( -11.73070664223724613, 307.9323905765656946, -11.32908994701042538 ) ) ;
#3758=CARTESIAN_POINT ( 'NONE',  ( -42.88789093042841927, 236.3073905683720284, 9.489475012073734561 ) ) ;
#3759=( BOUNDED_CURVE ( )  B_SPLINE_CURVE ( 2, ( #20392, #11953, #12281, #410, #12173, #3948, #18863, #13597, #20184, #8706, #2233, #4053, #8812, #18549, #10533, #16943, #15429 ),
 .UNSPECIFIED., .F., .T. ) 
 B_SPLINE_CURVE_WITH_KNOTS ( ( 3, 2, 2, 2, 2, 2, 2, 2, 3 ),
 ( 0.1718750000000001665, 0.1738281250000001665, 0.1757812500000001665, 0.1777343750000001665, 0.1796875000000001665, 0.1816406250000001665, 0.1835937500000001665, 0.1855468750000001665, 0.1875000000000001665 ),
 .UNSPECIFIED. ) 
 CURVE ( )  GEOMETRIC_REPRESENTATION_ITEM ( )  RATIONAL_B_SPLINE_CURVE ( ( 0.9999999999999983347, 0.9807852804032320959, 1.000000000000000000, 0.9807852804032304306, 1.000000000000000000, 0.9807852804032304306, 1.000000000000000000, 0.9807852804032304306, 1.000000000000000000, 0.9807852804032304306, 1.000000000000000000, 0.9807852804032304306, 1.000000000000000000, 0.9807852804032304306, 1.000000000000000000, 0.9807852804032287652, 1.000000000000001554 ) ) 
 REPRESENTATION_ITEM ( '' )  );
#3760=ADVANCED_FACE ( 'NONE', ( #19052 ), #6061, .T. ) ;
#3762=CARTESIAN_POINT ( 'NONE',  ( -18.67110661049051146, 223.9107902980306335, -17.31196565581893765 ) ) ;
#3764=CARTESIAN_POINT ( 'NONE',  ( -42.88789093042841927, 244.8073905683720568, 9.489475012073736337 ) ) ;
#3765=CARTESIAN_POINT ( 'NONE',  ( -44.16309181155857289, 364.7448905683720568, -6.410867750099231266 ) ) ;
#3766=CARTESIAN_POINT ( 'NONE',  ( -36.33955658999050797, 279.1198905601784759, 18.47759065022572500 ) ) ;
#3768=CARTESIAN_POINT ( 'NONE',  ( -19.19641293061498999, 400.4323905683720568, -14.20200298773971603 ) ) ;
#3770=CARTESIAN_POINT ( 'NONE',  ( -32.66413529028188378, 415.0573905601785327, -19.99999999999999289 ) ) ;
#3775=DIRECTION ( 'NONE',  ( -1.191790137725560488E-16, 1.000000000000000000, -0.000000000000000000 ) ) ;
#3776=CARTESIAN_POINT ( 'NONE',  ( -24.70764059509553690, 280.0573905601784759, 19.99999999999998934 ) ) ;
#3778=CARTESIAN_POINT ( 'NONE',  ( -40.53162694259543031, 316.6198905683720568, 11.84573899990672885 ) ) ;
#3779=CARTESIAN_POINT ( 'NONE',  ( -35.09675569278795138, 345.7448905683720568, 15.47720386886985366 ) ) ;
#3780=CARTESIAN_POINT ( 'NONE',  ( -45.43829269268871229, 364.1823905683720568, 3.332260488124734632 ) ) ;
#3782=CARTESIAN_POINT ( 'NONE',  ( -42.82802356641965247, 283.2448905765656377, 14.14213562373094923 ) ) ;
#3784=CARTESIAN_POINT ( 'NONE',  ( -32.01814843081344009, 276.0573905683720568, 16.75240474999999307 ) ) ;
#3787=CARTESIAN_POINT ( 'NONE',  ( -14.48388495494900496, 419.4323905683720568, 9.489475012073732785 ) ) ;
#3789=DIRECTION ( 'NONE',  ( -1.191790137725560488E-16, 1.000000000000000000, -0.000000000000000000 ) ) ;
#3790=CARTESIAN_POINT ( 'NONE',  ( -21.03221929538692692, 505.1198905765656946, 18.47759065022572500 ) ) ;
#3792=CARTESIAN_POINT ( 'NONE',  ( -42.88789093042842637, 326.3073905683721136, 9.489475012073736337 ) ) ;
#3793=CARTESIAN_POINT ( 'NONE',  ( -35.09675569278795848, 461.9948905683720000, -15.47720386886985544 ) ) ;
#3795=CARTESIAN_POINT ( 'NONE',  ( -42.82802356641967378, 468.4948905601785327, 14.14213562373094923 ) ) ;
#3796=CARTESIAN_POINT ( 'NONE',  ( -35.09675569278793716, 291.9948905683720000, -15.47720386886985544 ) ) ;
#3798=CARTESIAN_POINT ( 'NONE',  ( -36.33955658999051508, 339.1198905601784759, 18.47759065022572500 ) ) ;
#3801=CARTESIAN_POINT ( 'NONE',  ( -40.01497788969913216, 338.8073905601784759, 16.95518130045146776 ) ) ;
#3802=CARTESIAN_POINT ( 'NONE',  ( -11.93348319268871549, 308.8698905683720000, -2.051577885510841163E-15 ) ) ;
#3804=CARTESIAN_POINT ( 'NONE',  ( -28.68588794268871567, 377.8698905683720000, 16.75240474999999307 ) ) ;
#3805=CARTESIAN_POINT ( 'NONE',  ( -8.685887942688742314, 573.2448905601785327, 2.449293598294706119E-15 ) ) ;
#3806=CARTESIAN_POINT ( 'NONE',  ( -28.68588794268873343, 524.4948905765655809, 19.99999999999999289 ) ) ;
#3807=CARTESIAN_POINT ( 'NONE',  ( -42.88789093042844058, 412.9323905683720000, -9.489475012073736337 ) ) ;
#3808=CARTESIAN_POINT ( 'NONE',  ( -35.09675569278793716, 257.2448905683720000, 15.47720386886985366 ) ) ;
#3809=AXIS2_PLACEMENT_3D ( 'NONE', #17252, #13795, #18641 ) ;
#3810=CARTESIAN_POINT ( 'NONE',  ( -45.43829269268871940, 423.8698905683720568, 0.000000000000000000 ) ) ;
#3812=CARTESIAN_POINT ( 'NONE',  ( -8.685887942688722774, 356.9948905765655809, -2.449293598294705724E-15 ) ) ;
#3813=CARTESIAN_POINT ( 'NONE',  ( -8.685887942688722774, 362.2448905601784190, -2.449293598294705724E-15 ) ) ;
#3814=CARTESIAN_POINT ( 'NONE',  ( -16.84014894278198327, 327.6198905683720000, 11.84573899990672530 ) ) ;
#3815=CARTESIAN_POINT ( 'NONE',  ( -16.84014894278200103, 479.1198905683720000, 11.84573899990672530 ) ) ;
#3817=CARTESIAN_POINT ( 'NONE',  ( -11.73070664223725501, 436.0573905765656377, 11.32908994701042005 ) ) ;
#3820=VECTOR ( 'NONE', #14573, 1000.000000000000000 ) ;
#3821=CARTESIAN_POINT ( 'NONE',  ( -40.53162694259543741, 384.1198905683720568, -11.84573899990672707 ) ) ;
#3825=CARTESIAN_POINT ( 'NONE',  ( -11.73070664223727100, 533.1823905601785327, -11.32908994701042715 ) ) ;
#3826=CARTESIAN_POINT ( 'NONE',  ( -14.48388495494899786, 349.8073905683720000, -9.489475012073736337 ) ) ;
#3828=CARTESIAN_POINT ( 'NONE',  ( -32.01814843081346851, 521.6823905683720568, -16.75240474999999307 ) ) ;
#3834=CARTESIAN_POINT ( 'NONE',  ( -10.20829729246300666, 527.6198905765656946, -7.653668647301794969 ) ) ;
#3835=CARTESIAN_POINT ( 'NONE',  ( -44.16309181155857999, 474.4948905683720000, 6.410867750099241924 ) ) ;
#3836=ORIENTED_EDGE ( 'NONE', *, *, #453, .F. ) ;
#3837=CARTESIAN_POINT ( 'NONE',  ( -19.19641293061499709, 480.4323905683720568, -14.20200298773971603 ) ) ;
#3839=CARTESIAN_POINT ( 'NONE',  ( -42.82802356641966668, 423.2448905765656377, 14.14213562373094923 ) ) ;
#3843=CARTESIAN_POINT ( 'NONE',  ( -8.685887942688715668, 302.2448905601784190, -2.449293598294705724E-15 ) ) ;
#3844=CARTESIAN_POINT ( 'NONE',  ( -45.43829269268873361, 533.8698905683720568, 0.000000000000000000 ) ) ;
#3845=CARTESIAN_POINT ( 'NONE',  ( -21.03221929538692336, 485.1198905765656377, 18.47759065022572500 ) ) ;
#3846=CYLINDRICAL_SURFACE ( 'NONE', #16486, 19.99999999999999645 ) ;
#3847=CARTESIAN_POINT ( 'NONE',  ( -36.33955658999051508, 435.3698905601784759, -18.47759065022572855 ) ) ;
#3849=CARTESIAN_POINT ( 'NONE',  ( -28.68588794268870146, 277.8698905683720000, 16.75240474999999307 ) ) ;
#3850=CARTESIAN_POINT ( 'NONE',  ( -8.685887942688724550, 366.9948905765655809, -2.449293598294705724E-15 ) ) ;
#3851=CARTESIAN_POINT ( 'NONE',  ( -14.48388495494900852, 451.3073905683721136, -9.489475012073736337 ) ) ;
#3852=CARTESIAN_POINT ( 'NONE',  ( -8.685887942688594876, 397.3073905765656946, -3.978247347592846594 ) ) ;
#3853=CARTESIAN_POINT ( 'NONE',  ( -19.19641293061497578, 271.9323905683720568, -14.20200298773971603 ) ) ;
#3855=CARTESIAN_POINT ( 'NONE',  ( -8.685887942688742314, 532.2448905601784190, -2.449293598294705724E-15 ) ) ;
#3856=CARTESIAN_POINT ( 'NONE',  ( -28.68588794268872633, 477.8698905683720568, 16.75240474999999307 ) ) ;
#3859=CARTESIAN_POINT ( 'NONE',  ( -8.685887942688594876, 407.3073905765656946, -3.978247347592846594 ) ) ;
#3860=CARTESIAN_POINT ( 'NONE',  ( -11.93348319268871016, 258.5573905683720568, 3.332260488124728415 ) ) ;
#3863=CARTESIAN_POINT ( 'NONE',  ( -11.93348319268871016, 270.3698905683720000, -2.051577885510841163E-15 ) ) ;
#3864=CARTESIAN_POINT ( 'NONE',  ( -48.68588794268872277, 482.3073905765656377, 3.978247347593168115 ) ) ;
#3865=CARTESIAN_POINT ( 'NONE',  ( -17.35679799567828852, 308.5573905765656946, -16.95518130045146421 ) ) ;
#3866=CARTESIAN_POINT ( 'NONE',  ( -28.68588794268869790, 237.8698905683720568, 16.75240474999999307 ) ) ;
#3867=CARTESIAN_POINT ( 'NONE',  ( -16.84014894278201169, 521.6198905683719431, -11.84573899990672707 ) ) ;
#3868=CARTESIAN_POINT ( 'NONE',  ( -48.68588794268870856, 371.9948905765655809, 0.000000000000000000 ) ) ;
#3870=CARTESIAN_POINT ( 'NONE',  ( -32.01814843081343298, 246.0573905683720000, 16.75240474999999307 ) ) ;
#3872=CARTESIAN_POINT ( 'NONE',  ( -25.35362745456399125, 362.5573905683720568, -16.75240474999999307 ) ) ;
#3874=CARTESIAN_POINT ( 'NONE',  ( -24.70764059509553690, 280.0573905601784759, 19.99999999999998934 ) ) ;
#3875=CARTESIAN_POINT ( 'NONE',  ( -38.17536295476245556, 395.4323905683720000, 14.20200298773971781 ) ) ;
#3877=CARTESIAN_POINT ( 'NONE',  ( -17.35679799567829562, 400.6823905601784759, 16.95518130045146421 ) ) ;
#3878=EDGE_CURVE ( 'NONE', #16774, #17719, #16473, .T. ) ;
#3880=FACE_OUTER_BOUND ( 'NONE', #11169, .T. ) ;
#3883=CARTESIAN_POINT ( 'NONE',  ( -22.27502019258949417, 518.4948905683719431, 15.47720386886985189 ) ) ;
#3884=CARTESIAN_POINT ( 'NONE',  ( -32.66413529028186957, 279.4323905601785327, 19.99999999999999289 ) ) ;
#3885=CARTESIAN_POINT ( 'NONE',  ( -42.91714575264040121, 206.7622684196151965, -4.742258924317273916 ) ) ;
#3887=CARTESIAN_POINT ( 'NONE',  ( -13.20868407381885667, 330.9948905683720000, -6.410867750099233042 ) ) ;
#3888=CARTESIAN_POINT ( 'NONE',  ( -38.17536295476244845, 345.4323905683719431, 14.20200298773971781 ) ) ;
#3889=CARTESIAN_POINT ( 'NONE',  ( -22.27502019258948707, 370.7448905683720568, -15.47720386886985544 ) ) ;
#3890=CARTESIAN_POINT ( 'NONE',  ( -8.685887942688713892, 287.3073905765656377, -3.978247347593165895 ) ) ;
#3892=CARTESIAN_POINT ( 'NONE',  ( -45.43829269268870519, 273.8698905683720000, 0.000000000000000000 ) ) ;
#3896=CARTESIAN_POINT ( 'NONE',  ( -19.19641293061498999, 418.8073905683720568, 14.20200298773971426 ) ) ;
#3897=CARTESIAN_POINT ( 'NONE',  ( -45.64106924314017988, 336.3073905601784759, -11.32908994701042538 ) ) ;
#3898=CARTESIAN_POINT ( 'NONE',  ( -47.16347859291445843, 502.6198905765656377, 7.653668647301805628 ) ) ;
#3900=CARTESIAN_POINT ( 'NONE',  ( -35.09675569278794427, 327.2448905683720000, 15.47720386886985366 ) ) ;
#3901=CARTESIAN_POINT ( 'NONE',  ( -19.19641293061499354, 460.4323905683721136, -14.20200298773971603 ) ) ;
#3902=EDGE_LOOP ( 'NONE', ( #3568, #15957, #8962, #19985 ) ) ;
#3903=CARTESIAN_POINT ( 'NONE',  ( -8.685887942688735208, 462.5573905601784759, -3.978247347593165895 ) ) ;
#3904=CARTESIAN_POINT ( 'NONE',  ( -25.35362745456398414, 291.0573905683720000, -16.75240474999999307 ) ) ;
#3908=CARTESIAN_POINT ( 'NONE',  ( -48.68588794268870146, 281.9948905765656377, 0.000000000000000000 ) ) ;
#3909=CARTESIAN_POINT ( 'NONE',  ( -48.68588794268870856, 337.2448905601784759, 0.000000000000000000 ) ) ;
#3911=CARTESIAN_POINT ( 'NONE',  ( -38.17536295476244845, 292.3073905683720000, -14.20200298773971426 ) ) ;
#3912=CARTESIAN_POINT ( 'NONE',  ( -38.17536295476244845, 376.9323905683719431, 14.20200298773971781 ) ) ;
#3913=CARTESIAN_POINT ( 'NONE',  ( -10.20829729246297646, 292.8698905601784759, -7.653668647301794969 ) ) ;
#3914=CARTESIAN_POINT ( 'NONE',  ( -48.68588794268872988, 521.9948905765656946, 0.000000000000000000 ) ) ;
#3915=CARTESIAN_POINT ( 'NONE',  ( -19.19641293061498999, 407.3073905683720000, 14.20200298773971426 ) ) ;
#3916=CARTESIAN_POINT ( 'NONE',  ( -32.01814843081343298, 253.1823905683720568, -16.75240474999999307 ) ) ;
#3917=CARTESIAN_POINT ( 'NONE',  ( -19.19641293061498999, 420.4323905683720000, -14.20200298773971603 ) ) ;
#3918=CARTESIAN_POINT ( 'NONE',  ( -40.01497788969913927, 350.4323905765655809, -16.95518130045146421 ) ) ;
#3920=CARTESIAN_POINT ( 'NONE',  ( -42.88789093042842637, 322.9323905683720568, -9.489475012073734561 ) ) ;
#3921=CARTESIAN_POINT ( 'NONE',  ( -13.20868407381887266, 479.7448905683720568, 6.410867750099229490 ) ) ;
#3923=VECTOR ( 'NONE', #7411, 1000.000000000000000 ) ;
#3930=CARTESIAN_POINT ( 'NONE',  ( -25.35362745456398414, 388.1823905683720568, 16.75240474999998952 ) ) ;
#3932=CARTESIAN_POINT ( 'NONE',  ( -48.68588794268872988, 527.2448905601785327, 0.000000000000000000 ) ) ;
#3933=CARTESIAN_POINT ( 'NONE',  ( -22.27502019258947641, 346.9948905683720000, 15.47720386886985189 ) ) ;
#3935=CARTESIAN_POINT ( 'NONE',  ( -35.09675569278795848, 501.9948905683720000, -15.47720386886985544 ) ) ;
#3936=ORIENTED_EDGE ( 'NONE', *, *, #11596, .F. ) ;
#3941=CARTESIAN_POINT ( 'NONE',  ( -11.73070664223726567, 493.1823905601785327, -11.32908994701042538 ) ) ;
#3942=CARTESIAN_POINT ( 'NONE',  ( -35.09675569278795848, 471.9948905683720000, -15.47720386886985544 ) ) ;
#3944=CARTESIAN_POINT ( 'NONE',  ( -16.84014894278200458, 480.1198905683720000, -11.84573899990672707 ) ) ;
#3945=CARTESIAN_POINT ( 'NONE',  ( -8.685887942688884422, 251.9323905601784759, 3.978247347593586447 ) ) ;
#3946=AXIS2_PLACEMENT_3D ( 'NONE', #5420, #2299, #12022 ) ;
#3947=CARTESIAN_POINT ( 'NONE',  ( -28.68588794268872277, 409.4948905765656377, -19.99999999999999289 ) ) ;
#3948=CARTESIAN_POINT ( 'NONE',  ( -17.35679799567830273, 475.4323905765655809, 16.95518130045146421 ) ) ;
#3950=CARTESIAN_POINT ( 'NONE',  ( -24.70764059509557242, 484.4323905601785327, -19.99999999999999289 ) ) ;
#3951=CARTESIAN_POINT ( 'NONE',  ( -11.73070664223726212, 486.0573905765656377, 11.32908994701042005 ) ) ;
#3953=CARTESIAN_POINT ( 'NONE',  ( -14.54375231895777887, 433.4948905601784759, -14.14213562373094746 ) ) ;
#3955=CARTESIAN_POINT ( 'NONE',  ( -45.43829269268869808, 275.0573905683720568, -3.332260488124726194 ) ) ;
#3956=CARTESIAN_POINT ( 'NONE',  ( -21.03221929538690915, 254.1198905601784759, -18.47759065022572855 ) ) ;
#3957=CARTESIAN_POINT ( 'NONE',  ( -45.64106924314017988, 362.9323905765656377, 11.32908994701042538 ) ) ;
#3958=CARTESIAN_POINT ( 'NONE',  ( -11.93348319268873148, 450.0573905683719431, 3.332260488124728415 ) ) ;
#3959=CARTESIAN_POINT ( 'NONE',  ( -47.16347859291444422, 331.3698905765656377, -7.653668647301793193 ) ) ;
#3960=CARTESIAN_POINT ( 'NONE',  ( -38.17536295476244135, 276.9323905683720000, 14.20200298773971781 ) ) ;
#3961=ORIENTED_EDGE ( 'NONE', *, *, #14142, .T. ) ;
#3962=CARTESIAN_POINT ( 'NONE',  ( -45.43829269268872650, 485.0573905683721705, -3.332260488124726638 ) ) ;
#3964=DIRECTION ( 'NONE',  ( -1.000000000000000000, 0.000000000000000000, 0.000000000000000000 ) ) ;
#3965=CARTESIAN_POINT ( 'NONE',  ( -45.43829269268869808, 243.8698905683720568, 0.000000000000000000 ) ) ;
#3968=CARTESIAN_POINT ( 'NONE',  ( -40.01497788969914637, 483.5573905765655809, 16.95518130045146776 ) ) ;
#3970=CARTESIAN_POINT ( 'NONE',  ( -38.86787825240671168, 223.9102039777116318, -13.30301237467029019 ) ) ;
#3971=LINE ( 'NONE', #17395, #10841 ) ;
#3972=CARTESIAN_POINT ( 'NONE',  ( -40.53162694259545873, 514.1198905683720568, -11.84573899990672707 ) ) ;
#3974=CARTESIAN_POINT ( 'NONE',  ( -45.43829269268869098, 253.5573905683720284, -3.332260488124726194 ) ) ;
#3975=CARTESIAN_POINT ( 'NONE',  ( -14.48388495494899786, 341.3073905683720568, -9.489475012073736337 ) ) ;
#3976=EDGE_CURVE ( 'NONE', #19193, #18799, #11998, .T. ) ;
#3977=CARTESIAN_POINT ( 'NONE',  ( -48.68588794268870856, 351.9948905765656377, 0.000000000000000000 ) ) ;
#3978=CARTESIAN_POINT ( 'NONE',  ( -28.68588794268871922, 401.3698905683720000, -16.75240474999999307 ) ) ;
#3979=ADVANCED_FACE ( 'NONE', ( #10362 ), #18661, .T. ) ;
#3981=CARTESIAN_POINT ( 'NONE',  ( -48.68588794268870856, 386.9323905601785327, -3.978247347593158345 ) ) ;
#3985=CARTESIAN_POINT ( 'NONE',  ( -32.01814843081346851, 507.5573905683720568, 16.75240474999999307 ) ) ;
#3986=CARTESIAN_POINT ( 'NONE',  ( -8.685887942688539809, 317.3073905765655809, -3.978247347592740013 ) ) ;
#3988=CARTESIAN_POINT ( 'NONE',  ( -35.09675569278793716, 303.4948905683720568, -15.47720386886985544 ) ) ;
#3989=VERTEX_POINT ( 'NONE', #110 ) ;
#3990=CARTESIAN_POINT ( 'NONE',  ( -19.19641293061498288, 340.4323905683720000, -14.20200298773971603 ) ) ;
#3991=CARTESIAN_POINT ( 'NONE',  ( -22.27502019258948707, 350.7448905683720568, -15.47720386886985544 ) ) ;
#3992=CARTESIAN_POINT ( 'NONE',  ( -24.70764059509555466, 289.1823905765656377, -19.99999999999999289 ) ) ;
#3993=CARTESIAN_POINT ( 'NONE',  ( -8.685887942688738761, 496.9948905765655809, -2.449293598294705724E-15 ) ) ;
#3994=CARTESIAN_POINT ( 'NONE',  ( -44.16309181155855157, 244.4948905683720284, 6.410867750099241924 ) ) ;
#3995=CARTESIAN_POINT ( 'NONE',  ( -42.82802356641964536, 225.9948905601784759, -14.14213562373094746 ) ) ;
#3996=CARTESIAN_POINT ( 'NONE',  ( -45.43829269268871229, 395.6823905683719431, 3.332260488124734632 ) ) ;
#3998=CARTESIAN_POINT ( 'NONE',  ( -17.35679799567829207, 333.8073905601784759, -16.95518130045146421 ) ) ;
#3999=CARTESIAN_POINT ( 'NONE',  ( -17.35679799567830628, 448.5573905765656946, -16.95518130045146421 ) ) ;
#4001=CARTESIAN_POINT ( 'NONE',  ( -31.26501780185373391, 205.1437886375728965, -5.000000000000001776 ) ) ;
#4002=CARTESIAN_POINT ( 'NONE',  ( -42.88789093042842637, 314.4323905683720000, -9.489475012073736337 ) ) ;
#4003=CARTESIAN_POINT ( 'NONE',  ( -45.43829269268871940, 454.1823905683720568, 3.332260488124734632 ) ) ;
#4005=CARTESIAN_POINT ( 'NONE',  ( -36.33955658999052218, 475.3698905601784759, -18.47759065022572855 ) ) ;
#4006=CARTESIAN_POINT ( 'NONE',  ( -28.68588794268870146, 286.3698905683720568, 16.75240474999999307 ) ) ;
#4008=CARTESIAN_POINT ( 'NONE',  ( -40.01497788969913216, 338.8073905601784190, 16.95518130045146776 ) ) ;
#4009=ORIENTED_EDGE ( 'NONE', *, *, #2400, .F. ) ;
#4012=CARTESIAN_POINT ( 'NONE',  ( -47.16347859291444422, 347.8698905601784759, 7.653668647301805628 ) ) ;
#4013=CARTESIAN_POINT ( 'NONE',  ( -16.84014894278198327, 310.1198905683720000, -11.84573899990672707 ) ) ;
#4014=ADVANCED_FACE ( 'NONE', ( #2050 ), #8624, .T. ) ;
#4015=CARTESIAN_POINT ( 'NONE',  ( -40.53162694259543741, 386.6198905683720568, 11.84573899990672885 ) ) ;
#4017=CARTESIAN_POINT ( 'NONE',  ( -28.68588794268870856, 294.7448905601784759, -19.99999999999999289 ) ) ;
#4018=CARTESIAN_POINT ( 'NONE',  ( -21.03221929538694468, 528.8698905765656946, -18.47759065022572855 ) ) ;
#4019=CARTESIAN_POINT ( 'NONE',  ( -11.93348319268872615, 408.8698905683720568, -2.051577885510841163E-15 ) ) ;
#4020=CARTESIAN_POINT ( 'NONE',  ( -44.16309181155855867, 244.7448905683720000, -6.410867750099231266 ) ) ;
#4021=CARTESIAN_POINT ( 'NONE',  ( -40.53162694259544452, 402.6198905683720568, -11.84573899990672707 ) ) ;
#4024=CARTESIAN_POINT ( 'NONE',  ( -48.68588794268870856, 341.9948905765656377, 0.000000000000000000 ) ) ;
#4026=CARTESIAN_POINT ( 'NONE',  ( -45.43829269268870519, 313.8698905683720000, 0.000000000000000000 ) ) ;
#4028=CARTESIAN_POINT ( 'NONE',  ( -45.43829269268871940, 475.6823905683720000, 3.332260488124734632 ) ) ;
#4030=CARTESIAN_POINT ( 'NONE',  ( -10.20829729246299422, 436.3698905765656377, 7.653668647301790529 ) ) ;
#4034=CARTESIAN_POINT ( 'NONE',  ( -25.35362745456399480, 392.5573905683720000, -16.75240474999999307 ) ) ;
#4035=LINE ( 'NONE', #17033, #17849 ) ;
#4036=CARTESIAN_POINT ( 'NONE',  ( -14.54375231895779130, 533.4948905601785327, -14.14213562373094746 ) ) ;
#4037=CARTESIAN_POINT ( 'NONE',  ( -19.19641293061497933, 337.3073905683720568, 14.20200298773971426 ) ) ;
#4040=CARTESIAN_POINT ( 'NONE',  ( -16.84014894278200813, 510.1198905683720568, -11.84573899990672707 ) ) ;
#4047=CARTESIAN_POINT ( 'NONE',  ( -35.09675569278796559, 455.7448905683720568, 15.47720386886985366 ) ) ;
#4049=CARTESIAN_POINT ( 'NONE',  ( -16.84014894278200103, 477.6198905683720000, 11.84573899990672530 ) ) ;
#4050=CARTESIAN_POINT ( 'NONE',  ( -17.35679799567827786, 245.4323905765656377, 16.95518130045146421 ) ) ;
#4052=CARTESIAN_POINT ( 'NONE',  ( -21.03221929538691626, 405.1198905765656377, 18.47759065022572500 ) ) ;
#4053=CARTESIAN_POINT ( 'NONE',  ( -40.01497788969914637, 473.5573905765655809, 16.95518130045146776 ) ) ;
#4055=CARTESIAN_POINT ( 'NONE',  ( -8.685887942688719221, 332.2448905601784759, -2.449293598294705724E-15 ) ) ;
#4058=CARTESIAN_POINT ( 'NONE',  ( -28.68588794268870501, 259.4948905765655809, -19.99999999999999289 ) ) ;
#4059=CARTESIAN_POINT ( 'NONE',  ( -28.68588794268869790, 239.7448905601785043, 19.99999999999999289 ) ) ;
#4062=CARTESIAN_POINT ( 'NONE',  ( -42.88789093042842637, 274.4323905683720568, -9.489475012073736337 ) ) ;
#4064=CARTESIAN_POINT ( 'NONE',  ( -8.685887942688708563, 251.9323905601784475, 3.978247347593161010 ) ) ;
#4065=CARTESIAN_POINT ( 'NONE',  ( -36.33955658999052218, 403.8698905765656377, 18.47759065022572500 ) ) ;
#4066=CARTESIAN_POINT ( 'NONE',  ( -22.27502019258949773, 452.2448905683720000, -15.47720386886985544 ) ) ;
#4067=CARTESIAN_POINT ( 'NONE',  ( -11.73070664223724613, 327.9323905765656377, -11.32908994701042538 ) ) ;
#4068=CARTESIAN_POINT ( 'NONE',  ( -32.01814843081343298, 273.1823905683720568, -16.75240474999999307 ) ) ;
#4071=CARTESIAN_POINT ( 'NONE',  ( -22.27502019258949773, 482.2448905683720568, -15.47720386886985544 ) ) ;
#4072=ORIENTED_EDGE ( 'NONE', *, *, #4537, .F. ) ;
#4073=DIRECTION ( 'NONE',  ( -1.191790137725560488E-16, 1.000000000000000000, -0.000000000000000000 ) ) ;
#4074=CARTESIAN_POINT ( 'NONE',  ( -45.43829269268869098, 244.1823905683720568, 3.332260488124734632 ) ) ;
#4077=CARTESIAN_POINT ( 'NONE',  ( -8.685887942688717445, 306.9948905765655809, -2.449293598294705724E-15 ) ) ;
#4078=CARTESIAN_POINT ( 'NONE',  ( -47.16347859291445843, 461.3698905765656377, -7.653668647301793193 ) ) ;
#4079=CARTESIAN_POINT ( 'NONE',  ( -47.16347859291444422, 387.8698905601784759, 7.653668647301805628 ) ) ;
#4080=CARTESIAN_POINT ( 'NONE',  ( -32.66413529028188378, 455.0573905601785896, -19.99999999999999289 ) ) ;
#4081=CARTESIAN_POINT ( 'NONE',  ( -35.09675569278793006, 233.4948905683720284, -15.47720386886985544 ) ) ;
#4082=CARTESIAN_POINT ( 'NONE',  ( -32.01814843081346851, 513.1823905683720568, -16.75240474999999307 ) ) ;
#4084=CARTESIAN_POINT ( 'NONE',  ( -45.43829269268869808, 253.8698905683720000, 0.000000000000000000 ) ) ;
#4085=CARTESIAN_POINT ( 'NONE',  ( -14.48388495494899608, 339.4323905683720000, 9.489475012073732785 ) ) ;
#4086=CARTESIAN_POINT ( 'NONE',  ( -40.01497788969912506, 318.8073905601784759, 16.95518130045146776 ) ) ;
#4087=CARTESIAN_POINT ( 'NONE',  ( -32.66413529028186957, 359.4323905601785327, 19.99999999999999289 ) ) ;
#4088=CARTESIAN_POINT ( 'NONE',  ( -16.84014894278199392, 380.1198905683720568, -11.84573899990672707 ) ) ;
#4090=CARTESIAN_POINT ( 'NONE',  ( -11.73070664223725323, 393.1823905601785896, -11.32908994701042715 ) ) ;
#4092=DIRECTION ( 'NONE',  ( -1.191790137725560488E-16, 1.000000000000000000, -0.000000000000000000 ) ) ;
#4095=CARTESIAN_POINT ( 'NONE',  ( -11.93348319268873858, 510.0573905683720000, 3.332260488124728415 ) ) ;
#4097=ORIENTED_EDGE ( 'NONE', *, *, #8549, .T. ) ;
#4098=CARTESIAN_POINT ( 'NONE',  ( -11.93348319268871549, 310.3698905683720568, -2.051577885510841163E-15 ) ) ;
#4100=CARTESIAN_POINT ( 'NONE',  ( -14.48388495494899608, 337.9323905683720568, 9.489475012073732785 ) ) ;
#4101=CARTESIAN_POINT ( 'NONE',  ( -38.17536295476244845, 355.4323905683720568, 14.20200298773971781 ) ) ;
#4102=CARTESIAN_POINT ( 'NONE',  ( -17.35679799567829207, 288.5573905765656377, -16.95518130045146421 ) ) ;
#4103=CARTESIAN_POINT ( 'NONE',  ( -17.35679799567831338, 498.5573905765655809, -16.95518130045146421 ) ) ;
#4104=CARTESIAN_POINT ( 'NONE',  ( -35.09675569278793716, 245.7448905683720000, 15.47720386886985366 ) ) ;
#4105=CARTESIAN_POINT ( 'NONE',  ( -43.63022347157594538, 200.3131325479159273, 1.300740588846954759 ) ) ;
#4106=CARTESIAN_POINT ( 'NONE',  ( -42.88789093042844058, 404.4323905683721136, -9.489475012073736337 ) ) ;
#4109=CARTESIAN_POINT ( 'NONE',  ( -28.68588794268872988, 504.4948905765655809, 19.99999999999999289 ) ) ;
#4110=CARTESIAN_POINT ( 'NONE',  ( -32.66413529028185536, 245.0573905601785043, -19.99999999999999289 ) ) ;
#4111=CARTESIAN_POINT ( 'NONE',  ( -32.01814843081346140, 461.6823905683720568, -16.75240474999999307 ) ) ;
#4113=ORIENTED_EDGE ( 'NONE', *, *, #7561, .T. ) ;
#4114=CARTESIAN_POINT ( 'NONE',  ( -17.35679799567830273, 450.6823905601785327, 16.95518130045146421 ) ) ;
#4120=CARTESIAN_POINT ( 'NONE',  ( -28.68588794268871212, 334.7448905601784759, -19.99999999999999289 ) ) ;
#4121=CARTESIAN_POINT ( 'NONE',  ( -14.48388495494899075, 307.9323905683720000, 9.489475012073732785 ) ) ;
#4124=CARTESIAN_POINT ( 'NONE',  ( -32.01814843081344719, 357.5573905683720000, 16.75240474999999307 ) ) ;
#4125=CARTESIAN_POINT ( 'NONE',  ( -21.03221929538691626, 294.1198905601785327, -18.47759065022572855 ) ) ;
#4126=CARTESIAN_POINT ( 'NONE',  ( -45.64106924314020119, 531.0573905765656946, -11.32908994701042715 ) ) ;
#4127=CARTESIAN_POINT ( 'NONE',  ( -40.53162694259544452, 405.1198905683720000, 11.84573899990672885 ) ) ;
#4128=CARTESIAN_POINT ( 'NONE',  ( -19.19641293061497223, 231.9323905683720000, -14.20200298773971603 ) ) ;
#4129=CARTESIAN_POINT ( 'NONE',  ( -38.17536295476246266, 412.3073905683720000, -14.20200298773971426 ) ) ;
#4130=CARTESIAN_POINT ( 'NONE',  ( -47.16347859291444422, 352.6198905765656377, 7.653668647301805628 ) ) ;
#4132=CARTESIAN_POINT ( 'NONE',  ( -28.68588794268870856, 311.3698905683720568, -16.75240474999999307 ) ) ;
#4133=CARTESIAN_POINT ( 'NONE',  ( -32.01814843081346140, 463.1823905683720000, -16.75240474999999307 ) ) ;
#4134=CARTESIAN_POINT ( 'NONE',  ( -32.66413529028189089, 514.1823905765656946, 19.99999999999999289 ) ) ;
#4137=EDGE_CURVE ( 'NONE', #6325, #21365, #20888, .T. ) ;
#4138=CARTESIAN_POINT ( 'NONE',  ( -25.35362745456398059, 368.1823905683721136, 16.75240474999998952 ) ) ;
#4140=CARTESIAN_POINT ( 'NONE',  ( -32.66413529028189799, 509.4323905601784190, 19.99999999999999289 ) ) ;
#4141=CARTESIAN_POINT ( 'NONE',  ( -45.43829269268871229, 333.8698905683720000, 0.000000000000000000 ) ) ;
#4143=CARTESIAN_POINT ( 'NONE',  ( -42.88789093042845479, 512.9323905683719431, -9.489475012073736337 ) ) ;
#4145=CARTESIAN_POINT ( 'NONE',  ( -11.73070664223724613, 351.3073905601785327, 11.32908994701042005 ) ) ;
#4146=EDGE_CURVE ( 'NONE', #17095, #3367, #6026, .T. ) ;
#4149=CARTESIAN_POINT ( 'NONE',  ( -16.84014894278199748, 421.6198905683720000, -11.84573899990672707 ) ) ;
#4151=CARTESIAN_POINT ( 'NONE',  ( -28.68588794268874054, 573.2448905601785327, 0.000000000000000000 ) ) ;
#4152=CARTESIAN_POINT ( 'NONE',  ( -13.20868407381887444, 469.4948905683720000, -6.410867750099233042 ) ) ;
#4154=CARTESIAN_POINT ( 'NONE',  ( -42.88789093042844769, 462.9323905683720568, -9.489475012073734561 ) ) ;
#4156=CARTESIAN_POINT ( 'NONE',  ( -10.20829729246299067, 396.3698905765656377, 7.653668647301790529 ) ) ;
#4157=DIRECTION ( 'NONE',  ( -1.191790137725560488E-16, 1.000000000000000000, -0.000000000000000000 ) ) ;
#4158=CARTESIAN_POINT ( 'NONE',  ( -45.64106924314017277, 298.1823905601785327, 11.32908994701042538 ) ) ;
#4166=CARTESIAN_POINT ( 'NONE',  ( -40.53162694259543031, 274.1198905683720568, -11.84573899990672707 ) ) ;
#4167=CARTESIAN_POINT ( 'NONE',  ( -36.33955658999049376, 245.3698905601785043, -18.47759065022572855 ) ) ;
#4168=CARTESIAN_POINT ( 'NONE',  ( -45.64106924314018698, 402.9323905765656946, 11.32908994701042538 ) ) ;
#4169=CARTESIAN_POINT ( 'NONE',  ( -28.68588794268871922, 417.8698905683720568, 16.75240474999999307 ) ) ;
#4170=CARTESIAN_POINT ( 'NONE',  ( -42.82802356641966668, 400.7448905765656377, -14.14213562373094746 ) ) ;
#4172=CARTESIAN_POINT ( 'NONE',  ( -28.68588794268870501, 262.8698905683720000, -16.75240474999999307 ) ) ;
#4178=CARTESIAN_POINT ( 'NONE',  ( -44.16309181155858710, 474.7448905683720568, -6.410867750099231266 ) ) ;
#4181=VERTEX_POINT ( 'NONE', #7646 ) ;
#4182=CARTESIAN_POINT ( 'NONE',  ( -32.66413529028189089, 524.1823905765656946, 19.99999999999999289 ) ) ;
#4183=CARTESIAN_POINT ( 'NONE',  ( -16.84014894278197261, 237.6198905683720284, 11.84573899990672530 ) ) ;
#4186=CARTESIAN_POINT ( 'NONE',  ( -11.93348319268874214, 528.5573905683720568, 3.332260488124728859 ) ) ;
#4188=CARTESIAN_POINT ( 'NONE',  ( -17.35679799567830983, 468.5573905765655809, -16.95518130045146421 ) ) ;
#4193=CARTESIAN_POINT ( 'NONE',  ( -11.93348319268873858, 510.3698905683720000, -2.051577885510841163E-15 ) ) ;
#4195=CARTESIAN_POINT ( 'NONE',  ( -11.93348319268870839, 238.5573905683720000, 3.332260488124728415 ) ) ;
#4196=CARTESIAN_POINT ( 'NONE',  ( -28.68588794268870856, 337.8698905683720000, 16.75240474999999307 ) ) ;
#4198=CARTESIAN_POINT ( 'NONE',  ( -11.73070664223725856, 471.3073905601784759, 11.32908994701042005 ) ) ;
#4199=CARTESIAN_POINT ( 'NONE',  ( -8.685887942688985675, 361.9323905601784759, 3.978247347593800054 ) ) ;
#4203=CARTESIAN_POINT ( 'NONE',  ( -35.09675569278795138, 391.9948905683720568, -15.47720386886985544 ) ) ;
#4205=CARTESIAN_POINT ( 'NONE',  ( -14.54375231895776288, 325.7448905765655809, 14.14213562373094568 ) ) ;
#4206=SHAPE_REPRESENTATION ( 'Coarse Pitch Steep Screw Shaft', ( #12794 ), #4502 ) ;
#4207=CARTESIAN_POINT ( 'NONE',  ( -28.68588794268871922, 394.7448905601784759, -19.99999999999999289 ) ) ;
#4208=VERTEX_POINT ( 'NONE', #10780 ) ;
#4212=CARTESIAN_POINT ( 'NONE',  ( -14.48388495494901740, 501.3073905683720568, -9.489475012073736337 ) ) ;
#4213=CARTESIAN_POINT ( 'NONE',  ( -32.66413529028186247, 294.1823905765655809, 19.99999999999999289 ) ) ;
#4214=ORIENTED_EDGE ( 'NONE', *, *, #12793, .T. ) ;
#4216=CARTESIAN_POINT ( 'NONE',  ( -35.09675569278793716, 313.4948905683720000, -15.47720386886985544 ) ) ;
#4217=VERTEX_POINT ( 'NONE', #9271 ) ;
#4218=CARTESIAN_POINT ( 'NONE',  ( -38.17536295476245556, 342.3073905683721136, -14.20200298773971426 ) ) ;
#4220=CARTESIAN_POINT ( 'NONE',  ( -22.27502019258948351, 340.7448905683720568, -15.47720386886985544 ) ) ;
#4221=CARTESIAN_POINT ( 'NONE',  ( -14.54375231895775578, 275.7448905765656377, 14.14213562373094568 ) ) ;
#4222=CARTESIAN_POINT ( 'NONE',  ( -8.685887942688742314, 573.2448905601785327, 2.449293598294706119E-15 ) ) ;
#4223=CARTESIAN_POINT ( 'NONE',  ( -13.20868407381884779, 249.4948905683720284, -6.410867750099233042 ) ) ;
#4226=CARTESIAN_POINT ( 'NONE',  ( -28.68588794268871567, 397.8698905683720000, 16.75240474999999307 ) ) ;
#4230=CARTESIAN_POINT ( 'NONE',  ( -11.93348319268873148, 448.8698905683720000, -2.051577885510841163E-15 ) ) ;
#4233=CARTESIAN_POINT ( 'NONE',  ( -10.20829729246299600, 451.6198905601784759, 7.653668647301790529 ) ) ;
#4234=ORIENTED_EDGE ( 'NONE', *, *, #16908, .T. ) ;
#4238=CARTESIAN_POINT ( 'NONE',  ( -47.16347859291443712, 316.6198905601784759, -7.653668647301793193 ) ) ;
#4239=CARTESIAN_POINT ( 'NONE',  ( -44.16309181155855867, 294.4948905683720000, 6.410867750099241924 ) ) ;
#4240=CARTESIAN_POINT ( 'NONE',  ( -38.17536295476244845, 356.9323905683720000, 14.20200298773971781 ) ) ;
#4243=CARTESIAN_POINT ( 'NONE',  ( -38.17536295476245556, 405.4323905683721136, 14.20200298773971781 ) ) ;
#4244=CARTESIAN_POINT ( 'NONE',  ( -42.88789093042841927, 246.3073905683720284, 9.489475012073736337 ) ) ;
#4246=CARTESIAN_POINT ( 'NONE',  ( -22.27502019258949062, 400.7448905683720568, -15.47720386886985544 ) ) ;
#4247=CARTESIAN_POINT ( 'NONE',  ( -36.33955658999051508, 343.8698905765656377, 18.47759065022572500 ) ) ;
#4248=CARTESIAN_POINT ( 'NONE',  ( -45.64106924314017277, 326.3073905601784759, -11.32908994701042538 ) ) ;
#4249=CARTESIAN_POINT ( 'NONE',  ( -11.93348319268871371, 298.8698905683720000, -2.051577885510841163E-15 ) ) ;
#4250=CARTESIAN_POINT ( 'NONE',  ( -28.68588794268872277, 457.8698905683720000, 16.75240474999999307 ) ) ;
#4251=CARTESIAN_POINT ( 'NONE',  ( -28.68588794268872988, 514.4948905765655809, 19.99999999999999289 ) ) ;
#4255=CARTESIAN_POINT ( 'NONE',  ( -14.48388495494899963, 369.4323905683720000, 9.489475012073732785 ) ) ;
#4256=CARTESIAN_POINT ( 'NONE',  ( -11.93348319268873858, 508.5573905683720000, 3.332260488124728415 ) ) ;
#4257=CARTESIAN_POINT ( 'NONE',  ( -40.01497788969916058, 515.6823905601784190, -16.95518130045146421 ) ) ;
#4258=CARTESIAN_POINT ( 'NONE',  ( -32.01814843081344719, 351.6823905683720000, -16.75240474999999307 ) ) ;
#4260=CARTESIAN_POINT ( 'NONE',  ( -14.48388495494901562, 497.9323905683720568, 9.489475012073732785 ) ) ;
#4263=CARTESIAN_POINT ( 'NONE',  ( -40.01497788969912506, 313.5573905765655809, 16.95518130045146776 ) ) ;
#4264=CARTESIAN_POINT ( 'NONE',  ( -14.48388495494900674, 421.3073905683720000, -9.489475012073734561 ) ) ;
#4266=CARTESIAN_POINT ( 'NONE',  ( -11.73070664223726922, 517.9323905765655809, -11.32908994701042538 ) ) ;
#4267=CARTESIAN_POINT ( 'NONE',  ( -19.19641293061499709, 470.4323905683719431, -14.20200298773971603 ) ) ;
#4269=CARTESIAN_POINT ( 'NONE',  ( -45.43829269268872650, 463.8698905683720000, 0.000000000000000000 ) ) ;
#4270=CARTESIAN_POINT ( 'NONE',  ( -48.68588794268873698, 573.2448905601785327, 0.000000000000000000 ) ) ;
#4272=CARTESIAN_POINT ( 'NONE',  ( -48.68588794268871567, 401.6823905765655809, -3.978247347593158345 ) ) ;
#4281=CARTESIAN_POINT ( 'NONE',  ( -45.60737594483680368, 223.9102039777115749, 2.249240700863258002 ) ) ;
#4282=CARTESIAN_POINT ( 'NONE',  ( -38.17536295476244135, 276.9323905683720000, 14.20200298773971781 ) ) ;
#4284=CARTESIAN_POINT ( 'NONE',  ( -36.33955658999050087, 249.1198905601784759, 18.47759065022572500 ) ) ;
#4286=CARTESIAN_POINT ( 'NONE',  ( -14.48388495494900496, 419.4323905683720568, 9.489475012073732785 ) ) ;
#4288=CARTESIAN_POINT ( 'NONE',  ( -28.68588794268869790, 257.8698905683720000, 16.75240474999999307 ) ) ;
#4292=CARTESIAN_POINT ( 'NONE',  ( -38.17536295476246266, 486.9323905683720568, 14.20200298773971781 ) ) ;
#4294=CARTESIAN_POINT ( 'NONE',  ( -8.685887942688742314, 573.2448905601785327, 2.449293598294706119E-15 ) ) ;
#4295=CARTESIAN_POINT ( 'NONE',  ( -28.68588794268869790, 246.3698905683720000, 16.75240474999999307 ) ) ;
#4297=CARTESIAN_POINT ( 'NONE',  ( -42.88789093042845479, 524.8073905683720568, 9.489475012073734561 ) ) ;
#4299=EDGE_CURVE ( 'NONE', #6189, #2640, #2625, .T. ) ;
#4300=CARTESIAN_POINT ( 'NONE',  ( -11.73070664223726212, 457.9323905765655809, -11.32908994701042715 ) ) ;
#4301=CARTESIAN_POINT ( 'NONE',  ( -32.66413529028186957, 349.4323905601785327, 19.99999999999999289 ) ) ;
#4302=FACE_OUTER_BOUND ( 'NONE', #2059, .T. ) ;
#4305=CARTESIAN_POINT ( 'NONE',  ( -28.68588794268872988, 507.8698905683720568, 16.75240474999999307 ) ) ;
#4307=CARTESIAN_POINT ( 'NONE',  ( -40.53162694259542320, 235.1198905683720000, 11.84573899990672885 ) ) ;
#4308=CARTESIAN_POINT ( 'NONE',  ( -19.19641293061498288, 331.9323905683720000, -14.20200298773971603 ) ) ;
#4310=CARTESIAN_POINT ( 'NONE',  ( -11.73070664223724080, 321.3073905601784190, 11.32908994701042005 ) ) ;
#4311=CARTESIAN_POINT ( 'NONE',  ( -11.93348319268872260, 378.5573905683721136, 3.332260488124728415 ) ) ;
#4313=CARTESIAN_POINT ( 'NONE',  ( -48.68588794268870856, 377.2448905601784759, 0.000000000000000000 ) ) ;
#4316=ORIENTED_EDGE ( 'NONE', *, *, #11546, .F. ) ;
#4317=VERTEX_POINT ( 'NONE', #11215 ) ;
#4318=CARTESIAN_POINT ( 'NONE',  ( -45.43829269268872650, 515.6823905683720568, 3.332260488124734632 ) ) ;
#4319=CARTESIAN_POINT ( 'NONE',  ( -21.03221929538690205, 295.1198905765656377, 18.47759065022572500 ) ) ;
#4321=CARTESIAN_POINT ( 'NONE',  ( -14.48388495494899075, 309.4323905683720568, 9.489475012073731008 ) ) ;
#4322=VERTEX_POINT ( 'NONE', #6233 ) ;
#4323=CARTESIAN_POINT ( 'NONE',  ( -40.53162694259543031, 325.1198905683720568, 11.84573899990672885 ) ) ;
#4324=CARTESIAN_POINT ( 'NONE',  ( -16.84014894278198682, 340.1198905683720568, -11.84573899990672707 ) ) ;
#4325=CARTESIAN_POINT ( 'NONE',  ( -10.20829729246297468, 257.6198905765656377, -7.653668647301794969 ) ) ;
#4326=CARTESIAN_POINT ( 'NONE',  ( -14.54375231895777354, 393.4948905601784190, -14.14213562373094746 ) ) ;
#4327=CARTESIAN_POINT ( 'NONE',  ( -28.68588794268870146, 251.3698905683720000, -16.75240474999999307 ) ) ;
#4328=CARTESIAN_POINT ( 'NONE',  ( -28.68588794268869790, 224.7448905601784759, -19.99999999999999289 ) ) ;
#4329=CARTESIAN_POINT ( 'NONE',  ( -40.53162694259544452, 406.6198905683720568, 11.84573899990672885 ) ) ;
#4330=CARTESIAN_POINT ( 'NONE',  ( -28.68588794268871212, 334.7448905601784759, -19.99999999999999289 ) ) ;
#4333=( BOUNDED_CURVE ( )  B_SPLINE_CURVE ( 2, ( #7930, #12931, #20719, #4697, #176, #20059, #8366, #1465, #16501, #13466, #3406, #3615, #5234, #6415, #19951, #8141, #11511 ),
 .UNSPECIFIED., .F., .T. ) 
 B_SPLINE_CURVE_WITH_KNOTS ( ( 3, 2, 2, 2, 2, 2, 2, 2, 3 ),
 ( 0.3593750000000001110, 0.3613281250000001110, 0.3632812500000001110, 0.3652343750000001110, 0.3671875000000001110, 0.3691406250000001665, 0.3710937500000001665, 0.3730468750000001665, 0.3750000000000001665 ),
 .UNSPECIFIED. ) 
 CURVE ( )  GEOMETRIC_REPRESENTATION_ITEM ( )  RATIONAL_B_SPLINE_CURVE ( ( 0.9999999999999988898, 0.9807852804032315408, 1.000000000000000000, 0.9807852804032304306, 1.000000000000000000, 0.9807852804032304306, 1.000000000000000000, 0.9807852804032304306, 1.000000000000000000, 0.9807852804032304306, 1.000000000000000000, 0.9807852804032304306, 1.000000000000000000, 0.9807852804032304306, 1.000000000000000000, 0.9807852804032287652, 1.000000000000001554 ) ) 
 REPRESENTATION_ITEM ( '' )  );
#4334=CARTESIAN_POINT ( 'NONE',  ( -48.68588794268869435, 247.2448905601785043, 0.000000000000000000 ) ) ;
#4336=CARTESIAN_POINT ( 'NONE',  ( -11.93348319268872970, 438.5573905683720000, 3.332260488124728415 ) ) ;
#4338=CARTESIAN_POINT ( 'NONE',  ( -8.685887942688729879, 442.5573905601784759, -3.978247347593165895 ) ) ;
#4341=PRODUCT_DEFINITION ( 'UNKNOWN', '', #13173, #2078 ) ;
#4344=CARTESIAN_POINT ( 'NONE',  ( -36.33955658999050797, 329.1198905601784759, 18.47759065022572500 ) ) ;
#4345=CARTESIAN_POINT ( 'NONE',  ( -25.35362745456399125, 372.5573905683720568, -16.75240474999999307 ) ) ;
#4347=CARTESIAN_POINT ( 'NONE',  ( -45.64106924314020119, 511.0573905765656946, -11.32908994701042715 ) ) ;
#4348=CARTESIAN_POINT ( 'NONE',  ( -13.20868407381886200, 388.2448905683720000, 6.410867750099229490 ) ) ;
#4349=CARTESIAN_POINT ( 'NONE',  ( -16.84014894278197261, 249.1198905683720284, 11.84573899990672530 ) ) ;
#4350=CARTESIAN_POINT ( 'NONE',  ( -44.16309181155857289, 404.4948905683720000, 6.410867750099241924 ) ) ;
#4351=CARTESIAN_POINT ( 'NONE',  ( -10.20829729246298356, 336.3698905765656377, 7.653668647301790529 ) ) ;
#4353=CARTESIAN_POINT ( 'NONE',  ( -22.27502019258946930, 306.9948905683720568, 15.47720386886985189 ) ) ;
#4354=CARTESIAN_POINT ( 'NONE',  ( -40.53162694259545162, 466.6198905683720000, 11.84573899990672885 ) ) ;
#4357=CARTESIAN_POINT ( 'NONE',  ( -11.93348319268872082, 360.3698905683720568, -2.051577885510841163E-15 ) ) ;
#4358=CARTESIAN_POINT ( 'NONE',  ( -16.84014894278200813, 510.1198905683720568, -11.84573899990672707 ) ) ;
#4360=CARTESIAN_POINT ( 'NONE',  ( -45.64106924314020119, 498.1823905601784759, 11.32908994701042715 ) ) ;
#4361=CARTESIAN_POINT ( 'NONE',  ( -13.20868407381885312, 318.2448905683720000, 6.410867750099229490 ) ) ;
#4364=CARTESIAN_POINT ( 'NONE',  ( -42.88789093042844769, 494.8073905683720000, 9.489475012073736337 ) ) ;
#4365=ORIENTED_EDGE ( 'NONE', *, *, #520, .F. ) ;
#4368=CARTESIAN_POINT ( 'NONE',  ( -44.16309181155857999, 424.7448905683720000, -6.410867750099231266 ) ) ;
#4369=CARTESIAN_POINT ( 'NONE',  ( -8.685887942688735208, 472.2448905601784759, -2.449293598294705724E-15 ) ) ;
#4371=CARTESIAN_POINT ( 'NONE',  ( -13.20868407381887089, 458.2448905683720568, 6.410867750099229490 ) ) ;
#4373=CARTESIAN_POINT ( 'NONE',  ( -40.53162694259545162, 465.1198905683720568, 11.84573899990672885 ) ) ;
#4375=CARTESIAN_POINT ( 'NONE',  ( -11.73070664223725501, 407.9323905765656377, -11.32908994701042715 ) ) ;
#4380=ADVANCED_FACE ( 'NONE', ( #13492 ), #8391, .T. ) ;
#4383=CARTESIAN_POINT ( 'NONE',  ( -45.64106924314016567, 256.3073905601784759, -11.32908994701042538 ) ) ;
#4385=CARTESIAN_POINT ( 'NONE',  ( -45.46835912530129065, 223.9102039777117170, 4.966902868867238752 ) ) ;
#4386=CARTESIAN_POINT ( 'NONE',  ( -40.01497788969911795, 238.8073905601784759, 16.95518130045146776 ) ) ;
#4389=CARTESIAN_POINT ( 'NONE',  ( -45.43829269268871229, 435.6823905683720568, 3.332260488124734632 ) ) ;
#4390=CARTESIAN_POINT ( 'NONE',  ( -45.64106924314017988, 386.3073905601785327, -11.32908994701042538 ) ) ;
#4391=CARTESIAN_POINT ( 'NONE',  ( -42.88789093042841927, 256.3073905683720568, 9.489475012073736337 ) ) ;
#4394=DIRECTION ( 'NONE',  ( -1.000000000000000000, 0.000000000000000000, 0.000000000000000000 ) ) ;
#4396=CARTESIAN_POINT ( 'NONE',  ( -28.68588794268872988, 462.8698905683720000, -16.75240474999999307 ) ) ;
#4397=VECTOR ( 'NONE', #9456, 1000.000000000000000 ) ;
#4400=CARTESIAN_POINT ( 'NONE',  ( -28.68588794268870146, 231.3698905683720284, -16.75240474999999307 ) ) ;
#4402=CARTESIAN_POINT ( 'NONE',  ( -16.84014894278200458, 517.6198905683719431, 11.84573899990672530 ) ) ;
#4405=AXIS2_PLACEMENT_3D ( 'NONE', #17423, #5835, #10696 ) ;
#4406=CARTESIAN_POINT ( 'NONE',  ( -24.70764059509557242, 459.1823905765656377, -19.99999999999999289 ) ) ;
#4408=CARTESIAN_POINT ( 'NONE',  ( -42.82802356641965957, 348.4948905601785327, 14.14213562373094923 ) ) ;
#4410=CARTESIAN_POINT ( 'NONE',  ( -23.03786159879532036, 223.9102039777118023, -18.55174335541752839 ) ) ;
#4411=DIRECTION ( 'NONE',  ( -1.191790137725560488E-16, 1.000000000000000000, -0.000000000000000000 ) ) ;
#4412=CARTESIAN_POINT ( 'NONE',  ( -40.53162694259542320, 232.6198905683720000, -11.84573899990672707 ) ) ;
#4413=CARTESIAN_POINT ( 'NONE',  ( -14.48388495494899431, 329.4323905683720568, 9.489475012073732785 ) ) ;
#4414=CARTESIAN_POINT ( 'NONE',  ( -8.685887942688893304, 321.9323905601784190, 3.978247347593586447 ) ) ;
#4416=CARTESIAN_POINT ( 'NONE',  ( -32.01814843081344009, 303.1823905683720000, -16.75240474999999307 ) ) ;
#4418=CARTESIAN_POINT ( 'NONE',  ( -45.43829269268870519, 383.5573905683720000, -3.332260488124726194 ) ) ;
#4419=CARTESIAN_POINT ( 'NONE',  ( -19.19641293061500420, 521.9323905683720568, -14.20200298773971603 ) ) ;
#4420=CARTESIAN_POINT ( 'NONE',  ( -11.73070664223724968, 381.3073905601784759, 11.32908994701042005 ) ) ;
#4421=CARTESIAN_POINT ( 'NONE',  ( -24.70764059509556176, 404.4323905601785327, -19.99999999999999289 ) ) ;
#4424=CARTESIAN_POINT ( 'NONE',  ( -38.17536295476246977, 506.9323905683720568, 14.20200298773971781 ) ) ;
#4425=CARTESIAN_POINT ( 'NONE',  ( -24.70764059509554045, 294.8073905765655809, 19.99999999999998934 ) ) ;
#4428=CARTESIAN_POINT ( 'NONE',  ( -14.48388495494899253, 301.3073905683720000, -9.489475012073734561 ) ) ;
#4429=CARTESIAN_POINT ( 'NONE',  ( -45.43829269268869808, 324.1823905683720000, 3.332260488124734632 ) ) ;
#4430=CARTESIAN_POINT ( 'NONE',  ( -28.68588794268870501, 269.4948905765656377, -19.99999999999999289 ) ) ;
#4431=CARTESIAN_POINT ( 'NONE',  ( -21.03221929538692692, 394.1198905601784759, -18.47759065022572855 ) ) ;
#4432=CARTESIAN_POINT ( 'NONE',  ( -28.68588794268869790, 236.3698905683720568, 16.75240474999999307 ) ) ;
#4434=CARTESIAN_POINT ( 'NONE',  ( -11.93348319268872437, 390.0573905683720568, 3.332260488124728415 ) ) ;
#4439=CARTESIAN_POINT ( 'NONE',  ( -44.16309181155857289, 434.4948905683720568, 6.410867750099241924 ) ) ;
#4441=CARTESIAN_POINT ( 'NONE',  ( -21.03221929538693402, 444.1198905601784759, -18.47759065022572855 ) ) ;
#4446=CARTESIAN_POINT ( 'NONE',  ( -32.66413529028186957, 329.4323905601784759, 19.99999999999999289 ) ) ;
#4448=CARTESIAN_POINT ( 'NONE',  ( -42.88789093042843348, 364.4323905683720000, -9.489475012073734561 ) ) ;
#4450=CARTESIAN_POINT ( 'NONE',  ( -45.64106924314020119, 512.9323905765656946, 11.32908994701042715 ) ) ;
#4451=CARTESIAN_POINT ( 'NONE',  ( -25.35362745456399480, 391.0573905683720568, -16.75240474999999307 ) ) ;
#4454=CARTESIAN_POINT ( 'NONE',  ( -44.16309181155857999, 413.2448905683720568, -6.410867750099231266 ) ) ;
#4455=CARTESIAN_POINT ( 'NONE',  ( -11.73070664223724791, 327.9323905765656377, -11.32908994701042715 ) ) ;
#4457=CARTESIAN_POINT ( 'NONE',  ( -45.43829269268870519, 313.5573905683720000, -3.332260488124726638 ) ) ;
#4459=( BOUNDED_CURVE ( )  B_SPLINE_CURVE ( 2, ( #8640, #15267, #449, #7016, #8854, #5612, #20225, #12105, #552, #15475, #13846, #12000, #12220, #18590, #10364, #3986, #10577 ),
 .UNSPECIFIED., .F., .T. ) 
 B_SPLINE_CURVE_WITH_KNOTS ( ( 3, 2, 2, 2, 2, 2, 2, 2, 3 ),
 ( 0.6562500000000002220, 0.6582031250000002220, 0.6601562500000002220, 0.6621093750000002220, 0.6640625000000002220, 0.6660156250000002220, 0.6679687500000002220, 0.6699218750000002220, 0.6718750000000002220 ),
 .UNSPECIFIED. ) 
 CURVE ( )  GEOMETRIC_REPRESENTATION_ITEM ( )  RATIONAL_B_SPLINE_CURVE ( ( 0.9999999999999977796, 0.9807852804032326510, 1.000000000000000000, 0.9807852804032304306, 1.000000000000000000, 0.9807852804032304306, 1.000000000000000000, 0.9807852804032304306, 1.000000000000000000, 0.9807852804032304306, 1.000000000000000000, 0.9807852804032304306, 1.000000000000000000, 0.9807852804032304306, 1.000000000000000000, 0.9807852804032282101, 1.000000000000002220 ) ) 
 REPRESENTATION_ITEM ( '' )  );
#4460=CARTESIAN_POINT ( 'NONE',  ( -16.84014894278199748, 459.1198905683720568, 11.84573899990672530 ) ) ;
#4464=EDGE_CURVE ( 'NONE', #683, #13710, #15626, .T. ) ;
#4465=CARTESIAN_POINT ( 'NONE',  ( -32.01814843081344719, 363.1823905683720568, -16.75240474999999307 ) ) ;
#4466=CARTESIAN_POINT ( 'NONE',  ( -22.27502019258950128, 510.7448905683720000, -15.47720386886985544 ) ) ;
#4469=CARTESIAN_POINT ( 'NONE',  ( -8.685887942688738761, 512.2448905601784190, -2.449293598294705724E-15 ) ) ;
#4470=CARTESIAN_POINT ( 'NONE',  ( -35.09675569278794427, 325.7448905683720000, 15.47720386886985366 ) ) ;
#4472=EDGE_CURVE ( 'NONE', #18084, #13236, #14014, .T. ) ;
#4473=ORIENTED_EDGE ( 'NONE', *, *, #1603, .F. ) ;
#4476=DIRECTION ( 'NONE',  ( -1.191790137725560488E-16, 1.000000000000000000, -0.000000000000000000 ) ) ;
#4477=CARTESIAN_POINT ( 'NONE',  ( -19.19641293061498644, 418.8073905683720000, 14.20200298773971426 ) ) ;
#4478=CARTESIAN_POINT ( 'NONE',  ( -17.35679799567829207, 395.4323905765655809, 16.95518130045146421 ) ) ;
#4480=CARTESIAN_POINT ( 'NONE',  ( -14.48388495494900852, 449.8073905683720000, -9.489475012073736337 ) ) ;
#4481=EDGE_LOOP ( 'NONE', ( #21096, #20626, #19086, #11523 ) ) ;
#4482=CARTESIAN_POINT ( 'NONE',  ( -13.20868407381887444, 469.4948905683720000, -6.410867750099233042 ) ) ;
#4485=CARTESIAN_POINT ( 'NONE',  ( -28.68588794268871567, 374.4948905765656377, 19.99999999999999289 ) ) ;
#4487=CARTESIAN_POINT ( 'NONE',  ( -8.685887942688740537, 522.2448905601784190, -2.449293598294705724E-15 ) ) ;
#4488=DIRECTION ( 'NONE',  ( -1.191790137725560488E-16, 1.000000000000000000, -0.000000000000000000 ) ) ;
#4491=CARTESIAN_POINT ( 'NONE',  ( -8.685887942688731655, 452.2448905601784759, -2.449293598294705724E-15 ) ) ;
#4494=CARTESIAN_POINT ( 'NONE',  ( -13.20868407381886556, 419.7448905683720000, 6.410867750099229490 ) ) ;
#4496=CARTESIAN_POINT ( 'NONE',  ( -45.43829269268869098, 245.6823905683720284, 3.332260488124734632 ) ) ;
#4500=CARTESIAN_POINT ( 'NONE',  ( -11.93348319268873503, 470.6823905683720000, -3.332260488124732856 ) ) ;
#4501=CARTESIAN_POINT ( 'NONE',  ( -32.66413529028186247, 219.8073905765656377, -19.99999999999999289 ) ) ;
#4502=( GEOMETRIC_REPRESENTATION_CONTEXT ( 3 ) GLOBAL_UNCERTAINTY_ASSIGNED_CONTEXT ( ( #18501 ) ) GLOBAL_UNIT_ASSIGNED_CONTEXT ( ( #9106, #19067, #15620 ) ) REPRESENTATION_CONTEXT ( 'NONE', 'WORKASPACE' ) );
#4504=DIRECTION ( 'NONE',  ( -1.191790137725560488E-16, 1.000000000000000000, -0.000000000000000000 ) ) ;
#4505=CARTESIAN_POINT ( 'NONE',  ( -32.01814843081343298, 226.0573905683720568, 16.75240474999999307 ) ) ;
#4507=CARTESIAN_POINT ( 'NONE',  ( -45.43829269268873361, 533.8698905683720568, 0.000000000000000000 ) ) ;
#4511=CARTESIAN_POINT ( 'NONE',  ( -11.73070664223726389, 467.9323905765655809, -11.32908994701042715 ) ) ;
#4513=CARTESIAN_POINT ( 'NONE',  ( -8.685887942688712116, 276.9948905765656377, -2.449293598294705724E-15 ) ) ;
#4514=CARTESIAN_POINT ( 'NONE',  ( -10.20829729246297291, 237.6198905765656377, -7.653668647301794969 ) ) ;
#4517=CARTESIAN_POINT ( 'NONE',  ( -45.43829269268869098, 223.5573905683720284, -3.332260488124726194 ) ) ;
#4518=CARTESIAN_POINT ( 'NONE',  ( -16.84014894278198327, 319.1198905683720568, 11.84573899990672530 ) ) ;
#4521=CARTESIAN_POINT ( 'NONE',  ( -22.27502019258947996, 312.2448905683720000, -15.47720386886985544 ) ) ;
#4524=CARTESIAN_POINT ( 'NONE',  ( -22.27502019258947996, 386.9948905683720568, 15.47720386886985189 ) ) ;
#4526=CARTESIAN_POINT ( 'NONE',  ( -32.01814843081346140, 533.1823905683720568, -16.75240474999999307 ) ) ;
#4527=CARTESIAN_POINT ( 'NONE',  ( -48.68588794268870856, 367.5573905601785327, 3.978247347593168115 ) ) ;
#4528=CARTESIAN_POINT ( 'NONE',  ( -48.68588794268872277, 497.2448905601785327, 0.000000000000000000 ) ) ;
#4530=CARTESIAN_POINT ( 'NONE',  ( -44.16309181155857999, 485.9948905683720568, 6.410867750099241924 ) ) ;
#4532=CYLINDRICAL_SURFACE ( 'NONE', #6955, 19.99999999999999645 ) ;
#4533=VECTOR ( 'NONE', #10141, 1000.000000000000000 ) ;
#4534=ORIENTED_EDGE ( 'NONE', *, *, #11651, .F. ) ;
#4535=CARTESIAN_POINT ( 'NONE',  ( -32.01814843081344009, 293.1823905683720568, -16.75240474999999307 ) ) ;
#4536=CARTESIAN_POINT ( 'NONE',  ( -11.93348319268871727, 319.1823905683720568, -3.332260488124732856 ) ) ;
#4537=EDGE_CURVE ( 'NONE', #1608, #20007, #17602, .T. ) ;
#4539=CARTESIAN_POINT ( 'NONE',  ( -45.64106924314017277, 261.0573905765656377, -11.32908994701042715 ) ) ;
#4541=CARTESIAN_POINT ( 'NONE',  ( -14.48388495494898187, 227.9323905683720000, 9.489475012073731008 ) ) ;
#4542=CARTESIAN_POINT ( 'NONE',  ( -18.66955214161060894, 223.9106467678502383, -17.31106641270412183 ) ) ;
#4543=CARTESIAN_POINT ( 'NONE',  ( -22.27502019258947996, 378.4948905683720000, 15.47720386886985189 ) ) ;
#4547=CARTESIAN_POINT ( 'NONE',  ( -25.35362745456399125, 446.6823905683720568, 16.75240474999998952 ) ) ;
#4550=CARTESIAN_POINT ( 'NONE',  ( -21.03221929538691981, 450.3698905601784759, 18.47759065022572500 ) ) ;
#4552=ORIENTED_EDGE ( 'NONE', *, *, #14782, .T. ) ;
#4555=CARTESIAN_POINT ( 'NONE',  ( -32.66413529028187668, 335.0573905601784759, -19.99999999999999289 ) ) ;
#4558=CARTESIAN_POINT ( 'NONE',  ( -22.27502019258948707, 372.2448905683720000, -15.47720386886985544 ) ) ;
#4560=CARTESIAN_POINT ( 'NONE',  ( -47.16347859291445843, 502.6198905765656377, 7.653668647301805628 ) ) ;
#4561=CARTESIAN_POINT ( 'NONE',  ( -45.43829269268871229, 394.1823905683720000, 3.332260488124734632 ) ) ;
#4562=CARTESIAN_POINT ( 'NONE',  ( -32.01814843081343298, 227.5573905683720568, 16.75240474999999307 ) ) ;
#4563=CARTESIAN_POINT ( 'NONE',  ( -19.19641293061498288, 377.3073905683721136, 14.20200298773971426 ) ) ;
#4564=CARTESIAN_POINT ( 'NONE',  ( -40.01497788969913216, 333.5573905765655240, 16.95518130045146776 ) ) ;
#4566=CARTESIAN_POINT ( 'NONE',  ( -32.01814843081344009, 286.0573905683720568, 16.75240474999999307 ) ) ;
#4567=CARTESIAN_POINT ( 'NONE',  ( -35.09675569278795848, 453.4948905683720568, -15.47720386886985544 ) ) ;
#4568=CARTESIAN_POINT ( 'NONE',  ( -42.82802356641967378, 458.4948905601784759, 14.14213562373094923 ) ) ;
#4572=CARTESIAN_POINT ( 'NONE',  ( -13.20868407381886023, 369.7448905683720568, 6.410867750099229490 ) ) ;
#4573=CARTESIAN_POINT ( 'NONE',  ( -45.43829269268871940, 493.5573905683720568, -3.332260488124726194 ) ) ;
#4574=CARTESIAN_POINT ( 'NONE',  ( -45.64106924314020119, 506.3073905601784759, -11.32908994701042715 ) ) ;
#4575=CARTESIAN_POINT ( 'NONE',  ( -16.84014894278198682, 320.1198905683720568, -11.84573899990672707 ) ) ;
#4576=EDGE_LOOP ( 'NONE', ( #7682, #10156, #19212, #2994 ) ) ;
#4577=CARTESIAN_POINT ( 'NONE',  ( -47.16347859291443001, 257.8698905601785327, 7.653668647301805628 ) ) ;
#4581=CARTESIAN_POINT ( 'NONE',  ( -40.53162694259544452, 426.6198905683720000, 11.84573899990672885 ) ) ;
#4582=CARTESIAN_POINT ( 'NONE',  ( -48.68588794268869435, 231.9948905765656377, 0.000000000000000000 ) ) ;
#4583=CARTESIAN_POINT ( 'NONE',  ( -11.93348319268872970, 438.5573905683720000, 3.332260488124728415 ) ) ;
#4585=CARTESIAN_POINT ( 'NONE',  ( -22.27502019258949773, 460.7448905683720568, -15.47720386886985544 ) ) ;
#4587=CARTESIAN_POINT ( 'NONE',  ( -42.82802356641965957, 383.2448905765656377, 14.14213562373094923 ) ) ;
#4591=CARTESIAN_POINT ( 'NONE',  ( -8.685887942688886199, 256.6823905765655809, 3.978247347593586447 ) ) ;
#4596=CARTESIAN_POINT ( 'NONE',  ( -39.91673061078817852, 223.9102039777116886, 15.70339761151467606 ) ) ;
#4598=CARTESIAN_POINT ( 'NONE',  ( -44.16309181155857289, 435.9948905683720568, 6.410867750099241924 ) ) ;
#4600=CARTESIAN_POINT ( 'NONE',  ( -19.19641293061497223, 241.9323905683720284, -14.20200298773971603 ) ) ;
#4605=EDGE_LOOP ( 'NONE', ( #4072, #4113, #13010, #15980 ) ) ;
#4606=CARTESIAN_POINT ( 'NONE',  ( -11.93348319268873503, 470.0573905683720568, 3.332260488124728859 ) ) ;
#4607=CARTESIAN_POINT ( 'NONE',  ( -11.73070664223723369, 227.9323905765656662, -11.32908994701042715 ) ) ;
#4611=CARTESIAN_POINT ( 'NONE',  ( -14.48388495494901917, 531.3073905683719431, -9.489475012073736337 ) ) ;
#4615=CARTESIAN_POINT ( 'NONE',  ( -17.35679799567830983, 448.5573905765656946, -16.95518130045146421 ) ) ;
#4617=CARTESIAN_POINT ( 'NONE',  ( -28.68588794268874054, 573.2448905601785327, 0.000000000000000000 ) ) ;
#4619=DIRECTION ( 'NONE',  ( 1.000000000000000000, 1.191790137725560488E-16, 0.000000000000000000 ) ) ;
#4621=CARTESIAN_POINT ( 'NONE',  ( -28.68588794268869790, 236.3698905683720568, 16.75240474999999307 ) ) ;
#4622=CARTESIAN_POINT ( 'NONE',  ( -11.93348319268871727, 310.0573905683720568, 3.332260488124728415 ) ) ;
#4624=CARTESIAN_POINT ( 'NONE',  ( -36.33955658999049376, 235.3698905601784759, -18.47759065022572855 ) ) ;
#4625=CARTESIAN_POINT ( 'NONE',  ( -48.68588794268870856, 377.2448905601784759, 0.000000000000000000 ) ) ;
#4627=CARTESIAN_POINT ( 'NONE',  ( -11.93348319268871371, 300.3698905683720568, -2.051577885510841163E-15 ) ) ;
#4628=CARTESIAN_POINT ( 'NONE',  ( -44.16309181155857289, 363.2448905683720000, -6.410867750099231266 ) ) ;
#4629=CARTESIAN_POINT ( 'NONE',  ( -35.09675569278797269, 527.2448905683719431, 15.47720386886985366 ) ) ;
#4630=CARTESIAN_POINT ( 'NONE',  ( -11.73070664223725146, 363.1823905601784759, -11.32908994701042715 ) ) ;
#4631=CARTESIAN_POINT ( 'NONE',  ( -47.16347859291445133, 406.6198905601784759, -7.653668647301793193 ) ) ;
#4633=CARTESIAN_POINT ( 'NONE',  ( -14.48388495494901385, 489.4323905683720568, 9.489475012073732785 ) ) ;
#4634=DIRECTION ( 'NONE',  ( -1.191790137725560488E-16, 1.000000000000000000, -0.000000000000000000 ) ) ;
#4635=CARTESIAN_POINT ( 'NONE',  ( -22.27502019258946930, 286.9948905683720000, 15.47720386886985189 ) ) ;
#4636=VERTEX_POINT ( 'NONE', #7725 ) ;
#4637=CARTESIAN_POINT ( 'NONE',  ( -13.20868407381884779, 279.7448905683720568, 6.410867750099229490 ) ) ;
#4638=CARTESIAN_POINT ( 'NONE',  ( -32.01814843081344009, 316.0573905683720000, 16.75240474999999307 ) ) ;
#4639=CARTESIAN_POINT ( 'NONE',  ( -13.20868407381884779, 260.9948905683720568, -6.410867750099233042 ) ) ;
#4642=CARTESIAN_POINT ( 'NONE',  ( -21.03221929538689849, 255.1198905765656377, 18.47759065022572500 ) ) ;
#4644=CARTESIAN_POINT ( 'NONE',  ( -45.43280446313950449, 223.9102039777116602, 0.4287796227366179602 ) ) ;
#4645=CARTESIAN_POINT ( 'NONE',  ( -13.20868407381886023, 369.7448905683720568, 6.410867750099229490 ) ) ;
#4648=EDGE_CURVE ( 'NONE', #5794, #18805, #752, .T. ) ;
#4650=CARTESIAN_POINT ( 'NONE',  ( -45.43829269268871940, 433.8698905683720568, 0.000000000000000000 ) ) ;
#4653=CARTESIAN_POINT ( 'NONE',  ( -8.685887942688728103, 422.5573905601785327, -3.978247347593165895 ) ) ;
#4654=ORIENTED_EDGE ( 'NONE', *, *, #15114, .F. ) ;
#4657=CARTESIAN_POINT ( 'NONE',  ( -32.66413529028186957, 354.1823905765656377, 19.99999999999999289 ) ) ;
#4658=CARTESIAN_POINT ( 'NONE',  ( -11.73070664223724613, 313.1823905601784190, -11.32908994701042715 ) ) ;
#4659=DIRECTION ( 'NONE',  ( -1.000000000000000000, 0.000000000000000000, 0.000000000000000000 ) ) ;
#4660=CARTESIAN_POINT ( 'NONE',  ( -13.20868407381885667, 339.7448905683720568, 6.410867750099229490 ) ) ;
#4661=CARTESIAN_POINT ( 'NONE',  ( -17.35679799567831338, 498.5573905765655809, -16.95518130045146421 ) ) ;
#4662=CARTESIAN_POINT ( 'NONE',  ( -19.19641293061498644, 377.3073905683720568, 14.20200298773971426 ) ) ;
#4664=CARTESIAN_POINT ( 'NONE',  ( -45.43829269268871940, 394.1823905683720000, 3.332260488124734632 ) ) ;
#4666=CARTESIAN_POINT ( 'NONE',  ( -8.685887942688715668, 316.6823905765655240, 3.978247347593161010 ) ) ;
#4667=CARTESIAN_POINT ( 'NONE',  ( -11.73070664223725679, 423.1823905601785327, -11.32908994701042538 ) ) ;
#4668=CARTESIAN_POINT ( 'NONE',  ( -13.20868407381885135, 289.4948905683720000, -6.410867750099233042 ) ) ;
#4669=CARTESIAN_POINT ( 'NONE',  ( -25.35362745456400191, 442.5573905683720568, -16.75240474999999307 ) ) ;
#4670=CARTESIAN_POINT ( 'NONE',  ( -43.68588794268869435, 213.9102039777116602, 0.000000000000000000 ) ) ;
#4672=CYLINDRICAL_SURFACE ( 'NONE', #6080, 19.99999999999999645 ) ;
#4673=CARTESIAN_POINT ( 'NONE',  ( -14.48388495494899608, 339.4323905683720000, 9.489475012073732785 ) ) ;
#4674=CARTESIAN_POINT ( 'NONE',  ( -40.53162694259545873, 512.6198905683720568, -11.84573899990672707 ) ) ;
#4675=CARTESIAN_POINT ( 'NONE',  ( -42.82802356641967378, 495.9948905601784759, -14.14213562373094746 ) ) ;
#4676=CARTESIAN_POINT ( 'NONE',  ( -45.43829269268869808, 323.5573905683720000, -3.332260488124726194 ) ) ;
#4677=EDGE_CURVE ( 'NONE', #4217, #15177, #8039, .T. ) ;
#4679=CARTESIAN_POINT ( 'NONE',  ( -48.68588794268886488, 257.5573905601784190, 3.978247347592742678 ) ) ;
#4682=CARTESIAN_POINT ( 'NONE',  ( -28.68588794268871922, 402.8698905683720000, -16.75240474999999307 ) ) ;
#4683=CARTESIAN_POINT ( 'NONE',  ( -21.03221929538689849, 235.1198905765656377, 18.47759065022572500 ) ) ;
#4684=CARTESIAN_POINT ( 'NONE',  ( -44.16309181155858710, 453.2448905683720000, -6.410867750099231266 ) ) ;
#4685=CARTESIAN_POINT ( 'NONE',  ( -11.93348319268873148, 448.8698905683720000, -2.051577885510841163E-15 ) ) ;
#4689=CARTESIAN_POINT ( 'NONE',  ( -32.66413529028188378, 389.8073905765656377, -19.99999999999999289 ) ) ;
#4692=CARTESIAN_POINT ( 'NONE',  ( -10.20829729246299422, 427.6198905765656377, -7.653668647301794969 ) ) ;
#4694=CARTESIAN_POINT ( 'NONE',  ( -42.88789093042844769, 496.3073905683720568, 9.489475012073736337 ) ) ;
#4695=CARTESIAN_POINT ( 'NONE',  ( -8.685887942688742314, 573.2448905601785327, 2.449293598294706119E-15 ) ) ;
#4697=CARTESIAN_POINT ( 'NONE',  ( -11.73070664223725323, 421.3073905601784190, 11.32908994701042005 ) ) ;
#4698=CARTESIAN_POINT ( 'NONE',  ( -35.09675569278795848, 407.2448905683720568, 15.47720386886985366 ) ) ;
#4701=CARTESIAN_POINT ( 'NONE',  ( -32.01814843081343298, 257.5573905683720568, 16.75240474999999307 ) ) ;
#4704=ORIENTED_EDGE ( 'NONE', *, *, #14132, .F. ) ;
#4705=CARTESIAN_POINT ( 'NONE',  ( -42.88789093042844769, 466.3073905683721136, 9.489475012073734561 ) ) ;
#4706=CARTESIAN_POINT ( 'NONE',  ( -24.70764059509552979, 224.8073905765656662, 19.99999999999998934 ) ) ;
#4708=CARTESIAN_POINT ( 'NONE',  ( -40.01497788969915348, 523.5573905765656946, 16.95518130045146776 ) ) ;
#4709=CARTESIAN_POINT ( 'NONE',  ( -22.27502019258949773, 528.4948905683719431, 15.47720386886985189 ) ) ;
#4710=ORIENTED_EDGE ( 'NONE', *, *, #16903, .T. ) ;
#4711=CARTESIAN_POINT ( 'NONE',  ( -11.93348319268873858, 499.1823905683720568, -3.332260488124732856 ) ) ;
#4714=CARTESIAN_POINT ( 'NONE',  ( -42.82802356641966668, 443.2448905765656377, 14.14213562373094923 ) ) ;
#4715=CARTESIAN_POINT ( 'NONE',  ( -8.685887942688706786, 232.2448905601785043, -2.449293598294705724E-15 ) ) ;
#4716=CARTESIAN_POINT ( 'NONE',  ( -25.35362745456397704, 336.6823905683720568, 16.75240474999998952 ) ) ;
#4724=CARTESIAN_POINT ( 'NONE',  ( -25.35362745456398770, 322.5573905683720000, -16.75240474999999307 ) ) ;
#4725=CARTESIAN_POINT ( 'NONE',  ( -40.01497788969914637, 445.6823905601784190, -16.95518130045146421 ) ) ;
#4727=CARTESIAN_POINT ( 'NONE',  ( -22.27502019258947286, 318.4948905683720000, 15.47720386886985189 ) ) ;
#4729=CARTESIAN_POINT ( 'NONE',  ( -45.43829269268873361, 515.0573905683720568, -3.332260488124726638 ) ) ;
#4730=CARTESIAN_POINT ( 'NONE',  ( -45.64106924314018698, 366.3073905601785327, -11.32908994701042715 ) ) ;
#4732=CARTESIAN_POINT ( 'NONE',  ( -48.68588794268872988, 521.9948905765656946, 0.000000000000000000 ) ) ;
#4733=ORIENTED_EDGE ( 'NONE', *, *, #2098, .T. ) ;
#4734=CARTESIAN_POINT ( 'NONE',  ( -11.93348319268873503, 480.3698905683720568, -2.051577885510841163E-15 ) ) ;
#4736=CARTESIAN_POINT ( 'NONE',  ( -11.93348319268871371, 288.5573905683720000, 3.332260488124728415 ) ) ;
#4738=CARTESIAN_POINT ( 'NONE',  ( -19.19641293061497223, 288.8073905683719431, 14.20200298773971426 ) ) ;
#4739=CARTESIAN_POINT ( 'NONE',  ( -38.17536295476244845, 322.3073905683720568, -14.20200298773971426 ) ) ;
#4740=CARTESIAN_POINT ( 'NONE',  ( -38.17536295476243424, 266.9323905683720568, 14.20200298773971781 ) ) ;
#4741=CARTESIAN_POINT ( 'NONE',  ( -42.82802356641964536, 260.7448905765656377, -14.14213562373094746 ) ) ;
#4742=LINE ( 'NONE', #19775, #21056 ) ;
#4743=CARTESIAN_POINT ( 'NONE',  ( -28.68588794268869435, 226.3698905683720284, 16.75240474999999307 ) ) ;
#4744=CARTESIAN_POINT ( 'NONE',  ( -16.84014894278199037, 371.6198905683720000, -11.84573899990672707 ) ) ;
#4750=CARTESIAN_POINT ( 'NONE',  ( -11.93348319268872970, 429.1823905683720568, -3.332260488124732856 ) ) ;
#4753=CARTESIAN_POINT ( 'NONE',  ( -32.66413529028188378, 435.0573905601784759, -19.99999999999999289 ) ) ;
#4758=CARTESIAN_POINT ( 'NONE',  ( -17.35679799567828496, 300.6823905601784759, 16.95518130045146421 ) ) ;
#4760=CARTESIAN_POINT ( 'NONE',  ( -40.53162694259543741, 344.1198905683720568, -11.84573899990672707 ) ) ;
#4762=CARTESIAN_POINT ( 'NONE',  ( -32.66413529028189089, 499.8073905765656377, -19.99999999999999289 ) ) ;
#4763=CARTESIAN_POINT ( 'NONE',  ( -38.17536295476245556, 382.3073905683719431, -14.20200298773971426 ) ) ;
#4765=CARTESIAN_POINT ( 'NONE',  ( -11.93348319268872260, 378.5573905683721136, 3.332260488124728859 ) ) ;
#4766=( BOUNDED_CURVE ( )  B_SPLINE_CURVE ( 2, ( #12070, #18771, #3959, #10547, #5791, #2347, #10761, #15551, #843, #735, #7302, #12397, #18877, #4067, #10651, #17271, #14034 ),
 .UNSPECIFIED., .F., .T. ) 
 B_SPLINE_CURVE_WITH_KNOTS ( ( 3, 2, 2, 2, 2, 2, 2, 2, 3 ),
 ( 0.6250000000000002220, 0.6269531250000002220, 0.6289062500000002220, 0.6308593750000002220, 0.6328125000000002220, 0.6347656250000002220, 0.6367187500000002220, 0.6386718750000002220, 0.6406250000000002220 ),
 .UNSPECIFIED. ) 
 CURVE ( )  GEOMETRIC_REPRESENTATION_ITEM ( )  RATIONAL_B_SPLINE_CURVE ( ( 0.9999999999999977796, 0.9807852804032326510, 1.000000000000000000, 0.9807852804032304306, 1.000000000000000000, 0.9807852804032304306, 1.000000000000000000, 0.9807852804032304306, 1.000000000000000000, 0.9807852804032304306, 1.000000000000000000, 0.9807852804032304306, 1.000000000000000000, 0.9807852804032304306, 1.000000000000000000, 0.9807852804032282101, 1.000000000000002220 ) ) 
 REPRESENTATION_ITEM ( '' )  );
#4767=CARTESIAN_POINT ( 'NONE',  ( -10.20829729246298179, 326.3698905765656377, 7.653668647301790529 ) ) ;
#4769=CARTESIAN_POINT ( 'NONE',  ( -44.16309181155856578, 283.2448905683720568, -6.410867750099231266 ) ) ;
#4770=CARTESIAN_POINT ( 'NONE',  ( -40.53162694259544452, 444.1198905683720568, -11.84573899990672707 ) ) ;
#4774=CARTESIAN_POINT ( 'NONE',  ( -45.43829269268870519, 345.6823905683720568, 3.332260488124734632 ) ) ;
#4775=CARTESIAN_POINT ( 'NONE',  ( -44.16309181155858710, 473.2448905683720568, -6.410867750099231266 ) ) ;
#4776=CARTESIAN_POINT ( 'NONE',  ( -48.68588794268872277, 476.9323905601784759, -3.978247347593158345 ) ) ;
#4777=CARTESIAN_POINT ( 'NONE',  ( -25.35362745456397704, 326.6823905683720568, 16.75240474999998952 ) ) ;
#4781=ORIENTED_EDGE ( 'NONE', *, *, #14481, .F. ) ;
#4784=CARTESIAN_POINT ( 'NONE',  ( -28.68588794268871922, 407.8698905683720568, 16.75240474999999307 ) ) ;
#4785=CARTESIAN_POINT ( 'NONE',  ( -28.68588794268874054, 573.2448905601785327, 0.000000000000000000 ) ) ;
#4787=CARTESIAN_POINT ( 'NONE',  ( -45.43829269268871940, 454.1823905683720568, 3.332260488124734632 ) ) ;
#4788=CARTESIAN_POINT ( 'NONE',  ( -44.16309181155857289, 444.4948905683720568, 6.410867750099241924 ) ) ;
#4790=CARTESIAN_POINT ( 'NONE',  ( -48.68588794268858067, 416.9323905601784190, -3.978247347593477201 ) ) ;
#4791=CARTESIAN_POINT ( 'NONE',  ( -48.68588794268870856, 381.6823905765656377, -3.978247347593158345 ) ) ;
#4793=CARTESIAN_POINT ( 'NONE',  ( -24.70764059509554755, 264.4323905601784759, -19.99999999999999289 ) ) ;
#4796=CARTESIAN_POINT ( 'NONE',  ( -13.20868407381887621, 499.7448905683720000, 6.410867750099229490 ) ) ;
#4797=EDGE_CURVE ( 'NONE', #19523, #15642, #5970, .T. ) ;
#4802=CARTESIAN_POINT ( 'NONE',  ( -14.48388495494900496, 411.3073905683720000, -9.489475012073736337 ) ) ;
#4803=CARTESIAN_POINT ( 'NONE',  ( -32.66413529028188378, 469.8073905765656377, -19.99999999999999289 ) ) ;
#4804=CARTESIAN_POINT ( 'NONE',  ( -35.09675569278793716, 227.2448905683720568, 15.47720386886985366 ) ) ;
#4805=EDGE_CURVE ( 'NONE', #9261, #16878, #18427, .T. ) ;
#4807=CARTESIAN_POINT ( 'NONE',  ( -47.16347859291445133, 422.6198905765656377, 7.653668647301805628 ) ) ;
#4810=CARTESIAN_POINT ( 'NONE',  ( -13.20868407381887089, 469.7448905683720568, 6.410867750099229490 ) ) ;
#4811=CARTESIAN_POINT ( 'NONE',  ( -21.03221929538689494, 225.1198905765656093, 18.47759065022572500 ) ) ;
#4813=CARTESIAN_POINT ( 'NONE',  ( -43.04716123355245116, 207.6569251493015429, 4.334626618252812591 ) ) ;
#4814=CARTESIAN_POINT ( 'NONE',  ( -32.01814843081346851, 527.5573905683720568, 16.75240474999999307 ) ) ;
#4816=CARTESIAN_POINT ( 'NONE',  ( -35.09675569278797269, 515.7448905683720568, 15.47720386886985366 ) ) ;
#4819=CARTESIAN_POINT ( 'NONE',  ( -40.01497788969913927, 443.5573905765656377, 16.95518130045146776 ) ) ;
#4822=CARTESIAN_POINT ( 'NONE',  ( -40.01497788969914637, 453.5573905765656377, 16.95518130045146776 ) ) ;
#4826=CARTESIAN_POINT ( 'NONE',  ( -15.76477386065954356, 223.9102039777117739, -15.36505724430687714 ) ) ;
#4827=CARTESIAN_POINT ( 'NONE',  ( -35.09675569278793716, 323.4948905683720000, -15.47720386886985544 ) ) ;
#4828=CARTESIAN_POINT ( 'NONE',  ( -8.685887942688642838, 442.5573905601784759, -3.978247347592952732 ) ) ;
#4829=CARTESIAN_POINT ( 'NONE',  ( -45.64106924314017988, 276.3073905601785327, -11.32908994701042715 ) ) ;
#4831=CARTESIAN_POINT ( 'NONE',  ( -44.16309181155855867, 285.9948905683720000, 6.410867750099241924 ) ) ;
#4832=CARTESIAN_POINT ( 'NONE',  ( -38.17536295476247687, 523.8073905683720568, -14.20200298773971426 ) ) ;
#4833=CARTESIAN_POINT ( 'NONE',  ( -36.33955658999051508, 359.1198905601785327, 18.47759065022572500 ) ) ;
#4835=ORIENTED_EDGE ( 'NONE', *, *, #17610, .T. ) ;
#4836=CARTESIAN_POINT ( 'NONE',  ( -38.17536295476246266, 486.9323905683721136, 14.20200298773971781 ) ) ;
#4838=CARTESIAN_POINT ( 'NONE',  ( -35.09675569278793716, 281.9948905683720000, -15.47720386886985544 ) ) ;
#4841=CARTESIAN_POINT ( 'NONE',  ( -44.16309181155855867, 275.9948905683720000, 6.410867750099241924 ) ) ;
#4842=CARTESIAN_POINT ( 'NONE',  ( -45.43829269268870519, 313.8698905683720000, 0.000000000000000000 ) ) ;
#4844=CARTESIAN_POINT ( 'NONE',  ( -17.35679799567828496, 238.5573905765656093, -16.95518130045146421 ) ) ;
#4846=CARTESIAN_POINT ( 'NONE',  ( -48.68588794268870146, 321.9948905765655809, 0.000000000000000000 ) ) ;
#4849=CARTESIAN_POINT ( 'NONE',  ( -16.84014894278199037, 379.1198905683720568, 11.84573899990672530 ) ) ;
#4854=CARTESIAN_POINT ( 'NONE',  ( -40.01497788969915348, 460.4323905765656377, -16.95518130045146421 ) ) ;
#4856=CARTESIAN_POINT ( 'NONE',  ( -48.68588794268853803, 271.6823905765656377, -3.978247347593583783 ) ) ;
#4857=CARTESIAN_POINT ( 'NONE',  ( -22.27502019258949417, 420.7448905683720000, -15.47720386886985544 ) ) ;
#4861=CARTESIAN_POINT ( 'NONE',  ( -11.73070664223725679, 423.1823905601784759, -11.32908994701042715 ) ) ;
#4862=EDGE_CURVE ( 'NONE', #11055, #502, #19950, .T. ) ;
#4864=CARTESIAN_POINT ( 'NONE',  ( -22.27502019258947641, 262.2448905683720000, -15.47720386886985544 ) ) ;
#4866=VERTEX_POINT ( 'NONE', #15096 ) ;
#4867=ORIENTED_EDGE ( 'NONE', *, *, #16163, .F. ) ;
#4869=CARTESIAN_POINT ( 'NONE',  ( -48.68588794268870146, 306.9323905601785327, -3.978247347593158345 ) ) ;
#4871=CARTESIAN_POINT ( 'NONE',  ( -44.16309181155856578, 335.9948905683720000, 6.410867750099241924 ) ) ;
#4873=CARTESIAN_POINT ( 'NONE',  ( -45.64106924314020119, 492.9323905765655809, 11.32908994701042715 ) ) ;
#4874=CARTESIAN_POINT ( 'NONE',  ( -19.19641293061498644, 370.4323905683720000, -14.20200298773971603 ) ) ;
#4875=CARTESIAN_POINT ( 'NONE',  ( -47.16347859291443712, 311.3698905765656377, -7.653668647301793193 ) ) ;
#4876=CARTESIAN_POINT ( 'NONE',  ( -19.19641293061498644, 380.4323905683720568, -14.20200298773971603 ) ) ;
#4877=CARTESIAN_POINT ( 'NONE',  ( -47.16347859291443712, 321.3698905765656377, -7.653668647301793193 ) ) ;
#4879=CARTESIAN_POINT ( 'NONE',  ( -44.16309181155855867, 284.4948905683720000, 6.410867750099241924 ) ) ;
#4881=CARTESIAN_POINT ( 'NONE',  ( -25.35362745456399836, 432.5573905683719431, -16.75240474999999307 ) ) ;
#4884=CARTESIAN_POINT ( 'NONE',  ( -28.68588794268874054, 573.2448905601785327, 0.000000000000000000 ) ) ;
#4886=CARTESIAN_POINT ( 'NONE',  ( -28.68588794268871567, 352.8698905683720568, -16.75240474999999307 ) ) ;
#4887=CARTESIAN_POINT ( 'NONE',  ( -14.48388495494901562, 489.8073905683720568, -9.489475012073736337 ) ) ;
#4890=CARTESIAN_POINT ( 'NONE',  ( -32.66413529028189089, 489.4323905601784759, 19.99999999999999289 ) ) ;
#4891=CARTESIAN_POINT ( 'NONE',  ( -14.48388495494899431, 309.8073905683720568, -9.489475012073736337 ) ) ;
#4893=CARTESIAN_POINT ( 'NONE',  ( -21.03221929538694468, 524.1198905601785327, -18.47759065022572855 ) ) ;
#4896=( BOUNDED_CURVE ( )  B_SPLINE_CURVE ( 2, ( #8394, #18351, #15020, #19978, #10125, #15126, #12068, #13285, #13497, #11962, #203, #19870, #16746, #5046, #20190, #15225, #11647 ),
 .UNSPECIFIED., .F., .T. ) 
 B_SPLINE_CURVE_WITH_KNOTS ( ( 3, 2, 2, 2, 2, 2, 2, 2, 3 ),
 ( 0.01562500000000037470, 0.01757812500000033307, 0.01953125000000028796, 0.02148437500000024286, 0.02343750000000020123, 0.02539062500000015959, 0.02734375000000011449, 0.02929687500000006939, 0.03125000000000002776 ),
 .UNSPECIFIED. ) 
 CURVE ( )  GEOMETRIC_REPRESENTATION_ITEM ( )  RATIONAL_B_SPLINE_CURVE ( ( 0.9999999999999963363, 0.9807852804032340943, 1.000000000000000000, 0.9807852804032304306, 1.000000000000000000, 0.9807852804032304306, 1.000000000000000000, 0.9807852804032304306, 1.000000000000000000, 0.9807852804032304306, 1.000000000000000000, 0.9807852804032304306, 1.000000000000000000, 0.9807852804032304306, 1.000000000000000000, 0.9807852804032302085, 1.000000000000000222 ) ) 
 REPRESENTATION_ITEM ( '' )  );
#4897=CARTESIAN_POINT ( 'NONE',  ( -16.84014894278199392, 401.6198905683720568, -11.84573899990672707 ) ) ;
#4900=CARTESIAN_POINT ( 'NONE',  ( -13.20868407381886733, 438.2448905683720000, 6.410867750099229490 ) ) ;
#4902=CARTESIAN_POINT ( 'NONE',  ( -11.93348319268873148, 449.1823905683720000, -3.332260488124732856 ) ) ;
#4905=CARTESIAN_POINT ( 'NONE',  ( -28.68588794268871922, 379.4948905765656377, -19.99999999999999289 ) ) ;
#4906=FACE_OUTER_BOUND ( 'NONE', #18380, .T. ) ;
#4910=CARTESIAN_POINT ( 'NONE',  ( -13.20868407381887444, 489.7448905683720568, 6.410867750099229490 ) ) ;
#4912=CARTESIAN_POINT ( 'NONE',  ( -28.68588794268874054, 573.2448905601785327, 0.000000000000000000 ) ) ;
#4913=CARTESIAN_POINT ( 'NONE',  ( -45.64106924314020119, 518.1823905601785327, 11.32908994701042538 ) ) ;
#4915=CARTESIAN_POINT ( 'NONE',  ( -32.01814843081345430, 413.1823905683719431, -16.75240474999999307 ) ) ;
#4916=CARTESIAN_POINT ( 'NONE',  ( -8.685887942688724550, 372.2448905601784759, -2.449293598294705724E-15 ) ) ;
#4919=CARTESIAN_POINT ( 'NONE',  ( -38.17536295476244135, 233.8073905683720284, -14.20200298773971426 ) ) ;
#4923=CARTESIAN_POINT ( 'NONE',  ( -16.84014894278200103, 451.6198905683720568, -11.84573899990672707 ) ) ;
#4924=CARTESIAN_POINT ( 'NONE',  ( -32.01814843081346851, 531.6823905683719431, -16.75240474999999307 ) ) ;
#4927=CARTESIAN_POINT ( 'NONE',  ( -43.60132883224873268, 209.8855831874335820, 1.619299207070719726 ) ) ;
#4928=CARTESIAN_POINT ( 'NONE',  ( -40.53162694259542320, 222.6198905683720000, -11.84573899990672707 ) ) ;
#4930=CARTESIAN_POINT ( 'NONE',  ( -22.27502019258950128, 510.7448905683720000, -15.47720386886985544 ) ) ;
#4931=FACE_OUTER_BOUND ( 'NONE', #4605, .T. ) ;
#4932=CARTESIAN_POINT ( 'NONE',  ( -8.685887942688729879, 436.6823905765656377, 3.978247347593161010 ) ) ;
#4934=CARTESIAN_POINT ( 'NONE',  ( -48.68588794268870146, 327.5573905601784759, 3.978247347593168559 ) ) ;
#4940=CARTESIAN_POINT ( 'NONE',  ( -48.68588794268872277, 491.9948905765656377, 0.000000000000000000 ) ) ;
#4941=CARTESIAN_POINT ( 'NONE',  ( -40.53162694259543031, 314.1198905683720568, -11.84573899990672707 ) ) ;
#4942=CARTESIAN_POINT ( 'NONE',  ( -45.64106924314016567, 236.3073905601784759, -11.32908994701042538 ) ) ;
#4943=CARTESIAN_POINT ( 'NONE',  ( -32.66413529028186247, 269.4323905601785327, 19.99999999999999289 ) ) ;
#4945=CARTESIAN_POINT ( 'NONE',  ( -16.84014894278197971, 281.6198905683720000, -11.84573899990672707 ) ) ;
#4947=CARTESIAN_POINT ( 'NONE',  ( -32.01814843081345430, 503.1823905683721136, -16.75240474999999307 ) ) ;
#4949=CARTESIAN_POINT ( 'NONE',  ( -24.70764059509556176, 364.4323905601784759, -19.99999999999999289 ) ) ;
#4952=CARTESIAN_POINT ( 'NONE',  ( -45.43829269268871940, 485.0573905683720568, -3.332260488124726194 ) ) ;
#4954=CARTESIAN_POINT ( 'NONE',  ( -16.84014894278197971, 280.1198905683720000, -11.84573899990672707 ) ) ;
#4955=ORIENTED_EDGE ( 'NONE', *, *, #18846, .T. ) ;
#4957=CARTESIAN_POINT ( 'NONE',  ( -45.43829269268870519, 285.3698905683720568, 0.000000000000000000 ) ) ;
#4960=CARTESIAN_POINT ( 'NONE',  ( -21.03221929538690915, 248.8698905765656093, -18.47759065022572855 ) ) ;
#4963=CARTESIAN_POINT ( 'NONE',  ( -13.20868407381884957, 269.4948905683720000, -6.410867750099233042 ) ) ;
#4965=CARTESIAN_POINT ( 'NONE',  ( -40.53162694259543741, 386.6198905683720568, 11.84573899990672885 ) ) ;
#4967=CARTESIAN_POINT ( 'NONE',  ( -8.685887942688733432, 456.9948905765656377, -2.449293598294705724E-15 ) ) ;
#4968=CARTESIAN_POINT ( 'NONE',  ( -47.16347859291443712, 271.3698905765656377, -7.653668647301793193 ) ) ;
#4969=CARTESIAN_POINT ( 'NONE',  ( -45.43829269268871940, 423.8698905683720568, 0.000000000000000000 ) ) ;
#4972=CARTESIAN_POINT ( 'NONE',  ( -8.685887942688728103, 422.2448905601784759, -2.449293598294705724E-15 ) ) ;
#4976=CARTESIAN_POINT ( 'NONE',  ( -8.685887942688715668, 302.5573905601784759, -3.978247347593165895 ) ) ;
#4977=FACE_OUTER_BOUND ( 'NONE', #1089, .T. ) ;
#4978=CARTESIAN_POINT ( 'NONE',  ( -22.27502019258948707, 352.2448905683720000, -15.47720386886985544 ) ) ;
#4979=ORIENTED_EDGE ( 'NONE', *, *, #9999, .T. ) ;
#4980=CARTESIAN_POINT ( 'NONE',  ( -11.73070664223726567, 487.9323905765656377, -11.32908994701042715 ) ) ;
#4981=CARTESIAN_POINT ( 'NONE',  ( -42.88789093042843348, 362.9323905683720568, -9.489475012073736337 ) ) ;
#4983=CARTESIAN_POINT ( 'NONE',  ( -11.93348319268872260, 379.1823905683721136, -3.332260488124732856 ) ) ;
#4984=CARTESIAN_POINT ( 'NONE',  ( -40.01497788969913216, 300.4323905765656377, -16.95518130045146421 ) ) ;
#4986=CARTESIAN_POINT ( 'NONE',  ( -35.09675569278794427, 285.7448905683720568, 15.47720386886985366 ) ) ;
#4988=ADVANCED_FACE ( 'NONE', ( #5654 ), #12475, .T. ) ;
#4989=CARTESIAN_POINT ( 'NONE',  ( -45.43829269268871940, 435.3698905683720000, 0.000000000000000000 ) ) ;
#4992=CARTESIAN_POINT ( 'NONE',  ( -24.70764059509556532, 500.0573905601785896, 19.99999999999998934 ) ) ;
#4993=LINE ( 'NONE', #3056, #9879 ) ;
#4995=CARTESIAN_POINT ( 'NONE',  ( -22.27502019258947641, 348.4948905683720000, 15.47720386886985189 ) ) ;
#4996=CARTESIAN_POINT ( 'NONE',  ( -40.53162694259545162, 475.1198905683720000, 11.84573899990672885 ) ) ;
#4998=CARTESIAN_POINT ( 'NONE',  ( -17.35679799567830628, 480.6823905601784759, 16.95518130045146421 ) ) ;
#4999=CARTESIAN_POINT ( 'NONE',  ( -28.68588794268870501, 306.3698905683720568, 16.75240474999999307 ) ) ;
#5003=FACE_OUTER_BOUND ( 'NONE', #14285, .T. ) ;
#5004=CARTESIAN_POINT ( 'NONE',  ( -45.43829269268871940, 395.3698905683720000, 0.000000000000000000 ) ) ;
#5006=CARTESIAN_POINT ( 'NONE',  ( -11.73070664223724968, 386.0573905765656946, 11.32908994701042005 ) ) ;
#5007=CARTESIAN_POINT ( 'NONE',  ( -32.01814843081345430, 431.6823905683720000, -16.75240474999999307 ) ) ;
#5008=CARTESIAN_POINT ( 'NONE',  ( -44.16309181155857999, 454.4948905683720568, 6.410867750099241924 ) ) ;
#5011=CARTESIAN_POINT ( 'NONE',  ( -10.20829729246298712, 366.3698905765655809, 7.653668647301790529 ) ) ;
#5013=CARTESIAN_POINT ( 'NONE',  ( -40.01497788969912506, 265.6823905601785327, -16.95518130045146421 ) ) ;
#5016=CARTESIAN_POINT ( 'NONE',  ( -35.09675569278796559, 497.2448905683720000, 15.47720386886985366 ) ) ;
#5018=CARTESIAN_POINT ( 'NONE',  ( -48.68588794268857356, 466.9323905601784759, -3.978247347593530936 ) ) ;
#5020=CARTESIAN_POINT ( 'NONE',  ( -19.19641293061498644, 398.8073905683720568, 14.20200298773971426 ) ) ;
#5022=( BOUNDED_SURFACE ( )  B_SPLINE_SURFACE ( 1, 2, ( 
 ( #13475, #9991, #75, #19849, #15208, #8585, #6642, #10206, #18436, #15318, #8374, #13586, #7065, #20068, #5447, #288, #2219, #18637, #13684, #3724, #183, #2017, #16829, #5137, #10308, #13263, #503, #397, #16933, #14997, #2115, #3623, #6964, #5026, #19959, #8694, #20277, #10103, #12048, #3828, #1805, #18221, #20175, #5341, #11627, #3414, #16725, #11736, #18326, #16615, #10416, #6751, #5240, #11942, #13369, #17037, #14888, #3516, #1913, #8481, #15104, #6857, #11840, #2325, #18851, #2639, #819, #4143, #17247, #12372, #17351, #2534, #707, #10848, #5763, #15524, #4040, #5553, #9117, #9011, #15844, #603, #9226, #10738, #7490, #7386, #12159, #7278, #13901, #10950, #19078, #15738, #15418, #20491, #10629, #5662, #926, #5984, #12267, #18747, #8904, #7595, #3935, #20592, #2430, #13791, #20812, #8801, #15634, #12593, #10521, #12485, #7168, #14012, #17143, #4260, #1031, #20380, #14226, #18962, #14115, #20701, #5874, #17452, #19186, #4364, #17560, #6757, #82, #5453, #5246, #15213, #16622, #17045, #8487, #1812, #13375, #16732, #6863, #18333, #8380, #11846, #8590, #13269, #6969, #3420, #7071, #18443, #404, #5144, #18542, #12055, #9998, #15004, #19855, #10110, #16834, #3629, #3523, #190, #1919, #10423, #11742, #15110, #13691, #13482, #19965, #15323, #294, #2226, #8807, #20075, #10211, #6648, #5032, #2022, #18643, #11633, #13592, #20179, #5347, #11948, #3729, #16938, #10314, #2120, #18228, #8701, #508, #20283, #3835, #17458, #7285, #609, #932, #9123, #2758, #2647, #3942, #13908, #10744, #20598, #12378, #4267, #10527, #14232, #4152, #10854, #14019, #17254, #17358, #15532, #20498, #9233, #18971, #713, #10636, #12166, #15745, #15640, #1037, #7174, #15853, #2540, #12494, #18857, #5990, #2330, #19084, #7601, #12600, #13796, #20387, #826, #7498, #19192, #14121, #5668, #20820, #5561, #20708, #8911, #4371, #2437, #12276, #5881, #10957, #17566, #15424, #18754, #4047, #17149, #9018, #7392, #5771, #4787, #14545, #6196, #4684, #6304, #1452, #7713, #9447, #19400, #3181, #17877, #19294, #13130, #7917, #4480, #15956, #14342, #9654, #3070, #1142, #11279, #12916, #9760, #2864, #8025, #1559, #21131, #21346, #16168, #18094, #19717, #8129, #13018, #16065, #16275, #14658, #21026, #19610, #20922, #16384, #21239, #11384, #1241, #17982, #19506, #6405, #6089, #14446, #14761, #6514, #4583, #4900, #11497, #17670, #12703, #9335, #11063, #7815, #12808, #11175, #17777, #2970, #9548, #1344, #19832, #15084, #18413, #9863, #372, #20043, #6836, #13242, #5007, #3703, #3289, #16703, #18198, #13348, #18517, #1892, #5220, #11714, #13452, #11819, #3602, #10186, #6942, #6733, #15297, #11607, #13566, #20154, #484, #16489, #1671, #10082, #16807, #7048, #1997, #14975, #5322, #8240, #8566, #3395, #2092, #18306, #8351, #15187, #11923, #10291, #8673, #16912, #19936, #13668, #6621, #9975, #5428, #20257, #8459, #162, #12028, #269, #14871, #50, #16594, #5114, #1783, #3495, #7151, #1013, #17230, #13772, #3807, #2199, #18942, #12355, #10398, #13994, #801, #19061, #12141, #17333, #10828, #2413, #9203, #4019, #5962, #7579, #17438, #905, #3915, #5744, #20576, #8888, #7470, #17017, #4243, #4127, #14100, #18727, #20681, #7367, #10715, #8784, #2305, #5856, #12463, #13883, #2622, #15829, #5536, #583, #2516, #9100, #15400, #20361, #20474, #15505, #690, #10505, #14206, #17126, #8993, #15721, #7258, #20795, #18620, #5643, #12251, #18834, #10612, #15614, #4561, #6066, #1220, #6381, #11148, #7893, #21004, #16141, #21106, #6278, #4451, #14631, #9523, #19271, #7790, #9312, #12892, #12782, #19583, #4348, #12990, #15929, #12677, #11358, #7689, #2944, #11037, #17541, #3155, #12576, #19376, #16356, #1118, #16248, #10931, #17753, #14319, #7999, #4763, #2732, #17955, #14423, #20898, #1322, #17648, #2840, #9422, #19170, #9734, #16042, #6172, #1533, #14521, #19482, #4662, #8103, #11253, #17852, #3046, #9629, #1427, #21216, #14733, #21315, #15058, #19688, #13427, #9837, #13539, #11689, #241, #11580, #3576, #18491, #16460, #1643, #4874, #16568, #1865, #18280, #9948, #8215, #1754, #16884, #18171, #8326, #20128, #13324, #19, #350, #14843, #2068, #8643, #3369, #13216, #15271, #13103, #6595, #11898, #11468, #4981, #14948, #134, #6707, #19801, #1968, #20018, #5194, #6486, #19907, #15162, #11791, #18066, #8540, #5088, #3261, #18387, #6811, #3468, #6913, #10055, #16678, #8436, #10165, #16783, #5295, #3680, #10264, #10581, #17307, #20444, #2278, #17204, #555, #20553, #13853, #18594, #20336, #13750, #2598, #10688, #2383, #7020, #5508, #10477, #12109, #8966, #19033, #7124, #5617, #8858, #15590, #18702, #5719, #12225, #3779, #3888, #17099, #9178, #2492, #773, #13643, #15479, #664, #7230, #7337, #4218, #18808, #10369, #15377, #20656, #16994, #3990, #13970, #5399, #12436, #455, #12327, #10801, #2172, #4100, #20229, #18915, #8757, #9073, #15694, #12004, #14071, #881, #7445, #5826, #17416, #20770, #1096, #990, #7977, #7664, #15803, #21187, #20979, #9502, #10906, #11336, #2814, #17517, #14292, #11013, #1198, #12652, #2708, #6147, #2922, #7554, #1294, #19146, #1401, #12759, #16116, #20878, #12865, #6358, #4323, #9289, #14179, #4429, #11122, #19348, #19246, #15905, #17622, #4739, #6043, #9397, #14604, #7769, #16016, #9605, #14395, #17931, #3127, #4536, #17727, #5937, #12552, #7870, #12968, #14499, #21082, #6254, #19455, #4638, #11232, #17829, #3023, #16224, #19559, #1507, #4842, #13077, #9712, #11441, #8082, #16332, #18041, #14712, #21289, #6461, #19664, #576, #4013, #13879, #5639, #18938, #3802, #7465, #18830, #4121, #10394, #11119, #10709, #20469, #5531, #10607, #12247, #797, #7044, #8779, #18723, #2512, #17225, #18616, #12456, #7252, #17013, #15293, #13663, #8988, #2407, #480, #15610, #7362, #9097, #2195, #13990, #901, #20572, #20676, #15500, #17722, #19056, #14095, #12349, #15396, #5739, #17329, #20356, #15716, #20251, #5851, #4239, #8669, #7145, #5423, #12024, #13769, #12136, #3911, #10501, #17121, #2300, #8882, #685, #11229, #6251, #1611, #11438, #16112, #1290, #4736, #14601, #7972, #19452, #16538, #4635, #14708, #18038, #9499, #10383, #19658, #6458, #12862, #17826, #3337, #2919, #16328, #3019, #12965, #18142, #1504, #4838, #11332, #13074, #3233, #9810, #16220, #4954, #21285, #9602, #19555, #21077, #16433, #3124, #9919, #7867, #1723, #8184, #6563, #6355, #14920, #1397, #13184, #19768, #103, #14496, #21184, #9708, #14814, #6676, #11553, #17927, #8295, #8079, #13295, #19880, #5057, #11660, #1944, #6995, #8725, #11974, #17071, #10450, #320, #634, #215, #16653, #2253, #13508, #1835, #2043, #8407, #15031, #3550, #3443, #8830, #10137, #18251, #15451, #8614, #18571, #13402, #13823, #5270, #19989, #16757, #20101, #3654, #15139, #5169, #15239, #5369, #10027, #3753, #6782, #3860, #429, #10341, #8512, #15352, #7200, #11765, #18360, #6889, #11875, #13617, #20204, #18465, #10236, #16861, #20416, #16965, #2145, #5588, #533, #7098, #12080, #13717, #20310, #5480, #18671, #18888, #1167, #18781, #15560, #17592, #10555, #10660, #20625, #9044, #15666, #7310, #7635, #19113, #4295, #14369, #12299, #20846, #10879, #17177, #14260, #4074, #3965, #17484, #5909, #20948, #6017, #745, #17278, #7524, #17385, #9148, #1065, #13937, #10983, #960, #12626, #10770, #14043, #14149, #2464, #2674, #4183, #8935, #852, #7417, #12193, #19217, #20736, #2357, #5800, #12406, #18998, #12519, #15986, #2568, #20527, #5692, #2784, #15770, #9260, #15877, #4400, #7740, #6120, #6331, #9892, #9475, #9784, #19319, #11306, #16086, #1586, #21371, #18117, #14471, #16408, #8156, #3313, #4505, #11094, #12944, #21262, #16515, #6429, #17803, #14786, #17698, #16304, #21052, #4928, #14574, #11204, #1476, #18013, #13045, #11525, #19744, #9577 ),
 ( #1265, #6539, #2892, #17902, #7842, #13156, #1696, #6222, #8265, #1372, #12837, #3097, #19426, #4611, #2993, #16193, #14896, #7942, #21158, #19531, #9680, #19634, #4709, #8053, #14685, #4814, #11408, #3206, #12306, #2365, #7208, #17287, #14051, #18680, #12415, #8838, #12528, #10669, #20635, #10562, #2579, #17495, #15459, #642, #3867, #15567, #860, #2471, #8944, #13830, #753, #16177, #17185, #7318, #19123, #18896, #20424, #20745, #5597, #1354, #7927, #13946, #12201, #14556, #12088, #18788, #10888, #10457, #3972, #20533, #5700, #4082, #9052, #969, #19010, #15675, #5919, #5808, #7424, #9270, #4193, #10779, #17077, #17396, #9158, #15782, #7533, #14159, #4305, #2685, #5488, #19841, #13358, #19727, #11724, #6521, #8470, #3506, #19947, #3403, #6413, #8250, #16497, #11392, #9983, #6314, #6742, #14879, #16605, #21248, #1794, #9872, #62, #12928, #4796, #8362, #14985, #16394, #172, #5124, #8037, #3079, #5016, #6631, #19515, #4694, #1568, #17993, #3190, #16286, #18316, #1462, #11506, #13251, #11288, #18207, #1679, #3299, #9662, #14668, #10092, #21143, #13138, #13027, #9768, #16713, #4910, #11616, #8138, #1903, #17886, #19619, #14769, #21355, #18104, #383, #10298, #11830, #591, #15305, #697, #6847, #8895, #17025, #12148, #18525, #5651, #2007, #18737, #10511, #12257, #13462, #279, #491, #8791, #18840, #7158, #5331, #3921, #20055, #3815, #8575, #13890, #2103, #20164, #10407, #5542, #13780, #20480, #7266, #3711, #4028, #18424, #15198, #17236, #17133, #20264, #11932, #2205, #12036, #20368, #5231, #6953, #18627, #2314, #10196, #10620, #15513, #2420, #13674, #16922, #15094, #13576, #3611, #7056, #8681, #5435, #915, #11156, #19277, #4354, #15621, #7477, #19068, #14106, #10938, #6179, #15728, #5752, #2524, #7797, #4133, #20801, #20690, #14003, #21011, #9000, #9213, #12789, #12362, #12684, #809, #14214, #18952, #4460, #2846, #7375, #1226, #4250, #20582, #5971, #10725, #17339, #5864, #9107, #14430, #12472, #10837, #19382, #12582, #2739, #17443, #4567, #2630, #15834, #1021, #7585, #19176, #17549, #9320, #15937, #1125, #7696, #14325, #20905, #16048, #6072, #11044, #17654, #9430, #17760, #6285, #12899, #16148, #12999, #19695, #14742, #6388, #19489, #19591, #13332, #14639, #4770, #9954, #9741, #17859, #18179, #4669, #19914, #5095, #21224, #9637, #11696, #9530, #11260, #8332, #1328, #1435, #11365, #17961, #3163, #3053, #19812, #9844, #16468, #2951, #16257, #11587, #1651, #7900, #4989, #8005, #14528, #8223, #18074, #21113, #3377, #16362, #1540, #4881, #8111, #21326, #6494, #14955, #13111, #11477, #6715, #3269, #6602, #14852, #27, #13224, #16576, #1763, #141, #10484, #13545, #16685, #2074, #8442, #1872, #3582, #3476, #17105, #10170, #18288, #2285, #8652, #12011, #13433, #13863, #5303, #20026, #16790, #20136, #3686, #15168, #5201, #15279, #5406, #10062, #3787, #249, #3896, #462, #18603, #1977, #15384, #8865, #6818, #11798, #15066, #6921, #13650, #7028, #357, #18395, #11904, #7236, #8548, #18497, #15485, #10273, #16892, #12119, #20235, #20451, #5623, #10378, #17000, #2180, #8764, #563, #670, #7130, #13757, #20342, #5517, #18708, #7344, #7672, #19154, #4329, #14402, #12334, #20882, #10911, #10589, #14299, #4106, #18815, #17523, #5943, #20983, #6049, #782, #10695, #7559, #17422, #9185, #1101, #13977, #11017, #996, #12657, #10808, #14079, #14186, #18922, #2714, #4226, #8972, #17315, #2498, #12233, #19251, #20778, #3996, #9081, #888, #15701, #12560, #9403, #7451, #15597, #5726, #17627, #20559, #2604, #20662, #17210, #2390, #9295, #15909, #5833, #4434, #15810, #2819, #12442, #16022, #1203, #7773, #19041, #12973, #14932, #9928, #4965, #9818, #12872, #14716, #1513, #17834, #16442, #12764, #13197, #21294, #1621, #6259, #8195, #16338, #6466, #19353, #11236, #14823, #2, #1406, #6575, #19778, #14504, #9506, #4849, #13083, #4543, #11127, #7983, #3029, #9612, #1302, #11563, #7874, #17937, #19669, #17733, #3243, #8086, #9718, #16121, #21086, #18150, #6151, #19563, #19462, #16229, #3348, #4744, #11447, #14611, #18048, #16548, #1733, #4645, #8307, #3132, #21196, #6363, #2926, #11342, #330, #7109, #13306, #15362, #2052, #18579, #3560, #12092, #8418, #3765, #16975, #18683, #19891, #6688, #6897, #15250, #3872, #436, #11774, #10352, #5067, #10245, #15041, #20319, #8522, #5177, #16870, #11985, #7003, #5491, #13729, #10150, #10460, #3452, #1848, #2263, #2157, #5279, #18371, #8626, #18475, #13627, #11671, #225, #16766, #542, #20214, #10037, #17081, #20110, #8737, #18261, #8841, #5379, #114, #6792, #16663, #13410, #19999, #1953, #15148, #13519, #11884, #3662, #17498, #1077, #2368, #18793, #14163, #2583, #7211, #13833, #17289, #5703, #20537, #10565, #7648, #17188, #5811, #9161, #645, #12532, #10783, #19013, #3975, #8947, #15889, #15462, #7427, #15570, #4085, #9273, #14054, #17399, #2474, #4196, #15785, #972, #7322, #2688, #12419, #756, #10672, #12204, #7536, #15678, #14275, #20427, #20858, #20748, #19126, #18899, #6028, #13949, #4308, #10891, #12638, #5600, #12309, #864, #5922, #19230, #4413, #9057, #10996, #20638, #17605, #2796, #8172, #17816, #14484, #19544, #21273, #3112, #14802, #1598, #12848, #13171, #12741, #11106, #11540, #4827, #14588, #6236, #4724, #6343, #1491, #7751, #9488, #19439, #3220, #17915, #19332, #19757, #7958, #4518, #16000, #14380, #9695, #16316, #1181, #11320, #12955, #9798, #2905, #8066, #21386, #21172, #6552, #16207, #18131, #4941, #9382, #13061, #16098, #14696, #6444, #21064, #20962, #17710, #1277, #6133, #11424, #19647, #4622, #18026, #16420, #7855, #11217, #3006, #9591, #1385, #11859, #13284, #7083, #1932, #19869, #9906, #8279, #3642, #18454, #16527, #20089, #6876, #3740, #18240, #2033, #16950, #8499, #15338, #10124, #12067, #13704, #2132, #6983, #10013, #10223, #5259, #15018, #13603, #1711, #10328, #16848, #20189, #3432, #5358, #13496, #8601, #14910, #8393, #11960, #18557, #19977, #8713, #521, #11646, #6663, #15224, #417, #93, #5045, #5157, #202, #6769, #16638, #20297, #1823, #15125, #5467, #13390, #3324, #11753, #18349, #3536, #16745, #307, #18657, #12288, #5576, #15547, #9136, #5681, #2451, #7298, #10646, #15655, #841, #18767, #17373, #17266, #12181, #729, #15436, #7405, #13924, #945, #10437, #15757, #9029, #12391, #8923, #20721, #20401, #18985, #2555, #5896, #17058, #3849, #18872, #20611, #4282, #5787, #20512, #7512, #8819, #14031, #3955, #12506, #4062, #4166, #10758, #14135, #19099, #2241, #624, #7187, #2343, #13810, #10542, #17162, #13669, #11924, #20155, #5115, #18307, #17018, #16595, #8567, #10083, #5221, #10399, #15188, #18518, #3603, #5323, #3704, #10292, #8460, #18621, #13567, #1893, #11820, #13349, #16913, #16808, #2200, #8352, #8785, #2093, #20258, #20044, #7152, #3496, #5429, #12029, #13773, #14976, #1784, #1998, #8674, #20362, #15298, #6837, #3808, #163, #485, #16704, #15401, #10187, #270, #7049, #584, #5537, #12142, #18728, #18414, #3916, #19937, #15085, #6734, #11715, #373, #13453, #6943, #7471, #2623, #8889, #10613, #20577, #4349, #19062, #20475, #14320, #9101, #5644, #17127, #15506, #10829, #4244, #2306, #5857, #14101, #10932, #4020, #9204, #2733, #15722, #1119, #17334, #19272, #20899, #9313, #14207, #17231, #17439, #12464, #802, #20796, #691, #17542, #15830, #5963, #2414, #12577, #20682, #1014, #7259, #15615, #19171, #15930, #5745, #7690, #6067, #18835, #13884, #7580, #12678, #12252, #8994, #12356, #7368, #13995, #18943, #10506, #4128, #10716, #2517, #906, #9630, #1428, #14734, #21005, #3262, #14632, #21316, #3047, #6279, #21217, #4562, #3156, #17853, #1221, #2945, #17754, #6596, #6487, #6382, #11038, #9524, #14522, #16142, #12991, #1644, #11149, #7791, #19377, #9838, #6173 ) ),
 .UNSPECIFIED., .F., .F., .T. ) 
 B_SPLINE_SURFACE_WITH_KNOTS ( ( 2, 2 ),
 ( 3, 2, 2, 2, 2, 2, 2, 2, 2, 2, 2, 2, 2, 2, 2, 2, 2, 2, 2, 2, 2, 2, 2, 2, 2, 2, 2, 2, 2, 2, 2, 2, 2, 2, 2, 2, 2, 2, 2, 2, 2, 2, 2, 2, 2, 2, 2, 2, 2, 2, 2, 2, 2, 2, 2, 2, 2, 2, 2, 2, 2, 2, 2, 2, 2, 2, 2, 2, 2, 2, 2, 2, 2, 2, 2, 2, 2, 2, 2, 2, 2, 2, 2, 2, 2, 2, 2, 2, 2, 2, 2, 2, 2, 2, 2, 2, 2, 2, 2, 2, 2, 2, 2, 2, 2, 2, 2, 2, 2, 2, 2, 2, 2, 2, 2, 2, 2, 2, 2, 2, 2, 2, 2, 2, 2, 2, 2, 2, 2, 2, 2, 2, 2, 2, 2, 2, 2, 2, 2, 2, 2, 2, 2, 2, 2, 2, 2, 2, 2, 2, 2, 2, 2, 2, 2, 2, 2, 2, 2, 2, 2, 2, 2, 2, 2, 2, 2, 2, 2, 2, 2, 2, 2, 2, 2, 2, 2, 2, 2, 2, 2, 2, 2, 2, 2, 2, 2, 2, 2, 2, 2, 2, 2, 2, 2, 2, 2, 2, 2, 2, 2, 2, 2, 2, 2, 2, 2, 2, 2, 2, 2, 2, 2, 2, 2, 2, 2, 2, 2, 2, 2, 2, 2, 2, 2, 2, 2, 2, 2, 2, 2, 2, 2, 2, 2, 2, 2, 2, 2, 2, 2, 2, 2, 2, 2, 2, 2, 2, 2, 2, 2, 2, 2, 2, 2, 2, 2, 2, 2, 2, 2, 2, 2, 2, 2, 2, 2, 2, 2, 2, 2, 2, 2, 2, 2, 2, 2, 2, 2, 2, 2, 2, 2, 2, 2, 2, 2, 2, 2, 2, 2, 2, 2, 2, 2, 2, 2, 2, 2, 2, 2, 2, 2, 2, 2, 2, 2, 2, 2, 2, 2, 2, 2, 2, 2, 2, 2, 2, 2, 2, 2, 2, 2, 2, 2, 2, 2, 2, 2, 2, 2, 2, 2, 2, 2, 2, 2, 2, 2, 2, 2, 2, 2, 2, 2, 2, 2, 2, 2, 2, 2, 2, 2, 2, 2, 2, 2, 2, 2, 2, 2, 2, 2, 2, 2, 2, 2, 2, 2, 2, 2, 2, 2, 2, 2, 2, 2, 2, 2, 2, 2, 2, 2, 2, 2, 2, 2, 2, 2, 2, 2, 2, 2, 2, 2, 2, 2, 2, 2, 2, 2, 2, 2, 2, 2, 2, 2, 2, 2, 2, 2, 2, 2, 2, 2, 2, 2, 2, 2, 2, 2, 2, 2, 2, 2, 2, 2, 2, 2, 2, 2, 2, 2, 2, 2, 2, 2, 2, 2, 2, 2, 2, 2, 2, 2, 2, 2, 2, 2, 2, 2, 2, 2, 2, 2, 2, 2, 2, 2, 2, 2, 2, 2, 2, 2, 2, 2, 2, 2, 2, 2, 2, 2, 2, 2, 2, 2, 2, 2, 2, 2, 2, 2, 2, 2, 2, 2, 2, 2, 2, 2, 2, 2, 2, 2, 2, 2, 2, 2, 2, 2, 2, 3 ),
 ( 0.000000000000000000, 1.000000000000000000 ),
 ( 0.000000000000000000, 0.001953125000000000000, 0.003906250000000000000, 0.005859375000000000000, 0.007812500000000000000, 0.009765625000000000000, 0.01171875000000000000, 0.01367187500000000000, 0.01562500000000000000, 0.01757812500000000000, 0.01953125000000000000, 0.02148437500000000000, 0.02343750000000000000, 0.02539062500000000000, 0.02734375000000000000, 0.02929687500000000000, 0.03125000000000000000, 0.03320312500000000000, 0.03515625000000000000, 0.03710937500000000000, 0.03906250000000000000, 0.04101562500000000000, 0.04296875000000000000, 0.04492187500000000000, 0.04687500000000000000, 0.04882812500000000000, 0.05078125000000000000, 0.05273437500000000000, 0.05468750000000000000, 0.05664062500000000000, 0.05859375000000000000, 0.06054687500000000000, 0.06250000000000000000, 0.06445312500000000000, 0.06640625000000000000, 0.06835937500000000000, 0.07031250000000000000, 0.07226562500000000000, 0.07421875000000000000, 0.07617187500000000000, 0.07812500000000000000, 0.08007812500000000000, 0.08203125000000000000, 0.08398437500000000000, 0.08593750000000000000, 0.08789062500000000000, 0.08984375000000000000, 0.09179687500000000000, 0.09375000000000000000, 0.09570312500000000000, 0.09765625000000000000, 0.09960937500000000000, 0.1015625000000000000, 0.1035156250000000000, 0.1054687500000000000, 0.1074218750000000000, 0.1093750000000000000, 0.1113281250000000000, 0.1132812500000000000, 0.1152343750000000000, 0.1171875000000000000, 0.1191406250000000000, 0.1210937500000000000, 0.1230468750000000000, 0.1250000000000000000, 0.1269531250000000000, 0.1289062500000000000, 0.1308593750000000000, 0.1328125000000000000, 0.1347656250000000000, 0.1367187500000000000, 0.1386718750000000000, 0.1406250000000000000, 0.1425781250000000000, 0.1445312500000000000, 0.1464843750000000000, 0.1484375000000000000, 0.1503906250000000000, 0.1523437500000000000, 0.1542968750000000000, 0.1562500000000000000, 0.1582031250000000000, 0.1601562500000000000, 0.1621093750000000000, 0.1640625000000000000, 0.1660156250000000000, 0.1679687500000000000, 0.1699218750000000000, 0.1718750000000000000, 0.1738281250000000000, 0.1757812500000000000, 0.1777343750000000000, 0.1796875000000000000, 0.1816406250000000000, 0.1835937500000000000, 0.1855468750000000000, 0.1875000000000000000, 0.1894531250000000000, 0.1914062500000000000, 0.1933593750000000000, 0.1953125000000000000, 0.1972656250000000000, 0.1992187500000000000, 0.2011718750000000000, 0.2031250000000000000, 0.2050781250000000000, 0.2070312500000000000, 0.2089843750000000000, 0.2109375000000000000, 0.2128906250000000000, 0.2148437500000000000, 0.2167968750000000000, 0.2187500000000000000, 0.2207031250000000000, 0.2226562500000000000, 0.2246093750000000000, 0.2265625000000000000, 0.2285156250000000000, 0.2304687500000000000, 0.2324218750000000000, 0.2343750000000000000, 0.2363281250000000000, 0.2382812500000000000, 0.2402343750000000000, 0.2421875000000000000, 0.2441406250000000000, 0.2460937500000000000, 0.2480468750000000000, 0.2500000000000000000, 0.2519531250000000000, 0.2539062500000000000, 0.2558593750000000000, 0.2578125000000000000, 0.2597656250000000000, 0.2617187500000000000, 0.2636718750000000000, 0.2656250000000000000, 0.2675781250000000000, 0.2695312500000000000, 0.2714843750000000000, 0.2734375000000000000, 0.2753906250000000000, 0.2773437500000000000, 0.2792968750000000000, 0.2812500000000000000, 0.2832031250000000000, 0.2851562500000000000, 0.2871093750000000000, 0.2890625000000000000, 0.2910156250000000000, 0.2929687500000000000, 0.2949218750000000000, 0.2968750000000000000, 0.2988281250000000000, 0.3007812500000000000, 0.3027343750000000000, 0.3046875000000000000, 0.3066406250000000000, 0.3085937500000000000, 0.3105468750000000000, 0.3125000000000000000, 0.3144531250000000000, 0.3164062500000000000, 0.3183593750000000000, 0.3203125000000000000, 0.3222656250000000000, 0.3242187500000000000, 0.3261718750000000000, 0.3281250000000000000, 0.3300781250000000000, 0.3320312500000000000, 0.3339843750000000000, 0.3359375000000000000, 0.3378906250000000000, 0.3398437500000000000, 0.3417968750000000000, 0.3437500000000000000, 0.3457031250000000000, 0.3476562500000000000, 0.3496093750000000000, 0.3515625000000000000, 0.3535156250000000000, 0.3554687500000000000, 0.3574218750000000000, 0.3593750000000000000, 0.3613281250000000000, 0.3632812500000000000, 0.3652343750000000000, 0.3671875000000000000, 0.3691406250000000000, 0.3710937500000000000, 0.3730468750000000000, 0.3750000000000000000, 0.3769531250000000000, 0.3789062500000000000, 0.3808593750000000000, 0.3828125000000000000, 0.3847656250000000000, 0.3867187500000000000, 0.3886718750000000000, 0.3906250000000000000, 0.3925781250000000000, 0.3945312500000000000, 0.3964843750000000000, 0.3984375000000000000, 0.4003906250000000000, 0.4023437500000000000, 0.4042968750000000000, 0.4062500000000000000, 0.4082031250000000000, 0.4101562500000000000, 0.4121093750000000000, 0.4140625000000000000, 0.4160156250000000000, 0.4179687500000000000, 0.4199218750000000000, 0.4218750000000000000, 0.4238281250000000000, 0.4257812500000000000, 0.4277343750000000000, 0.4296875000000000000, 0.4316406250000000000, 0.4335937500000000000, 0.4355468750000000000, 0.4375000000000000000, 0.4394531250000000000, 0.4414062500000000000, 0.4433593750000000000, 0.4453125000000000000, 0.4472656250000000000, 0.4492187500000000000, 0.4511718750000000000, 0.4531250000000000000, 0.4550781250000000000, 0.4570312500000000000, 0.4589843750000000000, 0.4609375000000000000, 0.4628906250000000000, 0.4648437500000000000, 0.4667968750000000000, 0.4687500000000000000, 0.4707031250000000000, 0.4726562500000000000, 0.4746093750000000000, 0.4765625000000000000, 0.4785156250000000000, 0.4804687500000000000, 0.4824218750000000000, 0.4843750000000000000, 0.4863281250000000000, 0.4882812500000000000, 0.4902343750000000000, 0.4921875000000000000, 0.4941406250000000000, 0.4960937500000000000, 0.4980468750000000000, 0.5000000000000000000, 0.5019531250000000000, 0.5039062500000000000, 0.5058593750000000000, 0.5078125000000000000, 0.5097656250000000000, 0.5117187500000000000, 0.5136718750000000000, 0.5156250000000000000, 0.5175781250000000000, 0.5195312500000000000, 0.5214843750000000000, 0.5234375000000000000, 0.5253906250000000000, 0.5273437500000000000, 0.5292968750000000000, 0.5312500000000000000, 0.5332031250000000000, 0.5351562500000000000, 0.5371093750000000000, 0.5390625000000000000, 0.5410156250000000000, 0.5429687500000000000, 0.5449218750000000000, 0.5468750000000000000, 0.5488281250000000000, 0.5507812500000000000, 0.5527343750000000000, 0.5546875000000000000, 0.5566406250000000000, 0.5585937500000000000, 0.5605468750000000000, 0.5625000000000000000, 0.5644531250000000000, 0.5664062500000000000, 0.5683593750000000000, 0.5703125000000000000, 0.5722656250000000000, 0.5742187500000000000, 0.5761718750000000000, 0.5781250000000000000, 0.5800781250000000000, 0.5820312500000000000, 0.5839843750000000000, 0.5859375000000000000, 0.5878906250000000000, 0.5898437500000000000, 0.5917968750000000000, 0.5937500000000000000, 0.5957031250000000000, 0.5976562500000000000, 0.5996093750000000000, 0.6015625000000000000, 0.6035156250000000000, 0.6054687500000000000, 0.6074218750000000000, 0.6093750000000000000, 0.6113281250000000000, 0.6132812500000000000, 0.6152343750000000000, 0.6171875000000000000, 0.6191406250000000000, 0.6210937500000000000, 0.6230468750000000000, 0.6250000000000000000, 0.6269531250000000000, 0.6289062500000000000, 0.6308593750000000000, 0.6328125000000000000, 0.6347656250000000000, 0.6367187500000000000, 0.6386718750000000000, 0.6406250000000000000, 0.6425781250000000000, 0.6445312500000000000, 0.6464843750000000000, 0.6484375000000000000, 0.6503906250000000000, 0.6523437500000000000, 0.6542968750000000000, 0.6562500000000000000, 0.6582031250000000000, 0.6601562500000000000, 0.6621093750000000000, 0.6640625000000000000, 0.6660156250000000000, 0.6679687500000000000, 0.6699218750000000000, 0.6718750000000000000, 0.6738281250000000000, 0.6757812500000000000, 0.6777343750000000000, 0.6796875000000000000, 0.6816406250000000000, 0.6835937500000000000, 0.6855468750000000000, 0.6875000000000000000, 0.6894531250000000000, 0.6914062500000000000, 0.6933593750000000000, 0.6953125000000000000, 0.6972656250000000000, 0.6992187500000000000, 0.7011718750000000000, 0.7031250000000000000, 0.7050781250000000000, 0.7070312500000000000, 0.7089843750000000000, 0.7109375000000000000, 0.7128906250000000000, 0.7148437500000000000, 0.7167968750000000000, 0.7187500000000000000, 0.7207031250000000000, 0.7226562500000000000, 0.7246093750000000000, 0.7265625000000000000, 0.7285156250000000000, 0.7304687500000000000, 0.7324218750000000000, 0.7343750000000000000, 0.7363281250000000000, 0.7382812500000000000, 0.7402343750000000000, 0.7421875000000000000, 0.7441406250000000000, 0.7460937500000000000, 0.7480468750000000000, 0.7500000000000000000, 0.7519531250000000000, 0.7539062500000000000, 0.7558593750000000000, 0.7578125000000000000, 0.7597656250000000000, 0.7617187500000000000, 0.7636718750000000000, 0.7656250000000000000, 0.7675781250000000000, 0.7695312500000000000, 0.7714843750000000000, 0.7734375000000000000, 0.7753906250000000000, 0.7773437500000000000, 0.7792968750000000000, 0.7812500000000000000, 0.7832031250000000000, 0.7851562500000000000, 0.7871093750000000000, 0.7890625000000000000, 0.7910156250000000000, 0.7929687500000000000, 0.7949218750000000000, 0.7968750000000000000, 0.7988281250000000000, 0.8007812500000000000, 0.8027343750000000000, 0.8046875000000000000, 0.8066406250000000000, 0.8085937500000000000, 0.8105468750000000000, 0.8125000000000000000, 0.8144531250000000000, 0.8164062500000000000, 0.8183593750000000000, 0.8203125000000000000, 0.8222656250000000000, 0.8242187500000000000, 0.8261718750000000000, 0.8281250000000000000, 0.8300781250000000000, 0.8320312500000000000, 0.8339843750000000000, 0.8359375000000000000, 0.8378906250000000000, 0.8398437500000000000, 0.8417968750000000000, 0.8437500000000000000, 0.8457031250000000000, 0.8476562500000000000, 0.8496093750000000000, 0.8515625000000000000, 0.8535156250000000000, 0.8554687500000000000, 0.8574218750000000000, 0.8593750000000000000, 0.8613281250000000000, 0.8632812500000000000, 0.8652343750000000000, 0.8671875000000000000, 0.8691406250000000000, 0.8710937500000000000, 0.8730468750000000000, 0.8750000000000000000, 0.8769531250000000000, 0.8789062500000000000, 0.8808593750000000000, 0.8828125000000000000, 0.8847656250000000000, 0.8867187500000000000, 0.8886718750000000000, 0.8906250000000000000, 0.8925781250000000000, 0.8945312500000000000, 0.8964843750000000000, 0.8984375000000000000, 0.9003906250000000000, 0.9023437500000000000, 0.9042968750000000000, 0.9062500000000000000, 0.9082031250000000000, 0.9101562500000000000, 0.9121093750000000000, 0.9140625000000000000, 0.9160156250000000000, 0.9179687500000000000, 0.9199218750000000000, 0.9218750000000000000, 0.9238281250000000000, 0.9257812500000000000, 0.9277343750000000000, 0.9296875000000000000, 0.9316406250000000000, 0.9335937500000000000, 0.9355468750000000000, 0.9375000000000000000, 0.9394531250000000000, 0.9414062500000000000, 0.9433593750000000000, 0.9453125000000000000, 0.9472656250000000000, 0.9492187500000000000, 0.9511718750000000000, 0.9531250000000000000, 0.9550781250000000000, 0.9570312500000000000, 0.9589843750000000000, 0.9609375000000000000, 0.9628906250000000000, 0.9648437500000000000, 0.9667968750000000000, 0.9687500000000000000, 0.9707031250000000000, 0.9726562500000000000, 0.9746093750000000000, 0.9765625000000000000, 0.9785156250000000000, 0.9791718336226511443 ),
 .UNSPECIFIED. ) 
 GEOMETRIC_REPRESENTATION_ITEM ( )  RATIONAL_B_SPLINE_SURFACE ( (
 ( 1.000000000000000000, 0.9807852804032304306, 1.000000000000000000, 0.9807852804032304306, 1.000000000000000000, 0.9807852804032304306, 1.000000000000000000, 0.9807852804032304306, 1.000000000000000000, 0.9807852804032304306, 1.000000000000000000, 0.9807852804032304306, 1.000000000000000000, 0.9807852804032304306, 1.000000000000000000, 0.9807852804032304306, 1.000000000000000000, 0.9807852804032304306, 1.000000000000000000, 0.9807852804032304306, 1.000000000000000000, 0.9807852804032304306, 1.000000000000000000, 0.9807852804032304306, 1.000000000000000000, 0.9807852804032304306, 1.000000000000000000, 0.9807852804032304306, 1.000000000000000000, 0.9807852804032304306, 1.000000000000000000, 0.9807852804032304306, 1.000000000000000000, 0.9807852804032304306, 1.000000000000000000, 0.9807852804032304306, 1.000000000000000000, 0.9807852804032304306, 1.000000000000000000, 0.9807852804032304306, 1.000000000000000000, 0.9807852804032304306, 1.000000000000000000, 0.9807852804032304306, 1.000000000000000000, 0.9807852804032304306, 1.000000000000000000, 0.9807852804032304306, 1.000000000000000000, 0.9807852804032304306, 1.000000000000000000, 0.9807852804032304306, 1.000000000000000000, 0.9807852804032304306, 1.000000000000000000, 0.9807852804032304306, 1.000000000000000000, 0.9807852804032304306, 1.000000000000000000, 0.9807852804032304306, 1.000000000000000000, 0.9807852804032304306, 1.000000000000000000, 0.9807852804032304306, 1.000000000000000000, 0.9807852804032304306, 1.000000000000000000, 0.9807852804032304306, 1.000000000000000000, 0.9807852804032304306, 1.000000000000000000, 0.9807852804032304306, 1.000000000000000000, 0.9807852804032304306, 1.000000000000000000, 0.9807852804032304306, 1.000000000000000000, 0.9807852804032304306, 1.000000000000000000, 0.9807852804032304306, 1.000000000000000000, 0.9807852804032304306, 1.000000000000000000, 0.9807852804032304306, 1.000000000000000000, 0.9807852804032304306, 1.000000000000000000, 0.9807852804032304306, 1.000000000000000000, 0.9807852804032304306, 1.000000000000000000, 0.9807852804032304306, 1.000000000000000000, 0.9807852804032304306, 1.000000000000000000, 0.9807852804032304306, 1.000000000000000000, 0.9807852804032304306, 1.000000000000000000, 0.9807852804032304306, 1.000000000000000000, 0.9807852804032304306, 1.000000000000000000, 0.9807852804032304306, 1.000000000000000000, 0.9807852804032304306, 1.000000000000000000, 0.9807852804032304306, 1.000000000000000000, 0.9807852804032304306, 1.000000000000000000, 0.9807852804032304306, 1.000000000000000000, 0.9807852804032304306, 1.000000000000000000, 0.9807852804032304306, 1.000000000000000000, 0.9807852804032304306, 1.000000000000000000, 0.9807852804032304306, 1.000000000000000000, 0.9807852804032304306, 1.000000000000000000, 0.9807852804032304306, 1.000000000000000000, 0.9807852804032304306, 1.000000000000000000, 0.9807852804032304306, 1.000000000000000000, 0.9807852804032304306, 1.000000000000000000, 0.9807852804032304306, 1.000000000000000000, 0.9807852804032304306, 1.000000000000000000, 0.9807852804032304306, 1.000000000000000000, 0.9807852804032304306, 1.000000000000000000, 0.9807852804032304306, 1.000000000000000000, 0.9807852804032304306, 1.000000000000000000, 0.9807852804032304306, 1.000000000000000000, 0.9807852804032304306, 1.000000000000000000, 0.9807852804032304306, 1.000000000000000000, 0.9807852804032304306, 1.000000000000000000, 0.9807852804032304306, 1.000000000000000000, 0.9807852804032304306, 1.000000000000000000, 0.9807852804032304306, 1.000000000000000000, 0.9807852804032304306, 1.000000000000000000, 0.9807852804032304306, 1.000000000000000000, 0.9807852804032304306, 1.000000000000000000, 0.9807852804032304306, 1.000000000000000000, 0.9807852804032304306, 1.000000000000000000, 0.9807852804032304306, 1.000000000000000000, 0.9807852804032304306, 1.000000000000000000, 0.9807852804032304306, 1.000000000000000000, 0.9807852804032304306, 1.000000000000000000, 0.9807852804032304306, 1.000000000000000000, 0.9807852804032304306, 1.000000000000000000, 0.9807852804032304306, 1.000000000000000000, 0.9807852804032304306, 1.000000000000000000, 0.9807852804032304306, 1.000000000000000000, 0.9807852804032304306, 1.000000000000000000, 0.9807852804032304306, 1.000000000000000000, 0.9807852804032304306, 1.000000000000000000, 0.9807852804032304306, 1.000000000000000000, 0.9807852804032304306, 1.000000000000000000, 0.9807852804032304306, 1.000000000000000000, 0.9807852804032304306, 1.000000000000000000, 0.9807852804032304306, 1.000000000000000000, 0.9807852804032304306, 1.000000000000000000, 0.9807852804032304306, 1.000000000000000000, 0.9807852804032304306, 1.000000000000000000, 0.9807852804032304306, 1.000000000000000000, 0.9807852804032304306, 1.000000000000000000, 0.9807852804032304306, 1.000000000000000000, 0.9807852804032304306, 1.000000000000000000, 0.9807852804032304306, 1.000000000000000000, 0.9807852804032304306, 1.000000000000000000, 0.9807852804032304306, 1.000000000000000000, 0.9807852804032304306, 1.000000000000000000, 0.9807852804032304306, 1.000000000000000000, 0.9807852804032304306, 1.000000000000000000, 0.9807852804032304306, 1.000000000000000000, 0.9807852804032304306, 1.000000000000000000, 0.9807852804032304306, 1.000000000000000000, 0.9807852804032304306, 1.000000000000000000, 0.9807852804032304306, 1.000000000000000000, 0.9807852804032304306, 1.000000000000000000, 0.9807852804032304306, 1.000000000000000000, 0.9807852804032304306, 1.000000000000000000, 0.9807852804032304306, 1.000000000000000000, 0.9807852804032304306, 1.000000000000000000, 0.9807852804032304306, 1.000000000000000000, 0.9807852804032304306, 1.000000000000000000, 0.9807852804032304306, 1.000000000000000000, 0.9807852804032304306, 1.000000000000000000, 0.9807852804032304306, 1.000000000000000000, 0.9807852804032304306, 1.000000000000000000, 0.9807852804032304306, 1.000000000000000000, 0.9807852804032304306, 1.000000000000000000, 0.9807852804032304306, 1.000000000000000000, 0.9807852804032304306, 1.000000000000000000, 0.9807852804032304306, 1.000000000000000000, 0.9807852804032304306, 1.000000000000000000, 0.9807852804032304306, 1.000000000000000000, 0.9807852804032304306, 1.000000000000000000, 0.9807852804032304306, 1.000000000000000000, 0.9807852804032304306, 1.000000000000000000, 0.9807852804032304306, 1.000000000000000000, 0.9807852804032304306, 1.000000000000000000, 0.9807852804032304306, 1.000000000000000000, 0.9807852804032304306, 1.000000000000000000, 0.9807852804032304306, 1.000000000000000000, 0.9807852804032304306, 1.000000000000000000, 0.9807852804032304306, 1.000000000000000000, 0.9807852804032304306, 1.000000000000000000, 0.9807852804032304306, 1.000000000000000000, 0.9807852804032304306, 1.000000000000000000, 0.9807852804032304306, 1.000000000000000000, 0.9807852804032304306, 1.000000000000000000, 0.9807852804032304306, 1.000000000000000000, 0.9807852804032304306, 1.000000000000000000, 0.9807852804032304306, 1.000000000000000000, 0.9807852804032304306, 1.000000000000000000, 0.9807852804032304306, 1.000000000000000000, 0.9807852804032304306, 1.000000000000000000, 0.9807852804032304306, 1.000000000000000000, 0.9807852804032304306, 1.000000000000000000, 0.9807852804032304306, 1.000000000000000000, 0.9807852804032304306, 1.000000000000000000, 0.9807852804032304306, 1.000000000000000000, 0.9807852804032304306, 1.000000000000000000, 0.9807852804032304306, 1.000000000000000000, 0.9807852804032304306, 1.000000000000000000, 0.9807852804032304306, 1.000000000000000000, 0.9807852804032304306, 1.000000000000000000, 0.9807852804032304306, 1.000000000000000000, 0.9807852804032304306, 1.000000000000000000, 0.9807852804032304306, 1.000000000000000000, 0.9807852804032304306, 1.000000000000000000, 0.9807852804032304306, 1.000000000000000000, 0.9807852804032304306, 1.000000000000000000, 0.9807852804032304306, 1.000000000000000000, 0.9807852804032304306, 1.000000000000000000, 0.9807852804032304306, 1.000000000000000000, 0.9807852804032304306, 1.000000000000000000, 0.9807852804032304306, 1.000000000000000000, 0.9807852804032304306, 1.000000000000000000, 0.9807852804032304306, 1.000000000000000000, 0.9807852804032304306, 1.000000000000000000, 0.9807852804032304306, 1.000000000000000000, 0.9807852804032304306, 1.000000000000000000, 0.9807852804032304306, 1.000000000000000000, 0.9807852804032304306, 1.000000000000000000, 0.9807852804032304306, 1.000000000000000000, 0.9807852804032304306, 1.000000000000000000, 0.9807852804032304306, 1.000000000000000000, 0.9807852804032304306, 1.000000000000000000, 0.9807852804032304306, 1.000000000000000000, 0.9807852804032304306, 1.000000000000000000, 0.9807852804032304306, 1.000000000000000000, 0.9807852804032304306, 1.000000000000000000, 0.9807852804032304306, 1.000000000000000000, 0.9807852804032304306, 1.000000000000000000, 0.9807852804032304306, 1.000000000000000000, 0.9807852804032304306, 1.000000000000000000, 0.9807852804032304306, 1.000000000000000000, 0.9807852804032304306, 1.000000000000000000, 0.9807852804032304306, 1.000000000000000000, 0.9807852804032304306, 1.000000000000000000, 0.9807852804032304306, 1.000000000000000000, 0.9807852804032304306, 1.000000000000000000, 0.9807852804032304306, 1.000000000000000000, 0.9807852804032304306, 1.000000000000000000, 0.9807852804032304306, 1.000000000000000000, 0.9807852804032304306, 1.000000000000000000, 0.9807852804032304306, 1.000000000000000000, 0.9807852804032304306, 1.000000000000000000, 0.9807852804032304306, 1.000000000000000000, 0.9807852804032304306, 1.000000000000000000, 0.9807852804032304306, 1.000000000000000000, 0.9807852804032304306, 1.000000000000000000, 0.9807852804032304306, 1.000000000000000000, 0.9807852804032304306, 1.000000000000000000, 0.9807852804032304306, 1.000000000000000000, 0.9807852804032304306, 1.000000000000000000, 0.9807852804032304306, 1.000000000000000000, 0.9807852804032304306, 1.000000000000000000, 0.9807852804032304306, 1.000000000000000000, 0.9807852804032304306, 1.000000000000000000, 0.9807852804032304306, 1.000000000000000000, 0.9807852804032304306, 1.000000000000000000, 0.9807852804032304306, 1.000000000000000000, 0.9807852804032304306, 1.000000000000000000, 0.9807852804032304306, 1.000000000000000000, 0.9807852804032304306, 1.000000000000000000, 0.9807852804032304306, 1.000000000000000000, 0.9807852804032304306, 1.000000000000000000, 0.9807852804032304306, 1.000000000000000000, 0.9807852804032304306, 1.000000000000000000, 0.9807852804032304306, 1.000000000000000000, 0.9807852804032304306, 1.000000000000000000, 0.9807852804032304306, 1.000000000000000000, 0.9807852804032304306, 1.000000000000000000, 0.9807852804032304306, 1.000000000000000000, 0.9807852804032304306, 1.000000000000000000, 0.9807852804032304306, 1.000000000000000000, 0.9807852804032304306, 1.000000000000000000, 0.9807852804032304306, 1.000000000000000000, 0.9807852804032304306, 1.000000000000000000, 0.9807852804032304306, 1.000000000000000000, 0.9807852804032304306, 1.000000000000000000, 0.9807852804032304306, 1.000000000000000000, 0.9807852804032304306, 1.000000000000000000, 0.9807852804032304306, 1.000000000000000000, 0.9807852804032304306, 1.000000000000000000, 0.9807852804032304306, 1.000000000000000000, 0.9807852804032304306, 1.000000000000000000, 0.9807852804032304306, 1.000000000000000000, 0.9807852804032304306, 1.000000000000000000, 0.9807852804032304306, 1.000000000000000000, 0.9807852804032304306, 1.000000000000000000, 0.9807852804032304306, 1.000000000000000000, 0.9807852804032304306, 1.000000000000000000, 0.9807852804032304306, 1.000000000000000000, 0.9807852804032304306, 1.000000000000000000, 0.9807852804032304306, 1.000000000000000000, 0.9807852804032304306, 1.000000000000000000, 0.9807852804032304306, 1.000000000000000000, 0.9807852804032304306, 1.000000000000000000, 0.9807852804032304306, 1.000000000000000000, 0.9807852804032304306, 1.000000000000000000, 0.9807852804032304306, 1.000000000000000000, 0.9807852804032304306, 1.000000000000000000, 0.9807852804032304306, 1.000000000000000000, 0.9807852804032304306, 1.000000000000000000, 0.9807852804032304306, 1.000000000000000000, 0.9807852804032304306, 1.000000000000000000, 0.9807852804032304306, 1.000000000000000000, 0.9807852804032304306, 1.000000000000000000, 0.9807852804032304306, 1.000000000000000000, 0.9807852804032304306, 1.000000000000000000, 0.9807852804032304306, 1.000000000000000000, 0.9807852804032304306, 1.000000000000000000, 0.9807852804032304306, 1.000000000000000000, 0.9807852804032304306, 1.000000000000000000, 0.9807852804032304306, 1.000000000000000000, 0.9807852804032304306, 1.000000000000000000, 0.9807852804032304306, 1.000000000000000000, 0.9807852804032304306, 1.000000000000000000, 0.9807852804032304306, 1.000000000000000000, 0.9807852804032304306, 1.000000000000000000, 0.9807852804032304306, 1.000000000000000000, 0.9807852804032304306, 1.000000000000000000, 0.9807852804032304306, 1.000000000000000000, 0.9807852804032304306, 1.000000000000000000, 0.9807852804032304306, 1.000000000000000000, 0.9807852804032304306, 1.000000000000000000, 0.9807852804032304306, 1.000000000000000000, 0.9807852804032304306, 1.000000000000000000, 0.9807852804032304306, 1.000000000000000000, 0.9807852804032304306, 1.000000000000000000, 0.9807852804032304306, 1.000000000000000000, 0.9807852804032304306, 1.000000000000000000, 0.9807852804032304306, 1.000000000000000000, 0.9807852804032304306, 1.000000000000000000, 0.9807852804032304306, 1.000000000000000000, 0.9807852804032304306, 1.000000000000000000, 0.9807852804032304306, 1.000000000000000000, 0.9807852804032304306, 1.000000000000000000, 0.9807852804032304306, 1.000000000000000000, 0.9807852804032304306, 1.000000000000000000, 0.9807852804032304306, 1.000000000000000000, 0.9807852804032304306, 1.000000000000000000, 0.9807852804032304306, 1.000000000000000000, 0.9807852804032304306, 1.000000000000000000, 0.9807852804032304306, 1.000000000000000000, 0.9807852804032304306, 1.000000000000000000, 0.9807852804032304306, 1.000000000000000000, 0.9807852804032304306, 1.000000000000000000, 0.9807852804032304306, 1.000000000000000000, 0.9807852804032304306, 1.000000000000000000, 0.9807852804032304306, 1.000000000000000000, 0.9807852804032304306, 1.000000000000000000, 0.9807852804032304306, 1.000000000000000000, 0.9807852804032304306, 1.000000000000000000, 0.9807852804032304306, 1.000000000000000000, 0.9807852804032304306, 1.000000000000000000, 0.9807852804032304306, 1.000000000000000000, 0.9807852804032304306, 1.000000000000000000, 0.9807852804032304306, 1.000000000000000000, 0.9807852804032304306, 1.000000000000000000, 0.9807852804032304306, 1.000000000000000000, 0.9807852804032304306, 1.000000000000000000, 0.9807852804032304306, 1.000000000000000000, 0.9807852804032304306, 1.000000000000000000, 0.9807852804032304306, 1.000000000000000000, 0.9807852804032304306, 1.000000000000000000, 0.9807852804032304306, 1.000000000000000000, 0.9807852804032304306, 1.000000000000000000, 0.9807852804032304306, 1.000000000000000000, 0.9807852804032304306, 1.000000000000000000, 0.9807852804032304306, 1.000000000000000000, 0.9807852804032304306, 1.000000000000000000, 0.9807852804032304306, 1.000000000000000000, 0.9807852804032304306, 1.000000000000000000, 0.9807852804032304306, 1.000000000000000000, 0.9807852804032304306, 1.000000000000000000, 0.9807852804032304306, 1.000000000000000000, 0.9807852804032304306, 1.000000000000000000, 0.9807852804032304306, 1.000000000000000000, 0.9807852804032304306, 1.000000000000000000, 0.9807852804032304306, 1.000000000000000000, 0.9807852804032304306, 1.000000000000000000, 0.9807852804032304306, 1.000000000000000000, 0.9807852804032304306, 1.000000000000000000, 0.9807852804032304306, 1.000000000000000000, 0.9807852804032304306, 1.000000000000000000, 0.9807852804032304306, 1.000000000000000000, 0.9807852804032304306, 1.000000000000000000, 0.9807852804032304306, 1.000000000000000000, 0.9807852804032304306, 1.000000000000000000, 0.9807852804032304306, 1.000000000000000000, 0.9807852804032304306, 1.000000000000000000, 0.9807852804032304306, 1.000000000000000000, 0.9807852804032304306, 1.000000000000000000, 0.9807852804032304306, 1.000000000000000000, 0.9807852804032304306, 1.000000000000000000, 0.9807852804032304306, 1.000000000000000000, 0.9807852804032304306, 1.000000000000000000, 0.9807852804032304306, 1.000000000000000000, 0.9807852804032304306, 1.000000000000000000, 0.9807852804032304306, 1.000000000000000000, 0.9807852804032304306, 1.000000000000000000, 0.9807852804032304306, 1.000000000000000000, 0.9807852804032304306, 1.000000000000000000, 0.9807852804032304306, 1.000000000000000000, 0.9807852804032304306, 1.000000000000000000, 0.9807852804032304306, 1.000000000000000000, 0.9807852804032304306, 1.000000000000000000, 0.9807852804032304306, 1.000000000000000000, 0.9807852804032304306, 1.000000000000000000, 0.9807852804032304306, 1.000000000000000000, 0.9807852804032304306, 1.000000000000000000, 0.9807852804032304306, 1.000000000000000000, 0.9807852804032304306, 1.000000000000000000, 0.9807852804032304306, 1.000000000000000000, 0.9807852804032304306, 1.000000000000000000, 0.9807852804032304306, 1.000000000000000000, 0.9807852804032304306, 1.000000000000000000, 0.9807852804032304306, 1.000000000000000000, 0.9807852804032304306, 1.000000000000000000, 0.9807852804032304306, 1.000000000000000000, 0.9807852804032304306, 1.000000000000000000, 0.9807852804032304306, 1.000000000000000000, 0.9807852804032304306, 1.000000000000000000, 0.9807852804032304306, 1.000000000000000000, 0.9807852804032304306, 1.000000000000000000, 0.9807852804032304306, 1.000000000000000000, 0.9807852804032304306, 1.000000000000000000, 0.9807852804032304306, 1.000000000000000000, 0.9807852804032304306, 1.000000000000000000, 0.9807852804032304306, 1.000000000000000000, 0.9807852804032304306, 1.000000000000000000, 0.9807852804032304306, 1.000000000000000000, 0.9807852804032304306, 1.000000000000000000, 0.9807852804032304306, 1.000000000000000000, 0.9807852804032304306, 1.000000000000000000, 0.9807852804032304306, 1.000000000000000000, 0.9807852804032304306, 1.000000000000000000, 0.9807852804032304306, 1.000000000000000000, 0.9807852804032304306, 1.000000000000000000, 0.9807852804032304306, 1.000000000000000000, 0.9807852804032304306, 1.000000000000000000, 0.9807852804032304306, 1.000000000000000000, 0.9807852804032304306, 1.000000000000000000, 0.9807852804032304306, 1.000000000000000000, 0.9807852804032304306, 1.000000000000000000, 0.9807852804032304306, 1.000000000000000000, 0.9807852804032304306, 1.000000000000000000, 0.9807852804032304306, 1.000000000000000000, 0.9807852804032304306, 1.000000000000000000, 0.9807852804032304306, 1.000000000000000000, 0.9807852804032304306, 1.000000000000000000, 0.9807852804032304306, 1.000000000000000000, 0.9807852804032304306, 1.000000000000000000, 0.9807852804032304306, 1.000000000000000000, 0.9807852804032304306, 1.000000000000000000, 0.9807852804032304306, 1.000000000000000000, 0.9807852804032304306, 1.000000000000000000, 0.9807852804032304306, 1.000000000000000000, 0.9807852804032304306, 1.000000000000000000, 0.9807852804032304306, 1.000000000000000000, 0.9807852804032304306, 1.000000000000000000, 0.9807852804032304306, 1.000000000000000000, 0.9807852804032304306, 1.000000000000000000, 0.9807852804032304306, 1.000000000000000000, 0.9807852804032304306, 1.000000000000000000, 0.9807852804032304306, 1.000000000000000000, 0.9807852804032304306, 1.000000000000000000, 0.9807852804032304306, 1.000000000000000000, 0.9807852804032304306, 1.000000000000000000, 0.9807852804032304306, 1.000000000000000000, 0.9807852804032304306, 1.000000000000000000, 0.9807852804032304306, 1.000000000000000000, 0.9807852804032304306, 1.000000000000000000, 0.9807852804032304306, 1.000000000000000000, 0.9807852804032304306, 1.000000000000000000, 0.9807852804032304306, 1.000000000000000000, 0.9807852804032304306, 1.000000000000000000, 0.9807852804032304306, 1.000000000000000000, 0.9807852804032304306, 1.000000000000000000, 0.9807852804032304306, 1.000000000000000000, 0.9807852804032304306, 1.000000000000000000, 0.9807852804032304306, 1.000000000000000000, 0.9807852804032304306, 1.000000000000000000, 0.9807852804032304306, 1.000000000000000000, 0.9807852804032304306, 1.000000000000000000, 0.9807852804032304306, 1.000000000000000000, 0.9807852804032304306, 1.000000000000000000, 0.9807852804032304306, 1.000000000000000000, 0.9807852804032304306, 1.000000000000000000, 0.9807852804032304306, 1.000000000000000000, 0.9807852804032304306, 1.000000000000000000, 0.9807852804032304306, 1.000000000000000000, 0.9807852804032304306, 1.000000000000000000, 0.9807852804032304306, 1.000000000000000000, 0.9807852804032304306, 1.000000000000000000, 0.9807852804032304306, 1.000000000000000000, 0.9807852804032304306, 1.000000000000000000, 0.9807852804032304306, 1.000000000000000000, 0.9807852804032304306, 1.000000000000000000, 0.9807852804032304306, 1.000000000000000000, 0.9807852804032304306, 1.000000000000000000, 0.9807852804032304306, 1.000000000000000000, 0.9807852804032304306, 1.000000000000000000, 0.9807852804032304306, 1.000000000000000000, 0.9807852804032304306, 1.000000000000000000, 0.9807852804032304306, 1.000000000000000000, 0.9807852804032304306, 1.000000000000000000, 0.9807852804032304306, 1.000000000000000000, 0.9807852804032304306, 1.000000000000000000, 0.9807852804032304306, 1.000000000000000000, 0.9807852804032304306, 1.000000000000000000, 0.9807852804032304306, 1.000000000000000000, 0.9807852804032304306, 1.000000000000000000, 0.9807852804032304306, 1.000000000000000000, 0.9807852804032304306, 1.000000000000000000, 0.9807852804032304306, 1.000000000000000000, 0.9807852804032304306, 1.000000000000000000, 0.9807852804032304306, 1.000000000000000000, 0.9807852804032304306, 1.000000000000000000, 0.9807852804032304306, 1.000000000000000000, 0.9807852804032304306, 1.000000000000000000, 0.9807852804032304306, 1.000000000000000000, 0.9807852804032304306, 1.000000000000000000, 0.9807852804032304306, 1.000000000000000000, 0.9807852804032304306, 1.000000000000000000, 0.9807852804032304306, 1.000000000000000000, 0.9807852804032304306, 1.000000000000000000, 0.9807852804032304306, 1.000000000000000000, 0.9807852804032304306, 1.000000000000000000, 0.9807852804032304306, 1.000000000000000000, 0.9807852804032304306, 1.000000000000000000, 0.9807852804032304306, 1.000000000000000000, 0.9807852804032304306, 1.000000000000000000, 0.9807852804032304306, 1.000000000000000000, 0.9807852804032304306, 1.000000000000000000, 0.9807852804032304306, 1.000000000000000000, 0.9807852804032304306, 1.000000000000000000, 0.9935442612832132703, 0.9914265054518418552),
 ( 1.000000000000000000, 0.9807852804032304306, 1.000000000000000000, 0.9807852804032304306, 1.000000000000000000, 0.9807852804032304306, 1.000000000000000000, 0.9807852804032304306, 1.000000000000000000, 0.9807852804032304306, 1.000000000000000000, 0.9807852804032304306, 1.000000000000000000, 0.9807852804032304306, 1.000000000000000000, 0.9807852804032304306, 1.000000000000000000, 0.9807852804032304306, 1.000000000000000000, 0.9807852804032304306, 1.000000000000000000, 0.9807852804032304306, 1.000000000000000000, 0.9807852804032304306, 1.000000000000000000, 0.9807852804032304306, 1.000000000000000000, 0.9807852804032304306, 1.000000000000000000, 0.9807852804032304306, 1.000000000000000000, 0.9807852804032304306, 1.000000000000000000, 0.9807852804032304306, 1.000000000000000000, 0.9807852804032304306, 1.000000000000000000, 0.9807852804032304306, 1.000000000000000000, 0.9807852804032304306, 1.000000000000000000, 0.9807852804032304306, 1.000000000000000000, 0.9807852804032304306, 1.000000000000000000, 0.9807852804032304306, 1.000000000000000000, 0.9807852804032304306, 1.000000000000000000, 0.9807852804032304306, 1.000000000000000000, 0.9807852804032304306, 1.000000000000000000, 0.9807852804032304306, 1.000000000000000000, 0.9807852804032304306, 1.000000000000000000, 0.9807852804032304306, 1.000000000000000000, 0.9807852804032304306, 1.000000000000000000, 0.9807852804032304306, 1.000000000000000000, 0.9807852804032304306, 1.000000000000000000, 0.9807852804032304306, 1.000000000000000000, 0.9807852804032304306, 1.000000000000000000, 0.9807852804032304306, 1.000000000000000000, 0.9807852804032304306, 1.000000000000000000, 0.9807852804032304306, 1.000000000000000000, 0.9807852804032304306, 1.000000000000000000, 0.9807852804032304306, 1.000000000000000000, 0.9807852804032304306, 1.000000000000000000, 0.9807852804032304306, 1.000000000000000000, 0.9807852804032304306, 1.000000000000000000, 0.9807852804032304306, 1.000000000000000000, 0.9807852804032304306, 1.000000000000000000, 0.9807852804032304306, 1.000000000000000000, 0.9807852804032304306, 1.000000000000000000, 0.9807852804032304306, 1.000000000000000000, 0.9807852804032304306, 1.000000000000000000, 0.9807852804032304306, 1.000000000000000000, 0.9807852804032304306, 1.000000000000000000, 0.9807852804032304306, 1.000000000000000000, 0.9807852804032304306, 1.000000000000000000, 0.9807852804032304306, 1.000000000000000000, 0.9807852804032304306, 1.000000000000000000, 0.9807852804032304306, 1.000000000000000000, 0.9807852804032304306, 1.000000000000000000, 0.9807852804032304306, 1.000000000000000000, 0.9807852804032304306, 1.000000000000000000, 0.9807852804032304306, 1.000000000000000000, 0.9807852804032304306, 1.000000000000000000, 0.9807852804032304306, 1.000000000000000000, 0.9807852804032304306, 1.000000000000000000, 0.9807852804032304306, 1.000000000000000000, 0.9807852804032304306, 1.000000000000000000, 0.9807852804032304306, 1.000000000000000000, 0.9807852804032304306, 1.000000000000000000, 0.9807852804032304306, 1.000000000000000000, 0.9807852804032304306, 1.000000000000000000, 0.9807852804032304306, 1.000000000000000000, 0.9807852804032304306, 1.000000000000000000, 0.9807852804032304306, 1.000000000000000000, 0.9807852804032304306, 1.000000000000000000, 0.9807852804032304306, 1.000000000000000000, 0.9807852804032304306, 1.000000000000000000, 0.9807852804032304306, 1.000000000000000000, 0.9807852804032304306, 1.000000000000000000, 0.9807852804032304306, 1.000000000000000000, 0.9807852804032304306, 1.000000000000000000, 0.9807852804032304306, 1.000000000000000000, 0.9807852804032304306, 1.000000000000000000, 0.9807852804032304306, 1.000000000000000000, 0.9807852804032304306, 1.000000000000000000, 0.9807852804032304306, 1.000000000000000000, 0.9807852804032304306, 1.000000000000000000, 0.9807852804032304306, 1.000000000000000000, 0.9807852804032304306, 1.000000000000000000, 0.9807852804032304306, 1.000000000000000000, 0.9807852804032304306, 1.000000000000000000, 0.9807852804032304306, 1.000000000000000000, 0.9807852804032304306, 1.000000000000000000, 0.9807852804032304306, 1.000000000000000000, 0.9807852804032304306, 1.000000000000000000, 0.9807852804032304306, 1.000000000000000000, 0.9807852804032304306, 1.000000000000000000, 0.9807852804032304306, 1.000000000000000000, 0.9807852804032304306, 1.000000000000000000, 0.9807852804032304306, 1.000000000000000000, 0.9807852804032304306, 1.000000000000000000, 0.9807852804032304306, 1.000000000000000000, 0.9807852804032304306, 1.000000000000000000, 0.9807852804032304306, 1.000000000000000000, 0.9807852804032304306, 1.000000000000000000, 0.9807852804032304306, 1.000000000000000000, 0.9807852804032304306, 1.000000000000000000, 0.9807852804032304306, 1.000000000000000000, 0.9807852804032304306, 1.000000000000000000, 0.9807852804032304306, 1.000000000000000000, 0.9807852804032304306, 1.000000000000000000, 0.9807852804032304306, 1.000000000000000000, 0.9807852804032304306, 1.000000000000000000, 0.9807852804032304306, 1.000000000000000000, 0.9807852804032304306, 1.000000000000000000, 0.9807852804032304306, 1.000000000000000000, 0.9807852804032304306, 1.000000000000000000, 0.9807852804032304306, 1.000000000000000000, 0.9807852804032304306, 1.000000000000000000, 0.9807852804032304306, 1.000000000000000000, 0.9807852804032304306, 1.000000000000000000, 0.9807852804032304306, 1.000000000000000000, 0.9807852804032304306, 1.000000000000000000, 0.9807852804032304306, 1.000000000000000000, 0.9807852804032304306, 1.000000000000000000, 0.9807852804032304306, 1.000000000000000000, 0.9807852804032304306, 1.000000000000000000, 0.9807852804032304306, 1.000000000000000000, 0.9807852804032304306, 1.000000000000000000, 0.9807852804032304306, 1.000000000000000000, 0.9807852804032304306, 1.000000000000000000, 0.9807852804032304306, 1.000000000000000000, 0.9807852804032304306, 1.000000000000000000, 0.9807852804032304306, 1.000000000000000000, 0.9807852804032304306, 1.000000000000000000, 0.9807852804032304306, 1.000000000000000000, 0.9807852804032304306, 1.000000000000000000, 0.9807852804032304306, 1.000000000000000000, 0.9807852804032304306, 1.000000000000000000, 0.9807852804032304306, 1.000000000000000000, 0.9807852804032304306, 1.000000000000000000, 0.9807852804032304306, 1.000000000000000000, 0.9807852804032304306, 1.000000000000000000, 0.9807852804032304306, 1.000000000000000000, 0.9807852804032304306, 1.000000000000000000, 0.9807852804032304306, 1.000000000000000000, 0.9807852804032304306, 1.000000000000000000, 0.9807852804032304306, 1.000000000000000000, 0.9807852804032304306, 1.000000000000000000, 0.9807852804032304306, 1.000000000000000000, 0.9807852804032304306, 1.000000000000000000, 0.9807852804032304306, 1.000000000000000000, 0.9807852804032304306, 1.000000000000000000, 0.9807852804032304306, 1.000000000000000000, 0.9807852804032304306, 1.000000000000000000, 0.9807852804032304306, 1.000000000000000000, 0.9807852804032304306, 1.000000000000000000, 0.9807852804032304306, 1.000000000000000000, 0.9807852804032304306, 1.000000000000000000, 0.9807852804032304306, 1.000000000000000000, 0.9807852804032304306, 1.000000000000000000, 0.9807852804032304306, 1.000000000000000000, 0.9807852804032304306, 1.000000000000000000, 0.9807852804032304306, 1.000000000000000000, 0.9807852804032304306, 1.000000000000000000, 0.9807852804032304306, 1.000000000000000000, 0.9807852804032304306, 1.000000000000000000, 0.9807852804032304306, 1.000000000000000000, 0.9807852804032304306, 1.000000000000000000, 0.9807852804032304306, 1.000000000000000000, 0.9807852804032304306, 1.000000000000000000, 0.9807852804032304306, 1.000000000000000000, 0.9807852804032304306, 1.000000000000000000, 0.9807852804032304306, 1.000000000000000000, 0.9807852804032304306, 1.000000000000000000, 0.9807852804032304306, 1.000000000000000000, 0.9807852804032304306, 1.000000000000000000, 0.9807852804032304306, 1.000000000000000000, 0.9807852804032304306, 1.000000000000000000, 0.9807852804032304306, 1.000000000000000000, 0.9807852804032304306, 1.000000000000000000, 0.9807852804032304306, 1.000000000000000000, 0.9807852804032304306, 1.000000000000000000, 0.9807852804032304306, 1.000000000000000000, 0.9807852804032304306, 1.000000000000000000, 0.9807852804032304306, 1.000000000000000000, 0.9807852804032304306, 1.000000000000000000, 0.9807852804032304306, 1.000000000000000000, 0.9807852804032304306, 1.000000000000000000, 0.9807852804032304306, 1.000000000000000000, 0.9807852804032304306, 1.000000000000000000, 0.9807852804032304306, 1.000000000000000000, 0.9807852804032304306, 1.000000000000000000, 0.9807852804032304306, 1.000000000000000000, 0.9807852804032304306, 1.000000000000000000, 0.9807852804032304306, 1.000000000000000000, 0.9807852804032304306, 1.000000000000000000, 0.9807852804032304306, 1.000000000000000000, 0.9807852804032304306, 1.000000000000000000, 0.9807852804032304306, 1.000000000000000000, 0.9807852804032304306, 1.000000000000000000, 0.9807852804032304306, 1.000000000000000000, 0.9807852804032304306, 1.000000000000000000, 0.9807852804032304306, 1.000000000000000000, 0.9807852804032304306, 1.000000000000000000, 0.9807852804032304306, 1.000000000000000000, 0.9807852804032304306, 1.000000000000000000, 0.9807852804032304306, 1.000000000000000000, 0.9807852804032304306, 1.000000000000000000, 0.9807852804032304306, 1.000000000000000000, 0.9807852804032304306, 1.000000000000000000, 0.9807852804032304306, 1.000000000000000000, 0.9807852804032304306, 1.000000000000000000, 0.9807852804032304306, 1.000000000000000000, 0.9807852804032304306, 1.000000000000000000, 0.9807852804032304306, 1.000000000000000000, 0.9807852804032304306, 1.000000000000000000, 0.9807852804032304306, 1.000000000000000000, 0.9807852804032304306, 1.000000000000000000, 0.9807852804032304306, 1.000000000000000000, 0.9807852804032304306, 1.000000000000000000, 0.9807852804032304306, 1.000000000000000000, 0.9807852804032304306, 1.000000000000000000, 0.9807852804032304306, 1.000000000000000000, 0.9807852804032304306, 1.000000000000000000, 0.9807852804032304306, 1.000000000000000000, 0.9807852804032304306, 1.000000000000000000, 0.9807852804032304306, 1.000000000000000000, 0.9807852804032304306, 1.000000000000000000, 0.9807852804032304306, 1.000000000000000000, 0.9807852804032304306, 1.000000000000000000, 0.9807852804032304306, 1.000000000000000000, 0.9807852804032304306, 1.000000000000000000, 0.9807852804032304306, 1.000000000000000000, 0.9807852804032304306, 1.000000000000000000, 0.9807852804032304306, 1.000000000000000000, 0.9807852804032304306, 1.000000000000000000, 0.9807852804032304306, 1.000000000000000000, 0.9807852804032304306, 1.000000000000000000, 0.9807852804032304306, 1.000000000000000000, 0.9807852804032304306, 1.000000000000000000, 0.9807852804032304306, 1.000000000000000000, 0.9807852804032304306, 1.000000000000000000, 0.9807852804032304306, 1.000000000000000000, 0.9807852804032304306, 1.000000000000000000, 0.9807852804032304306, 1.000000000000000000, 0.9807852804032304306, 1.000000000000000000, 0.9807852804032304306, 1.000000000000000000, 0.9807852804032304306, 1.000000000000000000, 0.9807852804032304306, 1.000000000000000000, 0.9807852804032304306, 1.000000000000000000, 0.9807852804032304306, 1.000000000000000000, 0.9807852804032304306, 1.000000000000000000, 0.9807852804032304306, 1.000000000000000000, 0.9807852804032304306, 1.000000000000000000, 0.9807852804032304306, 1.000000000000000000, 0.9807852804032304306, 1.000000000000000000, 0.9807852804032304306, 1.000000000000000000, 0.9807852804032304306, 1.000000000000000000, 0.9807852804032304306, 1.000000000000000000, 0.9807852804032304306, 1.000000000000000000, 0.9807852804032304306, 1.000000000000000000, 0.9807852804032304306, 1.000000000000000000, 0.9807852804032304306, 1.000000000000000000, 0.9807852804032304306, 1.000000000000000000, 0.9807852804032304306, 1.000000000000000000, 0.9807852804032304306, 1.000000000000000000, 0.9807852804032304306, 1.000000000000000000, 0.9807852804032304306, 1.000000000000000000, 0.9807852804032304306, 1.000000000000000000, 0.9807852804032304306, 1.000000000000000000, 0.9807852804032304306, 1.000000000000000000, 0.9807852804032304306, 1.000000000000000000, 0.9807852804032304306, 1.000000000000000000, 0.9807852804032304306, 1.000000000000000000, 0.9807852804032304306, 1.000000000000000000, 0.9807852804032304306, 1.000000000000000000, 0.9807852804032304306, 1.000000000000000000, 0.9807852804032304306, 1.000000000000000000, 0.9807852804032304306, 1.000000000000000000, 0.9807852804032304306, 1.000000000000000000, 0.9807852804032304306, 1.000000000000000000, 0.9807852804032304306, 1.000000000000000000, 0.9807852804032304306, 1.000000000000000000, 0.9807852804032304306, 1.000000000000000000, 0.9807852804032304306, 1.000000000000000000, 0.9807852804032304306, 1.000000000000000000, 0.9807852804032304306, 1.000000000000000000, 0.9807852804032304306, 1.000000000000000000, 0.9807852804032304306, 1.000000000000000000, 0.9807852804032304306, 1.000000000000000000, 0.9807852804032304306, 1.000000000000000000, 0.9807852804032304306, 1.000000000000000000, 0.9807852804032304306, 1.000000000000000000, 0.9807852804032304306, 1.000000000000000000, 0.9807852804032304306, 1.000000000000000000, 0.9807852804032304306, 1.000000000000000000, 0.9807852804032304306, 1.000000000000000000, 0.9807852804032304306, 1.000000000000000000, 0.9807852804032304306, 1.000000000000000000, 0.9807852804032304306, 1.000000000000000000, 0.9807852804032304306, 1.000000000000000000, 0.9807852804032304306, 1.000000000000000000, 0.9807852804032304306, 1.000000000000000000, 0.9807852804032304306, 1.000000000000000000, 0.9807852804032304306, 1.000000000000000000, 0.9807852804032304306, 1.000000000000000000, 0.9807852804032304306, 1.000000000000000000, 0.9807852804032304306, 1.000000000000000000, 0.9807852804032304306, 1.000000000000000000, 0.9807852804032304306, 1.000000000000000000, 0.9807852804032304306, 1.000000000000000000, 0.9807852804032304306, 1.000000000000000000, 0.9807852804032304306, 1.000000000000000000, 0.9807852804032304306, 1.000000000000000000, 0.9807852804032304306, 1.000000000000000000, 0.9807852804032304306, 1.000000000000000000, 0.9807852804032304306, 1.000000000000000000, 0.9807852804032304306, 1.000000000000000000, 0.9807852804032304306, 1.000000000000000000, 0.9807852804032304306, 1.000000000000000000, 0.9807852804032304306, 1.000000000000000000, 0.9807852804032304306, 1.000000000000000000, 0.9807852804032304306, 1.000000000000000000, 0.9807852804032304306, 1.000000000000000000, 0.9807852804032304306, 1.000000000000000000, 0.9807852804032304306, 1.000000000000000000, 0.9807852804032304306, 1.000000000000000000, 0.9807852804032304306, 1.000000000000000000, 0.9807852804032304306, 1.000000000000000000, 0.9807852804032304306, 1.000000000000000000, 0.9807852804032304306, 1.000000000000000000, 0.9807852804032304306, 1.000000000000000000, 0.9807852804032304306, 1.000000000000000000, 0.9807852804032304306, 1.000000000000000000, 0.9807852804032304306, 1.000000000000000000, 0.9807852804032304306, 1.000000000000000000, 0.9807852804032304306, 1.000000000000000000, 0.9807852804032304306, 1.000000000000000000, 0.9807852804032304306, 1.000000000000000000, 0.9807852804032304306, 1.000000000000000000, 0.9807852804032304306, 1.000000000000000000, 0.9807852804032304306, 1.000000000000000000, 0.9807852804032304306, 1.000000000000000000, 0.9807852804032304306, 1.000000000000000000, 0.9807852804032304306, 1.000000000000000000, 0.9807852804032304306, 1.000000000000000000, 0.9807852804032304306, 1.000000000000000000, 0.9807852804032304306, 1.000000000000000000, 0.9807852804032304306, 1.000000000000000000, 0.9807852804032304306, 1.000000000000000000, 0.9807852804032304306, 1.000000000000000000, 0.9807852804032304306, 1.000000000000000000, 0.9807852804032304306, 1.000000000000000000, 0.9807852804032304306, 1.000000000000000000, 0.9807852804032304306, 1.000000000000000000, 0.9807852804032304306, 1.000000000000000000, 0.9807852804032304306, 1.000000000000000000, 0.9807852804032304306, 1.000000000000000000, 0.9807852804032304306, 1.000000000000000000, 0.9807852804032304306, 1.000000000000000000, 0.9807852804032304306, 1.000000000000000000, 0.9807852804032304306, 1.000000000000000000, 0.9807852804032304306, 1.000000000000000000, 0.9807852804032304306, 1.000000000000000000, 0.9807852804032304306, 1.000000000000000000, 0.9807852804032304306, 1.000000000000000000, 0.9807852804032304306, 1.000000000000000000, 0.9807852804032304306, 1.000000000000000000, 0.9807852804032304306, 1.000000000000000000, 0.9807852804032304306, 1.000000000000000000, 0.9807852804032304306, 1.000000000000000000, 0.9807852804032304306, 1.000000000000000000, 0.9807852804032304306, 1.000000000000000000, 0.9807852804032304306, 1.000000000000000000, 0.9807852804032304306, 1.000000000000000000, 0.9807852804032304306, 1.000000000000000000, 0.9807852804032304306, 1.000000000000000000, 0.9807852804032304306, 1.000000000000000000, 0.9807852804032304306, 1.000000000000000000, 0.9807852804032304306, 1.000000000000000000, 0.9807852804032304306, 1.000000000000000000, 0.9807852804032304306, 1.000000000000000000, 0.9807852804032304306, 1.000000000000000000, 0.9807852804032304306, 1.000000000000000000, 0.9807852804032304306, 1.000000000000000000, 0.9807852804032304306, 1.000000000000000000, 0.9807852804032304306, 1.000000000000000000, 0.9807852804032304306, 1.000000000000000000, 0.9807852804032304306, 1.000000000000000000, 0.9807852804032304306, 1.000000000000000000, 0.9807852804032304306, 1.000000000000000000, 0.9807852804032304306, 1.000000000000000000, 0.9807852804032304306, 1.000000000000000000, 0.9807852804032304306, 1.000000000000000000, 0.9807852804032304306, 1.000000000000000000, 0.9807852804032304306, 1.000000000000000000, 0.9807852804032304306, 1.000000000000000000, 0.9807852804032304306, 1.000000000000000000, 0.9807852804032304306, 1.000000000000000000, 0.9807852804032304306, 1.000000000000000000, 0.9807852804032304306, 1.000000000000000000, 0.9807852804032304306, 1.000000000000000000, 0.9807852804032304306, 1.000000000000000000, 0.9807852804032304306, 1.000000000000000000, 0.9807852804032304306, 1.000000000000000000, 0.9807852804032304306, 1.000000000000000000, 0.9807852804032304306, 1.000000000000000000, 0.9807852804032304306, 1.000000000000000000, 0.9807852804032304306, 1.000000000000000000, 0.9807852804032304306, 1.000000000000000000, 0.9807852804032304306, 1.000000000000000000, 0.9807852804032304306, 1.000000000000000000, 0.9807852804032304306, 1.000000000000000000, 0.9807852804032304306, 1.000000000000000000, 0.9807852804032304306, 1.000000000000000000, 0.9807852804032304306, 1.000000000000000000, 0.9807852804032304306, 1.000000000000000000, 0.9807852804032304306, 1.000000000000000000, 0.9807852804032304306, 1.000000000000000000, 0.9807852804032304306, 1.000000000000000000, 0.9807852804032304306, 1.000000000000000000, 0.9807852804032304306, 1.000000000000000000, 0.9807852804032304306, 1.000000000000000000, 0.9807852804032304306, 1.000000000000000000, 0.9807852804032304306, 1.000000000000000000, 0.9807852804032304306, 1.000000000000000000, 0.9807852804032304306, 1.000000000000000000, 0.9807852804032304306, 1.000000000000000000, 0.9807852804032304306, 1.000000000000000000, 0.9807852804032304306, 1.000000000000000000, 0.9807852804032304306, 1.000000000000000000, 0.9807852804032304306, 1.000000000000000000, 0.9807852804032304306, 1.000000000000000000, 0.9807852804032304306, 1.000000000000000000, 0.9807852804032304306, 1.000000000000000000, 0.9807852804032304306, 1.000000000000000000, 0.9807852804032304306, 1.000000000000000000, 0.9807852804032304306, 1.000000000000000000, 0.9807852804032304306, 1.000000000000000000, 0.9807852804032304306, 1.000000000000000000, 0.9807852804032304306, 1.000000000000000000, 0.9807852804032304306, 1.000000000000000000, 0.9807852804032304306, 1.000000000000000000, 0.9807852804032304306, 1.000000000000000000, 0.9807852804032304306, 1.000000000000000000, 0.9807852804032304306, 1.000000000000000000, 0.9807852804032304306, 1.000000000000000000, 0.9807852804032304306, 1.000000000000000000, 0.9807852804032304306, 1.000000000000000000, 0.9807852804032304306, 1.000000000000000000, 0.9807852804032304306, 1.000000000000000000, 0.9807852804032304306, 1.000000000000000000, 0.9807852804032304306, 1.000000000000000000, 0.9807852804032304306, 1.000000000000000000, 0.9807852804032304306, 1.000000000000000000, 0.9807852804032304306, 1.000000000000000000, 0.9807852804032304306, 1.000000000000000000, 0.9807852804032304306, 1.000000000000000000, 0.9807852804032304306, 1.000000000000000000, 0.9807852804032304306, 1.000000000000000000, 0.9807852804032304306, 1.000000000000000000, 0.9807852804032304306, 1.000000000000000000, 0.9807852804032304306, 1.000000000000000000, 0.9807852804032304306, 1.000000000000000000, 0.9807852804032304306, 1.000000000000000000, 0.9807852804032304306, 1.000000000000000000, 0.9807852804032304306, 1.000000000000000000, 0.9807852804032304306, 1.000000000000000000, 0.9807852804032304306, 1.000000000000000000, 0.9807852804032304306, 1.000000000000000000, 0.9807852804032304306, 1.000000000000000000, 0.9807852804032304306, 1.000000000000000000, 0.9807852804032304306, 1.000000000000000000, 0.9807852804032304306, 1.000000000000000000, 0.9807852804032304306, 1.000000000000000000, 0.9807852804032304306, 1.000000000000000000, 0.9807852804032304306, 1.000000000000000000, 0.9807852804032304306, 1.000000000000000000, 0.9807852804032304306, 1.000000000000000000, 0.9807852804032304306, 1.000000000000000000, 0.9807852804032304306, 1.000000000000000000, 0.9807852804032304306, 1.000000000000000000, 0.9807852804032304306, 1.000000000000000000, 0.9807852804032304306, 1.000000000000000000, 0.9807852804032304306, 1.000000000000000000, 0.9807852804032304306, 1.000000000000000000, 0.9807852804032304306, 1.000000000000000000, 0.9807852804032304306, 1.000000000000000000, 0.9807852804032304306, 1.000000000000000000, 0.9807852804032304306, 1.000000000000000000, 0.9807852804032304306, 1.000000000000000000, 0.9807852804032304306, 1.000000000000000000, 0.9807852804032304306, 1.000000000000000000, 0.9807852804032304306, 1.000000000000000000, 0.9807852804032304306, 1.000000000000000000, 0.9807852804032304306, 1.000000000000000000, 0.9807852804032304306, 1.000000000000000000, 0.9807852804032304306, 1.000000000000000000, 0.9807852804032304306, 1.000000000000000000, 0.9807852804032304306, 1.000000000000000000, 0.9807852804032304306, 1.000000000000000000, 0.9807852804032304306, 1.000000000000000000, 0.9807852804032304306, 1.000000000000000000, 0.9935442612832132703, 0.9914265054518418552) ) ) 
 REPRESENTATION_ITEM ( '' )  SURFACE ( )  );
#5023=CARTESIAN_POINT ( 'NONE',  ( -35.09675569278793006, 233.4948905683720284, -15.47720386886985544 ) ) ;
#5024=CARTESIAN_POINT ( 'NONE',  ( -14.48388495494899963, 367.9323905683720000, 9.489475012073732785 ) ) ;
#5026=CARTESIAN_POINT ( 'NONE',  ( -45.43829269268872650, 523.5573905683721705, -3.332260488124726194 ) ) ;
#5028=CARTESIAN_POINT ( 'NONE',  ( -38.17536295476245556, 446.9323905683720568, 14.20200298773971781 ) ) ;
#5029=CARTESIAN_POINT ( 'NONE',  ( -42.88789093042845479, 524.8073905683720568, 9.489475012073736337 ) ) ;
#5031=CARTESIAN_POINT ( 'NONE',  ( -45.64106924314019409, 496.3073905601784759, -11.32908994701042538 ) ) ;
#5032=CARTESIAN_POINT ( 'NONE',  ( -13.20868407381887444, 479.4948905683720000, -6.410867750099233042 ) ) ;
#5034=CARTESIAN_POINT ( 'NONE',  ( -16.84014894278200458, 507.6198905683720000, 11.84573899990672530 ) ) ;
#5036=CARTESIAN_POINT ( 'NONE',  ( -42.82802356641967378, 450.7448905765656377, -14.14213562373094746 ) ) ;
#5043=CARTESIAN_POINT ( 'NONE',  ( -48.68588794268862330, 436.9323905601784759, -3.978247347593371508 ) ) ;
#5044=CARTESIAN_POINT ( 'NONE',  ( -43.52287249567941529, 200.6548609068916278, -2.226397062484288814 ) ) ;
#5045=CARTESIAN_POINT ( 'NONE',  ( -25.35362745456398414, 292.5573905683720568, -16.75240474999999307 ) ) ;
#5046=CARTESIAN_POINT ( 'NONE',  ( -45.64106924314020119, 528.1823905601785327, 11.32908994701042538 ) ) ;
#5047=CARTESIAN_POINT ( 'NONE',  ( -17.35679799567828852, 273.8073905601784759, -16.95518130045146421 ) ) ;
#5049=CARTESIAN_POINT ( 'NONE',  ( -45.43829269268870519, 295.3698905683720568, 0.000000000000000000 ) ) ;
#5050=CARTESIAN_POINT ( 'NONE',  ( -44.16309181155857999, 505.9948905683720000, 6.410867750099241924 ) ) ;
#5055=CARTESIAN_POINT ( 'NONE',  ( -42.88789093042844769, 464.4323905683720000, -9.489475012073736337 ) ) ;
#5056=FACE_OUTER_BOUND ( 'NONE', #7657, .T. ) ;
#5057=CARTESIAN_POINT ( 'NONE',  ( -25.35362745456398059, 271.0573905683720000, -16.75240474999999307 ) ) ;
#5061=CARTESIAN_POINT ( 'NONE',  ( -40.53162694259542320, 254.1198905683720284, -11.84573899990672707 ) ) ;
#5062=CARTESIAN_POINT ( 'NONE',  ( -11.73070664223723192, 246.0573905765656377, 11.32908994701042005 ) ) ;
#5064=CARTESIAN_POINT ( 'NONE',  ( -17.35679799567827430, 230.6823905601784759, 16.95518130045146421 ) ) ;
#5066=CARTESIAN_POINT ( 'NONE',  ( -19.19641293061497578, 270.4323905683720000, -14.20200298773971603 ) ) ;
#5067=CARTESIAN_POINT ( 'NONE',  ( -14.48388495494899963, 361.3073905683721136, -9.489475012073736337 ) ) ;
#5070=CARTESIAN_POINT ( 'NONE',  ( -48.68588794268887199, 277.5573905601784190, 3.978247347592742678 ) ) ;
#5073=CARTESIAN_POINT ( 'NONE',  ( -11.93348319268872970, 428.8698905683720568, -2.051577885510841163E-15 ) ) ;
#5076=CARTESIAN_POINT ( 'NONE',  ( -8.685887942688729879, 431.9323905601784190, 3.978247347593161010 ) ) ;
#5080=ORIENTED_EDGE ( 'NONE', *, *, #4805, .F. ) ;
#5082=CARTESIAN_POINT ( 'NONE',  ( -32.01814843081346851, 533.1823905683720568, -16.75240474999999307 ) ) ;
#5083=CARTESIAN_POINT ( 'NONE',  ( -24.70764059509554045, 300.0573905601784759, 19.99999999999998934 ) ) ;
#5085=CARTESIAN_POINT ( 'NONE',  ( -11.93348319268872260, 340.0573905683720568, 3.332260488124728859 ) ) ;
#5086=ORIENTED_EDGE ( 'NONE', *, *, #6536, .F. ) ;
#5087=CARTESIAN_POINT ( 'NONE',  ( -24.70764059509557597, 479.1823905765656377, -19.99999999999999289 ) ) ;
#5088=CARTESIAN_POINT ( 'NONE',  ( -11.93348319268872260, 358.5573905683720000, 3.332260488124728415 ) ) ;
#5089=CARTESIAN_POINT ( 'NONE',  ( -44.16309181155856578, 364.4948905683720568, 6.410867750099241924 ) ) ;
#5091=CARTESIAN_POINT ( 'NONE',  ( -40.01497788969912506, 313.5573905765655809, 16.95518130045146776 ) ) ;
#5093=CARTESIAN_POINT ( 'NONE',  ( -11.93348319268871016, 269.1823905683720000, -3.332260488124732856 ) ) ;
#5095=CARTESIAN_POINT ( 'NONE',  ( -19.19641293061499354, 441.9323905683720568, -14.20200298773971603 ) ) ;
#5098=DIRECTION ( 'NONE',  ( -1.191790137725560488E-16, 1.000000000000000000, -0.000000000000000000 ) ) ;
#5101=CARTESIAN_POINT ( 'NONE',  ( -11.93348319268872260, 340.0573905683720000, 3.332260488124728415 ) ) ;
#5102=CARTESIAN_POINT ( 'NONE',  ( -14.48388495494901385, 479.8073905683720568, -9.489475012073736337 ) ) ;
#5104=CARTESIAN_POINT ( 'NONE',  ( -24.70764059509557597, 484.4323905601785327, -19.99999999999999289 ) ) ;
#5105=CARTESIAN_POINT ( 'NONE',  ( -22.27502019258946930, 296.9948905683720000, 15.47720386886985189 ) ) ;
#5107=CARTESIAN_POINT ( 'NONE',  ( -47.16347859291444422, 342.6198905765656377, 7.653668647301805628 ) ) ;
#5111=CARTESIAN_POINT ( 'NONE',  ( -11.93348319268872615, 400.0573905683720568, 3.332260488124728859 ) ) ;
#5112=CARTESIAN_POINT ( 'NONE',  ( -32.66413529028188378, 479.4323905601785327, 19.99999999999999289 ) ) ;
#5113=CARTESIAN_POINT ( 'NONE',  ( -14.54375231895776999, 385.7448905765656377, 14.14213562373094568 ) ) ;
#5114=CARTESIAN_POINT ( 'NONE',  ( -40.53162694259544452, 415.1198905683720000, 11.84573899990672885 ) ) ;
#5115=CARTESIAN_POINT ( 'NONE',  ( -13.20868407381884779, 269.7448905683720568, 6.410867750099229490 ) ) ;
#5116=CARTESIAN_POINT ( 'NONE',  ( -22.27502019258948707, 436.9948905683720568, 15.47720386886985189 ) ) ;
#5118=CARTESIAN_POINT ( 'NONE',  ( -14.54375231895777176, 400.9948905601785327, 14.14213562373094568 ) ) ;
#5119=CARTESIAN_POINT ( 'NONE',  ( -14.54375231895776643, 355.7448905765655809, 14.14213562373094568 ) ) ;
#5121=CARTESIAN_POINT ( 'NONE',  ( -36.33955658999051508, 390.1198905765656377, -18.47759065022572855 ) ) ;
#5122=CARTESIAN_POINT ( 'NONE',  ( -42.88789093042843348, 332.9323905683719431, -9.489475012073734561 ) ) ;
#5123=CARTESIAN_POINT ( 'NONE',  ( -28.68588794268873343, 489.4948905765656377, -19.99999999999999289 ) ) ;
#5124=CARTESIAN_POINT ( 'NONE',  ( -25.35362745456399836, 498.1823905683720000, 16.75240474999998952 ) ) ;
#5127=CARTESIAN_POINT ( 'NONE',  ( -24.70764059509556887, 464.4323905601784190, -19.99999999999999289 ) ) ;
#5128=DIRECTION ( 'NONE',  ( -1.191790137725560488E-16, 1.000000000000000000, -0.000000000000000000 ) ) ;
#5131=CARTESIAN_POINT ( 'NONE',  ( -45.43829269268871229, 405.0573905683721136, -3.332260488124726194 ) ) ;
#5133=CARTESIAN_POINT ( 'NONE',  ( -14.48388495494898365, 239.4323905683720000, 9.489475012073732785 ) ) ;
#5134=CARTESIAN_POINT ( 'NONE',  ( -38.17536295476244845, 365.4323905683720000, 14.20200298773971781 ) ) ;
#5137=CARTESIAN_POINT ( 'NONE',  ( -25.35362745456400191, 526.6823905683720568, 16.75240474999998952 ) ) ;
#5139=CARTESIAN_POINT ( 'NONE',  ( -32.01814843081344719, 447.5573905683720000, 16.75240474999999307 ) ) ;
#5140=CARTESIAN_POINT ( 'NONE',  ( -28.68588794268873698, 521.3698905683720568, -16.75240474999999307 ) ) ;
#5143=CARTESIAN_POINT ( 'NONE',  ( -48.68588794268871567, 427.2448905601784759, 0.000000000000000000 ) ) ;
#5144=CARTESIAN_POINT ( 'NONE',  ( -19.19641293061499354, 487.3073905683719431, 14.20200298773971426 ) ) ;
#5145=ORIENTED_EDGE ( 'NONE', *, *, #4677, .T. ) ;
#5146=CARTESIAN_POINT ( 'NONE',  ( -19.19641293061500065, 500.4323905683720568, -14.20200298773971603 ) ) ;
#5148=CARTESIAN_POINT ( 'NONE',  ( -36.33955658999052218, 423.8698905765655809, 18.47759065022572500 ) ) ;
#5154=CIRCLE ( 'NONE', #13448, 15.00000000000000000 ) ;
#5155=CARTESIAN_POINT ( 'NONE',  ( -12.23124753831989509, 223.9102039777117739, -11.50152087354334007 ) ) ;
#5156=( BOUNDED_CURVE ( )  B_SPLINE_CURVE ( 2, ( #18642, #5245, #11845, #5031, #10422, #18442, #5346, #17044, #2225, #14895, #16833, #3728, #10313, #3941, #17457, #10853, #15531 ),
 .UNSPECIFIED., .F., .T. ) 
 B_SPLINE_CURVE_WITH_KNOTS ( ( 3, 2, 2, 2, 2, 2, 2, 2, 3 ),
 ( 0.1250000000000001110, 0.1269531250000001110, 0.1289062500000001110, 0.1308593750000001110, 0.1328125000000001110, 0.1347656250000001388, 0.1367187500000001388, 0.1386718750000001388, 0.1406250000000001388 ),
 .UNSPECIFIED. ) 
 CURVE ( )  GEOMETRIC_REPRESENTATION_ITEM ( )  RATIONAL_B_SPLINE_CURVE ( ( 0.9999999999999988898, 0.9807852804032315408, 1.000000000000000000, 0.9807852804032304306, 1.000000000000000000, 0.9807852804032304306, 1.000000000000000000, 0.9807852804032304306, 1.000000000000000000, 0.9807852804032304306, 1.000000000000000000, 0.9807852804032304306, 1.000000000000000000, 0.9807852804032304306, 1.000000000000000000, 0.9807852804032290983, 1.000000000000001332 ) ) 
 REPRESENTATION_ITEM ( '' )  );
#5157=CARTESIAN_POINT ( 'NONE',  ( -22.27502019258947996, 292.2448905683720000, -15.47720386886985544 ) ) ;
#5159=CARTESIAN_POINT ( 'NONE',  ( -40.01497788969913216, 275.6823905601784759, -16.95518130045146421 ) ) ;
#5161=CARTESIAN_POINT ( 'NONE',  ( -22.27502019258947641, 282.2448905683720568, -15.47720386886985544 ) ) ;
#5164=CARTESIAN_POINT ( 'NONE',  ( -19.19641293061500065, 501.9323905683720000, -14.20200298773971603 ) ) ;
#5167=CARTESIAN_POINT ( 'NONE',  ( -16.84014894278200103, 461.6198905683720568, -11.84573899990672707 ) ) ;
#5168=CARTESIAN_POINT ( 'NONE',  ( -21.03221929538693047, 408.8698905765656377, -18.47759065022572855 ) ) ;
#5169=CARTESIAN_POINT ( 'NONE',  ( -19.19641293061497578, 260.4323905683720000, -14.20200298773971603 ) ) ;
#5172=CARTESIAN_POINT ( 'NONE',  ( -14.48388495494898542, 251.3073905683720284, -9.489475012073734561 ) ) ;
#5173=CARTESIAN_POINT ( 'NONE',  ( -42.82802356641964536, 250.7448905765656377, -14.14213562373094746 ) ) ;
#5175=CARTESIAN_POINT ( 'NONE',  ( -8.685887942688706786, 231.9323905601785043, 3.978247347593161010 ) ) ;
#5176=CARTESIAN_POINT ( 'NONE',  ( -44.16309181155855157, 264.4948905683720000, 6.410867750099241924 ) ) ;
#5177=CARTESIAN_POINT ( 'NONE',  ( -13.20868407381885845, 359.7448905683720568, 6.410867750099229490 ) ) ;
#5179=CARTESIAN_POINT ( 'NONE',  ( -40.01497788969915348, 505.6823905601784759, -16.95518130045146421 ) ) ;
#5185=CARTESIAN_POINT ( 'NONE',  ( -21.03221929538692692, 404.1198905601784759, -18.47759065022572855 ) ) ;
#5186=EDGE_LOOP ( 'NONE', ( #7249, #19963, #5241, #14308 ) ) ;
#5188=ORIENTED_EDGE ( 'NONE', *, *, #18160, .F. ) ;
#5189=CARTESIAN_POINT ( 'NONE',  ( -44.16309181155858710, 525.9948905683720568, 6.410867750099241924 ) ) ;
#5190=CARTESIAN_POINT ( 'NONE',  ( -14.54375231895775755, 290.9948905601784759, 14.14213562373094568 ) ) ;
#5191=CARTESIAN_POINT ( 'NONE',  ( -42.99906419454242013, 207.3703986995724335, -4.488953568700487118 ) ) ;
#5193=CARTESIAN_POINT ( 'NONE',  ( -14.48388495494899253, 319.4323905683720000, 9.489475012073731008 ) ) ;
#5194=CARTESIAN_POINT ( 'NONE',  ( -22.27502019258948707, 360.7448905683720568, -15.47720386886985544 ) ) ;
#5195=CARTESIAN_POINT ( 'NONE',  ( -19.19641293061497933, 367.3073905683720000, 14.20200298773971426 ) ) ;
#5196=CARTESIAN_POINT ( 'NONE',  ( -8.685887942688715668, 296.6823905765655809, 3.978247347593161010 ) ) ;
#5198=CARTESIAN_POINT ( 'NONE',  ( -11.93348319268871016, 268.5573905683720000, 3.332260488124728859 ) ) ;
#5199=CARTESIAN_POINT ( 'NONE',  ( -45.64106924314018698, 438.1823905601784190, 11.32908994701042538 ) ) ;
#5201=CARTESIAN_POINT ( 'NONE',  ( -11.93348319268872793, 420.6823905683720000, -3.332260488124732856 ) ) ;
#5204=CARTESIAN_POINT ( 'NONE',  ( -21.03221929538694113, 514.1198905601785327, -18.47759065022572855 ) ) ;
#5206=CARTESIAN_POINT ( 'NONE',  ( -45.64106924314018698, 408.1823905601784759, 11.32908994701042538 ) ) ;
#5207=CARTESIAN_POINT ( 'NONE',  ( -25.35362745456398770, 332.5573905683720000, -16.75240474999999307 ) ) ;
#5208=CARTESIAN_POINT ( 'NONE',  ( -25.35362745456399480, 476.6823905683720000, 16.75240474999998952 ) ) ;
#5210=CARTESIAN_POINT ( 'NONE',  ( -10.20829729246299777, 461.6198905601784759, 7.653668647301790529 ) ) ;
#5211=CARTESIAN_POINT ( 'NONE',  ( -25.35362745456398414, 311.0573905683720568, -16.75240474999999307 ) ) ;
#5212=AXIS2_PLACEMENT_3D ( 'NONE', #18871, #13809, #18983 ) ;
#5217=CARTESIAN_POINT ( 'NONE',  ( -22.27502019258949062, 382.2448905683720000, -15.47720386886985544 ) ) ;
#5218=CARTESIAN_POINT ( 'NONE',  ( -21.03221929538692336, 480.3698905601784759, 18.47759065022572500 ) ) ;
#5220=CARTESIAN_POINT ( 'NONE',  ( -11.93348319268872970, 429.1823905683720568, -3.332260488124732856 ) ) ;
#5221=CARTESIAN_POINT ( 'NONE',  ( -28.68588794268870146, 267.8698905683720000, 16.75240474999999307 ) ) ;
#5222=AXIS2_PLACEMENT_3D ( 'NONE', #14316, #2838, #9420 ) ;
#5223=CARTESIAN_POINT ( 'NONE',  ( -45.43829269268871940, 433.5573905683719431, -3.332260488124726638 ) ) ;
#5226=CARTESIAN_POINT ( 'NONE',  ( -10.20829729246298534, 357.6198905765656377, -7.653668647301794969 ) ) ;
#5227=CARTESIAN_POINT ( 'NONE',  ( -32.66413529028185536, 275.0573905601784759, -19.99999999999999289 ) ) ;
#5228=CARTESIAN_POINT ( 'NONE',  ( -8.685887942688726326, 386.9948905765655809, -2.449293598294705724E-15 ) ) ;
#5229=CARTESIAN_POINT ( 'NONE',  ( -28.68588794268870856, 326.3698905683720000, 16.75240474999999307 ) ) ;
#5231=CARTESIAN_POINT ( 'NONE',  ( -25.35362745456400546, 472.5573905683720568, -16.75240474999999307 ) ) ;
#5234=CARTESIAN_POINT ( 'NONE',  ( -42.82802356641966668, 418.4948905601784759, 14.14213562373094923 ) ) ;
#5235=CARTESIAN_POINT ( 'NONE',  ( -44.16309181155857289, 384.7448905683720000, -6.410867750099231266 ) ) ;
#5237=CARTESIAN_POINT ( 'NONE',  ( -14.48388495494898365, 231.3073905683720000, -9.489475012073736337 ) ) ;
#5238=CARTESIAN_POINT ( 'NONE',  ( -14.48388495494899786, 357.9323905683720568, 9.489475012073732785 ) ) ;
#5239=ORIENTED_EDGE ( 'NONE', *, *, #1041, .T. ) ;
#5240=CARTESIAN_POINT ( 'NONE',  ( -16.84014894278200458, 517.6198905683719431, 11.84573899990672530 ) ) ;
#5241=ORIENTED_EDGE ( 'NONE', *, *, #401, .T. ) ;
#5242=CARTESIAN_POINT ( 'NONE',  ( -14.48388495494900852, 449.4323905683721705, 9.489475012073731008 ) ) ;
#5243=CARTESIAN_POINT ( 'NONE',  ( -32.01814843081346851, 516.0573905683720568, 16.75240474999999307 ) ) ;
#5245=CARTESIAN_POINT ( 'NONE',  ( -48.68588794268863040, 496.9323905601785327, -3.978247347593371508 ) ) ;
#5246=CARTESIAN_POINT ( 'NONE',  ( -44.16309181155858710, 493.2448905683720000, -6.410867750099231266 ) ) ;
#5250=CARTESIAN_POINT ( 'NONE',  ( -38.17536295476246977, 492.3073905683720000, -14.20200298773971426 ) ) ;
#5251=CARTESIAN_POINT ( 'NONE',  ( -21.03221929538692336, 490.3698905601784759, 18.47759065022572500 ) ) ;
#5252=CARTESIAN_POINT ( 'NONE',  ( -48.68588794268871567, 421.6823905765655809, -3.978247347593158345 ) ) ;
#5255=CARTESIAN_POINT ( 'NONE',  ( -28.68588794268872988, 484.7448905601784759, -19.99999999999999289 ) ) ;
#5258=CARTESIAN_POINT ( 'NONE',  ( -8.685887942688969687, 496.6823905765655240, 3.978247347593719230 ) ) ;
#5259=CARTESIAN_POINT ( 'NONE',  ( -13.20868407381885135, 299.7448905683720568, 6.410867750099229490 ) ) ;
#5261=CARTESIAN_POINT ( 'NONE',  ( -48.68588794268873698, 573.2448905601785327, 0.000000000000000000 ) ) ;
#5262=CARTESIAN_POINT ( 'NONE',  ( -45.43829269268871940, 455.0573905683720568, -3.332260488124726194 ) ) ;
#5263=CARTESIAN_POINT ( 'NONE',  ( -36.33955658999052218, 413.8698905765655809, 18.47759065022572500 ) ) ;
#5266=CARTESIAN_POINT ( 'NONE',  ( -45.43829269268872650, 495.3698905683720568, 0.000000000000000000 ) ) ;
#5268=CARTESIAN_POINT ( 'NONE',  ( -11.93348319268873503, 470.3698905683720568, -2.051577885510841163E-15 ) ) ;
#5269=DIRECTION ( 'NONE',  ( -1.191790137725560488E-16, 1.000000000000000000, -0.000000000000000000 ) ) ;
#5270=CARTESIAN_POINT ( 'NONE',  ( -38.17536295476244135, 262.3073905683720568, -14.20200298773971426 ) ) ;
#5272=VERTEX_POINT ( 'NONE', #11159 ) ;
#5273=CARTESIAN_POINT ( 'NONE',  ( -32.66413529028186957, 334.1823905765656946, 19.99999999999999289 ) ) ;
#5274=CARTESIAN_POINT ( 'NONE',  ( -42.88789093042841927, 246.3073905683720284, 9.489475012073734561 ) ) ;
#5278=CARTESIAN_POINT ( 'NONE',  ( -40.53162694259542320, 262.6198905683720568, -11.84573899990672707 ) ) ;
#5279=CARTESIAN_POINT ( 'NONE',  ( -44.16309181155856578, 355.9948905683720000, 6.410867750099241924 ) ) ;
#5280=CARTESIAN_POINT ( 'NONE',  ( -8.685887942688738761, 502.2448905601784190, -2.449293598294705724E-15 ) ) ;
#5282=CARTESIAN_POINT ( 'NONE',  ( -35.09675569278795138, 411.9948905683720000, -15.47720386886985544 ) ) ;
#5283=CARTESIAN_POINT ( 'NONE',  ( -21.03221929538692692, 510.3698905601785896, 18.47759065022572500 ) ) ;
#5285=CARTESIAN_POINT ( 'NONE',  ( -14.54375231895777176, 400.9948905601785327, 14.14213562373094568 ) ) ;
#5286=ORIENTED_EDGE ( 'NONE', *, *, #2140, .F. ) ;
#5289=ORIENTED_EDGE ( 'NONE', *, *, #18674, .F. ) ;
#5290=CARTESIAN_POINT ( 'NONE',  ( -22.27502019258950483, 522.2448905683720568, -15.47720386886985544 ) ) ;
#5291=CARTESIAN_POINT ( 'NONE',  ( -28.68588794268870146, 289.7448905601784759, 19.99999999999999289 ) ) ;
#5293=CARTESIAN_POINT ( 'NONE',  ( -11.93348319268871549, 320.0573905683720000, 3.332260488124728859 ) ) ;
#5295=CARTESIAN_POINT ( 'NONE',  ( -40.53162694259543741, 355.1198905683720568, 11.84573899990672885 ) ) ;
#5297=CARTESIAN_POINT ( 'NONE',  ( -11.93348319268872260, 358.5573905683720000, 3.332260488124728859 ) ) ;
#5298=CARTESIAN_POINT ( 'NONE',  ( -48.68588794268870146, 312.3073905765655809, 3.978247347593168115 ) ) ;
#5300=EDGE_CURVE ( 'NONE', #14361, #10309, #14710, .T. ) ;
#5301=CARTESIAN_POINT ( 'NONE',  ( -25.35362745456398059, 261.0573905683720000, -16.75240474999999307 ) ) ;
#5302=CARTESIAN_POINT ( 'NONE',  ( -32.66413529028187668, 439.4323905601785327, 19.99999999999999289 ) ) ;
#5303=CARTESIAN_POINT ( 'NONE',  ( -25.35362745456399836, 422.5573905683721136, -16.75240474999999307 ) ) ;
#5304=CARTESIAN_POINT ( 'NONE',  ( -48.68588794268873698, 573.2448905601785327, 0.000000000000000000 ) ) ;
#5305=CARTESIAN_POINT ( 'NONE',  ( -8.685887942688720997, 352.2448905601784759, -2.449293598294705724E-15 ) ) ;
#5306=CARTESIAN_POINT ( 'NONE',  ( -8.685887942688893304, 306.6823905765655240, 3.978247347593586447 ) ) ;
#5307=CARTESIAN_POINT ( 'NONE',  ( -11.73070664223724968, 411.3073905601784759, 11.32908994701042005 ) ) ;
#5308=CARTESIAN_POINT ( 'NONE',  ( -13.20868407381885667, 330.9948905683720000, -6.410867750099233042 ) ) ;
#5309=CARTESIAN_POINT ( 'NONE',  ( -32.01814843081346140, 456.0573905683720000, 16.75240474999999307 ) ) ;
#5311=CARTESIAN_POINT ( 'NONE',  ( -48.68588794268872277, 457.5573905601784190, 3.978247347593168115 ) ) ;
#5312=CARTESIAN_POINT ( 'NONE',  ( -13.20868407381885490, 309.4948905683720568, -6.410867750099233042 ) ) ;
#5314=CARTESIAN_POINT ( 'NONE',  ( -8.685887942688898633, 341.9323905601785327, 3.978247347593586447 ) ) ;
#5316=DIRECTION ( 'NONE',  ( -1.000000000000000000, 0.000000000000000000, 0.000000000000000000 ) ) ;
#5317=CARTESIAN_POINT ( 'NONE',  ( -11.73070664223724613, 341.3073905601785327, 11.32908994701042005 ) ) ;
#5319=CARTESIAN_POINT ( 'NONE',  ( -14.48388495494900141, 389.4323905683720568, 9.489475012073731008 ) ) ;
#5320=CARTESIAN_POINT ( 'NONE',  ( -48.68588794268854514, 376.9323905601785327, -3.978247347593583783 ) ) ;
#5322=CARTESIAN_POINT ( 'NONE',  ( -42.88789093042844058, 422.9323905683720000, -9.489475012073736337 ) ) ;
#5323=CARTESIAN_POINT ( 'NONE',  ( -42.88789093042841927, 266.3073905683720000, 9.489475012073736337 ) ) ;
#5324=CARTESIAN_POINT ( 'NONE',  ( -32.01814843081344719, 421.6823905683720568, -16.75240474999999307 ) ) ;
#5327=CARTESIAN_POINT ( 'NONE',  ( -42.82802356641965957, 373.2448905765656377, 14.14213562373094923 ) ) ;
#5329=CARTESIAN_POINT ( 'NONE',  ( -40.53162694259543031, 322.6198905683720568, -11.84573899990672707 ) ) ;
#5330=CARTESIAN_POINT ( 'NONE',  ( -45.64106924314019409, 491.0573905765656377, -11.32908994701042538 ) ) ;
#5331=CARTESIAN_POINT ( 'NONE',  ( -11.93348319268873503, 480.0573905683720568, 3.332260488124728415 ) ) ;
#5332=CARTESIAN_POINT ( 'NONE',  ( -28.68588794268872277, 434.4948905765655809, 19.99999999999999289 ) ) ;
#5336=CARTESIAN_POINT ( 'NONE',  ( -44.16309181155857999, 394.7448905683720568, -6.410867750099231266 ) ) ;
#5338=CARTESIAN_POINT ( 'NONE',  ( -11.73070664223726567, 521.3073905601785327, 11.32908994701042005 ) ) ;
#5339=CARTESIAN_POINT ( 'NONE',  ( -19.19641293061498288, 367.3073905683720000, 14.20200298773971426 ) ) ;
#5340=ORIENTED_EDGE ( 'NONE', *, *, #992, .F. ) ;
#5341=CARTESIAN_POINT ( 'NONE',  ( -19.19641293061500420, 520.4323905683720568, -14.20200298773971603 ) ) ;
#5343=CARTESIAN_POINT ( 'NONE',  ( -44.16309181155859420, 523.2448905683719431, -6.410867750099231266 ) ) ;
#5346=CARTESIAN_POINT ( 'NONE',  ( -36.33955658999052218, 495.3698905601784759, -18.47759065022572855 ) ) ;
#5347=CARTESIAN_POINT ( 'NONE',  ( -16.84014894278200103, 477.6198905683720000, 11.84573899990672530 ) ) ;
#5349=CARTESIAN_POINT ( 'NONE',  ( -44.16309181155858710, 483.2448905683720000, -6.410867750099231266 ) ) ;
#5350=CARTESIAN_POINT ( 'NONE',  ( -47.16347859291445843, 487.8698905601784759, 7.653668647301805628 ) ) ;
#5351=CARTESIAN_POINT ( 'NONE',  ( -11.73070664223725679, 417.9323905765656377, -11.32908994701042715 ) ) ;
#5354=CARTESIAN_POINT ( 'NONE',  ( -45.64106924314019409, 486.3073905601785327, -11.32908994701042538 ) ) ;
#5358=CARTESIAN_POINT ( 'NONE',  ( -35.09675569278794427, 297.2448905683720000, 15.47720386886985366 ) ) ;
#5359=CARTESIAN_POINT ( 'NONE',  ( -8.685887942688616192, 232.5573905601784759, -3.978247347592952732 ) ) ;
#5360=CARTESIAN_POINT ( 'NONE',  ( -11.93348319268873148, 450.3698905683720000, -2.051577885510841163E-15 ) ) ;
#5362=CARTESIAN_POINT ( 'NONE',  ( -25.35362745456398059, 262.5573905683720000, -16.75240474999999307 ) ) ;
#5363=ORIENTED_EDGE ( 'NONE', *, *, #557, .F. ) ;
#5364=CARTESIAN_POINT ( 'NONE',  ( -21.03221929538690205, 270.3698905601784759, 18.47759065022572500 ) ) ;
#5365=CARTESIAN_POINT ( 'NONE',  ( -45.43829269268872650, 495.0573905683719431, -3.332260488124726638 ) ) ;
#5367=CARTESIAN_POINT ( 'NONE',  ( -13.20868407381887089, 469.7448905683720568, 6.410867750099229490 ) ) ;
#5369=CARTESIAN_POINT ( 'NONE',  ( -14.48388495494898720, 259.8073905683720000, -9.489475012073736337 ) ) ;
#5373=EDGE_CURVE ( 'NONE', #14145, #6799, #18417, .T. ) ;
#5375=CARTESIAN_POINT ( 'NONE',  ( -35.09675569278793716, 237.2448905683720000, 15.47720386886985366 ) ) ;
#5376=CARTESIAN_POINT ( 'NONE',  ( -45.64106924314017277, 308.1823905601784759, 11.32908994701042538 ) ) ;
#5377=CARTESIAN_POINT ( 'NONE',  ( -42.82802356641964536, 225.9948905601784759, -14.14213562373094746 ) ) ;
#5378=CARTESIAN_POINT ( 'NONE',  ( -28.68588794268870501, 271.3698905683720000, -16.75240474999999307 ) ) ;
#5379=CARTESIAN_POINT ( 'NONE',  ( -13.20868407381885845, 350.9948905683720000, -6.410867750099233042 ) ) ;
#5381=CARTESIAN_POINT ( 'NONE',  ( -17.35679799567827786, 280.6823905601784759, 16.95518130045146421 ) ) ;
#5383=AXIS2_PLACEMENT_3D ( 'NONE', #12903, #16688, #6605 ) ;
#5384=CARTESIAN_POINT ( 'NONE',  ( -40.53162694259544452, 402.6198905683720568, -11.84573899990672707 ) ) ;
#5385=CARTESIAN_POINT ( 'NONE',  ( -8.685887942688738761, 512.2448905601784190, -2.449293598294705724E-15 ) ) ;
#5386=CARTESIAN_POINT ( 'NONE',  ( -14.54375231895777532, 413.4948905601784759, -14.14213562373094746 ) ) ;
#5389=CARTESIAN_POINT ( 'NONE',  ( -45.64106924314017988, 351.0573905765656377, -11.32908994701042538 ) ) ;
#5392=CARTESIAN_POINT ( 'NONE',  ( -28.68588794268872988, 517.8698905683720568, 16.75240474999999307 ) ) ;
#5393=CARTESIAN_POINT ( 'NONE',  ( -24.70764059509555111, 284.4323905601784759, -19.99999999999999289 ) ) ;
#5396=EDGE_CURVE ( 'NONE', #4208, #629, #8043, .T. ) ;
#5397=CARTESIAN_POINT ( 'NONE',  ( -38.17536295476245556, 333.8073905683720000, -14.20200298773971426 ) ) ;
#5398=ORIENTED_EDGE ( 'NONE', *, *, #18124, .F. ) ;
#5399=CARTESIAN_POINT ( 'NONE',  ( -14.48388495494899786, 339.8073905683720568, -9.489475012073736337 ) ) ;
#5400=CARTESIAN_POINT ( 'NONE',  ( -32.01814843081344719, 366.0573905683720568, 16.75240474999999307 ) ) ;
#5402=CARTESIAN_POINT ( 'NONE',  ( -17.35679799567828496, 305.4323905765655809, 16.95518130045146421 ) ) ;
#5403=CARTESIAN_POINT ( 'NONE',  ( -48.68588794268869435, 261.9948905765655809, 0.000000000000000000 ) ) ;
#5404=CARTESIAN_POINT ( 'NONE',  ( -22.27502019258946575, 266.9948905683720000, 15.47720386886985189 ) ) ;
#5405=CARTESIAN_POINT ( 'NONE',  ( -42.91927816222972325, 203.5270276421415474, 4.734255112268844101 ) ) ;
#5406=CARTESIAN_POINT ( 'NONE',  ( -11.93348319268872793, 420.0573905683720000, 3.332260488124728415 ) ) ;
#5408=FACE_OUTER_BOUND ( 'NONE', #20228, .T. ) ;
#5409=CARTESIAN_POINT ( 'NONE',  ( -47.16347859291445843, 451.3698905765656377, -7.653668647301793193 ) ) ;
#5411=CARTESIAN_POINT ( 'NONE',  ( -45.43829269268870519, 335.6823905683720568, 3.332260488124734632 ) ) ;
#5412=CARTESIAN_POINT ( 'NONE',  ( -40.53162694259545162, 462.6198905683720000, -11.84573899990672707 ) ) ;
#5414=CARTESIAN_POINT ( 'NONE',  ( -17.35679799567830983, 473.8073905601784190, -16.95518130045146421 ) ) ;
#5415=CARTESIAN_POINT ( 'NONE',  ( -45.43829269268870519, 283.8698905683720568, 0.000000000000000000 ) ) ;
#5418=CARTESIAN_POINT ( 'NONE',  ( -17.35679799567828496, 340.6823905601785896, 16.95518130045146421 ) ) ;
#5419=ORIENTED_EDGE ( 'NONE', *, *, #1712, .F. ) ;
#5420=CARTESIAN_POINT ( 'NONE',  ( -28.68588794268874054, 573.2448905601785327, 0.000000000000000000 ) ) ;
#5421=EDGE_CURVE ( 'NONE', #7041, #3989, #8029, .T. ) ;
#5422=CARTESIAN_POINT ( 'NONE',  ( -8.685887942688720997, 342.2448905601784759, -2.449293598294705724E-15 ) ) ;
#5423=CARTESIAN_POINT ( 'NONE',  ( -45.43829269268869808, 293.5573905683720568, -3.332260488124726194 ) ) ;
#5425=CARTESIAN_POINT ( 'NONE',  ( -28.68588794268871567, 387.8698905683720000, 16.75240474999999307 ) ) ;
#5427=CARTESIAN_POINT ( 'NONE',  ( -17.35679799567829207, 385.4323905765655809, 16.95518130045146421 ) ) ;
#5428=CARTESIAN_POINT ( 'NONE',  ( -14.48388495494900496, 417.9323905683720568, 9.489475012073732785 ) ) ;
#5429=CARTESIAN_POINT ( 'NONE',  ( -11.93348319268870839, 260.3698905683720000, -2.051577885510841163E-15 ) ) ;
#5430=CARTESIAN_POINT ( 'NONE',  ( -22.27502019258949417, 420.7448905683720000, -15.47720386886985544 ) ) ;
#5431=CARTESIAN_POINT ( 'NONE',  ( -28.68588794268871567, 359.4948905765656377, -19.99999999999999289 ) ) ;
#5432=CARTESIAN_POINT ( 'NONE',  ( -11.73070664223723902, 273.1823905601785327, -11.32908994701042538 ) ) ;
#5433=CARTESIAN_POINT ( 'NONE',  ( -11.93348319268871549, 318.8698905683720000, -2.051577885510841163E-15 ) ) ;
#5435=CARTESIAN_POINT ( 'NONE',  ( -28.68588794268872633, 467.8698905683720000, 16.75240474999999307 ) ) ;
#5436=CIRCLE ( 'NONE', #12002, 20.00000000000000000 ) ;
#5437=CARTESIAN_POINT ( 'NONE',  ( -32.66413529028187668, 434.1823905765656377, 19.99999999999999289 ) ) ;
#5439=CARTESIAN_POINT ( 'NONE',  ( -8.685887942688706786, 226.9948905765656377, -2.449293598294705724E-15 ) ) ;
#5442=CARTESIAN_POINT ( 'NONE',  ( -16.84014894278199392, 381.6198905683720568, -11.84573899990672707 ) ) ;
#5444=CARTESIAN_POINT ( 'NONE',  ( -40.01497788969915348, 528.8073905601785327, 16.95518130045146776 ) ) ;
#5445=CARTESIAN_POINT ( 'NONE',  ( -16.84014894278198682, 347.6198905683720000, 11.84573899990672530 ) ) ;
#5446=ORIENTED_EDGE ( 'NONE', *, *, #5300, .F. ) ;
#5447=CARTESIAN_POINT ( 'NONE',  ( -13.20868407381888154, 529.4948905683720568, -6.410867750099233042 ) ) ;
#5451=CARTESIAN_POINT ( 'NONE',  ( -10.20829729246297646, 287.6198905765656377, -7.653668647301794969 ) ) ;
#5453=CARTESIAN_POINT ( 'NONE',  ( -45.43829269268871940, 493.5573905683720568, -3.332260488124726194 ) ) ;
#5455=CARTESIAN_POINT ( 'NONE',  ( -19.19641293061500065, 490.4323905683720568, -14.20200298773971603 ) ) ;
#5458=CARTESIAN_POINT ( 'NONE',  ( -11.73070664223725323, 416.0573905765656377, 11.32908994701042005 ) ) ;
#5461=CARTESIAN_POINT ( 'NONE',  ( -48.68588794268872277, 487.2448905601784759, 0.000000000000000000 ) ) ;
#5463=( BOUNDED_CURVE ( )  B_SPLINE_CURVE ( 2, ( #13891, #12258, #18841, #2421, #10621, #20583, #12685, #916, #4251, #4134, #14004, #2525, #9108, #1227, #19069, #15730, #2632 ),
 .UNSPECIFIED., .F., .T. ) 
 B_SPLINE_CURVE_WITH_KNOTS ( ( 3, 2, 2, 2, 2, 2, 2, 2, 3 ),
 ( 0.04687500000000040246, 0.04882812500000036082, 0.05078125000000031919, 0.05273437500000027062, 0.05468750000000022898, 0.05664062500000018735, 0.05859375000000013878, 0.06054687500000009714, 0.06250000000000005551 ),
 .UNSPECIFIED. ) 
 CURVE ( )  GEOMETRIC_REPRESENTATION_ITEM ( )  RATIONAL_B_SPLINE_CURVE ( ( 0.9999999999999960032, 0.9807852804032344274, 1.000000000000000000, 0.9807852804032304306, 1.000000000000000000, 0.9807852804032304306, 1.000000000000000000, 0.9807852804032304306, 1.000000000000000000, 0.9807852804032304306, 1.000000000000000000, 0.9807852804032304306, 1.000000000000000000, 0.9807852804032304306, 1.000000000000000000, 0.9807852804032298755, 1.000000000000000444 ) ) 
 REPRESENTATION_ITEM ( '' )  );
#5465=CARTESIAN_POINT ( 'NONE',  ( -17.35679799567827786, 240.6823905601784759, 16.95518130045146421 ) ) ;
#5467=CARTESIAN_POINT ( 'NONE',  ( -11.93348319268871371, 290.0573905683720000, 3.332260488124728415 ) ) ;
#5468=EDGE_CURVE ( 'NONE', #349, #7167, #16222, .T. ) ;
#5469=CARTESIAN_POINT ( 'NONE',  ( -14.54375231895775400, 233.4948905601784759, -14.14213562373094746 ) ) ;
#5471=CARTESIAN_POINT ( 'NONE',  ( -22.27502019258949773, 442.2448905683720000, -15.47720386886985544 ) ) ;
#5473=CARTESIAN_POINT ( 'NONE',  ( -22.27502019258947641, 272.2448905683720568, -15.47720386886985544 ) ) ;
#5475=CARTESIAN_POINT ( 'NONE',  ( -10.20829729246300666, 532.8698905601785327, -7.653668647301794969 ) ) ;
#5476=CARTESIAN_POINT ( 'NONE',  ( -11.93348319268873503, 480.0573905683720568, 3.332260488124728859 ) ) ;
#5478=CARTESIAN_POINT ( 'NONE',  ( -42.88789093042844058, 426.3073905683720000, 9.489475012073734561 ) ) ;
#5480=CARTESIAN_POINT ( 'NONE',  ( -25.35362745456397704, 251.0573905683720000, -16.75240474999999307 ) ) ;
#5484=CARTESIAN_POINT ( 'NONE',  ( -35.09675569278793716, 273.4948905683720000, -15.47720386886985544 ) ) ;
#5485=CARTESIAN_POINT ( 'NONE',  ( -28.68588794268873343, 489.4948905765656377, -19.99999999999999289 ) ) ;
#5486=FACE_OUTER_BOUND ( 'NONE', #5954, .T. ) ;
#5487=CARTESIAN_POINT ( 'NONE',  ( -22.27502019258946220, 248.4948905683720284, 15.47720386886985189 ) ) ;
#5488=CARTESIAN_POINT ( 'NONE',  ( -35.09675569278797269, 507.2448905683719431, 15.47720386886985366 ) ) ;
#5489=CARTESIAN_POINT ( 'NONE',  ( -8.685887942688706786, 232.2448905601785043, -2.449293598294705724E-15 ) ) ;
#5490=CARTESIAN_POINT ( 'NONE',  ( -11.93348319268870661, 248.8698905683720000, -2.051577885510841163E-15 ) ) ;
#5491=CARTESIAN_POINT ( 'NONE',  ( -22.27502019258947641, 358.4948905683720000, 15.47720386886985189 ) ) ;
#5494=CARTESIAN_POINT ( 'NONE',  ( -40.53162694259544452, 405.1198905683720000, 11.84573899990672885 ) ) ;
#5495=CARTESIAN_POINT ( 'NONE',  ( -24.70764059509556532, 510.0573905601785327, 19.99999999999998934 ) ) ;
#5496=CARTESIAN_POINT ( 'NONE',  ( -47.16347859291445133, 416.6198905601785327, -7.653668647301793193 ) ) ;
#5498=CARTESIAN_POINT ( 'NONE',  ( -8.685887942688720997, 346.9948905765656377, -2.449293598294705724E-15 ) ) ;
#5500=ORIENTED_EDGE ( 'NONE', *, *, #6160, .T. ) ;
#5501=CARTESIAN_POINT ( 'NONE',  ( -13.20868407381887977, 529.7448905683720568, 6.410867750099229490 ) ) ;
#5502=CARTESIAN_POINT ( 'NONE',  ( -11.73070664223724080, 293.1823905601784759, -11.32908994701042715 ) ) ;
#5505=EDGE_CURVE ( 'NONE', #19049, #17928, #15404, .T. ) ;
#5506=CARTESIAN_POINT ( 'NONE',  ( -22.27502019258947286, 328.4948905683720568, 15.47720386886985189 ) ) ;
#5508=CARTESIAN_POINT ( 'NONE',  ( -13.20868407381885845, 349.4948905683720000, -6.410867750099233042 ) ) ;
#5509=EDGE_CURVE ( 'NONE', #4217, #17801, #1408, .T. ) ;
#5510=CARTESIAN_POINT ( 'NONE',  ( -42.88789093042843348, 374.8073905683720568, 9.489475012073734561 ) ) ;
#5512=EDGE_CURVE ( 'NONE', #19311, #13531, #10251, .T. ) ;
#5513=CARTESIAN_POINT ( 'NONE',  ( -36.33955658999050087, 290.1198905765656377, -18.47759065022572855 ) ) ;
#5515=CARTESIAN_POINT ( 'NONE',  ( -14.48388495494898720, 259.8073905683720568, -9.489475012073734561 ) ) ;
#5517=CARTESIAN_POINT ( 'NONE',  ( -25.35362745456398770, 408.1823905683720568, 16.75240474999998952 ) ) ;
#5518=CARTESIAN_POINT ( 'NONE',  ( -13.68588794268874054, 573.2448905601785327, 1.836970198721029589E-15 ) ) ;
#5522=CARTESIAN_POINT ( 'NONE',  ( -19.19641293061498288, 331.9323905683720000, -14.20200298773971603 ) ) ;
#5523=CARTESIAN_POINT ( 'NONE',  ( -25.35362745456400546, 471.0573905683720568, -16.75240474999999307 ) ) ;
#5525=CARTESIAN_POINT ( 'NONE',  ( -21.03221929538693402, 464.1198905601784759, -18.47759065022572855 ) ) ;
#5526=CARTESIAN_POINT ( 'NONE',  ( -32.01814843081344009, 291.6823905683720568, -16.75240474999999307 ) ) ;
#5530=CARTESIAN_POINT ( 'NONE',  ( -48.68588794268870856, 346.9323905601784759, -3.978247347593158345 ) ) ;
#5531=CARTESIAN_POINT ( 'NONE',  ( -28.68588794268870501, 306.3698905683720568, 16.75240474999999307 ) ) ;
#5532=CARTESIAN_POINT ( 'NONE',  ( -11.93348319268872437, 390.6823905683720568, -3.332260488124732856 ) ) ;
#5534=CARTESIAN_POINT ( 'NONE',  ( -28.68588794268871567, 374.7448905601785327, -19.99999999999999289 ) ) ;
#5535=CARTESIAN_POINT ( 'NONE',  ( -21.03221929538693047, 525.1198905765655809, 18.47759065022572500 ) ) ;
#5536=CARTESIAN_POINT ( 'NONE',  ( -25.35362745456399480, 401.0573905683720000, -16.75240474999999307 ) ) ;
#5537=CARTESIAN_POINT ( 'NONE',  ( -42.88789093042841927, 254.4323905683720284, -9.489475012073736337 ) ) ;
#5538=CARTESIAN_POINT ( 'NONE',  ( -40.53162694259544452, 432.6198905683720000, -11.84573899990672707 ) ) ;
#5539=CARTESIAN_POINT ( 'NONE',  ( -45.64106924314018698, 352.9323905765656377, 11.32908994701042715 ) ) ;
#5541=CARTESIAN_POINT ( 'NONE',  ( -45.43829269268871229, 333.5573905683720568, -3.332260488124726638 ) ) ;
#5542=CARTESIAN_POINT ( 'NONE',  ( -35.09675569278796559, 477.2448905683720568, 15.47720386886985366 ) ) ;
#5543=CARTESIAN_POINT ( 'NONE',  ( -31.26501780185373391, 205.1437886375728965, 5.000000000000001776 ) ) ;
#5545=DIRECTION ( 'NONE',  ( -1.000000000000000000, 0.000000000000000000, 0.000000000000000000 ) ) ;
#5546=AXIS2_PLACEMENT_3D ( 'NONE', #18305, #18093, #10185 ) ;
#5547=CARTESIAN_POINT ( 'NONE',  ( -16.84014894278199037, 379.1198905683720568, 11.84573899990672530 ) ) ;
#5550=CARTESIAN_POINT ( 'NONE',  ( -45.64106924314020119, 518.1823905601785327, 11.32908994701042715 ) ) ;
#5551=CARTESIAN_POINT ( 'NONE',  ( -44.16309181155857289, 353.2448905683720000, -6.410867750099231266 ) ) ;
#5553=CARTESIAN_POINT ( 'NONE',  ( -14.48388495494901740, 509.8073905683720000, -9.489475012073736337 ) ) ;
#5555=CARTESIAN_POINT ( 'NONE',  ( -17.35679799567829207, 350.6823905601785327, 16.95518130045146421 ) ) ;
#5556=CARTESIAN_POINT ( 'NONE',  ( -8.685887942688641061, 417.3073905765655809, -3.978247347592952732 ) ) ;
#5557=CARTESIAN_POINT ( 'NONE',  ( -14.54375231895775400, 228.2448905765656093, -14.14213562373094746 ) ) ;
#5558=CARTESIAN_POINT ( 'NONE',  ( -28.68588794268870146, 287.8698905683720568, 16.75240474999999307 ) ) ;
#5561=CARTESIAN_POINT ( 'NONE',  ( -11.93348319268873325, 459.1823905683720000, -3.332260488124732856 ) ) ;
#5563=CARTESIAN_POINT ( 'NONE',  ( -38.17536295476246266, 485.4323905683720000, 14.20200298773971781 ) ) ;
#5566=VECTOR ( 'NONE', #9797, 1000.000000000000000 ) ;
#5567=CARTESIAN_POINT ( 'NONE',  ( -21.03221929538691626, 425.1198905765656377, 18.47759065022572500 ) ) ;
#5569=CARTESIAN_POINT ( 'NONE',  ( -21.03221929538690205, 300.3698905601784759, 18.47759065022572500 ) ) ;
#5570=DIRECTION ( 'NONE',  ( 1.191790137725560488E-16, -1.000000000000000000, 0.000000000000000000 ) ) ;
#5572=CARTESIAN_POINT ( 'NONE',  ( -48.68588794268852382, 261.6823905765655809, -3.978247347593583783 ) ) ;
#5576=CARTESIAN_POINT ( 'NONE',  ( -38.17536295476244135, 286.9323905683720000, 14.20200298773971781 ) ) ;
#5577=CARTESIAN_POINT ( 'NONE',  ( -14.54375231895775755, 253.4948905601784759, -14.14213562373094746 ) ) ;
#5578=CARTESIAN_POINT ( 'NONE',  ( -10.20829729246299067, 406.3698905765656377, 7.653668647301790529 ) ) ;
#5579=CARTESIAN_POINT ( 'NONE',  ( -42.88789093042844058, 446.3073905683720000, 9.489475012073736337 ) ) ;
#5580=CARTESIAN_POINT ( 'NONE',  ( -48.68588794268858067, 401.6823905765655809, -3.978247347593477201 ) ) ;
#5581=CARTESIAN_POINT ( 'NONE',  ( -16.84014894278197616, 269.1198905683720568, 11.84573899990672530 ) ) ;
#5583=CARTESIAN_POINT ( 'NONE',  ( -8.685887942688742314, 573.2448905601785327, 2.449293598294706119E-15 ) ) ;
#5585=CARTESIAN_POINT ( 'NONE',  ( -16.84014894278200458, 491.6198905683720000, -11.84573899990672707 ) ) ;
#5586=ORIENTED_EDGE ( 'NONE', *, *, #11731, .F. ) ;
#5587=CARTESIAN_POINT ( 'NONE',  ( -21.03221929538693047, 525.1198905765655809, 18.47759065022572500 ) ) ;
#5588=CARTESIAN_POINT ( 'NONE',  ( -42.88789093042841927, 252.9323905683720284, -9.489475012073736337 ) ) ;
#5589=ORIENTED_EDGE ( 'NONE', *, *, #9958, .T. ) ;
#5590=( BOUNDED_CURVE ( )  B_SPLINE_CURVE ( 2, ( #10089, #6627, #11503, #18100, #9981, #5013, #16390, #9765, #19616, #4793, #13248, #1565, #18313, #15091, #8358, #3503, #14766 ),
 .UNSPECIFIED., .F., .T. ) 
 B_SPLINE_CURVE_WITH_KNOTS ( ( 3, 2, 2, 2, 2, 2, 2, 2, 3 ),
 ( 0.8437500000000002220, 0.8457031250000002220, 0.8476562500000002220, 0.8496093750000002220, 0.8515625000000002220, 0.8535156250000002220, 0.8554687500000002220, 0.8574218750000002220, 0.8593750000000002220 ),
 .UNSPECIFIED. ) 
 CURVE ( )  GEOMETRIC_REPRESENTATION_ITEM ( )  RATIONAL_B_SPLINE_CURVE ( ( 0.9999999999999977796, 0.9807852804032326510, 1.000000000000000000, 0.9807852804032304306, 1.000000000000000000, 0.9807852804032304306, 1.000000000000000000, 0.9807852804032304306, 1.000000000000000000, 0.9807852804032304306, 1.000000000000000000, 0.9807852804032304306, 1.000000000000000000, 0.9807852804032304306, 1.000000000000000000, 0.9807852804032282101, 1.000000000000002220 ) ) 
 REPRESENTATION_ITEM ( '' )  );
#5591=CARTESIAN_POINT ( 'NONE',  ( -28.68588794268869790, 213.9102039777116602, 0.000000000000000000 ) ) ;
#5593=CARTESIAN_POINT ( 'NONE',  ( -40.01497788969915348, 480.4323905765655809, -16.95518130045146421 ) ) ;
#5596=CARTESIAN_POINT ( 'NONE',  ( -14.48388495494898365, 249.4323905683720284, 9.489475012073731008 ) ) ;
#5597=CARTESIAN_POINT ( 'NONE',  ( -35.09675569278797269, 517.2448905683719431, 15.47720386886985366 ) ) ;
#5599=CARTESIAN_POINT ( 'NONE',  ( -14.48388495494898542, 249.8073905683720568, -9.489475012073736337 ) ) ;
#5600=CARTESIAN_POINT ( 'NONE',  ( -13.20868407381885667, 330.9948905683720000, -6.410867750099233042 ) ) ;
#5601=CARTESIAN_POINT ( 'NONE',  ( -10.20829729246298001, 321.6198905601784759, 7.653668647301790529 ) ) ;
#5603=CARTESIAN_POINT ( 'NONE',  ( -13.20868407381886378, 408.2448905683720568, 6.410867750099229490 ) ) ;
#5604=CARTESIAN_POINT ( 'NONE',  ( -8.685887942688719221, 326.9948905765656377, -2.449293598294705724E-15 ) ) ;
#5606=CARTESIAN_POINT ( 'NONE',  ( -17.35679799567830273, 403.8073905601785327, -16.95518130045146421 ) ) ;
#5611=CARTESIAN_POINT ( 'NONE',  ( -44.16309181155859420, 514.7448905683720568, -6.410867750099231266 ) ) ;
#5612=CARTESIAN_POINT ( 'NONE',  ( -40.01497788969913216, 320.4323905765656377, -16.95518130045146421 ) ) ;
#5615=CARTESIAN_POINT ( 'NONE',  ( -42.88789093042842637, 324.4323905683720000, -9.489475012073734561 ) ) ;
#5617=CARTESIAN_POINT ( 'NONE',  ( -16.84014894278198682, 347.6198905683720000, 11.84573899990672530 ) ) ;
#5618=CARTESIAN_POINT ( 'NONE',  ( -44.16309181155856578, 354.4948905683720000, 6.410867750099241924 ) ) ;
#5619=CARTESIAN_POINT ( 'NONE',  ( -45.64106924314017988, 291.0573905765656377, -11.32908994701042715 ) ) ;
#5620=CARTESIAN_POINT ( 'NONE',  ( -36.33955658999052218, 500.1198905765655809, -18.47759065022572855 ) ) ;
#5621=CARTESIAN_POINT ( 'NONE',  ( -13.20868407381884602, 248.2448905683720000, 6.410867750099229490 ) ) ;
#5622=CARTESIAN_POINT ( 'NONE',  ( -43.58160426315849634, 200.4655464737082582, 1.772246553899823329 ) ) ;
#5623=CARTESIAN_POINT ( 'NONE',  ( -14.48388495494900496, 411.3073905683720000, -9.489475012073736337 ) ) ;
#5624=DIRECTION ( 'NONE',  ( -1.191790137725560488E-16, 1.000000000000000000, -0.000000000000000000 ) ) ;
#5625=CARTESIAN_POINT ( 'NONE',  ( -28.68588794268869435, 193.9102039777116602, 0.000000000000000000 ) ) ;
#5627=CARTESIAN_POINT ( 'NONE',  ( -13.20868407381885135, 309.7448905683720568, 6.410867750099229490 ) ) ;
#5628=CARTESIAN_POINT ( 'NONE',  ( -14.48388495494900852, 457.9323905683720568, 9.489475012073732785 ) ) ;
#5630=CARTESIAN_POINT ( 'NONE',  ( -24.70764059509557242, 464.4323905601784759, -19.99999999999999289 ) ) ;
#5631=CARTESIAN_POINT ( 'NONE',  ( -42.88789093042842637, 292.9323905683720568, -9.489475012073736337 ) ) ;
#5632=VECTOR ( 'NONE', #14090, 1000.000000000000000 ) ;
#5633=ORIENTED_EDGE ( 'NONE', *, *, #20396, .T. ) ;
#5635=CARTESIAN_POINT ( 'NONE',  ( -14.48388495494900674, 439.4323905683719431, 9.489475012073731008 ) ) ;
#5636=ORIENTED_EDGE ( 'NONE', *, *, #6246, .T. ) ;
#5638=AXIS2_PLACEMENT_3D ( 'NONE', #2872, #4488, #9025 ) ;
#5639=CARTESIAN_POINT ( 'NONE',  ( -13.20868407381885490, 309.4948905683720568, -6.410867750099233042 ) ) ;
#5640=CARTESIAN_POINT ( 'NONE',  ( -32.01814843081344719, 377.5573905683721136, 16.75240474999999307 ) ) ;
#5641=CARTESIAN_POINT ( 'NONE',  ( -36.33955658999050087, 229.1198905601785043, 18.47759065022572500 ) ) ;
#5642=CARTESIAN_POINT ( 'NONE',  ( -8.685887942688744090, 527.3073905765656946, -3.978247347593165895 ) ) ;
#5643=CARTESIAN_POINT ( 'NONE',  ( -35.09675569278795848, 395.7448905683720568, 15.47720386886985366 ) ) ;
#5644=CARTESIAN_POINT ( 'NONE',  ( -32.01814843081343298, 247.5573905683720000, 16.75240474999999307 ) ) ;
#5646=CARTESIAN_POINT ( 'NONE',  ( -19.19641293061498999, 430.4323905683720000, -14.20200298773971603 ) ) ;
#5648=CARTESIAN_POINT ( 'NONE',  ( -40.01497788969913216, 353.5573905765656377, 16.95518130045146776 ) ) ;
#5650=CARTESIAN_POINT ( 'NONE',  ( -38.17536295476244845, 302.3073905683720568, -14.20200298773971426 ) ) ;
#5651=CARTESIAN_POINT ( 'NONE',  ( -35.09675569278795848, 483.4948905683720000, -15.47720386886985544 ) ) ;
#5653=CARTESIAN_POINT ( 'NONE',  ( -8.685887942688715668, 302.2448905601784190, -2.449293598294705724E-15 ) ) ;
#5654=FACE_OUTER_BOUND ( 'NONE', #17798, .T. ) ;
#5656=AXIS2_PLACEMENT_3D ( 'NONE', #11316, #12845, #4619 ) ;
#5657=CARTESIAN_POINT ( 'NONE',  ( -32.01814843081344719, 377.5573905683720568, 16.75240474999999307 ) ) ;
#5659=CARTESIAN_POINT ( 'NONE',  ( -32.66413529028189799, 535.0573905601784190, -19.99999999999999289 ) ) ;
#5660=CARTESIAN_POINT ( 'NONE',  ( -19.19641293061498288, 340.4323905683720000, -14.20200298773971603 ) ) ;
#5662=CARTESIAN_POINT ( 'NONE',  ( -45.43829269268871940, 504.1823905683721136, 3.332260488124734632 ) ) ;
#5665=CARTESIAN_POINT ( 'NONE',  ( -48.68588794268887199, 312.3073905765655240, 3.978247347592742678 ) ) ;
#5666=CARTESIAN_POINT ( 'NONE',  ( -48.68588794268870146, 291.9948905765656377, 0.000000000000000000 ) ) ;
#5668=CARTESIAN_POINT ( 'NONE',  ( -14.48388495494901029, 459.8073905683720000, -9.489475012073736337 ) ) ;
#5670=CARTESIAN_POINT ( 'NONE',  ( -38.17536295476246977, 482.3073905683720000, -14.20200298773971426 ) ) ;
#5671=CARTESIAN_POINT ( 'NONE',  ( -40.01497788969911795, 248.8073905601784759, 16.95518130045146776 ) ) ;
#5673=CARTESIAN_POINT ( 'NONE',  ( -48.68588794268871567, 411.6823905765656377, -3.978247347593158345 ) ) ;
#5676=CARTESIAN_POINT ( 'NONE',  ( -10.20829729246299955, 482.8698905601784759, -7.653668647301794969 ) ) ;
#5679=CARTESIAN_POINT ( 'NONE',  ( -36.33955658999050087, 239.1198905601784475, 18.47759065022572500 ) ) ;
#5681=CARTESIAN_POINT ( 'NONE',  ( -44.16309181155855867, 285.9948905683720000, 6.410867750099241924 ) ) ;
#5682=CARTESIAN_POINT ( 'NONE',  ( -10.20829729246297291, 251.6198905601784759, 7.653668647301790529 ) ) ;
#5683=CARTESIAN_POINT ( 'NONE',  ( -17.35679799567829562, 405.4323905765655240, 16.95518130045146421 ) ) ;
#5684=CARTESIAN_POINT ( 'NONE',  ( -19.19641293061499354, 441.9323905683720568, -14.20200298773971603 ) ) ;
#5685=CARTESIAN_POINT ( 'NONE',  ( -36.33955658999051508, 400.1198905765656377, -18.47759065022572855 ) ) ;
#5686=CARTESIAN_POINT ( 'NONE',  ( -11.93348319268871016, 260.6823905683720000, -3.332260488124732856 ) ) ;
#5689=CARTESIAN_POINT ( 'NONE',  ( -25.35362745456399480, 488.1823905683720568, 16.75240474999998952 ) ) ;
#5691=DIRECTION ( 'NONE',  ( -1.191790137725560488E-16, 1.000000000000000000, -0.000000000000000000 ) ) ;
#5692=CARTESIAN_POINT ( 'NONE',  ( -42.88789093042841927, 232.9323905683720000, -9.489475012073736337 ) ) ;
#5694=CYLINDRICAL_SURFACE ( 'NONE', #13513, 15.00000000000000000 ) ;
#5695=CARTESIAN_POINT ( 'NONE',  ( -32.66413529028189089, 454.1823905765656377, 19.99999999999999289 ) ) ;
#5696=CARTESIAN_POINT ( 'NONE',  ( -21.03221929538691626, 308.8698905765655809, -18.47759065022572855 ) ) ;
#5697=CARTESIAN_POINT ( 'NONE',  ( -38.22409075892743857, 223.9102039777116886, -13.96110877218534085 ) ) ;
#5700=CARTESIAN_POINT ( 'NONE',  ( -35.09675569278796559, 513.4948905683720568, -15.47720386886985544 ) ) ;
#5702=CARTESIAN_POINT ( 'NONE',  ( -28.68588794268870146, 251.3698905683720000, -16.75240474999999307 ) ) ;
#5703=CARTESIAN_POINT ( 'NONE',  ( -44.16309181155857289, 344.7448905683720568, -6.410867750099231266 ) ) ;
#5704=CARTESIAN_POINT ( 'NONE',  ( -45.64106924314019409, 468.1823905601785327, 11.32908994701042538 ) ) ;
#5706=CARTESIAN_POINT ( 'NONE',  ( -14.48388495494900141, 379.8073905683720568, -9.489475012073736337 ) ) ;
#5707=CARTESIAN_POINT ( 'NONE',  ( -24.70764059509554755, 324.8073905765656377, 19.99999999999998934 ) ) ;
#5708=( BOUNDED_CURVE ( )  B_SPLINE_CURVE ( 2, ( #7416, #15985, #14042, #20624, #2673, #1166, #5587, #7739, #5799, #4182, #16303, #4708, #17901, #9783, #16085, #19743, #9679 ),
 .UNSPECIFIED., .F., .T. ) 
 B_SPLINE_CURVE_WITH_KNOTS ( ( 3, 2, 2, 2, 2, 2, 2, 2, 3 ),
 ( 0.01562500000000037470, 0.01757812500000033307, 0.01953125000000028796, 0.02148437500000024286, 0.02343750000000020123, 0.02539062500000015959, 0.02734375000000011449, 0.02929687500000006939, 0.03125000000000002776 ),
 .UNSPECIFIED. ) 
 CURVE ( )  GEOMETRIC_REPRESENTATION_ITEM ( )  RATIONAL_B_SPLINE_CURVE ( ( 0.9999999999999963363, 0.9807852804032340943, 1.000000000000000000, 0.9807852804032304306, 1.000000000000000000, 0.9807852804032304306, 1.000000000000000000, 0.9807852804032304306, 1.000000000000000000, 0.9807852804032304306, 1.000000000000000000, 0.9807852804032304306, 1.000000000000000000, 0.9807852804032304306, 1.000000000000000000, 0.9807852804032302085, 1.000000000000000222 ) ) 
 REPRESENTATION_ITEM ( '' )  );
#5709=CARTESIAN_POINT ( 'NONE',  ( -40.01497788969913216, 378.8073905601785327, 16.95518130045146776 ) ) ;
#5711=CARTESIAN_POINT ( 'NONE',  ( -8.685887942688632180, 347.3073905765656377, -3.978247347592952732 ) ) ;
#5714=CARTESIAN_POINT ( 'NONE',  ( -44.16309181155858710, 515.9948905683720568, 6.410867750099241924 ) ) ;
#5717=CARTESIAN_POINT ( 'NONE',  ( -11.93348319268871371, 300.6823905683720568, -3.332260488124732856 ) ) ;
#5719=CARTESIAN_POINT ( 'NONE',  ( -28.68588794268871212, 346.3698905683720568, 16.75240474999999307 ) ) ;
#5720=CARTESIAN_POINT ( 'NONE',  ( -28.68588794268871212, 346.3698905683720568, 16.75240474999999307 ) ) ;
#5722=CARTESIAN_POINT ( 'NONE',  ( -47.16347859291443712, 292.6198905765656377, 7.653668647301805628 ) ) ;
#5723=CARTESIAN_POINT ( 'NONE',  ( -48.68588794268855224, 396.9323905601784759, -3.978247347593583783 ) ) ;
#5724=CARTESIAN_POINT ( 'NONE',  ( -38.17536295476244135, 252.3073905683720284, -14.20200298773971426 ) ) ;
#5726=CARTESIAN_POINT ( 'NONE',  ( -32.01814843081345430, 393.1823905683721136, -16.75240474999999307 ) ) ;
#5728=CARTESIAN_POINT ( 'NONE',  ( -8.685887942688555796, 447.3073905765654672, -3.978247347592740013 ) ) ;
#5731=CARTESIAN_POINT ( 'NONE',  ( -42.88789093042844769, 464.8073905683720568, 9.489475012073736337 ) ) ;
#5732=EDGE_LOOP ( 'NONE', ( #19187, #7415, #20117, #17431 ) ) ;
#5733=CARTESIAN_POINT ( 'NONE',  ( -10.20829729246299422, 441.6198905601784759, 7.653668647301790529 ) ) ;
#5734=CARTESIAN_POINT ( 'NONE',  ( -13.20868407381884779, 278.2448905683720568, 6.410867750099229490 ) ) ;
#5737=ORIENTED_EDGE ( 'NONE', *, *, #2893, .T. ) ;
#5739=CARTESIAN_POINT ( 'NONE',  ( -28.68588794268870501, 296.3698905683720568, 16.75240474999999307 ) ) ;
#5740=CARTESIAN_POINT ( 'NONE',  ( -19.19641293061497933, 368.8073905683720000, 14.20200298773971426 ) ) ;
#5743=CARTESIAN_POINT ( 'NONE',  ( -40.01497788969916058, 530.4323905765655809, -16.95518130045146421 ) ) ;
#5744=CARTESIAN_POINT ( 'NONE',  ( -22.27502019258948351, 406.9948905683720000, 15.47720386886985189 ) ) ;
#5745=CARTESIAN_POINT ( 'NONE',  ( -42.88789093042841927, 236.3073905683720284, 9.489475012073736337 ) ) ;
#5746=CARTESIAN_POINT ( 'NONE',  ( -32.01814843081344719, 406.0573905683720000, 16.75240474999999307 ) ) ;
#5749=CARTESIAN_POINT ( 'NONE',  ( -32.66413529028187668, 349.8073905765655809, -19.99999999999999289 ) ) ;
#5751=CARTESIAN_POINT ( 'NONE',  ( -28.68588794268870501, 306.3698905683720568, 16.75240474999999307 ) ) ;
#5752=CARTESIAN_POINT ( 'NONE',  ( -40.53162694259545162, 464.1198905683720568, -11.84573899990672707 ) ) ;
#5755=CARTESIAN_POINT ( 'NONE',  ( -28.68588794268874054, 573.2448905601785327, 0.000000000000000000 ) ) ;
#5756=VECTOR ( 'NONE', #11081, 1000.000000000000000 ) ;
#5757=CARTESIAN_POINT ( 'NONE',  ( -45.43829269268871229, 375.3698905683720568, 0.000000000000000000 ) ) ;
#5759=CARTESIAN_POINT ( 'NONE',  ( -17.35679799567830983, 530.6823905601785327, 16.95518130045146421 ) ) ;
#5760=CARTESIAN_POINT ( 'NONE',  ( -42.88789093042843348, 342.9323905683721136, -9.489475012073736337 ) ) ;
#5763=CARTESIAN_POINT ( 'NONE',  ( -22.27502019258950128, 510.7448905683720000, -15.47720386886985544 ) ) ;
#5766=CARTESIAN_POINT ( 'NONE',  ( -21.03221929538692336, 354.1198905601785327, -18.47759065022572855 ) ) ;
#5767=CARTESIAN_POINT ( 'NONE',  ( -38.86787825240671168, 223.9102039777116318, -13.30301237467029019 ) ) ;
#5768=CARTESIAN_POINT ( 'NONE',  ( -45.64106924314017277, 312.9323905765655809, 11.32908994701042538 ) ) ;
#5771=CARTESIAN_POINT ( 'NONE',  ( -44.16309181155857999, 454.4948905683720568, 6.410867750099241924 ) ) ;
#5773=CARTESIAN_POINT ( 'NONE',  ( -13.20868407381887089, 468.2448905683720568, 6.410867750099229490 ) ) ;
#5777=CARTESIAN_POINT ( 'NONE',  ( -17.35679799567830273, 398.5573905765656377, -16.95518130045146421 ) ) ;
#5779=CARTESIAN_POINT ( 'NONE',  ( -14.54375231895775933, 300.9948905601784759, 14.14213562373094568 ) ) ;
#5781=CARTESIAN_POINT ( 'NONE',  ( -48.68588794268872277, 481.9948905765656377, 0.000000000000000000 ) ) ;
#5786=FACE_OUTER_BOUND ( 'NONE', #6502, .T. ) ;
#5787=CARTESIAN_POINT ( 'NONE',  ( -40.53162694259543031, 276.6198905683720568, 11.84573899990672885 ) ) ;
#5788=CARTESIAN_POINT ( 'NONE',  ( -48.68588794268869435, 256.9323905601784759, -3.978247347593158345 ) ) ;
#5789=CARTESIAN_POINT ( 'NONE',  ( -11.73070664223724791, 366.0573905765656377, 11.32908994701042005 ) ) ;
#5790=CARTESIAN_POINT ( 'NONE',  ( -35.09675569278795848, 437.2448905683720000, 15.47720386886985366 ) ) ;
#5791=CARTESIAN_POINT ( 'NONE',  ( -42.82802356641965957, 330.7448905765655809, -14.14213562373094746 ) ) ;
#5792=CARTESIAN_POINT ( 'NONE',  ( -25.35362745456396993, 268.1823905683720000, 16.75240474999998952 ) ) ;
#5793=ADVANCED_FACE ( 'NONE', ( #2822 ), #1103, .T. ) ;
#5794=VERTEX_POINT ( 'NONE', #11130 ) ;
#5796=VERTEX_POINT ( 'NONE', #9508 ) ;
#5797=CARTESIAN_POINT ( 'NONE',  ( -13.20868407381887621, 490.9948905683720568, -6.410867750099233042 ) ) ;
#5799=CARTESIAN_POINT ( 'NONE',  ( -28.68588794268873343, 524.4948905765655809, 19.99999999999999289 ) ) ;
#5800=CARTESIAN_POINT ( 'NONE',  ( -40.53162694259542320, 235.1198905683720000, 11.84573899990672885 ) ) ;
#5803=CARTESIAN_POINT ( 'NONE',  ( -47.16347859291445843, 472.6198905765656377, 7.653668647301805628 ) ) ;
#5805=CARTESIAN_POINT ( 'NONE',  ( -48.68588794268869435, 241.9948905765656377, 0.000000000000000000 ) ) ;
#5807=CARTESIAN_POINT ( 'NONE',  ( -45.43829269268869808, 225.3698905683720284, 0.000000000000000000 ) ) ;
#5808=CARTESIAN_POINT ( 'NONE',  ( -14.48388495494901740, 511.3073905683721136, -9.489475012073736337 ) ) ;
#5810=CARTESIAN_POINT ( 'NONE',  ( -19.19641293061497223, 240.4323905683720284, -14.20200298773971603 ) ) ;
#5811=CARTESIAN_POINT ( 'NONE',  ( -32.01814843081344719, 343.1823905683721136, -16.75240474999999307 ) ) ;
#5812=CARTESIAN_POINT ( 'NONE',  ( -40.01497788969914637, 468.8073905601785327, 16.95518130045146776 ) ) ;
#5813=CARTESIAN_POINT ( 'NONE',  ( -11.73070664223724613, 361.3073905601785327, 11.32908994701042005 ) ) ;
#5814=CARTESIAN_POINT ( 'NONE',  ( -32.01814843081344719, 386.0573905683720000, 16.75240474999999307 ) ) ;
#5815=CARTESIAN_POINT ( 'NONE',  ( -42.82802356641965247, 323.2448905765656377, 14.14213562373094923 ) ) ;
#5816=CARTESIAN_POINT ( 'NONE',  ( -10.20829729246298712, 381.6198905601784759, 7.653668647301790529 ) ) ;
#5821=CARTESIAN_POINT ( 'NONE',  ( -19.19641293061500065, 501.9323905683720000, -14.20200298773971603 ) ) ;
#5824=CARTESIAN_POINT ( 'NONE',  ( -19.19641293061497223, 298.8073905683719431, 14.20200298773971426 ) ) ;
#5826=CARTESIAN_POINT ( 'NONE',  ( -42.88789093042843348, 334.8073905683720000, 9.489475012073736337 ) ) ;
#5827=CARTESIAN_POINT ( 'NONE',  ( -44.16309181155857289, 343.2448905683720000, -6.410867750099231266 ) ) ;
#5829=CARTESIAN_POINT ( 'NONE',  ( -48.68588794268870146, 281.6823905765656377, -3.978247347593158345 ) ) ;
#5830=CARTESIAN_POINT ( 'NONE',  ( -32.66413529028187668, 395.0573905601784190, -19.99999999999999289 ) ) ;
#5831=CARTESIAN_POINT ( 'NONE',  ( -22.27502019258947286, 250.7448905683720000, -15.47720386886985544 ) ) ;
#5832=CARTESIAN_POINT ( 'NONE',  ( -40.01497788969914637, 463.5573905765655809, 16.95518130045146776 ) ) ;
#5833=CARTESIAN_POINT ( 'NONE',  ( -11.93348319268872437, 390.3698905683720568, -2.051577885510841163E-15 ) ) ;
#5834=VECTOR ( 'NONE', #4157, 1000.000000000000000 ) ;
#5835=DIRECTION ( 'NONE',  ( -1.191790137725560488E-16, 1.000000000000000000, -0.000000000000000000 ) ) ;
#5837=B_SPLINE_CURVE_WITH_KNOTS ( 'NONE', 3,
 ( #11305, #3096, #8155, #1264, #4927, #1475, #6538, #19530, #1371, #14684, #21051, #4813, #12943, #2891, #19425, #12836, #1695, #11524 ),
 .UNSPECIFIED., .F., .F.,
 ( 4, 2, 2, 2, 2, 2, 2, 2, 4 ),
 ( 0.01574578602456869897, 0.01672957298347709301, 0.01771335994238548706, 0.01869714690129388110, 0.01968093386020227514, 0.02066472081911067266, 0.02164850777801906670, 0.02263229473692746074, 0.02361608169583585826 ),
 .UNSPECIFIED. ) ;
#5839=( BOUNDED_CURVE ( )  B_SPLINE_CURVE ( 2, ( #1980, #8552, #15172, #11108, #13064, #11220, #2909, #1494, #3008, #11323, #14590, #7754, #17712, #9490, #12743, #16319, #4625 ),
 .UNSPECIFIED., .F., .T. ) 
 B_SPLINE_CURVE_WITH_KNOTS ( ( 3, 2, 2, 2, 2, 2, 2, 2, 3 ),
 ( 0.4843750000000002220, 0.4863281250000002220, 0.4882812500000002220, 0.4902343750000002220, 0.4921875000000002220, 0.4941406250000002220, 0.4960937500000002220, 0.4980468750000002220, 0.5000000000000002220 ),
 .UNSPECIFIED. ) 
 CURVE ( )  GEOMETRIC_REPRESENTATION_ITEM ( )  RATIONAL_B_SPLINE_CURVE ( ( 0.9999999999999977796, 0.9807852804032326510, 1.000000000000000000, 0.9807852804032304306, 1.000000000000000000, 0.9807852804032304306, 1.000000000000000000, 0.9807852804032304306, 1.000000000000000000, 0.9807852804032304306, 1.000000000000000000, 0.9807852804032304306, 1.000000000000000000, 0.9807852804032304306, 1.000000000000000000, 0.9807852804032282101, 1.000000000000002220 ) ) 
 REPRESENTATION_ITEM ( '' )  );
#5841=CARTESIAN_POINT ( 'NONE',  ( -45.43829269268871229, 444.1823905683719431, 3.332260488124734632 ) ) ;
#5843=CARTESIAN_POINT ( 'NONE',  ( -10.20829729246299600, 442.8698905601784759, -7.653668647301794969 ) ) ;
#5846=CARTESIAN_POINT ( 'NONE',  ( -47.16347859291444422, 337.8698905601785327, 7.653668647301805628 ) ) ;
#5850=CARTESIAN_POINT ( 'NONE',  ( -42.82802356641965247, 318.4948905601784759, 14.14213562373094923 ) ) ;
#5851=CARTESIAN_POINT ( 'NONE',  ( -42.88789093042842637, 294.8073905683720000, 9.489475012073736337 ) ) ;
#5853=CARTESIAN_POINT ( 'NONE',  ( -22.27502019258948707, 362.2448905683720000, -15.47720386886985544 ) ) ;
#5855=FACE_OUTER_BOUND ( 'NONE', #10368, .T. ) ;
#5856=CARTESIAN_POINT ( 'NONE',  ( -40.53162694259544452, 402.6198905683720568, -11.84573899990672707 ) ) ;
#5857=CARTESIAN_POINT ( 'NONE',  ( -45.43829269268869098, 245.6823905683720284, 3.332260488124734632 ) ) ;
#5858=CARTESIAN_POINT ( 'NONE',  ( -44.16309181155857999, 403.2448905683720568, -6.410867750099231266 ) ) ;
#5861=CARTESIAN_POINT ( 'NONE',  ( -47.16347859291444422, 342.6198905765656377, 7.653668647301805628 ) ) ;
#5862=CARTESIAN_POINT ( 'NONE',  ( -8.685887942688717445, 322.2448905601784759, -2.449293598294705724E-15 ) ) ;
#5863=CARTESIAN_POINT ( 'NONE',  ( -42.88789093042842637, 312.9323905683720000, -9.489475012073734561 ) ) ;
#5864=CARTESIAN_POINT ( 'NONE',  ( -42.88789093042844769, 456.3073905683720000, 9.489475012073736337 ) ) ;
#5865=CARTESIAN_POINT ( 'NONE',  ( -28.68588794268872277, 459.7448905601784759, 19.99999999999999289 ) ) ;
#5868=CARTESIAN_POINT ( 'NONE',  ( -19.19641293061498644, 371.9323905683720568, -14.20200298773971603 ) ) ;
#5869=CARTESIAN_POINT ( 'NONE',  ( -11.93348319268873858, 499.1823905683720568, -3.332260488124732856 ) ) ;
#5870=CARTESIAN_POINT ( 'NONE',  ( -14.54375231895778775, 513.4948905601785327, -14.14213562373094746 ) ) ;
#5871=CARTESIAN_POINT ( 'NONE',  ( -28.68588794268870856, 336.3698905683720000, 16.75240474999999307 ) ) ;
#5873=ORIENTED_EDGE ( 'NONE', *, *, #19748, .F. ) ;
#5874=CARTESIAN_POINT ( 'NONE',  ( -35.09675569278796559, 495.7448905683720000, 15.47720386886985366 ) ) ;
#5875=ORIENTED_EDGE ( 'NONE', *, *, #16648, .F. ) ;
#5878=CARTESIAN_POINT ( 'NONE',  ( -11.93348319268872793, 420.6823905683720000, -3.332260488124732856 ) ) ;
#5879=CARTESIAN_POINT ( 'NONE',  ( -17.35679799567828852, 288.5573905765655809, -16.95518130045146421 ) ) ;
#5881=CARTESIAN_POINT ( 'NONE',  ( -19.19641293061498999, 457.3073905683720568, 14.20200298773971426 ) ) ;
#5883=CARTESIAN_POINT ( 'NONE',  ( -11.93348319268873325, 459.1823905683720000, -3.332260488124732856 ) ) ;
#5884=CARTESIAN_POINT ( 'NONE',  ( -47.16347859291443001, 247.8698905601785043, 7.653668647301805628 ) ) ;
#5886=CARTESIAN_POINT ( 'NONE',  ( -17.35679799567830628, 408.5573905765655809, -16.95518130045146421 ) ) ;
#5887=CARTESIAN_POINT ( 'NONE',  ( -8.685887942688536256, 277.3073905765655240, -3.978247347592740013 ) ) ;
#5888=CARTESIAN_POINT ( 'NONE',  ( -48.68588794268854514, 371.6823905765655809, -3.978247347593583783 ) ) ;
#5893=CARTESIAN_POINT ( 'NONE',  ( -32.66413529028187668, 435.0573905601784759, -19.99999999999999289 ) ) ;
#5894=CARTESIAN_POINT ( 'NONE',  ( -10.20829729246298356, 342.8698905601785327, -7.653668647301794969 ) ) ;
#5895=AXIS2_PLACEMENT_3D ( 'NONE', #4785, #17565, #2862 ) ;
#5896=CARTESIAN_POINT ( 'NONE',  ( -22.27502019258946575, 278.4948905683720000, 15.47720386886985189 ) ) ;
#5897=CARTESIAN_POINT ( 'NONE',  ( -8.685887942688708563, 252.5573905601784759, -3.978247347593165895 ) ) ;
#5899=CARTESIAN_POINT ( 'NONE',  ( -38.17536295476246266, 433.8073905683720568, -14.20200298773971426 ) ) ;
#5900=CARTESIAN_POINT ( 'NONE',  ( -17.35679799567829917, 398.5573905765656377, -16.95518130045146421 ) ) ;
#5901=CARTESIAN_POINT ( 'NONE',  ( -38.17536295476244135, 243.8073905683720284, -14.20200298773971426 ) ) ;
#5904=CARTESIAN_POINT ( 'NONE',  ( -42.82802356641967378, 480.7448905765655809, -14.14213562373094746 ) ) ;
#5906=CARTESIAN_POINT ( 'NONE',  ( -32.01814843081345430, 477.5573905683721136, 16.75240474999999307 ) ) ;
#5909=CARTESIAN_POINT ( 'NONE',  ( -44.16309181155855867, 243.2448905683720000, -6.410867750099231266 ) ) ;
#5911=CARTESIAN_POINT ( 'NONE',  ( -13.20868407381887977, 519.4948905683720568, -6.410867750099233042 ) ) ;
#5913=CARTESIAN_POINT ( 'NONE',  ( -40.01497788969915348, 460.4323905765656377, -16.95518130045146421 ) ) ;
#5915=CARTESIAN_POINT ( 'NONE',  ( -48.68588794268855935, 456.9323905601784190, -3.978247347593583783 ) ) ;
#5917=VECTOR ( 'NONE', #11767, 1000.000000000000000 ) ;
#5919=CARTESIAN_POINT ( 'NONE',  ( -16.84014894278200813, 511.6198905683720000, -11.84573899990672707 ) ) ;
#5920=CARTESIAN_POINT ( 'NONE',  ( -21.03221929538691271, 375.1198905765656377, 18.47759065022572500 ) ) ;
#5921=CARTESIAN_POINT ( 'NONE',  ( -42.88789093042841927, 252.9323905683720284, -9.489475012073736337 ) ) ;
#5922=CARTESIAN_POINT ( 'NONE',  ( -11.93348319268871904, 330.0573905683720568, 3.332260488124728415 ) ) ;
#5924=CARTESIAN_POINT ( 'NONE',  ( -28.68588794268870146, 274.4948905765656377, 19.99999999999999289 ) ) ;
#5926=CARTESIAN_POINT ( 'NONE',  ( -40.53162694259543741, 385.1198905683720568, 11.84573899990672885 ) ) ;
#5927=CARTESIAN_POINT ( 'NONE',  ( -10.20829729246298889, 392.8698905601784759, -7.653668647301794969 ) ) ;
#5932=CARTESIAN_POINT ( 'NONE',  ( -35.09675569278796559, 497.2448905683720000, 15.47720386886985366 ) ) ;
#5935=CARTESIAN_POINT ( 'NONE',  ( -14.48388495494899075, 299.4323905683720568, 9.489475012073731008 ) ) ;
#5937=CARTESIAN_POINT ( 'NONE',  ( -11.93348319268871727, 318.5573905683720000, 3.332260488124728415 ) ) ;
#5939=CARTESIAN_POINT ( 'NONE',  ( -45.43829269268871229, 353.5573905683721136, -3.332260488124726638 ) ) ;
#5940=CARTESIAN_POINT ( 'NONE',  ( -21.03221929538690205, 275.1198905765655809, 18.47759065022572500 ) ) ;
#5942=CARTESIAN_POINT ( 'NONE',  ( -38.17536295476243424, 255.4323905683720284, 14.20200298773971781 ) ) ;
#5943=CARTESIAN_POINT ( 'NONE',  ( -35.09675569278795138, 403.4948905683720000, -15.47720386886985544 ) ) ;
#5947=CARTESIAN_POINT ( 'NONE',  ( -24.70764059509554755, 244.4323905601784475, -19.99999999999999289 ) ) ;
#5948=CARTESIAN_POINT ( 'NONE',  ( -14.48388495494900852, 449.8073905683720000, -9.489475012073736337 ) ) ;
#5951=CARTESIAN_POINT ( 'NONE',  ( -47.16347859291445133, 447.8698905601785327, 7.653668647301805628 ) ) ;
#5953=ORIENTED_EDGE ( 'NONE', *, *, #2699, .F. ) ;
#5954=EDGE_LOOP ( 'NONE', ( #15319, #14835, #8075, #16484 ) ) ;
#5956=CARTESIAN_POINT ( 'NONE',  ( -32.66413529028186957, 319.4323905601785327, 19.99999999999999289 ) ) ;
#5957=EDGE_CURVE ( 'NONE', #14447, #13267, #14832, .T. ) ;
#5958=CARTESIAN_POINT ( 'NONE',  ( -28.68588794268871567, 362.8698905683720000, -16.75240474999999307 ) ) ;
#5959=FACE_OUTER_BOUND ( 'NONE', #12594, .T. ) ;
#5961=CARTESIAN_POINT ( 'NONE',  ( -10.20829729246300310, 507.6198905765656377, -7.653668647301794969 ) ) ;
#5962=CARTESIAN_POINT ( 'NONE',  ( -11.93348319268872615, 408.5573905683720568, 3.332260488124728415 ) ) ;
#5963=CARTESIAN_POINT ( 'NONE',  ( -16.84014894278197261, 239.1198905683720284, 11.84573899990672530 ) ) ;
#5965=CARTESIAN_POINT ( 'NONE',  ( -38.17536295476245556, 415.4323905683721136, 14.20200298773971781 ) ) ;
#5966=CARTESIAN_POINT ( 'NONE',  ( -40.01497788969913927, 340.4323905765656946, -16.95518130045146421 ) ) ;
#5967=CARTESIAN_POINT ( 'NONE',  ( -14.54375231895776466, 323.4948905601784759, -14.14213562373094746 ) ) ;
#5968=CARTESIAN_POINT ( 'NONE',  ( -45.43829269268870519, 303.5573905683720568, -3.332260488124726638 ) ) ;
#5970=( BOUNDED_CURVE ( )  B_SPLINE_CURVE ( 2, ( #67, #5018, #11726, #6744, #11618, #175, #3508, #16396, #6849, #5127, #13360, #19730, #11509, #10198, #9770, #1797, #3301 ),
 .UNSPECIFIED., .F., .T. ) 
 B_SPLINE_CURVE_WITH_KNOTS ( ( 3, 2, 2, 2, 2, 2, 2, 2, 3 ),
 ( 0.2187500000000001943, 0.2207031250000001943, 0.2226562500000001943, 0.2246093750000001943, 0.2265625000000001943, 0.2285156250000001943, 0.2304687500000001943, 0.2324218750000001943, 0.2343750000000001943 ),
 .UNSPECIFIED. ) 
 CURVE ( )  GEOMETRIC_REPRESENTATION_ITEM ( )  RATIONAL_B_SPLINE_CURVE ( ( 0.9999999999999981126, 0.9807852804032323180, 1.000000000000000000, 0.9807852804032304306, 1.000000000000000000, 0.9807852804032304306, 1.000000000000000000, 0.9807852804032304306, 1.000000000000000000, 0.9807852804032304306, 1.000000000000000000, 0.9807852804032304306, 1.000000000000000000, 0.9807852804032304306, 1.000000000000000000, 0.9807852804032285432, 1.000000000000001998 ) ) 
 REPRESENTATION_ITEM ( '' )  );
#5971=CARTESIAN_POINT ( 'NONE',  ( -35.09675569278796559, 457.2448905683720568, 15.47720386886985366 ) ) ;
#5972=CARTESIAN_POINT ( 'NONE',  ( -36.33955658999052929, 459.1198905601784759, 18.47759065022572500 ) ) ;
#5976=CARTESIAN_POINT ( 'NONE',  ( -14.48388495494899963, 361.3073905683721136, -9.489475012073736337 ) ) ;
#5977=CARTESIAN_POINT ( 'NONE',  ( -11.93348319268873858, 509.1823905683719431, -3.332260488124732856 ) ) ;
#5980=CARTESIAN_POINT ( 'NONE',  ( -11.73070664223726389, 511.3073905601785327, 11.32908994701042005 ) ) ;
#5981=CARTESIAN_POINT ( 'NONE',  ( -42.88789093042842637, 322.9323905683720000, -9.489475012073736337 ) ) ;
#5984=CARTESIAN_POINT ( 'NONE',  ( -45.43829269268871940, 503.5573905683720000, -3.332260488124726194 ) ) ;
#5986=CARTESIAN_POINT ( 'NONE',  ( -8.685887942688720997, 352.2448905601784759, -2.449293598294705724E-15 ) ) ;
#5987=CARTESIAN_POINT ( 'NONE',  ( -11.93348319268872793, 420.0573905683720000, 3.332260488124728859 ) ) ;
#5988=CARTESIAN_POINT ( 'NONE',  ( -40.01497788969913927, 393.5573905765655809, 16.95518130045146776 ) ) ;
#5990=CARTESIAN_POINT ( 'NONE',  ( -44.16309181155858710, 463.2448905683720568, -6.410867750099231266 ) ) ;
#5991=ORIENTED_EDGE ( 'NONE', *, *, #2055, .T. ) ;
#5992=CARTESIAN_POINT ( 'NONE',  ( -25.35362745456399125, 456.6823905683720000, 16.75240474999998952 ) ) ;
#5993=CARTESIAN_POINT ( 'NONE',  ( -11.73070664223723192, 251.3073905601784759, 11.32908994701042005 ) ) ;
#5995=CARTESIAN_POINT ( 'NONE',  ( -17.35679799567829917, 405.4323905765655240, 16.95518130045146421 ) ) ;
#6000=VECTOR ( 'NONE', #12385, 1000.000000000000000 ) ;
#6003=CARTESIAN_POINT ( 'NONE',  ( -43.91866333689311830, 223.9102039777115749, 10.20022563105532676 ) ) ;
#6004=CARTESIAN_POINT ( 'NONE',  ( -17.35679799567828496, 243.8073905601784475, -16.95518130045146421 ) ) ;
#6005=CARTESIAN_POINT ( 'NONE',  ( -14.54375231895776821, 365.7448905765656377, 14.14213562373094568 ) ) ;
#6006=CARTESIAN_POINT ( 'NONE',  ( -32.01814843081345430, 433.1823905683721136, -16.75240474999999307 ) ) ;
#6008=CARTESIAN_POINT ( 'NONE',  ( -45.43829269268869098, 255.6823905683720000, 3.332260488124734632 ) ) ;
#6009=EDGE_CURVE ( 'NONE', #9261, #5794, #19811, .T. ) ;
#6012=DIRECTION ( 'NONE',  ( -1.000000000000000000, -1.191790137725560488E-16, 0.000000000000000000 ) ) ;
#6014=CARTESIAN_POINT ( 'NONE',  ( -14.48388495494901029, 461.3073905683720568, -9.489475012073734561 ) ) ;
#6015=ORIENTED_EDGE ( 'NONE', *, *, #11793, .F. ) ;
#6017=CARTESIAN_POINT ( 'NONE',  ( -40.53162694259542320, 242.6198905683720284, -11.84573899990672707 ) ) ;
#6019=CARTESIAN_POINT ( 'NONE',  ( -11.93348319268874036, 518.8698905683719431, -2.051577885510841163E-15 ) ) ;
#6021=CARTESIAN_POINT ( 'NONE',  ( -48.68588794268872277, 461.6823905765656377, -3.978247347593158345 ) ) ;
#6023=CARTESIAN_POINT ( 'NONE',  ( -21.03221929538690205, 285.1198905765656377, 18.47759065022572500 ) ) ;
#6024=CARTESIAN_POINT ( 'NONE',  ( -35.32494336579074456, 223.9102039777116602, -16.19735568274630921 ) ) ;
#6025=CARTESIAN_POINT ( 'NONE',  ( -13.20868407381884424, 229.7448905683720568, 6.410867750099229490 ) ) ;
#6026=LINE ( 'NONE', #19124, #18384 ) ;
#6027=CARTESIAN_POINT ( 'NONE',  ( -21.25396403206155682, 220.6412462828192247, -15.05426855923459328 ) ) ;
#6028=CARTESIAN_POINT ( 'NONE',  ( -25.35362745456398770, 332.5573905683720000, -16.75240474999999307 ) ) ;
#6030=CARTESIAN_POINT ( 'NONE',  ( -40.53162694259543031, 314.1198905683720568, -11.84573899990672707 ) ) ;
#6031=CARTESIAN_POINT ( 'NONE',  ( -38.17536295476245556, 382.3073905683719431, -14.20200298773971426 ) ) ;
#6032=CARTESIAN_POINT ( 'NONE',  ( -38.17536295476246977, 526.9323905683720568, 14.20200298773971781 ) ) ;
#6034=CARTESIAN_POINT ( 'NONE',  ( -48.68588794268870856, 387.5573905601784759, 3.978247347593168115 ) ) ;
#6039=CARTESIAN_POINT ( 'NONE',  ( -14.48388495494901740, 511.3073905683721136, -9.489475012073736337 ) ) ;
#6042=CARTESIAN_POINT ( 'NONE',  ( -25.35362745456397349, 308.1823905683719431, 16.75240474999998952 ) ) ;
#6043=CARTESIAN_POINT ( 'NONE',  ( -35.09675569278793716, 321.9948905683720568, -15.47720386886985544 ) ) ;
#6045=CARTESIAN_POINT ( 'NONE',  ( -17.35679799567828852, 258.5573905765655809, -16.95518130045146421 ) ) ;
#6046=CARTESIAN_POINT ( 'NONE',  ( -48.68588794268871567, 397.2448905601784759, 0.000000000000000000 ) ) ;
#6047=CARTESIAN_POINT ( 'NONE',  ( -25.35362745456396638, 236.6823905683720284, 16.75240474999998952 ) ) ;
#6048=EDGE_CURVE ( 'NONE', #4866, #15132, #623, .T. ) ;
#6049=CARTESIAN_POINT ( 'NONE',  ( -28.68588794268871922, 402.8698905683720000, -16.75240474999999307 ) ) ;
#6053=CARTESIAN_POINT ( 'NONE',  ( -24.70764059509557597, 509.1823905765655809, -19.99999999999999289 ) ) ;
#6054=CARTESIAN_POINT ( 'NONE',  ( -40.53162694259544452, 435.1198905683720000, 11.84573899990672885 ) ) ;
#6056=CARTESIAN_POINT ( 'NONE',  ( -8.685887942688729879, 442.2448905601785327, -2.449293598294705724E-15 ) ) ;
#6059=ORIENTED_EDGE ( 'NONE', *, *, #14317, .T. ) ;
#6061=CYLINDRICAL_SURFACE ( 'NONE', #21155, 19.99999999999999645 ) ;
#6062=CARTESIAN_POINT ( 'NONE',  ( -47.16347859291443712, 327.8698905601785327, 7.653668647301805628 ) ) ;
#6063=CARTESIAN_POINT ( 'NONE',  ( -42.88789093042843348, 356.3073905683720000, 9.489475012073734561 ) ) ;
#6064=CYLINDRICAL_SURFACE ( 'NONE', #3135, 19.99999999999999645 ) ;
#6065=CARTESIAN_POINT ( 'NONE',  ( -21.03221929538694113, 498.8698905765656377, -18.47759065022572855 ) ) ;
#6066=CARTESIAN_POINT ( 'NONE',  ( -45.43829269268871940, 393.8698905683720000, 0.000000000000000000 ) ) ;
#6067=CARTESIAN_POINT ( 'NONE',  ( -45.43829269268869098, 235.6823905683720284, 3.332260488124734632 ) ) ;
#6068=CARTESIAN_POINT ( 'NONE',  ( -11.93348319268872615, 408.8698905683720568, -2.051577885510841163E-15 ) ) ;
#6069=CARTESIAN_POINT ( 'NONE',  ( -45.64106924314017988, 321.0573905765656377, -11.32908994701042715 ) ) ;
#6071=CARTESIAN_POINT ( 'NONE',  ( -19.19641293061497578, 300.4323905683720568, -14.20200298773971603 ) ) ;
#6072=CARTESIAN_POINT ( 'NONE',  ( -16.84014894278199748, 449.1198905683720568, 11.84573899990672530 ) ) ;
#6074=CARTESIAN_POINT ( 'NONE',  ( -28.68588794268871212, 369.7448905601785327, 19.99999999999999289 ) ) ;
#6075=CARTESIAN_POINT ( 'NONE',  ( -8.685887942688729879, 432.2448905601785327, -2.449293598294705724E-15 ) ) ;
#6076=CARTESIAN_POINT ( 'NONE',  ( -19.19641293061498288, 358.8073905683720000, 14.20200298773971426 ) ) ;
#6077=CARTESIAN_POINT ( 'NONE',  ( -45.43829269268871940, 494.1823905683720000, 3.332260488124734632 ) ) ;
#6078=CARTESIAN_POINT ( 'NONE',  ( -11.73070664223726745, 503.1823905601785327, -11.32908994701042715 ) ) ;
#6079=CARTESIAN_POINT ( 'NONE',  ( -32.01814843081344719, 331.6823905683720000, -16.75240474999999307 ) ) ;
#6080=AXIS2_PLACEMENT_3D ( 'NONE', #4884, #6821, #13226 ) ;
#6083=ORIENTED_EDGE ( 'NONE', *, *, #15630, .F. ) ;
#6086=CARTESIAN_POINT ( 'NONE',  ( -32.01814843081344719, 423.1823905683721136, -16.75240474999999307 ) ) ;
#6087=CARTESIAN_POINT ( 'NONE',  ( -42.82802356641964536, 233.2448905765656093, 14.14213562373094923 ) ) ;
#6089=CARTESIAN_POINT ( 'NONE',  ( -14.48388495494900852, 439.8073905683721136, -9.489475012073736337 ) ) ;
#6091=CARTESIAN_POINT ( 'NONE',  ( -45.43829269268872650, 474.1823905683720000, 3.332260488124734632 ) ) ;
#6092=CARTESIAN_POINT ( 'NONE',  ( -21.03221929538693047, 414.1198905601785327, -18.47759065022572855 ) ) ;
#6093=CARTESIAN_POINT ( 'NONE',  ( -21.03221929538693047, 408.8698905765656377, -18.47759065022572855 ) ) ;
#6101=DIRECTION ( 'NONE',  ( -1.191790137725560488E-16, 1.000000000000000000, -0.000000000000000000 ) ) ;
#6102=CARTESIAN_POINT ( 'NONE',  ( -47.16347859291444422, 346.6198905601784190, -7.653668647301793193 ) ) ;
#6104=CARTESIAN_POINT ( 'NONE',  ( -28.68588794268869790, 239.7448905601785043, 19.99999999999999289 ) ) ;
#6106=CARTESIAN_POINT ( 'NONE',  ( -8.685887942688911068, 451.9323905601784759, 3.978247347593586447 ) ) ;
#6107=CARTESIAN_POINT ( 'NONE',  ( -14.48388495494900674, 431.3073905683719431, -9.489475012073736337 ) ) ;
#6109=CARTESIAN_POINT ( 'NONE',  ( -25.35362745456397704, 252.5573905683720284, -16.75240474999999307 ) ) ;
#6110=VERTEX_POINT ( 'NONE', #11377 ) ;
#6111=ORIENTED_EDGE ( 'NONE', *, *, #15232, .T. ) ;
#6112=CARTESIAN_POINT ( 'NONE',  ( -45.64106924314018698, 422.9323905765656946, 11.32908994701042538 ) ) ;
#6114=CARTESIAN_POINT ( 'NONE',  ( -45.43829269268872650, 465.6823905683720000, 3.332260488124734632 ) ) ;
#6115=CARTESIAN_POINT ( 'NONE',  ( -36.33955658999050087, 233.8698905765656093, 18.47759065022572500 ) ) ;
#6117=AXIS2_PLACEMENT_3D ( 'NONE', #20052, #3608, #10193 ) ;
#6120=CARTESIAN_POINT ( 'NONE',  ( -22.27502019258947286, 230.7448905683720000, -15.47720386886985544 ) ) ;
#6122=CARTESIAN_POINT ( 'NONE',  ( -45.43829269268873361, 533.5573905683720568, -3.332260488124726638 ) ) ;
#6124=CARTESIAN_POINT ( 'NONE',  ( -14.54375231895777887, 465.7448905765655809, 14.14213562373094568 ) ) ;
#6125=PRODUCT_DEFINITION_SHAPE ( 'NONE', 'NONE',  #4341 ) ;
#6129=CARTESIAN_POINT ( 'NONE',  ( -14.48388495494898365, 231.3073905683720284, -9.489475012073734561 ) ) ;
#6131=CARTESIAN_POINT ( 'NONE',  ( -8.882341142746135176, 223.9102039777117454, 3.228969530591021098 ) ) ;
#6132=CARTESIAN_POINT ( 'NONE',  ( -44.16309181155855157, 224.4948905683720284, 6.410867750099241924 ) ) ;
#6133=CARTESIAN_POINT ( 'NONE',  ( -13.20868407381885490, 310.9948905683720568, -6.410867750099233042 ) ) ;
#6134=CARTESIAN_POINT ( 'NONE',  ( -42.82802356641966668, 445.9948905601784759, -14.14213562373094746 ) ) ;
#6136=CARTESIAN_POINT ( 'NONE',  ( -14.48388495494899253, 301.3073905683720568, -9.489475012073736337 ) ) ;
#6137=CARTESIAN_POINT ( 'NONE',  ( -44.16309181155857289, 383.2448905683720000, -6.410867750099231266 ) ) ;
#6138=CARTESIAN_POINT ( 'NONE',  ( -11.93348319268874036, 520.0573905683719431, 3.332260488124728859 ) ) ;
#6139=CARTESIAN_POINT ( 'NONE',  ( -24.70764059509556532, 394.4323905601784190, -19.99999999999999289 ) ) ;
#6140=CARTESIAN_POINT ( 'NONE',  ( -36.33955658999049376, 230.1198905765656093, -18.47759065022572855 ) ) ;
#6143=CARTESIAN_POINT ( 'NONE',  ( -14.48388495494901562, 491.3073905683720000, -9.489475012073736337 ) ) ;
#6146=CARTESIAN_POINT ( 'NONE',  ( -22.27502019258946930, 288.4948905683720000, 15.47720386886985189 ) ) ;
#6147=CARTESIAN_POINT ( 'NONE',  ( -11.93348319268871904, 328.5573905683720568, 3.332260488124728415 ) ) ;
#6148=CARTESIAN_POINT ( 'NONE',  ( -14.54375231895775578, 265.7448905765656377, 14.14213562373094568 ) ) ;
#6151=CARTESIAN_POINT ( 'NONE',  ( -32.01814843081344719, 373.1823905683720000, -16.75240474999999307 ) ) ;
#6153=DIRECTION ( 'NONE',  ( -1.000000000000000000, 0.000000000000000000, 0.000000000000000000 ) ) ;
#6154=CARTESIAN_POINT ( 'NONE',  ( -8.685887942688742314, 573.2448905601785327, 2.449293598294706119E-15 ) ) ;
#6156=CARTESIAN_POINT ( 'NONE',  ( -40.53162694259544452, 442.6198905683720568, -11.84573899990672707 ) ) ;
#6159=CARTESIAN_POINT ( 'NONE',  ( -40.01497788969914637, 445.6823905601784759, -16.95518130045146421 ) ) ;
#6160=EDGE_CURVE ( 'NONE', #9040, #13902, #12488, .T. ) ;
#6164=CARTESIAN_POINT ( 'NONE',  ( -14.54375231895776288, 330.9948905601784190, 14.14213562373094568 ) ) ;
#6165=CARTESIAN_POINT ( 'NONE',  ( -10.20829729246298712, 377.6198905765655809, -7.653668647301794969 ) ) ;
#6166=EDGE_CURVE ( 'NONE', #16379, #18572, #19797, .T. ) ;
#6169=CARTESIAN_POINT ( 'NONE',  ( -45.43829269268871229, 365.3698905683720568, 0.000000000000000000 ) ) ;
#6170=CARTESIAN_POINT ( 'NONE',  ( -48.68588794268878672, 227.5573905601784475, 3.978247347592954952 ) ) ;
#6171=CARTESIAN_POINT ( 'NONE',  ( -45.64106924314020119, 502.9323905765656946, 11.32908994701042715 ) ) ;
#6172=CARTESIAN_POINT ( 'NONE',  ( -11.93348319268872260, 378.5573905683721136, 3.332260488124728415 ) ) ;
#6173=CARTESIAN_POINT ( 'NONE',  ( -20.29730442459490547, 222.0357903062123341, -14.50085278415678403 ) ) ;
#6174=CARTESIAN_POINT ( 'NONE',  ( -35.09675569278795848, 415.7448905683720000, 15.47720386886985366 ) ) ;
#6176=CARTESIAN_POINT ( 'NONE',  ( -40.01497788969913216, 320.4323905765655809, -16.95518130045146421 ) ) ;
#6178=CARTESIAN_POINT ( 'NONE',  ( -11.93348319268871194, 288.5573905683720000, 3.332260488124728859 ) ) ;
#6179=CARTESIAN_POINT ( 'NONE',  ( -44.16309181155858710, 464.7448905683720568, -6.410867750099231266 ) ) ;
#6181=CARTESIAN_POINT ( 'NONE',  ( -40.01497788969914637, 458.8073905601784759, 16.95518130045146776 ) ) ;
#6184=CARTESIAN_POINT ( 'NONE',  ( -40.53162694259543741, 374.1198905683720000, -11.84573899990672707 ) ) ;
#6185=CARTESIAN_POINT ( 'NONE',  ( -16.84014894278200458, 507.6198905683720000, 11.84573899990672530 ) ) ;
#6186=CARTESIAN_POINT ( 'NONE',  ( -48.68588794268872277, 506.9323905601784759, -3.978247347593158345 ) ) ;
#6187=CARTESIAN_POINT ( 'NONE',  ( -22.27502019258948351, 320.7448905683720000, -15.47720386886985544 ) ) ;
#6189=VERTEX_POINT ( 'NONE', #20246 ) ;
#6190=CARTESIAN_POINT ( 'NONE',  ( -8.685887942688740537, 522.2448905601784190, -2.449293598294705724E-15 ) ) ;
#6193=CARTESIAN_POINT ( 'NONE',  ( -14.48388495494900674, 429.4323905683720000, 9.489475012073731008 ) ) ;
#6194=CARTESIAN_POINT ( 'NONE',  ( -48.68588794268887909, 392.3073905765655240, 3.978247347592742678 ) ) ;
#6195=FACE_OUTER_BOUND ( 'NONE', #13821, .T. ) ;
#6196=CARTESIAN_POINT ( 'NONE',  ( -45.43829269268871940, 453.5573905683720568, -3.332260488124726194 ) ) ;
#6198=CARTESIAN_POINT ( 'NONE',  ( -42.88789093042844769, 472.9323905683720568, -9.489475012073734561 ) ) ;
#6201=CARTESIAN_POINT ( 'NONE',  ( -40.01497788969913216, 383.5573905765655809, 16.95518130045146776 ) ) ;
#6209=CARTESIAN_POINT ( 'NONE',  ( -11.93348319268872970, 430.6823905683720568, -3.332260488124732856 ) ) ;
#6210=CARTESIAN_POINT ( 'NONE',  ( -40.01497788969913927, 385.6823905601784190, -16.95518130045146421 ) ) ;
#6211=CARTESIAN_POINT ( 'NONE',  ( -13.20868407381884779, 240.9948905683720284, -6.410867750099233042 ) ) ;
#6212=ORIENTED_EDGE ( 'NONE', *, *, #16648, .T. ) ;
#6216=CARTESIAN_POINT ( 'NONE',  ( -45.43829269268872650, 465.0573905683720568, -3.332260488124726638 ) ) ;
#6217=CARTESIAN_POINT ( 'NONE',  ( -42.82802356641964536, 223.2448905765656093, 14.14213562373094923 ) ) ;
#6219=VECTOR ( 'NONE', #8574, 1000.000000000000000 ) ;
#6222=CARTESIAN_POINT ( 'NONE',  ( -32.01814843081346851, 533.1823905683720568, -16.75240474999999307 ) ) ;
#6224=CARTESIAN_POINT ( 'NONE',  ( -14.48388495494901740, 527.9323905683720568, 9.489475012073731008 ) ) ;
#6227=CARTESIAN_POINT ( 'NONE',  ( -36.33955658999052218, 433.8698905765655809, 18.47759065022572500 ) ) ;
#6228=CARTESIAN_POINT ( 'NONE',  ( -21.03221929538690915, 350.3698905601784759, 18.47759065022572500 ) ) ;
#6231=CARTESIAN_POINT ( 'NONE',  ( -13.68588794268874054, 573.2448905601785327, 1.836970198721029589E-15 ) ) ;
#6232=PLANE ( 'NONE',  #5656 ) ;
#6233=CARTESIAN_POINT ( 'NONE',  ( -8.685887942688726326, 406.9948905765656377, -2.449293598294705724E-15 ) ) ;
#6236=CARTESIAN_POINT ( 'NONE',  ( -28.68588794268871212, 322.8698905683720000, -16.75240474999999307 ) ) ;
#6240=CARTESIAN_POINT ( 'NONE',  ( -25.35362745456398414, 302.5573905683720000, -16.75240474999999307 ) ) ;
#6242=CARTESIAN_POINT ( 'NONE',  ( -40.53162694259543741, 355.1198905683720568, 11.84573899990672885 ) ) ;
#6244=CARTESIAN_POINT ( 'NONE',  ( -22.27502019258949417, 518.4948905683719431, 15.47720386886985189 ) ) ;
#6245=CARTESIAN_POINT ( 'NONE',  ( -42.82802356641965957, 375.9948905601784759, -14.14213562373094746 ) ) ;
#6246=EDGE_CURVE ( 'NONE', #11848, #15984, #20766, .T. ) ;
#6249=CARTESIAN_POINT ( 'NONE',  ( -28.68588794268872988, 482.8698905683720568, -16.75240474999999307 ) ) ;
#6251=CARTESIAN_POINT ( 'NONE',  ( -16.84014894278198327, 290.1198905683720568, -11.84573899990672707 ) ) ;
#6253=CARTESIAN_POINT ( 'NONE',  ( -25.35362745456398059, 282.5573905683720568, -16.75240474999999307 ) ) ;
#6254=CARTESIAN_POINT ( 'NONE',  ( -25.35362745456397704, 316.6823905683720000, 16.75240474999998952 ) ) ;
#6255=CARTESIAN_POINT ( 'NONE',  ( -35.09675569278793006, 263.4948905683720000, -15.47720386886985544 ) ) ;
#6256=CARTESIAN_POINT ( 'NONE',  ( -14.54375231895775400, 255.7448905765656377, 14.14213562373094568 ) ) ;
#6257=CARTESIAN_POINT ( 'NONE',  ( -47.16347859291445843, 476.6198905601785327, -7.653668647301793193 ) ) ;
#6258=CARTESIAN_POINT ( 'NONE',  ( -11.93348319268870483, 228.8698905683720284, -2.051577885510841163E-15 ) ) ;
#6259=CARTESIAN_POINT ( 'NONE',  ( -32.01814843081344719, 383.1823905683720568, -16.75240474999999307 ) ) ;
#6264=CARTESIAN_POINT ( 'NONE',  ( -22.27502019258949773, 450.7448905683720000, -15.47720386886985544 ) ) ;
#6267=CARTESIAN_POINT ( 'NONE',  ( -45.64106924314019409, 426.3073905601785327, -11.32908994701042715 ) ) ;
#6273=CARTESIAN_POINT ( 'NONE',  ( -28.68588794268870856, 319.7448905601785327, 19.99999999999999289 ) ) ;
#6274=CARTESIAN_POINT ( 'NONE',  ( -28.68588794268869790, 223.9102039777116602, 0.000000000000000000 ) ) ;
#6276=CARTESIAN_POINT ( 'NONE',  ( -13.20868407381885845, 350.9948905683720000, -6.410867750099233042 ) ) ;
#6277=CARTESIAN_POINT ( 'NONE',  ( -48.68588794268872988, 511.6823905765655809, -3.978247347593158345 ) ) ;
#6278=CARTESIAN_POINT ( 'NONE',  ( -28.68588794268871922, 391.3698905683720000, -16.75240474999999307 ) ) ;
#6279=CARTESIAN_POINT ( 'NONE',  ( -25.35362745456396283, 228.1823905683720284, 16.75240474999998952 ) ) ;
#6280=CARTESIAN_POINT ( 'NONE',  ( -22.27502019258947996, 376.9948905683720568, 15.47720386886985189 ) ) ;
#6281=CARTESIAN_POINT ( 'NONE',  ( -11.73070664223724613, 317.9323905765656377, -11.32908994701042715 ) ) ;
#6283=CARTESIAN_POINT ( 'NONE',  ( -45.43829269268870519, 293.8698905683720568, 0.000000000000000000 ) ) ;
#6285=CARTESIAN_POINT ( 'NONE',  ( -32.01814843081345430, 447.5573905683720000, 16.75240474999999307 ) ) ;
#6290=CARTESIAN_POINT ( 'NONE',  ( -35.09675569278795138, 347.2448905683720000, 15.47720386886985366 ) ) ;
#6291=CARTESIAN_POINT ( 'NONE',  ( -42.88789093042844769, 502.9323905683720000, -9.489475012073736337 ) ) ;
#6292=CARTESIAN_POINT ( 'NONE',  ( -14.54375231895778242, 490.9948905601784759, 14.14213562373094568 ) ) ;
#6293=CARTESIAN_POINT ( 'NONE',  ( -42.88789093042843348, 332.9323905683720568, -9.489475012073736337 ) ) ;
#6302=CARTESIAN_POINT ( 'NONE',  ( -25.35362745456398770, 408.1823905683720000, 16.75240474999998952 ) ) ;
#6303=CARTESIAN_POINT ( 'NONE',  ( -48.68588794268870146, 291.9948905765656377, 0.000000000000000000 ) ) ;
#6304=CARTESIAN_POINT ( 'NONE',  ( -42.88789093042844769, 452.9323905683720568, -9.489475012073736337 ) ) ;
#6305=ORIENTED_EDGE ( 'NONE', *, *, #14782, .F. ) ;
#6306=CARTESIAN_POINT ( 'NONE',  ( -45.43829269268872650, 453.5573905683720568, -3.332260488124726638 ) ) ;
#6309=CARTESIAN_POINT ( 'NONE',  ( -10.20829729246298889, 386.3698905765656377, 7.653668647301790529 ) ) ;
#6310=CARTESIAN_POINT ( 'NONE',  ( -31.26501780185373391, 205.1437886375728965, 0.000000000000000000 ) ) ;
#6311=CARTESIAN_POINT ( 'NONE',  ( -47.16347859291444422, 371.3698905765655809, -7.653668647301793193 ) ) ;
#6312=CARTESIAN_POINT ( 'NONE',  ( -14.54375231895777887, 428.2448905765656377, -14.14213562373094746 ) ) ;
#6314=CARTESIAN_POINT ( 'NONE',  ( -25.35362745456400901, 502.5573905683719431, -16.75240474999999307 ) ) ;
#6319=CARTESIAN_POINT ( 'NONE',  ( -11.93348319268872615, 410.3698905683720568, -2.051577885510841163E-15 ) ) ;
#6320=CARTESIAN_POINT ( 'NONE',  ( -21.03221929538690205, 265.1198905765655809, 18.47759065022572500 ) ) ;
#6321=CARTESIAN_POINT ( 'NONE',  ( -40.53162694259542320, 244.1198905683720284, -11.84573899990672707 ) ) ;
#6324=DIRECTION ( 'NONE',  ( -1.191790137725560488E-16, 1.000000000000000000, -0.000000000000000000 ) ) ;
#6325=VERTEX_POINT ( 'NONE', #2402 ) ;
#6326=CARTESIAN_POINT ( 'NONE',  ( -11.93348319268873503, 470.3698905683720568, -2.051577885510841163E-15 ) ) ;
#6327=CARTESIAN_POINT ( 'NONE',  ( -11.73070664223723014, 226.0573905765655809, 11.32908994701042005 ) ) ;
#6330=CARTESIAN_POINT ( 'NONE',  ( -8.685887942688729879, 432.2448905601785327, -2.449293598294705724E-15 ) ) ;
#6331=CARTESIAN_POINT ( 'NONE',  ( -19.19641293061497223, 230.4323905683720000, -14.20200298773971603 ) ) ;
#6334=CARTESIAN_POINT ( 'NONE',  ( -22.27502019258950483, 530.7448905683720568, -15.47720386886985544 ) ) ;
#6336=CARTESIAN_POINT ( 'NONE',  ( -21.03221929538693402, 448.8698905765656377, -18.47759065022572855 ) ) ;
#6337=CARTESIAN_POINT ( 'NONE',  ( -13.20868407381885667, 338.2448905683720568, 6.410867750099229490 ) ) ;
#6338=CARTESIAN_POINT ( 'NONE',  ( -47.16347859291445843, 452.6198905765656377, 7.653668647301805628 ) ) ;
#6339=CARTESIAN_POINT ( 'NONE',  ( -14.54375231895775578, 238.2448905765656093, -14.14213562373094746 ) ) ;
#6340=CARTESIAN_POINT ( 'NONE',  ( -36.33955658999050797, 289.1198905601785327, 18.47759065022572500 ) ) ;
#6343=CARTESIAN_POINT ( 'NONE',  ( -22.27502019258948351, 322.2448905683720000, -15.47720386886985544 ) ) ;
#6344=CARTESIAN_POINT ( 'NONE',  ( -8.685887942688742314, 532.2448905601784190, -2.449293598294705724E-15 ) ) ;
#6347=CARTESIAN_POINT ( 'NONE',  ( -16.84014894278197971, 309.1198905683720000, 11.84573899990672530 ) ) ;
#6349=CARTESIAN_POINT ( 'NONE',  ( -45.43829269268873361, 515.3698905683720568, 0.000000000000000000 ) ) ;
#6350=CARTESIAN_POINT ( 'NONE',  ( -45.64106924314018698, 376.3073905601784759, -11.32908994701042715 ) ) ;
#6353=CARTESIAN_POINT ( 'NONE',  ( -44.16309181155858710, 484.7448905683720568, -6.410867750099231266 ) ) ;
#6355=CARTESIAN_POINT ( 'NONE',  ( -28.68588794268870146, 276.3698905683720000, 16.75240474999999307 ) ) ;
#6357=CARTESIAN_POINT ( 'NONE',  ( -11.93348319268871016, 280.3698905683720000, -2.051577885510841163E-15 ) ) ;
#6358=CARTESIAN_POINT ( 'NONE',  ( -38.17536295476244135, 325.4323905683720000, 14.20200298773971781 ) ) ;
#6359=CARTESIAN_POINT ( 'NONE',  ( -38.17536295476243424, 256.9323905683720000, 14.20200298773971781 ) ) ;
#6360=CARTESIAN_POINT ( 'NONE',  ( -48.68588794268869435, 261.9948905765655809, 0.000000000000000000 ) ) ;
#6361=CARTESIAN_POINT ( 'NONE',  ( -10.20829729246299955, 472.8698905601784759, -7.653668647301794969 ) ) ;
#6362=CARTESIAN_POINT ( 'NONE',  ( -42.88789093042841927, 224.8073905683720000, 9.489475012073734561 ) ) ;
#6363=CARTESIAN_POINT ( 'NONE',  ( -22.27502019258947641, 368.4948905683720568, 15.47720386886985189 ) ) ;
#6364=EDGE_CURVE ( 'NONE', #8749, #18802, #896, .T. ) ;
#6366=CARTESIAN_POINT ( 'NONE',  ( -8.685887942688710339, 262.2448905601784759, -2.449293598294705724E-15 ) ) ;
#6368=CARTESIAN_POINT ( 'NONE',  ( -40.53162694259544452, 422.6198905683720000, -11.84573899990672707 ) ) ;
#6371=CARTESIAN_POINT ( 'NONE',  ( -28.68588794268872277, 424.7448905601784759, -19.99999999999999289 ) ) ;
#6374=ORIENTED_EDGE ( 'NONE', *, *, #388, .F. ) ;
#6376=CARTESIAN_POINT ( 'NONE',  ( -40.01497788969912506, 308.8073905601784759, 16.95518130045146776 ) ) ;
#6379=CARTESIAN_POINT ( 'NONE',  ( -28.68588794268870856, 337.8698905683720000, 16.75240474999999307 ) ) ;
#6380=CARTESIAN_POINT ( 'NONE',  ( -21.03221929538694113, 508.8698905765656377, -18.47759065022572855 ) ) ;
#6381=CARTESIAN_POINT ( 'NONE',  ( -44.16309181155857999, 393.2448905683720568, -6.410867750099231266 ) ) ;
#6382=CARTESIAN_POINT ( 'NONE',  ( -45.43829269268869098, 225.0573905683720568, -3.332260488124726194 ) ) ;
#6383=CARTESIAN_POINT ( 'NONE',  ( -13.20868407381886200, 388.2448905683720000, 6.410867750099229490 ) ) ;
#6384=CARTESIAN_POINT ( 'NONE',  ( -14.54375231895776643, 328.2448905765656377, -14.14213562373094746 ) ) ;
#6385=CARTESIAN_POINT ( 'NONE',  ( -48.68588794268871567, 427.2448905601784759, 0.000000000000000000 ) ) ;
#6386=CARTESIAN_POINT ( 'NONE',  ( -11.93348319268871016, 278.5573905683720568, 3.332260488124728859 ) ) ;
#6388=CARTESIAN_POINT ( 'NONE',  ( -45.43829269268871229, 445.6823905683720000, 3.332260488124734632 ) ) ;
#6390=CARTESIAN_POINT ( 'NONE',  ( -36.33955658999050087, 285.3698905601784759, -18.47759065022572855 ) ) ;
#6393=CARTESIAN_POINT ( 'NONE',  ( -35.09675569278794427, 353.4948905683720000, -15.47720386886985544 ) ) ;
#6394=CARTESIAN_POINT ( 'NONE',  ( -45.43829269268871940, 473.5573905683720000, -3.332260488124726194 ) ) ;
#6395=CARTESIAN_POINT ( 'NONE',  ( -48.68588794268872277, 477.2448905601784759, 0.000000000000000000 ) ) ;
#6396=CARTESIAN_POINT ( 'NONE',  ( -14.48388495494899608, 329.8073905683720000, -9.489475012073736337 ) ) ;
#6401=( BOUNDED_CURVE ( )  B_SPLINE_CURVE ( 2, ( #8683, #6848, #4030, #3817, #18628, #20369, #16818, #20166, #5332, #5437, #13464, #15410, #3613, #16924, #11933, #8576, #11831 ),
 .UNSPECIFIED., .F., .T. ) 
 B_SPLINE_CURVE_WITH_KNOTS ( ( 3, 2, 2, 2, 2, 2, 2, 2, 3 ),
 ( 0.2968750000000001110, 0.2988281250000001110, 0.3007812500000001110, 0.3027343750000001110, 0.3046875000000001110, 0.3066406250000001110, 0.3085937500000001110, 0.3105468750000001110, 0.3125000000000001110 ),
 .UNSPECIFIED. ) 
 CURVE ( )  GEOMETRIC_REPRESENTATION_ITEM ( )  RATIONAL_B_SPLINE_CURVE ( ( 0.9999999999999988898, 0.9807852804032315408, 1.000000000000000000, 0.9807852804032304306, 1.000000000000000000, 0.9807852804032304306, 1.000000000000000000, 0.9807852804032304306, 1.000000000000000000, 0.9807852804032304306, 1.000000000000000000, 0.9807852804032304306, 1.000000000000000000, 0.9807852804032304306, 1.000000000000000000, 0.9807852804032293204, 1.000000000000001110 ) ) 
 REPRESENTATION_ITEM ( '' )  );
#6402=CARTESIAN_POINT ( 'NONE',  ( -42.88789093042844058, 406.3073905683719431, 9.489475012073734561 ) ) ;
#6403=CARTESIAN_POINT ( 'NONE',  ( -32.66413529028187668, 394.1823905765655809, 19.99999999999999289 ) ) ;
#6405=CARTESIAN_POINT ( 'NONE',  ( -16.84014894278200103, 440.1198905683720568, -11.84573899990672707 ) ) ;
#6406=CARTESIAN_POINT ( 'NONE',  ( -45.43829269268871940, 443.8698905683720568, 0.000000000000000000 ) ) ;
#6407=CARTESIAN_POINT ( 'NONE',  ( -48.68588794268873698, 573.2448905601785327, 0.000000000000000000 ) ) ;
#6408=CARTESIAN_POINT ( 'NONE',  ( -10.20829729246298889, 387.6198905765655809, -7.653668647301794969 ) ) ;
#6410=CARTESIAN_POINT ( 'NONE',  ( -11.73070664223725323, 387.9323905765656377, -11.32908994701042538 ) ) ;
#6413=CARTESIAN_POINT ( 'NONE',  ( -40.53162694259545162, 504.1198905683720568, -11.84573899990672707 ) ) ;
#6415=CARTESIAN_POINT ( 'NONE',  ( -45.64106924314018698, 418.1823905601784759, 11.32908994701042538 ) ) ;
#6417=CARTESIAN_POINT ( 'NONE',  ( -42.88789093042844058, 416.3073905683720568, 9.489475012073736337 ) ) ;
#6418=CARTESIAN_POINT ( 'NONE',  ( -28.68588794268871922, 384.7448905601785327, -19.99999999999999289 ) ) ;
#6419=CARTESIAN_POINT ( 'NONE',  ( -25.35362745456396283, 228.1823905683720284, 16.75240474999998952 ) ) ;
#6422=CARTESIAN_POINT ( 'NONE',  ( -14.54375231895777532, 425.7448905765656377, 14.14213562373094568 ) ) ;
#6423=EDGE_LOOP ( 'NONE', ( #14122, #10495 ) ) ;
#6424=CARTESIAN_POINT ( 'NONE',  ( -42.88789093042844769, 454.4323905683720568, -9.489475012073734561 ) ) ;
#6425=CARTESIAN_POINT ( 'NONE',  ( -17.35679799567827430, 225.4323905765655809, 16.95518130045146421 ) ) ;
#6429=CARTESIAN_POINT ( 'NONE',  ( -44.16309181155855157, 224.4948905683720284, 6.410867750099241924 ) ) ;
#6431=EDGE_LOOP ( 'NONE', ( #4316, #2920, #6613, #11994 ) ) ;
#6432=CARTESIAN_POINT ( 'NONE',  ( -44.16309181155857999, 504.4948905683720568, 6.410867750099241924 ) ) ;
#6436=CARTESIAN_POINT ( 'NONE',  ( -42.82802356641967378, 453.2448905765656377, 14.14213562373094923 ) ) ;
#6438=CARTESIAN_POINT ( 'NONE',  ( -11.73070664223724258, 331.3073905601785327, 11.32908994701042005 ) ) ;
#6443=CARTESIAN_POINT ( 'NONE',  ( -40.53162694259542320, 222.6198905683720000, -11.84573899990672707 ) ) ;
#6444=CARTESIAN_POINT ( 'NONE',  ( -25.35362745456398414, 312.5573905683720000, -16.75240474999999307 ) ) ;
#6446=CARTESIAN_POINT ( 'NONE',  ( -17.35679799567830628, 443.8073905601784759, -16.95518130045146421 ) ) ;
#6447=CARTESIAN_POINT ( 'NONE',  ( -42.82802356641964536, 268.4948905601784759, 14.14213562373094923 ) ) ;
#6449=CARTESIAN_POINT ( 'NONE',  ( -35.09675569278794427, 287.2448905683720000, 15.47720386886985366 ) ) ;
#6451=CARTESIAN_POINT ( 'NONE',  ( -25.35362745456401257, 522.5573905683720568, -16.75240474999999307 ) ) ;
#6452=CARTESIAN_POINT ( 'NONE',  ( -28.68588794268871567, 374.7448905601785327, -19.99999999999999289 ) ) ;
#6453=VECTOR ( 'NONE', #5624, 1000.000000000000000 ) ;
#6454=CARTESIAN_POINT ( 'NONE',  ( -24.70764059509555111, 314.4323905601784190, -19.99999999999999289 ) ) ;
#6456=CARTESIAN_POINT ( 'NONE',  ( -40.53162694259545162, 486.6198905683720000, 11.84573899990672885 ) ) ;
#6458=CARTESIAN_POINT ( 'NONE',  ( -40.53162694259543031, 285.1198905683720568, 11.84573899990672885 ) ) ;
#6459=ORIENTED_EDGE ( 'NONE', *, *, #7452, .F. ) ;
#6460=CARTESIAN_POINT ( 'NONE',  ( -38.17536295476244135, 276.9323905683720000, 14.20200298773971781 ) ) ;
#6461=CARTESIAN_POINT ( 'NONE',  ( -25.35362745456398414, 311.0573905683720568, -16.75240474999999307 ) ) ;
#6462=CARTESIAN_POINT ( 'NONE',  ( -11.93348319268870839, 260.0573905683720000, 3.332260488124728859 ) ) ;
#6464=CARTESIAN_POINT ( 'NONE',  ( -36.33955658999049376, 260.1198905765655809, -18.47759065022572855 ) ) ;
#6466=CARTESIAN_POINT ( 'NONE',  ( -22.27502019258949062, 382.2448905683720000, -15.47720386886985544 ) ) ;
#6471=CARTESIAN_POINT ( 'NONE',  ( -32.66413529028185536, 269.8073905765655809, -19.99999999999999289 ) ) ;
#6473=CARTESIAN_POINT ( 'NONE',  ( -14.48388495494900674, 429.8073905683720000, -9.489475012073736337 ) ) ;
#6476=CARTESIAN_POINT ( 'NONE',  ( -24.70764059509556887, 434.4323905601784759, -19.99999999999999289 ) ) ;
#6481=CARTESIAN_POINT ( 'NONE',  ( -24.70764059509555466, 304.4323905601784759, -19.99999999999999289 ) ) ;
#6482=CARTESIAN_POINT ( 'NONE',  ( -42.88454851406326185, 206.4494888775581103, -4.837634058829628714 ) ) ;
#6484=CARTESIAN_POINT ( 'NONE',  ( -42.88789093042843348, 336.3073905683720568, 9.489475012073734561 ) ) ;
#6485=CARTESIAN_POINT ( 'NONE',  ( -11.73070664223726389, 477.9323905765656377, -11.32908994701042715 ) ) ;
#6486=CARTESIAN_POINT ( 'NONE',  ( -19.19641293061498644, 360.4323905683720000, -14.20200298773971603 ) ) ;
#6487=CARTESIAN_POINT ( 'NONE',  ( -45.43829269268869808, 225.3698905683720284, 0.000000000000000000 ) ) ;
#6488=CARTESIAN_POINT ( 'NONE',  ( -45.43829269268871229, 383.5573905683720000, -3.332260488124726638 ) ) ;
#6489=CARTESIAN_POINT ( 'NONE',  ( -48.68588794268870146, 321.9948905765655809, 0.000000000000000000 ) ) ;
#6492=CARTESIAN_POINT ( 'NONE',  ( -16.84014894278197971, 280.1198905683720000, -11.84573899990672707 ) ) ;
#6494=CARTESIAN_POINT ( 'NONE',  ( -16.84014894278199748, 431.6198905683720000, -11.84573899990672707 ) ) ;
#6496=CARTESIAN_POINT ( 'NONE',  ( -28.68588794268872988, 499.7448905601785327, 19.99999999999999289 ) ) ;
#6498=CARTESIAN_POINT ( 'NONE',  ( -8.685887942688731655, 452.2448905601784759, -2.449293598294705724E-15 ) ) ;
#6499=CARTESIAN_POINT ( 'NONE',  ( -25.35362745456398770, 342.5573905683720568, -16.75240474999999307 ) ) ;
#6500=CARTESIAN_POINT ( 'NONE',  ( -44.16309181155857999, 484.4948905683720000, 6.410867750099241924 ) ) ;
#6502=EDGE_LOOP ( 'NONE', ( #12886, #5145, #1960, #7766, #6810, #17299, #15693 ) ) ;
#6503=CARTESIAN_POINT ( 'NONE',  ( -45.64106924314020119, 486.3073905601785327, -11.32908994701042715 ) ) ;
#6504=CARTESIAN_POINT ( 'NONE',  ( -40.53162694259543031, 302.6198905683720000, -11.84573899990672707 ) ) ;
#6511=CARTESIAN_POINT ( 'NONE',  ( -16.84014894278199037, 399.1198905683720000, 11.84573899990672530 ) ) ;
#6514=CARTESIAN_POINT ( 'NONE',  ( -11.93348319268872970, 438.8698905683720568, -2.051577885510841163E-15 ) ) ;
#6515=CARTESIAN_POINT ( 'NONE',  ( -14.48388495494901029, 439.8073905683721136, -9.489475012073734561 ) ) ;
#6516=CARTESIAN_POINT ( 'NONE',  ( -8.685887942688726326, 412.2448905601784759, -2.449293598294705724E-15 ) ) ;
#6517=CARTESIAN_POINT ( 'NONE',  ( -17.35679799567829562, 385.4323905765655809, 16.95518130045146421 ) ) ;
#6518=CARTESIAN_POINT ( 'NONE',  ( -28.68588794268874054, 573.2448905601785327, 0.000000000000000000 ) ) ;
#6520=CARTESIAN_POINT ( 'NONE',  ( -8.685887942688628627, 487.3073905765656377, -3.978247347592898553 ) ) ;
#6521=CARTESIAN_POINT ( 'NONE',  ( -45.43829269268871940, 505.6823905683720568, 3.332260488124734632 ) ) ;
#6524=CARTESIAN_POINT ( 'NONE',  ( -14.54375231895778597, 520.9948905601784190, 14.14213562373094568 ) ) ;
#6526=ADVANCED_FACE ( 'NONE', ( #10680 ), #7117, .T. ) ;
#6527=CARTESIAN_POINT ( 'NONE',  ( -22.27502019258949062, 402.2448905683720568, -15.47720386886985544 ) ) ;
#6528=CARTESIAN_POINT ( 'NONE',  ( -47.16347859291443001, 262.6198905765655809, 7.653668647301805628 ) ) ;
#6529=( BOUNDED_CURVE ( )  B_SPLINE_CURVE ( 2, ( #18950, #1224, #15934, #4248, #17337, #20799, #2627, #12580, #2522, #7474, #14104, #14323, #5967, #20687, #2844, #19174, #5862 ),
 .UNSPECIFIED., .F., .T. ) 
 B_SPLINE_CURVE_WITH_KNOTS ( ( 3, 2, 2, 2, 2, 2, 2, 2, 3 ),
 ( 0.6562500000000000000, 0.6582031250000000000, 0.6601562500000000000, 0.6621093750000001110, 0.6640625000000001110, 0.6660156250000001110, 0.6679687500000002220, 0.6699218750000002220, 0.6718750000000002220 ),
 .UNSPECIFIED. ) 
 CURVE ( )  GEOMETRIC_REPRESENTATION_ITEM ( )  RATIONAL_B_SPLINE_CURVE ( ( 1.000000000000000000, 0.9807852804032304306, 1.000000000000000000, 0.9807852804032304306, 1.000000000000000000, 0.9807852804032304306, 1.000000000000000000, 0.9807852804032304306, 1.000000000000000000, 0.9807852804032304306, 1.000000000000000000, 0.9807852804032304306, 1.000000000000000000, 0.9807852804032304306, 1.000000000000000000, 0.9807852804032282101, 1.000000000000002220 ) ) 
 REPRESENTATION_ITEM ( '' )  );
#6530=CARTESIAN_POINT ( 'NONE',  ( -14.48388495494898187, 229.4323905683720000, 9.489475012073732785 ) ) ;
#6533=ORIENTED_EDGE ( 'NONE', *, *, #14198, .F. ) ;
#6534=CARTESIAN_POINT ( 'NONE',  ( -22.27502019258948707, 448.4948905683720568, 15.47720386886985189 ) ) ;
#6535=CARTESIAN_POINT ( 'NONE',  ( -14.54375231895775222, 235.7448905765656093, 14.14213562373094568 ) ) ;
#6536=EDGE_CURVE ( 'NONE', #18572, #16379, #13609, .T. ) ;
#6538=CARTESIAN_POINT ( 'NONE',  ( -43.47609127650945737, 209.4774105891669933, 2.515022083182097745 ) ) ;
#6539=CARTESIAN_POINT ( 'NONE',  ( -45.43829269268872650, 535.0573905683720568, -3.332260488124726194 ) ) ;
#6541=CARTESIAN_POINT ( 'NONE',  ( -35.09675569278795848, 501.9948905683720000, -15.47720386886985544 ) ) ;
#6544=CARTESIAN_POINT ( 'NONE',  ( -10.20829729246299422, 436.3698905765656377, 7.653668647301790529 ) ) ;
#6545=CARTESIAN_POINT ( 'NONE',  ( -42.82802356641965957, 360.7448905765656377, -14.14213562373094746 ) ) ;
#6546=CARTESIAN_POINT ( 'NONE',  ( -40.01497788969912506, 328.8073905601784759, 16.95518130045146776 ) ) ;
#6547=CARTESIAN_POINT ( 'NONE',  ( -48.68588794268870146, 307.2448905601784759, 0.000000000000000000 ) ) ;
#6552=CARTESIAN_POINT ( 'NONE',  ( -45.43829269268869808, 315.0573905683720000, -3.332260488124726194 ) ) ;
#6554=CARTESIAN_POINT ( 'NONE',  ( -8.685887942688712116, 272.2448905601784759, -2.449293598294705724E-15 ) ) ;
#6556=CARTESIAN_POINT ( 'NONE',  ( -32.01814843081344009, 287.5573905683719431, 16.75240474999999307 ) ) ;
#6557=CARTESIAN_POINT ( 'NONE',  ( -42.88789093042845479, 506.3073905683720568, 9.489475012073734561 ) ) ;
#6558=CARTESIAN_POINT ( 'NONE',  ( -14.54375231895776999, 363.4948905601784759, -14.14213562373094746 ) ) ;
#6560=ORIENTED_EDGE ( 'NONE', *, *, #18795, .T. ) ;
#6561=CARTESIAN_POINT ( 'NONE',  ( -13.20868407381887444, 480.9948905683720000, -6.410867750099233042 ) ) ;
#6563=CARTESIAN_POINT ( 'NONE',  ( -25.35362745456396993, 276.6823905683720000, 16.75240474999998952 ) ) ;
#6568=CARTESIAN_POINT ( 'NONE',  ( -42.88789093042842637, 274.4323905683720568, -9.489475012073734561 ) ) ;
#6569=CARTESIAN_POINT ( 'NONE',  ( -45.43829269268869808, 255.0573905683720000, -3.332260488124726638 ) ) ;
#6570=CARTESIAN_POINT ( 'NONE',  ( -45.64106924314017277, 241.0573905765656093, -11.32908994701042715 ) ) ;
#6573=CARTESIAN_POINT ( 'NONE',  ( -14.48388495494898365, 229.8073905683720284, -9.489475012073734561 ) ) ;
#6574=CARTESIAN_POINT ( 'NONE',  ( -44.16309181155855867, 274.4948905683720000, 6.410867750099241924 ) ) ;
#6575=CARTESIAN_POINT ( 'NONE',  ( -11.93348319268872260, 380.3698905683720568, -2.051577885510841163E-15 ) ) ;
#6579=CARTESIAN_POINT ( 'NONE',  ( -24.70764059509556887, 459.1823905765656946, -19.99999999999999289 ) ) ;
#6581=CARTESIAN_POINT ( 'NONE',  ( -11.93348319268872793, 418.8698905683720568, -2.051577885510841163E-15 ) ) ;
#6584=CARTESIAN_POINT ( 'NONE',  ( -10.20829729246299422, 432.8698905601784759, -7.653668647301794969 ) ) ;
#6589=CARTESIAN_POINT ( 'NONE',  ( -28.68588794268870856, 314.7448905601785327, -19.99999999999999289 ) ) ;
#6591=CARTESIAN_POINT ( 'NONE',  ( -38.17536295476244845, 346.9323905683720568, 14.20200298773971781 ) ) ;
#6594=CARTESIAN_POINT ( 'NONE',  ( -47.16347859291445843, 491.3698905765655809, -7.653668647301793193 ) ) ;
#6595=CARTESIAN_POINT ( 'NONE',  ( -45.43829269268871229, 363.8698905683720000, 0.000000000000000000 ) ) ;
#6596=CARTESIAN_POINT ( 'NONE',  ( -45.43829269268869098, 225.6823905683720568, 3.332260488124734632 ) ) ;
#6597=CARTESIAN_POINT ( 'NONE',  ( -14.48388495494900141, 387.9323905683720000, 9.489475012073731008 ) ) ;
#6598=CARTESIAN_POINT ( 'NONE',  ( -28.68588794268870856, 299.4948905765656377, -19.99999999999999289 ) ) ;
#6600=CARTESIAN_POINT ( 'NONE',  ( -22.27502019258947996, 290.7448905683720568, -15.47720386886985544 ) ) ;
#6601=CARTESIAN_POINT ( 'NONE',  ( -28.68588794268874054, 573.2448905601785327, 0.000000000000000000 ) ) ;
#6602=CARTESIAN_POINT ( 'NONE',  ( -13.20868407381886733, 429.7448905683720000, 6.410867750099229490 ) ) ;
#6603=CARTESIAN_POINT ( 'NONE',  ( -42.82802356641965247, 285.9948905601784759, -14.14213562373094746 ) ) ;
#6604=CARTESIAN_POINT ( 'NONE',  ( -42.82802356641968089, 515.9948905601785327, -14.14213562373094746 ) ) ;
#6605=DIRECTION ( 'NONE',  ( -1.000000000000000000, 0.000000000000000000, 0.000000000000000000 ) ) ;
#6606=CARTESIAN_POINT ( 'NONE',  ( -8.685887942688726326, 402.2448905601784759, -2.449293598294705724E-15 ) ) ;
#6607=CARTESIAN_POINT ( 'NONE',  ( -44.16309181155857289, 354.7448905683720568, -6.410867750099231266 ) ) ;
#6608=CARTESIAN_POINT ( 'NONE',  ( -11.93348319268873503, 478.8698905683720568, -2.051577885510841163E-15 ) ) ;
#6610=ORIENTED_EDGE ( 'NONE', *, *, #11334, .T. ) ;
#6611=CARTESIAN_POINT ( 'NONE',  ( -47.16347859291445843, 487.8698905601784759, 7.653668647301805628 ) ) ;
#6612=CARTESIAN_POINT ( 'NONE',  ( -13.20868407381885135, 298.2448905683720000, 6.410867750099229490 ) ) ;
#6613=ORIENTED_EDGE ( 'NONE', *, *, #1250, .T. ) ;
#6615=ORIENTED_EDGE ( 'NONE', *, *, #10142, .T. ) ;
#6617=ADVANCED_FACE ( 'NONE', ( #3880 ), #7437, .T. ) ;
#6618=CARTESIAN_POINT ( 'NONE',  ( -42.88789093042844058, 396.3073905683720000, 9.489475012073734561 ) ) ;
#6619=CARTESIAN_POINT ( 'NONE',  ( -47.16347859291445133, 442.6198905765656377, 7.653668647301805628 ) ) ;
#6621=CARTESIAN_POINT ( 'NONE',  ( -11.93348319268872793, 418.5573905683720568, 3.332260488124728415 ) ) ;
#6622=CARTESIAN_POINT ( 'NONE',  ( -22.27502019258949773, 450.7448905683720000, -15.47720386886985544 ) ) ;
#6624=CARTESIAN_POINT ( 'NONE',  ( -8.685887942688859553, 401.9323905601783622, 3.978247347593479866 ) ) ;
#6625=CARTESIAN_POINT ( 'NONE',  ( -24.70764059509556176, 369.1823905765655240, -19.99999999999999289 ) ) ;
#6627=CARTESIAN_POINT ( 'NONE',  ( -48.68588794268852382, 266.9323905601784190, -3.978247347593583783 ) ) ;
#6629=CARTESIAN_POINT ( 'NONE',  ( -32.66413529028188378, 489.8073905765656377, -19.99999999999999289 ) ) ;
#6631=CARTESIAN_POINT ( 'NONE',  ( -38.17536295476246266, 496.9323905683720568, 14.20200298773971781 ) ) ;
#6632=FACE_OUTER_BOUND ( 'NONE', #5186, .T. ) ;
#6635=EDGE_CURVE ( 'NONE', #17719, #9040, #18287, .T. ) ;
#6636=CARTESIAN_POINT ( 'NONE',  ( -28.68588794268872277, 412.8698905683720568, -16.75240474999999307 ) ) ;
#6637=CARTESIAN_POINT ( 'NONE',  ( -48.68588794268872277, 461.9948905765656377, 0.000000000000000000 ) ) ;
#6639=CARTESIAN_POINT ( 'NONE',  ( -5.991983113971217634, 220.4588630705976584, -6.225382068641771127 ) ) ;
#6640=CARTESIAN_POINT ( 'NONE',  ( -45.43829269268871229, 363.8698905683720000, 0.000000000000000000 ) ) ;
#6642=CARTESIAN_POINT ( 'NONE',  ( -35.09675569278796559, 531.9948905683720568, -15.47720386886985544 ) ) ;
#6644=CARTESIAN_POINT ( 'NONE',  ( -13.20868407381886911, 449.7448905683720000, 6.410867750099229490 ) ) ;
#6645=CARTESIAN_POINT ( 'NONE',  ( -11.93348319268874036, 518.8698905683719431, -2.051577885510841163E-15 ) ) ;
#6647=CARTESIAN_POINT ( 'NONE',  ( -14.54375231895777532, 430.9948905601784759, 14.14213562373094568 ) ) ;
#6648=CARTESIAN_POINT ( 'NONE',  ( -14.48388495494901385, 479.8073905683720568, -9.489475012073736337 ) ) ;
#6649=EDGE_LOOP ( 'NONE', ( #2705, #12545, #14143, #5633 ) ) ;
#6650=CARTESIAN_POINT ( 'NONE',  ( -11.93348319268873858, 498.8698905683720000, -2.051577885510841163E-15 ) ) ;
#6653=CARTESIAN_POINT ( 'NONE',  ( -45.64106924314020119, 452.9323905765656377, 11.32908994701042715 ) ) ;
#6654=CARTESIAN_POINT ( 'NONE',  ( -47.16347859291444422, 361.3698905765655809, -7.653668647301793193 ) ) ;
#6662=( BOUNDED_CURVE ( )  B_SPLINE_CURVE ( 2, ( #20752, #5306, #7430, #10893, #17292, #16896, #17500, #2476, #759, #7538, #15680, #2585, #20641, #11907, #7324, #13952, #20540 ),
 .UNSPECIFIED., .F., .T. ) 
 B_SPLINE_CURVE_WITH_KNOTS ( ( 3, 2, 2, 2, 2, 2, 2, 2, 3 ),
 ( 0.7031250000000002220, 0.7050781250000002220, 0.7070312500000002220, 0.7089843750000002220, 0.7109375000000002220, 0.7128906250000002220, 0.7148437500000002220, 0.7167968750000002220, 0.7187500000000002220 ),
 .UNSPECIFIED. ) 
 CURVE ( )  GEOMETRIC_REPRESENTATION_ITEM ( )  RATIONAL_B_SPLINE_CURVE ( ( 0.9999999999999977796, 0.9807852804032326510, 1.000000000000000000, 0.9807852804032304306, 1.000000000000000000, 0.9807852804032304306, 1.000000000000000000, 0.9807852804032304306, 1.000000000000000000, 0.9807852804032304306, 1.000000000000000000, 0.9807852804032304306, 1.000000000000000000, 0.9807852804032304306, 1.000000000000000000, 0.9807852804032282101, 1.000000000000002220 ) ) 
 REPRESENTATION_ITEM ( '' )  );
#6663=CARTESIAN_POINT ( 'NONE',  ( -38.17536295476244845, 293.8073905683720568, -14.20200298773971426 ) ) ;
#6665=CARTESIAN_POINT ( 'NONE',  ( -11.73070664223723369, 233.1823905601784759, -11.32908994701042538 ) ) ;
#6666=CARTESIAN_POINT ( 'NONE',  ( -32.66413529028186247, 275.0573905601784759, -19.99999999999999289 ) ) ;
#6667=CARTESIAN_POINT ( 'NONE',  ( -11.73070664223725323, 416.0573905765656377, 11.32908994701042005 ) ) ;
#6668=CARTESIAN_POINT ( 'NONE',  ( -25.35362745456397349, 298.1823905683720000, 16.75240474999998952 ) ) ;
#6670=CARTESIAN_POINT ( 'NONE',  ( -42.88789093042844769, 504.4323905683720568, -9.489475012073734561 ) ) ;
#6674=CARTESIAN_POINT ( 'NONE',  ( -42.88789093042844769, 474.4323905683721136, -9.489475012073736337 ) ) ;
#6676=CARTESIAN_POINT ( 'NONE',  ( -44.16309181155856578, 273.2448905683720568, -6.410867750099231266 ) ) ;
#6678=DIRECTION ( 'NONE',  ( -1.000000000000000000, 0.000000000000000000, 0.000000000000000000 ) ) ;
#6679=CARTESIAN_POINT ( 'NONE',  ( -25.35362745456396638, 258.1823905683720000, 16.75240474999998952 ) ) ;
#6681=CARTESIAN_POINT ( 'NONE',  ( -47.16347859291443001, 252.6198905765656377, 7.653668647301805628 ) ) ;
#6683=CARTESIAN_POINT ( 'NONE',  ( -47.16347859291443001, 237.8698905601784759, 7.653668647301805628 ) ) ;
#6685=CARTESIAN_POINT ( 'NONE',  ( -42.88789093042842637, 272.9323905683720568, -9.489475012073736337 ) ) ;
#6688=CARTESIAN_POINT ( 'NONE',  ( -35.09675569278794427, 363.4948905683720568, -15.47720386886985544 ) ) ;
#6689=CARTESIAN_POINT ( 'NONE',  ( -42.82802356641967378, 505.9948905601785327, -14.14213562373094746 ) ) ;
#6691=EDGE_CURVE ( 'NONE', #19361, #18296, #16916, .T. ) ;
#6692=CARTESIAN_POINT ( 'NONE',  ( -11.93348319268872970, 428.5573905683720568, 3.332260488124728415 ) ) ;
#6693=CARTESIAN_POINT ( 'NONE',  ( -17.35679799567830628, 510.6823905601784759, 16.95518130045146421 ) ) ;
#6694=VERTEX_POINT ( 'NONE', #4732 ) ;
#6695=CARTESIAN_POINT ( 'NONE',  ( -17.35679799567829917, 420.6823905601784190, 16.95518130045146421 ) ) ;
#6696=EDGE_LOOP ( 'NONE', ( #5586, #1291, #4710, #19263 ) ) ;
#6700=CARTESIAN_POINT ( 'NONE',  ( -8.685887942688715668, 312.5573905601784190, -3.978247347593165895 ) ) ;
#6704=CARTESIAN_POINT ( 'NONE',  ( -28.68588794268871212, 342.8698905683720000, -16.75240474999999307 ) ) ;
#6706=CARTESIAN_POINT ( 'NONE',  ( -42.82802356641967378, 480.7448905765655809, -14.14213562373094746 ) ) ;
#6707=CARTESIAN_POINT ( 'NONE',  ( -35.09675569278794427, 361.9948905683720568, -15.47720386886985544 ) ) ;
#6709=CARTESIAN_POINT ( 'NONE',  ( -16.84014894278199037, 377.6198905683720568, 11.84573899990672530 ) ) ;
#6711=CARTESIAN_POINT ( 'NONE',  ( -42.82802356641965247, 310.7448905765656377, -14.14213562373094746 ) ) ;
#6712=FACE_OUTER_BOUND ( 'NONE', #15476, .T. ) ;
#6713=CARTESIAN_POINT ( 'NONE',  ( -35.09675569278793006, 261.9948905683720000, -15.47720386886985544 ) ) ;
#6714=CARTESIAN_POINT ( 'NONE',  ( -8.685887942688712116, 272.2448905601784759, -2.449293598294705724E-15 ) ) ;
#6715=CARTESIAN_POINT ( 'NONE',  ( -11.93348319268872970, 430.3698905683720568, -2.051577885510841163E-15 ) ) ;
#6716=CARTESIAN_POINT ( 'NONE',  ( -21.03221929538691271, 284.1198905601784759, -18.47759065022572855 ) ) ;
#6717=CARTESIAN_POINT ( 'NONE',  ( -48.68588794268872277, 497.2448905601785327, 0.000000000000000000 ) ) ;
#6721=CARTESIAN_POINT ( 'NONE',  ( -11.93348319268871904, 340.3698905683720000, -2.051577885510841163E-15 ) ) ;
#6722=CARTESIAN_POINT ( 'NONE',  ( -35.09675569278795848, 491.9948905683720568, -15.47720386886985544 ) ) ;
#6724=CARTESIAN_POINT ( 'NONE',  ( -11.73070664223726212, 491.3073905601784190, 11.32908994701042005 ) ) ;
#6725=CARTESIAN_POINT ( 'NONE',  ( -25.35362745456397349, 306.6823905683720000, 16.75240474999998952 ) ) ;
#6730=CARTESIAN_POINT ( 'NONE',  ( -40.53162694259544452, 394.1198905683720000, -11.84573899990672707 ) ) ;
#6731=CARTESIAN_POINT ( 'NONE',  ( -10.20829729246299955, 481.6198905601785327, 7.653668647301790529 ) ) ;
#6733=CARTESIAN_POINT ( 'NONE',  ( -22.27502019258948351, 426.9948905683720568, 15.47720386886985189 ) ) ;
#6734=CARTESIAN_POINT ( 'NONE',  ( -22.27502019258947286, 252.2448905683720284, -15.47720386886985544 ) ) ;
#6735=CARTESIAN_POINT ( 'NONE',  ( -14.48388495494900674, 437.9323905683720000, 9.489475012073731008 ) ) ;
#6737=CARTESIAN_POINT ( 'NONE',  ( -42.82802356641965957, 360.7448905765656377, -14.14213562373094746 ) ) ;
#6739=CARTESIAN_POINT ( 'NONE',  ( -10.20829729246298889, 387.6198905765655809, -7.653668647301794969 ) ) ;
#6742=CARTESIAN_POINT ( 'NONE',  ( -22.27502019258950128, 502.2448905683720568, -15.47720386886985544 ) ) ;
#6744=CARTESIAN_POINT ( 'NONE',  ( -45.64106924314019409, 466.3073905601785327, -11.32908994701042538 ) ) ;
#6746=CARTESIAN_POINT ( 'NONE',  ( -22.27502019258948351, 408.4948905683720000, 15.47720386886985189 ) ) ;
#6747=CARTESIAN_POINT ( 'NONE',  ( -14.54375231895778420, 468.2448905765656377, -14.14213562373094746 ) ) ;
#6748=CARTESIAN_POINT ( 'NONE',  ( -25.35362745456397349, 222.5573905683720568, -16.75240474999999307 ) ) ;
#6749=CARTESIAN_POINT ( 'NONE',  ( -19.19641293061498644, 370.4323905683720000, -14.20200298773971603 ) ) ;
#6751=CARTESIAN_POINT ( 'NONE',  ( -14.48388495494901740, 517.9323905683720568, 9.489475012073732785 ) ) ;
#6753=CARTESIAN_POINT ( 'NONE',  ( -40.53162694259544452, 446.6198905683720568, 11.84573899990672885 ) ) ;
#6754=CARTESIAN_POINT ( 'NONE',  ( -16.84014894278200458, 517.6198905683719431, 11.84573899990672530 ) ) ;
#6756=CARTESIAN_POINT ( 'NONE',  ( -24.70764059509557953, 529.1823905765656946, -19.99999999999999289 ) ) ;
#6757=CARTESIAN_POINT ( 'NONE',  ( -45.43829269268871940, 494.1823905683720000, 3.332260488124734632 ) ) ;
#6759=CARTESIAN_POINT ( 'NONE',  ( -25.35362745456399836, 496.6823905683721136, 16.75240474999998952 ) ) ;
#6760=CARTESIAN_POINT ( 'NONE',  ( -10.20829729246300133, 491.6198905601784759, 7.653668647301790529 ) ) ;
#6762=CARTESIAN_POINT ( 'NONE',  ( -32.66413529028188378, 414.1823905765656946, 19.99999999999999289 ) ) ;
#6763=CARTESIAN_POINT ( 'NONE',  ( -45.64106924314017988, 361.0573905765656377, -11.32908994701042538 ) ) ;
#6768=CARTESIAN_POINT ( 'NONE',  ( -40.01497788969914637, 493.5573905765655809, 16.95518130045146776 ) ) ;
#6769=CARTESIAN_POINT ( 'NONE',  ( -16.84014894278198327, 291.6198905683720000, -11.84573899990672707 ) ) ;
#6771=CARTESIAN_POINT ( 'NONE',  ( -45.64106924314017277, 268.1823905601785327, 11.32908994701042715 ) ) ;
#6773=CARTESIAN_POINT ( 'NONE',  ( -42.88789093042842637, 296.3073905683720000, 9.489475012073736337 ) ) ;
#6775=CARTESIAN_POINT ( 'NONE',  ( -48.68588794268872988, 537.2448905601785327, 0.000000000000000000 ) ) ;
#6776=CARTESIAN_POINT ( 'NONE',  ( -14.48388495494901385, 499.4323905683720000, 9.489475012073731008 ) ) ;
#6778=CARTESIAN_POINT ( 'NONE',  ( -21.03221929538691626, 314.1198905601784759, -18.47759065022572855 ) ) ;
#6780=CARTESIAN_POINT ( 'NONE',  ( -19.19641293061499354, 468.8073905683720000, 14.20200298773971426 ) ) ;
#6782=CARTESIAN_POINT ( 'NONE',  ( -11.93348319268870839, 258.8698905683720000, -2.051577885510841163E-15 ) ) ;
#6784=FACE_OUTER_BOUND ( 'NONE', #7816, .T. ) ;
#6787=CARTESIAN_POINT ( 'NONE',  ( -22.27502019258947286, 252.2448905683720284, -15.47720386886985544 ) ) ;
#6788=CARTESIAN_POINT ( 'NONE',  ( -8.685887942688708563, 246.6823905765656377, 3.978247347593161010 ) ) ;
#6790=CARTESIAN_POINT ( 'NONE',  ( -24.70764059509554755, 234.4323905601785043, -19.99999999999999289 ) ) ;
#6791=CARTESIAN_POINT ( 'NONE',  ( -40.53162694259543031, 275.1198905683720568, 11.84573899990672885 ) ) ;
#6792=CARTESIAN_POINT ( 'NONE',  ( -11.93348319268871904, 350.3698905683720568, -2.051577885510841163E-15 ) ) ;
#6797=CARTESIAN_POINT ( 'NONE',  ( -16.84014894278199392, 417.6198905683720000, 11.84573899990672530 ) ) ;
#6798=CARTESIAN_POINT ( 'NONE',  ( -45.64106924314017988, 341.0573905765656946, -11.32908994701042538 ) ) ;
#6799=VERTEX_POINT ( 'NONE', #4528 ) ;
#6800=CARTESIAN_POINT ( 'NONE',  ( -24.70764059509556532, 404.4323905601785327, -19.99999999999999289 ) ) ;
#6804=CARTESIAN_POINT ( 'NONE',  ( -28.68588794268873698, 532.8698905683719431, -16.75240474999999307 ) ) ;
#6805=CARTESIAN_POINT ( 'NONE',  ( -11.73070664223723902, 301.3073905601784759, 11.32908994701042005 ) ) ;
#6806=CARTESIAN_POINT ( 'NONE',  ( -43.63240380007614050, 209.9813597091836641, -1.306460585600322188 ) ) ;
#6808=CARTESIAN_POINT ( 'NONE',  ( -28.68588794268871212, 322.8698905683720000, -16.75240474999999307 ) ) ;
#6810=ORIENTED_EDGE ( 'NONE', *, *, #11651, .T. ) ;
#6811=CARTESIAN_POINT ( 'NONE',  ( -16.84014894278198682, 357.6198905683720000, 11.84573899990672530 ) ) ;
#6812=CARTESIAN_POINT ( 'NONE',  ( -32.01814843081344719, 376.0573905683720000, 16.75240474999999307 ) ) ;
#6814=CARTESIAN_POINT ( 'NONE',  ( -32.66413529028186957, 309.8073905765656377, -19.99999999999999289 ) ) ;
#6816=CARTESIAN_POINT ( 'NONE',  ( -32.01814843081343298, 261.6823905683720568, -16.75240474999999307 ) ) ;
#6818=CARTESIAN_POINT ( 'NONE',  ( -38.17536295476245556, 416.9323905683720568, 14.20200298773971781 ) ) ;
#6820=CARTESIAN_POINT ( 'NONE',  ( -36.33955658999052929, 499.1198905601784759, 18.47759065022572500 ) ) ;
#6821=DIRECTION ( 'NONE',  ( -1.191790137725560488E-16, 1.000000000000000000, -0.000000000000000000 ) ) ;
#6822=CARTESIAN_POINT ( 'NONE',  ( -21.03221929538691626, 410.3698905601784759, 18.47759065022572500 ) ) ;
#6823=CARTESIAN_POINT ( 'NONE',  ( -14.48388495494899253, 319.4323905683720568, 9.489475012073732785 ) ) ;
#6824=CARTESIAN_POINT ( 'NONE',  ( -13.20868407381887621, 489.4948905683720568, -6.410867750099233042 ) ) ;
#6827=CARTESIAN_POINT ( 'NONE',  ( -11.73070664223725856, 461.3073905601784759, 11.32908994701042005 ) ) ;
#6828=CARTESIAN_POINT ( 'NONE',  ( -35.09675569278794427, 295.7448905683720568, 15.47720386886985366 ) ) ;
#6831=ORIENTED_EDGE ( 'NONE', *, *, #14518, .T. ) ;
#6833=CARTESIAN_POINT ( 'NONE',  ( -13.20868407381886378, 390.9948905683720568, -6.410867750099233042 ) ) ;
#6834=CARTESIAN_POINT ( 'NONE',  ( -11.73070664223726034, 481.3073905601785896, 11.32908994701042005 ) ) ;
#6836=CARTESIAN_POINT ( 'NONE',  ( -38.17536295476246266, 432.3073905683720000, -14.20200298773971426 ) ) ;
#6837=CARTESIAN_POINT ( 'NONE',  ( -32.01814843081343298, 257.5573905683720568, 16.75240474999999307 ) ) ;
#6838=CARTESIAN_POINT ( 'NONE',  ( -38.17536295476246266, 422.3073905683720000, -14.20200298773971426 ) ) ;
#6840=LINE ( 'NONE', #16237, #21035 ) ;
#6842=CARTESIAN_POINT ( 'NONE',  ( -8.685887942688720997, 357.3073905765656377, -3.978247347593165895 ) ) ;
#6843=CARTESIAN_POINT ( 'NONE',  ( -17.35679799567828496, 273.8073905601784759, -16.95518130045146421 ) ) ;
#6845=CARTESIAN_POINT ( 'NONE',  ( -19.19641293061497578, 327.3073905683721136, 14.20200298773971426 ) ) ;
#6847=CARTESIAN_POINT ( 'NONE',  ( -45.43829269268871940, 485.0573905683720568, -3.332260488124726194 ) ) ;
#6848=CARTESIAN_POINT ( 'NONE',  ( -8.685887942688820473, 436.6823905765655809, 3.978247347593374172 ) ) ;
#6849=CARTESIAN_POINT ( 'NONE',  ( -28.68588794268872988, 464.7448905601784759, -19.99999999999999289 ) ) ;
#6851=CARTESIAN_POINT ( 'NONE',  ( -11.93348319268872437, 390.0573905683720568, 3.332260488124728415 ) ) ;
#6852=CARTESIAN_POINT ( 'NONE',  ( -36.33955658999050087, 263.8698905765656377, 18.47759065022572500 ) ) ;
#6853=CARTESIAN_POINT ( 'NONE',  ( -40.53162694259542320, 224.1198905683720000, -11.84573899990672707 ) ) ;
#6854=CARTESIAN_POINT ( 'NONE',  ( -38.17536295476245556, 362.3073905683719431, -14.20200298773971426 ) ) ;
#6857=CARTESIAN_POINT ( 'NONE',  ( -42.88789093042845479, 514.8073905683720568, 9.489475012073736337 ) ) ;
#6859=CARTESIAN_POINT ( 'NONE',  ( -16.84014894278199748, 439.1198905683720568, 11.84573899990672530 ) ) ;
#6860=CARTESIAN_POINT ( 'NONE',  ( -40.53162694259545873, 522.6198905683720568, -11.84573899990672707 ) ) ;
#6861=ORIENTED_EDGE ( 'NONE', *, *, #6246, .F. ) ;
#6862=CARTESIAN_POINT ( 'NONE',  ( -11.73070664223725501, 431.3073905601785327, 11.32908994701042005 ) ) ;
#6863=CARTESIAN_POINT ( 'NONE',  ( -22.27502019258950128, 490.7448905683720000, -15.47720386886985544 ) ) ;
#6865=CARTESIAN_POINT ( 'NONE',  ( -35.09675569278795848, 491.9948905683720568, -15.47720386886985544 ) ) ;
#6867=CARTESIAN_POINT ( 'NONE',  ( -47.16347859291445133, 422.6198905765656377, 7.653668647301805628 ) ) ;
#6869=CARTESIAN_POINT ( 'NONE',  ( -14.54375231895776288, 330.9948905601784190, 14.14213562373094568 ) ) ;
#6870=CARTESIAN_POINT ( 'NONE',  ( -47.16347859291445133, 441.3698905765656377, -7.653668647301793193 ) ) ;
#6873=VECTOR ( 'NONE', #18625, 1000.000000000000000 ) ;
#6875=CARTESIAN_POINT ( 'NONE',  ( -42.88695301665256920, 203.8419814082757568, -4.830353110044838694 ) ) ;
#6876=CARTESIAN_POINT ( 'NONE',  ( -40.53162694259543031, 304.1198905683720000, -11.84573899990672707 ) ) ;
#6877=CARTESIAN_POINT ( 'NONE',  ( -10.20829729246297113, 232.8698905601784759, -7.653668647301794969 ) ) ;
#6878=CARTESIAN_POINT ( 'NONE',  ( -47.16347859291443712, 277.8698905601784759, 7.653668647301805628 ) ) ;
#6880=CARTESIAN_POINT ( 'NONE',  ( -45.43829269268869808, 295.6823905683720000, 3.332260488124734632 ) ) ;
#6882=CARTESIAN_POINT ( 'NONE',  ( -8.685887942688712116, 272.2448905601784759, -2.449293598294705724E-15 ) ) ;
#6883=CARTESIAN_POINT ( 'NONE',  ( -44.16309181155857999, 495.9948905683720568, 6.410867750099241924 ) ) ;
#6886=CARTESIAN_POINT ( 'NONE',  ( -25.35362745456399480, 468.1823905683721136, 16.75240474999998952 ) ) ;
#6887=EDGE_CURVE ( 'NONE', #11943, #8642, #19122, .T. ) ;
#6889=CARTESIAN_POINT ( 'NONE',  ( -32.01814843081343298, 256.0573905683720000, 16.75240474999999307 ) ) ;
#6891=CARTESIAN_POINT ( 'NONE',  ( -17.35679799567828496, 335.4323905765656377, 16.95518130045146421 ) ) ;
#6892=CARTESIAN_POINT ( 'NONE',  ( -45.43829269268869808, 245.6823905683720568, 3.332260488124734632 ) ) ;
#6893=CARTESIAN_POINT ( 'NONE',  ( -36.33955658999050087, 243.8698905765656093, 18.47759065022572500 ) ) ;
#6894=CARTESIAN_POINT ( 'NONE',  ( -47.16347859291445133, 421.3698905765656377, -7.653668647301793193 ) ) ;
#6895=CARTESIAN_POINT ( 'NONE',  ( -24.70764059509554045, 224.4323905601784759, -19.99999999999999289 ) ) ;
#6896=CARTESIAN_POINT ( 'NONE',  ( -16.84014894278197616, 257.6198905683720568, 11.84573899990672530 ) ) ;
#6897=CARTESIAN_POINT ( 'NONE',  ( -32.01814843081344719, 363.1823905683720568, -16.75240474999999307 ) ) ;
#6898=CARTESIAN_POINT ( 'NONE',  ( -11.73070664223726745, 503.1823905601785327, -11.32908994701042538 ) ) ;
#6900=CARTESIAN_POINT ( 'NONE',  ( -11.93348319268872615, 408.8698905683720568, -2.051577885510841163E-15 ) ) ;
#6904=CARTESIAN_POINT ( 'NONE',  ( -10.20829729246299067, 412.8698905601784759, -7.653668647301794969 ) ) ;
#6909=CARTESIAN_POINT ( 'NONE',  ( -45.43829269268872650, 535.0573905683720568, -3.332260488124726194 ) ) ;
#6910=CARTESIAN_POINT ( 'NONE',  ( -11.73070664223724080, 283.1823905601784759, -11.32908994701042715 ) ) ;
#6912=CARTESIAN_POINT ( 'NONE',  ( -40.53162694259543031, 326.6198905683720568, 11.84573899990672885 ) ) ;
#6913=CARTESIAN_POINT ( 'NONE',  ( -22.27502019258947641, 356.9948905683720000, 15.47720386886985189 ) ) ;
#6914=CARTESIAN_POINT ( 'NONE',  ( -11.93348319268872260, 359.1823905683720568, -3.332260488124732856 ) ) ;
#6915=EDGE_CURVE ( 'NONE', #18327, #16131, #19939, .T. ) ;
#6916=CARTESIAN_POINT ( 'NONE',  ( -32.66413529028186957, 294.1823905765655809, 19.99999999999999289 ) ) ;
#6918=LINE ( 'NONE', #559, #15542 ) ;
#6919=CARTESIAN_POINT ( 'NONE',  ( -22.27502019258946220, 256.9948905683720568, 15.47720386886985189 ) ) ;
#6921=CARTESIAN_POINT ( 'NONE',  ( -44.16309181155857289, 415.9948905683720000, 6.410867750099241924 ) ) ;
#6923=DIRECTION ( 'NONE',  ( 1.000000000000000000, 0.000000000000000000, 0.000000000000000000 ) ) ;
#6924=CARTESIAN_POINT ( 'NONE',  ( -14.54375231895775578, 275.7448905765656377, 14.14213562373094568 ) ) ;
#6928=CARTESIAN_POINT ( 'NONE',  ( -35.09675569278795138, 337.2448905683720568, 15.47720386886985366 ) ) ;
#6929=CARTESIAN_POINT ( 'NONE',  ( -13.20868407381887089, 458.2448905683720568, 6.410867750099229490 ) ) ;
#6931=CARTESIAN_POINT ( 'NONE',  ( -47.16347859291445843, 466.6198905601784759, -7.653668647301793193 ) ) ;
#6932=CARTESIAN_POINT ( 'NONE',  ( -38.17536295476244135, 295.4323905683720000, 14.20200298773971781 ) ) ;
#6936=CARTESIAN_POINT ( 'NONE',  ( -40.01497788969913216, 343.5573905765655240, 16.95518130045146776 ) ) ;
#6939=CARTESIAN_POINT ( 'NONE',  ( -16.84014894278199392, 381.6198905683720568, -11.84573899990672707 ) ) ;
#6942=CARTESIAN_POINT ( 'NONE',  ( -19.19641293061498999, 427.3073905683720568, 14.20200298773971426 ) ) ;
#6943=CARTESIAN_POINT ( 'NONE',  ( -13.20868407381884779, 250.9948905683720284, -6.410867750099233042 ) ) ;
#6945=CARTESIAN_POINT ( 'NONE',  ( -40.53162694259544452, 425.1198905683720000, 11.84573899990672885 ) ) ;
#6947=CARTESIAN_POINT ( 'NONE',  ( -48.68588794268887909, 397.5573905601784190, 3.978247347592742678 ) ) ;
#6948=CARTESIAN_POINT ( 'NONE',  ( -36.33955658999051508, 353.8698905765656377, 18.47759065022572500 ) ) ;
#6950=DIRECTION ( 'NONE',  ( -1.191790137725560488E-16, 1.000000000000000000, -0.000000000000000000 ) ) ;
#6951=CARTESIAN_POINT ( 'NONE',  ( -45.43829269268870519, 324.1823905683720000, 3.332260488124734632 ) ) ;
#6952=CARTESIAN_POINT ( 'NONE',  ( -48.68588794268870856, 371.9948905765655809, 0.000000000000000000 ) ) ;
#6953=CARTESIAN_POINT ( 'NONE',  ( -22.27502019258949773, 472.2448905683720568, -15.47720386886985544 ) ) ;
#6955=AXIS2_PLACEMENT_3D ( 'NONE', #2594, #9173, #11118 ) ;
#6956=CARTESIAN_POINT ( 'NONE',  ( -48.68588794268870146, 307.2448905601784759, 0.000000000000000000 ) ) ;
#6957=CARTESIAN_POINT ( 'NONE',  ( -13.20868407381886200, 389.7448905683720000, 6.410867750099229490 ) ) ;
#6958=CARTESIAN_POINT ( 'NONE',  ( -24.70764059509553690, 264.8073905765656377, 19.99999999999998934 ) ) ;
#6959=EDGE_CURVE ( 'NONE', #15181, #573, #8180, .T. ) ;
#6960=CARTESIAN_POINT ( 'NONE',  ( -24.70764059509557242, 530.0573905601785327, 19.99999999999998934 ) ) ;
#6961=CARTESIAN_POINT ( 'NONE',  ( -13.20868407381885845, 358.2448905683720000, 6.410867750099229490 ) ) ;
#6964=CARTESIAN_POINT ( 'NONE',  ( -45.43829269268873361, 523.8698905683720568, 0.000000000000000000 ) ) ;
#6966=CARTESIAN_POINT ( 'NONE',  ( -28.68588794268873698, 531.3698905683720568, -16.75240474999999307 ) ) ;
#6968=DIRECTION ( 'NONE',  ( -1.000000000000000000, 0.000000000000000000, 0.000000000000000000 ) ) ;
#6969=CARTESIAN_POINT ( 'NONE',  ( -11.93348319268873681, 488.8698905683720568, -2.051577885510841163E-15 ) ) ;
#6970=ORIENTED_EDGE ( 'NONE', *, *, #15650, .F. ) ;
#6971=CARTESIAN_POINT ( 'NONE',  ( -22.27502019258950128, 490.7448905683720000, -15.47720386886985544 ) ) ;
#6974=CARTESIAN_POINT ( 'NONE',  ( -28.68588794268871922, 424.4948905765656377, 19.99999999999999289 ) ) ;
#6975=CARTESIAN_POINT ( 'NONE',  ( -8.685887942688449215, 297.3073905765655809, -3.978247347592526850 ) ) ;
#6976=CARTESIAN_POINT ( 'NONE',  ( -36.33955658999050797, 299.1198905601785327, 18.47759065022572500 ) ) ;
#6977=CARTESIAN_POINT ( 'NONE',  ( -48.68588794268865882, 441.6823905765655809, -3.978247347593264927 ) ) ;
#6979=( BOUNDED_CURVE ( )  B_SPLINE_CURVE ( 2, ( #8546, #356, #10376, #12010, #10588, #10693, #16889, #2388, #460, #3685, #781, #5832, #12333, #18496, #2497, #17209, #16999 ),
 .UNSPECIFIED., .F., .T. ) 
 B_SPLINE_CURVE_WITH_KNOTS ( ( 3, 2, 2, 2, 2, 2, 2, 2, 3 ),
 ( 0.2031250000000001665, 0.2050781250000001665, 0.2070312500000001665, 0.2089843750000001665, 0.2109375000000001665, 0.2128906250000001943, 0.2148437500000001943, 0.2167968750000001943, 0.2187500000000001943 ),
 .UNSPECIFIED. ) 
 CURVE ( )  GEOMETRIC_REPRESENTATION_ITEM ( )  RATIONAL_B_SPLINE_CURVE ( ( 0.9999999999999983347, 0.9807852804032320959, 1.000000000000000000, 0.9807852804032304306, 1.000000000000000000, 0.9807852804032304306, 1.000000000000000000, 0.9807852804032304306, 1.000000000000000000, 0.9807852804032304306, 1.000000000000000000, 0.9807852804032304306, 1.000000000000000000, 0.9807852804032304306, 1.000000000000000000, 0.9807852804032285432, 1.000000000000001998 ) ) 
 REPRESENTATION_ITEM ( '' )  );
#6983=CARTESIAN_POINT ( 'NONE',  ( -11.93348319268871549, 300.6823905683720568, -3.332260488124732856 ) ) ;
#6985=CARTESIAN_POINT ( 'NONE',  ( -42.88789093042844058, 444.4323905683720568, -9.489475012073736337 ) ) ;
#6986=CARTESIAN_POINT ( 'NONE',  ( -48.68588794268871567, 411.9948905765656377, 0.000000000000000000 ) ) ;
#6987=CARTESIAN_POINT ( 'NONE',  ( -42.88789093042841927, 266.3073905683720000, 9.489475012073736337 ) ) ;
#6991=CARTESIAN_POINT ( 'NONE',  ( -40.53162694259545162, 494.1198905683720000, -11.84573899990672707 ) ) ;
#6993=CARTESIAN_POINT ( 'NONE',  ( -40.53162694259545162, 474.1198905683720568, -11.84573899990672707 ) ) ;
#6995=CARTESIAN_POINT ( 'NONE',  ( -16.84014894278197971, 270.1198905683720568, -11.84573899990672707 ) ) ;
#6999=CARTESIAN_POINT ( 'NONE',  ( -11.93348319268870661, 250.3698905683720000, -2.051577885510841163E-15 ) ) ;
#7000=CARTESIAN_POINT ( 'NONE',  ( -48.68588794268887199, 307.5573905601784759, 3.978247347592742678 ) ) ;
#7001=DIRECTION ( 'NONE',  ( -1.000000000000000000, 0.000000000000000000, 0.000000000000000000 ) ) ;
#7002=CARTESIAN_POINT ( 'NONE',  ( -11.93348319268871016, 258.5573905683720568, 3.332260488124728415 ) ) ;
#7003=CARTESIAN_POINT ( 'NONE',  ( -19.19641293061498288, 358.8073905683720000, 14.20200298773971426 ) ) ;
#7007=CARTESIAN_POINT ( 'NONE',  ( -45.43829269268871940, 403.8698905683720000, 0.000000000000000000 ) ) ;
#7009=CARTESIAN_POINT ( 'NONE',  ( -48.68588794268871567, 407.2448905601784759, 0.000000000000000000 ) ) ;
#7014=CARTESIAN_POINT ( 'NONE',  ( -38.17536295476247687, 533.8073905683720568, -14.20200298773971426 ) ) ;
#7015=CARTESIAN_POINT ( 'NONE',  ( -17.35679799567829207, 293.8073905601784759, -16.95518130045146421 ) ) ;
#7016=CARTESIAN_POINT ( 'NONE',  ( -45.64106924314017277, 321.0573905765656377, -11.32908994701042538 ) ) ;
#7018=CARTESIAN_POINT ( 'NONE',  ( -45.43829269268870519, 315.6823905683720000, 3.332260488124734632 ) ) ;
#7020=CARTESIAN_POINT ( 'NONE',  ( -14.48388495494899786, 349.8073905683720000, -9.489475012073736337 ) ) ;
#7022=CARTESIAN_POINT ( 'NONE',  ( -38.17536295476245556, 362.3073905683719431, -14.20200298773971426 ) ) ;
#7024=CARTESIAN_POINT ( 'NONE',  ( -24.70764059509554045, 304.8073905765656377, 19.99999999999998934 ) ) ;
#7026=CARTESIAN_POINT ( 'NONE',  ( -19.19641293061497223, 260.4323905683720568, -14.20200298773971603 ) ) ;
#7027=CARTESIAN_POINT ( 'NONE',  ( -43.15185836128295449, 202.0883771310974169, 3.971358459629988236 ) ) ;
#7028=CARTESIAN_POINT ( 'NONE',  ( -45.43829269268871940, 415.3698905683720568, 0.000000000000000000 ) ) ;
#7030=CARTESIAN_POINT ( 'NONE',  ( -40.01497788969915348, 503.5573905765656946, 16.95518130045146776 ) ) ;
#7032=CARTESIAN_POINT ( 'NONE',  ( -14.48388495494899608, 331.3073905683720000, -9.489475012073736337 ) ) ;
#7033=CARTESIAN_POINT ( 'NONE',  ( -11.93348319268873503, 469.1823905683719431, -3.332260488124732856 ) ) ;
#7035=CARTESIAN_POINT ( 'NONE',  ( -14.54375231895777887, 460.9948905601785327, 14.14213562373094568 ) ) ;
#7036=CARTESIAN_POINT ( 'NONE',  ( -38.17536295476244845, 292.3073905683720000, -14.20200298773971426 ) ) ;
#7040=CARTESIAN_POINT ( 'NONE',  ( -45.64106924314017988, 342.9323905765655240, 11.32908994701042538 ) ) ;
#7041=VERTEX_POINT ( 'NONE', #14117 ) ;
#7043=CARTESIAN_POINT ( 'NONE',  ( -21.03221929538690560, 340.3698905601784759, 18.47759065022572500 ) ) ;
#7044=CARTESIAN_POINT ( 'NONE',  ( -40.53162694259543031, 305.1198905683720000, 11.84573899990672885 ) ) ;
#7045=CARTESIAN_POINT ( 'NONE',  ( -38.17536295476245556, 383.8073905683720568, -14.20200298773971426 ) ) ;
#7046=CARTESIAN_POINT ( 'NONE',  ( -14.54375231895775045, 230.9948905601784759, 14.14213562373094568 ) ) ;
#7047=CARTESIAN_POINT ( 'NONE',  ( -8.685887942688905738, 386.6823905765655240, 3.978247347593586447 ) ) ;
#7048=CARTESIAN_POINT ( 'NONE',  ( -45.43829269268871940, 423.8698905683720568, 0.000000000000000000 ) ) ;
#7049=CARTESIAN_POINT ( 'NONE',  ( -45.43829269268869098, 255.0573905683720000, -3.332260488124726194 ) ) ;
#7050=CARTESIAN_POINT ( 'NONE',  ( -19.19641293061498644, 417.3073905683720568, 14.20200298773971426 ) ) ;
#7053=CARTESIAN_POINT ( 'NONE',  ( -32.66413529028187668, 369.8073905765655240, -19.99999999999999289 ) ) ;
#7054=CARTESIAN_POINT ( 'NONE',  ( -28.68588794268870501, 274.7448905601784759, -19.99999999999999289 ) ) ;
#7055=CARTESIAN_POINT ( 'NONE',  ( -11.93348319268871727, 329.1823905683720568, -3.332260488124732856 ) ) ;
#7056=CARTESIAN_POINT ( 'NONE',  ( -22.27502019258949062, 468.4948905683720000, 15.47720386886985189 ) ) ;
#7059=CARTESIAN_POINT ( 'NONE',  ( -47.16347859291443712, 306.6198905601784759, -7.653668647301793193 ) ) ;
#7060=CARTESIAN_POINT ( 'NONE',  ( -35.09675569278794427, 383.4948905683720000, -15.47720386886985544 ) ) ;
#7062=CARTESIAN_POINT ( 'NONE',  ( -45.64106924314020119, 536.3073905601785327, -11.32908994701042715 ) ) ;
#7063=CARTESIAN_POINT ( 'NONE',  ( -40.53162694259543741, 345.1198905683720568, 11.84573899990672885 ) ) ;
#7065=CARTESIAN_POINT ( 'NONE',  ( -16.84014894278201169, 530.1198905683720568, -11.84573899990672707 ) ) ;
#7067=CARTESIAN_POINT ( 'NONE',  ( -14.54375231895776466, 350.9948905601784759, 14.14213562373094568 ) ) ;
#7068=CARTESIAN_POINT ( 'NONE',  ( -22.27502019258949773, 526.9948905683720568, 15.47720386886985189 ) ) ;
#7070=CARTESIAN_POINT ( 'NONE',  ( -47.16347859291446554, 531.3698905765655809, -7.653668647301793193 ) ) ;
#7071=CARTESIAN_POINT ( 'NONE',  ( -13.20868407381887444, 488.2448905683720000, 6.410867750099229490 ) ) ;
#7072=ORIENTED_EDGE ( 'NONE', *, *, #2140, .T. ) ;
#7073=CARTESIAN_POINT ( 'NONE',  ( -35.09675569278796559, 485.7448905683720568, 15.47720386886985366 ) ) ;
#7074=CARTESIAN_POINT ( 'NONE',  ( -21.03221929538693047, 428.8698905765655809, -18.47759065022572855 ) ) ;
#7076=CARTESIAN_POINT ( 'NONE',  ( -42.82802356641965247, 298.4948905601784759, 14.14213562373094923 ) ) ;
#7081=CARTESIAN_POINT ( 'NONE',  ( -40.01497788969914637, 435.6823905601784759, -16.95518130045146421 ) ) ;
#7083=CARTESIAN_POINT ( 'NONE',  ( -38.17536295476244135, 306.9323905683719431, 14.20200298773971781 ) ) ;
#7085=CARTESIAN_POINT ( 'NONE',  ( -13.20868407381887089, 450.9948905683720000, -6.410867750099233042 ) ) ;
#7086=CARTESIAN_POINT ( 'NONE',  ( -11.73070664223725501, 397.9323905765656377, -11.32908994701042538 ) ) ;
#7087=CARTESIAN_POINT ( 'NONE',  ( -16.84014894278197616, 279.1198905683720568, 11.84573899990672530 ) ) ;
#7091=CARTESIAN_POINT ( 'NONE',  ( -14.48388495494901385, 491.3073905683720000, -9.489475012073734561 ) ) ;
#7094=EDGE_CURVE ( 'NONE', #13710, #1213, #20703, .T. ) ;
#7096=CARTESIAN_POINT ( 'NONE',  ( -28.68588794268872633, 467.8698905683720000, 16.75240474999999307 ) ) ;
#7098=CARTESIAN_POINT ( 'NONE',  ( -38.17536295476244135, 252.3073905683720284, -14.20200298773971426 ) ) ;
#7100=( BOUNDED_CURVE ( )  B_SPLINE_CURVE ( 2, ( #16445, #4856, #4968, #3033, #11451, #11239, #9616, #6471, #18155, #14720, #21200, #16552, #13086, #12977, #6, #19674, #1626 ),
 .UNSPECIFIED., .F., .T. ) 
 B_SPLINE_CURVE_WITH_KNOTS ( ( 3, 2, 2, 2, 2, 2, 2, 2, 3 ),
 ( 0.8125000000000002220, 0.8144531250000002220, 0.8164062500000002220, 0.8183593750000002220, 0.8203125000000002220, 0.8222656250000002220, 0.8242187500000002220, 0.8261718750000002220, 0.8281250000000002220 ),
 .UNSPECIFIED. ) 
 CURVE ( )  GEOMETRIC_REPRESENTATION_ITEM ( )  RATIONAL_B_SPLINE_CURVE ( ( 0.9999999999999977796, 0.9807852804032326510, 1.000000000000000000, 0.9807852804032304306, 1.000000000000000000, 0.9807852804032304306, 1.000000000000000000, 0.9807852804032304306, 1.000000000000000000, 0.9807852804032304306, 1.000000000000000000, 0.9807852804032304306, 1.000000000000000000, 0.9807852804032304306, 1.000000000000000000, 0.9807852804032282101, 1.000000000000002220 ) ) 
 REPRESENTATION_ITEM ( '' )  );
#7102=CARTESIAN_POINT ( 'NONE',  ( -8.685887942688735208, 476.9948905765656377, -2.449293598294705724E-15 ) ) ;
#7104=CARTESIAN_POINT ( 'NONE',  ( -13.20868407381884779, 240.9948905683720284, -6.410867750099233042 ) ) ;
#7106=CARTESIAN_POINT ( 'NONE',  ( -32.66413529028187668, 419.8073905765655809, -19.99999999999999289 ) ) ;
#7107=CARTESIAN_POINT ( 'NONE',  ( -47.16347859291443001, 236.6198905601784475, -7.653668647301793193 ) ) ;
#7108=CARTESIAN_POINT ( 'NONE',  ( -16.84014894278197261, 237.6198905683720284, 11.84573899990672530 ) ) ;
#7109=CARTESIAN_POINT ( 'NONE',  ( -35.09675569278795138, 367.2448905683720000, 15.47720386886985366 ) ) ;
#7112=CARTESIAN_POINT ( 'NONE',  ( -19.19641293061498644, 397.3073905683720000, 14.20200298773971426 ) ) ;
#7113=CARTESIAN_POINT ( 'NONE',  ( -28.68588794268872988, 509.7448905601784759, 19.99999999999999289 ) ) ;
#7114=CARTESIAN_POINT ( 'NONE',  ( -8.685887942688726326, 411.9323905601785896, 3.978247347593161010 ) ) ;
#7116=ORIENTED_EDGE ( 'NONE', *, *, #13467, .T. ) ;
#7117=CYLINDRICAL_SURFACE ( 'NONE', #16017, 19.99999999999999645 ) ;
#7119=CARTESIAN_POINT ( 'NONE',  ( -22.27502019258949773, 528.4948905683719431, 15.47720386886985189 ) ) ;
#7120=CARTESIAN_POINT ( 'NONE',  ( -47.16347859291443712, 287.8698905601784759, 7.653668647301805628 ) ) ;
#7121=CARTESIAN_POINT ( 'NONE',  ( -43.47642916300955562, 209.4785612017895176, -2.513052019990858366 ) ) ;
#7122=CARTESIAN_POINT ( 'NONE',  ( -16.84014894278198327, 319.1198905683720568, 11.84573899990672530 ) ) ;
#7123=ORIENTED_EDGE ( 'NONE', *, *, #5957, .T. ) ;
#7124=CARTESIAN_POINT ( 'NONE',  ( -14.48388495494899608, 347.9323905683720000, 9.489475012073732785 ) ) ;
#7125=CARTESIAN_POINT ( 'NONE',  ( -11.93348319268872260, 368.8698905683720000, -2.051577885510841163E-15 ) ) ;
#7126=CARTESIAN_POINT ( 'NONE',  ( -14.54375231895776110, 278.2448905765655809, -14.14213562373094746 ) ) ;
#7127=CYLINDRICAL_SURFACE ( 'NONE', #10675, 5.000000000000001776 ) ;
#7128=CARTESIAN_POINT ( 'NONE',  ( -16.84014894278197971, 260.1198905683720568, -11.84573899990672707 ) ) ;
#7130=CARTESIAN_POINT ( 'NONE',  ( -16.84014894278199392, 409.1198905683720000, 11.84573899990672530 ) ) ;
#7132=CARTESIAN_POINT ( 'NONE',  ( -47.16347859291444422, 336.6198905601784759, -7.653668647301793193 ) ) ;
#7133=CARTESIAN_POINT ( 'NONE',  ( -32.66413529028186957, 355.0573905601785327, -19.99999999999999289 ) ) ;
#7135=CARTESIAN_POINT ( 'NONE',  ( -42.88789093042842637, 324.4323905683719431, -9.489475012073736337 ) ) ;
#7136=CARTESIAN_POINT ( 'NONE',  ( -11.93348319268873325, 458.5573905683720568, 3.332260488124728415 ) ) ;
#7137=VERTEX_POINT ( 'NONE', #7597 ) ;
#7138=CARTESIAN_POINT ( 'NONE',  ( -47.16347859291445843, 467.8698905601784759, 7.653668647301805628 ) ) ;
#7139=CARTESIAN_POINT ( 'NONE',  ( -14.48388495494899075, 289.8073905683720000, -9.489475012073736337 ) ) ;
#7140=EDGE_CURVE ( 'NONE', #11348, #10847, #2823, .T. ) ;
#7144=CARTESIAN_POINT ( 'NONE',  ( -45.64106924314018698, 338.1823905601784759, 11.32908994701042715 ) ) ;
#7145=CARTESIAN_POINT ( 'NONE',  ( -45.43829269268870519, 293.8698905683720568, 0.000000000000000000 ) ) ;
#7147=CARTESIAN_POINT ( 'NONE',  ( -45.43829269268871229, 375.3698905683720568, 0.000000000000000000 ) ) ;
#7150=CARTESIAN_POINT ( 'NONE',  ( -24.70764059509558308, 529.1823905765656946, -19.99999999999999289 ) ) ;
#7151=CARTESIAN_POINT ( 'NONE',  ( -45.43829269268871229, 414.1823905683720000, 3.332260488124734632 ) ) ;
#7152=CARTESIAN_POINT ( 'NONE',  ( -13.20868407381884779, 260.9948905683720568, -6.410867750099233042 ) ) ;
#7153=CARTESIAN_POINT ( 'NONE',  ( -14.48388495494900674, 427.9323905683720568, 9.489475012073731008 ) ) ;
#7155=CARTESIAN_POINT ( 'NONE',  ( -28.68588794268870856, 334.4948905765656377, 19.99999999999999289 ) ) ;
#7156=CARTESIAN_POINT ( 'NONE',  ( -48.68588794268873698, 573.2448905601785327, 0.000000000000000000 ) ) ;
#7157=CARTESIAN_POINT ( 'NONE',  ( -44.16309181155857289, 333.2448905683720568, -6.410867750099231266 ) ) ;
#7158=CARTESIAN_POINT ( 'NONE',  ( -11.93348319268873503, 480.3698905683720568, -2.051577885510841163E-15 ) ) ;
#7162=CARTESIAN_POINT ( 'NONE',  ( -42.88789093042843348, 386.3073905683720000, 9.489475012073736337 ) ) ;
#7164=CARTESIAN_POINT ( 'NONE',  ( -21.03221929538692692, 520.3698905601785327, 18.47759065022572500 ) ) ;
#7165=CARTESIAN_POINT ( 'NONE',  ( -44.16309181155856578, 334.4948905683720568, 6.410867750099241924 ) ) ;
#7167=VERTEX_POINT ( 'NONE', #5986 ) ;
#7168=CARTESIAN_POINT ( 'NONE',  ( -11.93348319268873858, 498.8698905683720000, -2.051577885510841163E-15 ) ) ;
#7170=CARTESIAN_POINT ( 'NONE',  ( -24.70764059509555111, 350.0573905601785327, 19.99999999999998934 ) ) ;
#7171=CARTESIAN_POINT ( 'NONE',  ( -48.68588794268871567, 427.2448905601784759, 0.000000000000000000 ) ) ;
#7173=CARTESIAN_POINT ( 'NONE',  ( -8.685887942688740537, 516.9948905765655809, -2.449293598294705724E-15 ) ) ;
#7174=CARTESIAN_POINT ( 'NONE',  ( -42.88789093042844769, 464.8073905683720568, 9.489475012073736337 ) ) ;
#7176=CARTESIAN_POINT ( 'NONE',  ( -32.01814843081345430, 491.6823905683720568, -16.75240474999999307 ) ) ;
#7177=CARTESIAN_POINT ( 'NONE',  ( -42.82802356641964536, 243.2448905765656093, 14.14213562373094923 ) ) ;
#7178=CARTESIAN_POINT ( 'NONE',  ( -48.68588794268871567, 431.6823905765655809, -3.978247347593158345 ) ) ;
#7185=CARTESIAN_POINT ( 'NONE',  ( -11.73070664223723192, 241.3073905601784759, 11.32908994701042005 ) ) ;
#7187=CARTESIAN_POINT ( 'NONE',  ( -22.27502019258947641, 272.2448905683720568, -15.47720386886985544 ) ) ;
#7189=CARTESIAN_POINT ( 'NONE',  ( -42.82802356641964536, 258.4948905601784759, 14.14213562373094923 ) ) ;
#7191=CARTESIAN_POINT ( 'NONE',  ( -11.93348319268873148, 450.6823905683721136, -3.332260488124732856 ) ) ;
#7192=CARTESIAN_POINT ( 'NONE',  ( -14.54375231895777532, 398.2448905765655809, -14.14213562373094746 ) ) ;
#7193=CARTESIAN_POINT ( 'NONE',  ( -44.16309181155856578, 274.7448905683720568, -6.410867750099231266 ) ) ;
#7196=CARTESIAN_POINT ( 'NONE',  ( -45.64106924314016567, 268.1823905601785327, 11.32908994701042538 ) ) ;
#7197=CARTESIAN_POINT ( 'NONE',  ( -16.84014894278200103, 479.1198905683720000, 11.84573899990672530 ) ) ;
#7198=ORIENTED_EDGE ( 'NONE', *, *, #3976, .F. ) ;
#7199=CARTESIAN_POINT ( 'NONE',  ( -42.82802356641966668, 410.7448905765656377, -14.14213562373094746 ) ) ;
#7200=CARTESIAN_POINT ( 'NONE',  ( -22.27502019258946220, 256.9948905683720568, 15.47720386886985189 ) ) ;
#7202=CARTESIAN_POINT ( 'NONE',  ( -8.685887942688720997, 336.9948905765656377, -2.449293598294705724E-15 ) ) ;
#7204=CARTESIAN_POINT ( 'NONE',  ( -47.16347859291445843, 482.6198905765656377, 7.653668647301805628 ) ) ;
#7205=CARTESIAN_POINT ( 'NONE',  ( -10.20829729246298889, 391.6198905601784759, 7.653668647301790529 ) ) ;
#7206=CARTESIAN_POINT ( 'NONE',  ( -38.55245932946841947, 223.9102039777118023, -13.63907185705690495 ) ) ;
#7207=CARTESIAN_POINT ( 'NONE',  ( -28.68588794268870146, 252.8698905683720000, -16.75240474999999307 ) ) ;
#7208=CARTESIAN_POINT ( 'NONE',  ( -44.16309181155858710, 525.9948905683720568, 6.410867750099241924 ) ) ;
#7209=CARTESIAN_POINT ( 'NONE',  ( -45.64106924314017988, 372.9323905765656377, 11.32908994701042538 ) ) ;
#7210=CARTESIAN_POINT ( 'NONE',  ( -25.35362745456397704, 251.0573905683720000, -16.75240474999999307 ) ) ;
#7211=CARTESIAN_POINT ( 'NONE',  ( -45.43829269268870519, 345.6823905683720568, 3.332260488124734632 ) ) ;
#7212=CARTESIAN_POINT ( 'NONE',  ( -47.16347859291443712, 317.8698905601784190, 7.653668647301805628 ) ) ;
#7214=CARTESIAN_POINT ( 'NONE',  ( -42.88789093042844058, 394.8073905683720000, 9.489475012073736337 ) ) ;
#7216=( BOUNDED_CURVE ( )  B_SPLINE_CURVE ( 2, ( #7849, #15776, #14476, #12524, #7529, #21059, #6228, #1377, #12842, #4301, #17491, #15994, #4408, #10988, #19432, #2680, #2999 ),
 .UNSPECIFIED., .F., .T. ) 
 B_SPLINE_CURVE_WITH_KNOTS ( ( 3, 2, 2, 2, 2, 2, 2, 2, 3 ),
 ( 0.5781250000000001110, 0.5800781250000001110, 0.5820312500000001110, 0.5839843750000001110, 0.5859375000000002220, 0.5878906250000002220, 0.5898437500000002220, 0.5917968750000002220, 0.5937500000000002220 ),
 .UNSPECIFIED. ) 
 CURVE ( )  GEOMETRIC_REPRESENTATION_ITEM ( )  RATIONAL_B_SPLINE_CURVE ( ( 0.9999999999999988898, 0.9807852804032315408, 1.000000000000000000, 0.9807852804032304306, 1.000000000000000000, 0.9807852804032304306, 1.000000000000000000, 0.9807852804032304306, 1.000000000000000000, 0.9807852804032304306, 1.000000000000000000, 0.9807852804032304306, 1.000000000000000000, 0.9807852804032304306, 1.000000000000000000, 0.9807852804032282101, 1.000000000000002220 ) ) 
 REPRESENTATION_ITEM ( '' )  );
#7217=CARTESIAN_POINT ( 'NONE',  ( -28.68588794268871922, 409.7448905601784759, 19.99999999999999289 ) ) ;
#7221=ORIENTED_EDGE ( 'NONE', *, *, #13941, .F. ) ;
#7223=CARTESIAN_POINT ( 'NONE',  ( -25.35362745456400901, 502.5573905683719431, -16.75240474999999307 ) ) ;
#7224=CARTESIAN_POINT ( 'NONE',  ( -24.70764059509555466, 294.4323905601784759, -19.99999999999999289 ) ) ;
#7227=CARTESIAN_POINT ( 'NONE',  ( -35.09675569278794427, 327.2448905683720000, 15.47720386886985366 ) ) ;
#7229=ORIENTED_EDGE ( 'NONE', *, *, #4299, .F. ) ;
#7230=CARTESIAN_POINT ( 'NONE',  ( -42.88789093042843348, 342.9323905683721136, -9.489475012073736337 ) ) ;
#7231=CARTESIAN_POINT ( 'NONE',  ( -11.93348319268872260, 348.5573905683720568, 3.332260488124728859 ) ) ;
#7232=CARTESIAN_POINT ( 'NONE',  ( -14.54375231895776110, 288.2448905765656377, -14.14213562373094746 ) ) ;
#7233=DIRECTION ( 'NONE',  ( -1.191790137725560488E-16, 1.000000000000000000, -0.000000000000000000 ) ) ;
#7234=CARTESIAN_POINT ( 'NONE',  ( -45.43829269268869808, 254.1823905683720000, 3.332260488124734632 ) ) ;
#7236=CARTESIAN_POINT ( 'NONE',  ( -40.53162694259544452, 414.1198905683720000, -11.84573899990672707 ) ) ;
#7238=CARTESIAN_POINT ( 'NONE',  ( -40.01497788969915348, 450.4323905765656377, -16.95518130045146421 ) ) ;
#7240=CARTESIAN_POINT ( 'NONE',  ( -40.53162694259543741, 334.1198905683720568, -11.84573899990672707 ) ) ;
#7241=CARTESIAN_POINT ( 'NONE',  ( -22.27502019258949773, 470.7448905683720568, -15.47720386886985544 ) ) ;
#7243=CARTESIAN_POINT ( 'NONE',  ( -32.66413529028189089, 465.0573905601784759, -19.99999999999999289 ) ) ;
#7244=CARTESIAN_POINT ( 'NONE',  ( -32.01814843081344009, 286.0573905683720568, 16.75240474999999307 ) ) ;
#7248=CARTESIAN_POINT ( 'NONE',  ( -13.20868407381886733, 439.7448905683720000, 6.410867750099229490 ) ) ;
#7249=ORIENTED_EDGE ( 'NONE', *, *, #20021, .F. ) ;
#7251=CARTESIAN_POINT ( 'NONE',  ( -42.82802356641965957, 345.9948905601784759, -14.14213562373094746 ) ) ;
#7252=CARTESIAN_POINT ( 'NONE',  ( -42.88789093042842637, 302.9323905683720568, -9.489475012073736337 ) ) ;
#7253=CARTESIAN_POINT ( 'NONE',  ( -40.53162694259543741, 384.1198905683720568, -11.84573899990672707 ) ) ;
#7254=VECTOR ( 'NONE', #4504, 1000.000000000000000 ) ;
#7255=CARTESIAN_POINT ( 'NONE',  ( -11.73070664223724968, 373.1823905601784759, -11.32908994701042538 ) ) ;
#7257=CARTESIAN_POINT ( 'NONE',  ( -32.66413529028189799, 519.8073905765655809, -19.99999999999999289 ) ) ;
#7258=CARTESIAN_POINT ( 'NONE',  ( -25.35362745456398414, 396.6823905683720000, 16.75240474999998952 ) ) ;
#7259=CARTESIAN_POINT ( 'NONE',  ( -32.01814843081343298, 237.5573905683720568, 16.75240474999999307 ) ) ;
#7261=CARTESIAN_POINT ( 'NONE',  ( -11.93348319268872793, 418.5573905683720568, 3.332260488124728859 ) ) ;
#7263=CARTESIAN_POINT ( 'NONE',  ( -11.73070664223724613, 336.0573905765656377, 11.32908994701042005 ) ) ;
#7265=CARTESIAN_POINT ( 'NONE',  ( -28.68588794268870856, 316.3698905683720568, 16.75240474999999307 ) ) ;
#7266=CARTESIAN_POINT ( 'NONE',  ( -42.88789093042844769, 476.3073905683720000, 9.489475012073736337 ) ) ;
#7268=DIRECTION ( 'NONE',  ( -1.000000000000000000, 0.000000000000000000, 0.000000000000000000 ) ) ;
#7271=CARTESIAN_POINT ( 'NONE',  ( -28.68588794268871567, 377.8698905683720000, 16.75240474999999307 ) ) ;
#7274=EDGE_CURVE ( 'NONE', #15642, #4181, #11171, .T. ) ;
#7275=CARTESIAN_POINT ( 'NONE',  ( -48.68588794268872988, 517.2448905601785327, 0.000000000000000000 ) ) ;
#7276=CARTESIAN_POINT ( 'NONE',  ( -42.88789093042843348, 334.8073905683720000, 9.489475012073736337 ) ) ;
#7278=CARTESIAN_POINT ( 'NONE',  ( -25.35362745456399836, 506.6823905683720568, 16.75240474999998952 ) ) ;
#7281=CARTESIAN_POINT ( 'NONE',  ( -47.16347859291444422, 381.3698905765656377, -7.653668647301793193 ) ) ;
#7284=CARTESIAN_POINT ( 'NONE',  ( -28.68588794268873698, 519.4948905765655809, -19.99999999999999289 ) ) ;
#7285=CARTESIAN_POINT ( 'NONE',  ( -45.43829269268872650, 473.8698905683720568, 0.000000000000000000 ) ) ;
#7287=CARTESIAN_POINT ( 'NONE',  ( -14.48388495494901029, 479.8073905683720568, -9.489475012073734561 ) ) ;
#7288=CARTESIAN_POINT ( 'NONE',  ( -36.33955658999050087, 249.1198905601784759, 18.47759065022572500 ) ) ;
#7289=CARTESIAN_POINT ( 'NONE',  ( -45.64106924314019409, 401.0573905765656377, -11.32908994701042715 ) ) ;
#7291=CARTESIAN_POINT ( 'NONE',  ( -32.66413529028186247, 299.4323905601785327, 19.99999999999999289 ) ) ;
#7292=CARTESIAN_POINT ( 'NONE',  ( -17.35679799567830983, 483.8073905601784190, -16.95518130045146421 ) ) ;
#7293=CARTESIAN_POINT ( 'NONE',  ( -28.68588794268872633, 484.4948905765656377, 19.99999999999999289 ) ) ;
#7295=CARTESIAN_POINT ( 'NONE',  ( -8.685887942688532704, 257.3073905765655240, -3.978247347592740013 ) ) ;
#7296=CARTESIAN_POINT ( 'NONE',  ( -21.03221929538689849, 240.3698905601784759, 18.47759065022572500 ) ) ;
#7298=CARTESIAN_POINT ( 'NONE',  ( -45.43829269268870519, 285.3698905683720568, 0.000000000000000000 ) ) ;
#7299=CARTESIAN_POINT ( 'NONE',  ( -11.73070664223723192, 251.3073905601784759, 11.32908994701042005 ) ) ;
#7300=CARTESIAN_POINT ( 'NONE',  ( -48.68588794268898567, 362.3073905765656946, 3.978247347592529071 ) ) ;
#7301=CARTESIAN_POINT ( 'NONE',  ( -40.53162694259545162, 456.6198905683720568, 11.84573899990672885 ) ) ;
#7302=CARTESIAN_POINT ( 'NONE',  ( -21.03221929538691981, 328.8698905765656377, -18.47759065022572855 ) ) ;
#7303=CARTESIAN_POINT ( 'NONE',  ( -19.19641293061497223, 268.8073905683720568, 14.20200298773971426 ) ) ;
#7306=CARTESIAN_POINT ( 'NONE',  ( -44.16309181155858710, 484.7448905683720568, -6.410867750099231266 ) ) ;
#7308=ORIENTED_EDGE ( 'NONE', *, *, #2400, .T. ) ;
#7310=CARTESIAN_POINT ( 'NONE',  ( -19.19641293061496867, 247.3073905683720284, 14.20200298773971426 ) ) ;
#7313=CARTESIAN_POINT ( 'NONE',  ( -28.68588794268872277, 454.4948905765656377, 19.99999999999999289 ) ) ;
#7316=CARTESIAN_POINT ( 'NONE',  ( -38.86787825240671168, 223.9102039777116318, -13.30301237467029019 ) ) ;
#7318=CARTESIAN_POINT ( 'NONE',  ( -19.19641293061499709, 518.8073905683720568, 14.20200298773971426 ) ) ;
#7320=CARTESIAN_POINT ( 'NONE',  ( -28.68588794268870146, 241.3698905683720568, -16.75240474999999307 ) ) ;
#7322=CARTESIAN_POINT ( 'NONE',  ( -38.17536295476244845, 336.9323905683720568, 14.20200298773971781 ) ) ;
#7323=CARTESIAN_POINT ( 'NONE',  ( -14.54375231895776110, 320.9948905601784759, 14.14213562373094568 ) ) ;
#7324=CARTESIAN_POINT ( 'NONE',  ( -47.16347859291443712, 302.6198905765656377, 7.653668647301805628 ) ) ;
#7325=CARTESIAN_POINT ( 'NONE',  ( -11.93348319268872615, 398.5573905683720568, 3.332260488124728415 ) ) ;
#7327=CARTESIAN_POINT ( 'NONE',  ( -28.68588794268871922, 384.7448905601785327, -19.99999999999999289 ) ) ;
#7329=CARTESIAN_POINT ( 'NONE',  ( -47.16347859291444422, 351.3698905765655809, -7.653668647301793193 ) ) ;
#7332=CARTESIAN_POINT ( 'NONE',  ( -22.27502019258950128, 502.2448905683720568, -15.47720386886985544 ) ) ;
#7335=CARTESIAN_POINT ( 'NONE',  ( -40.53162694259543031, 306.6198905683720000, 11.84573899990672885 ) ) ;
#7337=CARTESIAN_POINT ( 'NONE',  ( -40.53162694259543741, 342.6198905683720000, -11.84573899990672707 ) ) ;
#7338=CARTESIAN_POINT ( 'NONE',  ( -42.88789093042843348, 344.8073905683719431, 9.489475012073734561 ) ) ;
#7339=CARTESIAN_POINT ( 'NONE',  ( -17.35679799567828852, 278.5573905765656377, -16.95518130045146421 ) ) ;
#7340=CARTESIAN_POINT ( 'NONE',  ( -11.73070664223726745, 497.9323905765656377, -11.32908994701042538 ) ) ;
#7341=CARTESIAN_POINT ( 'NONE',  ( -35.09675569278793006, 241.9948905683720284, -15.47720386886985544 ) ) ;
#7344=CARTESIAN_POINT ( 'NONE',  ( -32.01814843081345430, 407.5573905683720568, 16.75240474999999307 ) ) ;
#7346=CARTESIAN_POINT ( 'NONE',  ( -48.68588794268855935, 451.6823905765656377, -3.978247347593583783 ) ) ;
#7347=( BOUNDED_CURVE ( )  B_SPLINE_CURVE ( 2, ( #19756, #5258, #16847, #9905, #1597, #18130, #2032, #10012, #10222, #8600, #1822, #6768, #13389, #13283, #11645, #15223, #4940 ),
 .UNSPECIFIED., .F., .T. ) 
 B_SPLINE_CURVE_WITH_KNOTS ( ( 3, 2, 2, 2, 2, 2, 2, 2, 3 ),
 ( 0.1093750000000002914, 0.1113281250000002637, 0.1132812500000002498, 0.1152343750000002220, 0.1171875000000001943, 0.1191406250000001804, 0.1210937500000001527, 0.1230468750000001388, 0.1250000000000001110 ),
 .UNSPECIFIED. ) 
 CURVE ( )  GEOMETRIC_REPRESENTATION_ITEM ( )  RATIONAL_B_SPLINE_CURVE ( ( 0.9999999999999971134, 0.9807852804032333172, 1.000000000000000000, 0.9807852804032304306, 1.000000000000000000, 0.9807852804032304306, 1.000000000000000000, 0.9807852804032304306, 1.000000000000000000, 0.9807852804032304306, 1.000000000000000000, 0.9807852804032304306, 1.000000000000000000, 0.9807852804032304306, 1.000000000000000000, 0.9807852804032293204, 1.000000000000001110 ) ) 
 REPRESENTATION_ITEM ( '' )  );
#7349=CARTESIAN_POINT ( 'NONE',  ( -45.43829269268871940, 453.5573905683720568, -3.332260488124726194 ) ) ;
#7351=CARTESIAN_POINT ( 'NONE',  ( -28.68588794268872633, 444.7448905601784759, -19.99999999999999289 ) ) ;
#7352=CARTESIAN_POINT ( 'NONE',  ( -22.27502019258947641, 280.7448905683720568, -15.47720386886985544 ) ) ;
#7360=EDGE_CURVE ( 'NONE', #3989, #17870, #11083, .T. ) ;
#7362=CARTESIAN_POINT ( 'NONE',  ( -19.19641293061497933, 300.4323905683721136, -14.20200298773971603 ) ) ;
#7364=CARTESIAN_POINT ( 'NONE',  ( -40.53162694259543741, 366.6198905683720000, 11.84573899990672885 ) ) ;
#7365=CARTESIAN_POINT ( 'NONE',  ( -32.66413529028186247, 295.0573905601784759, -19.99999999999999289 ) ) ;
#7366=CARTESIAN_POINT ( 'NONE',  ( -17.35679799567830983, 525.4323905765655809, 16.95518130045146421 ) ) ;
#7367=CARTESIAN_POINT ( 'NONE',  ( -45.43829269268871940, 403.8698905683720000, 0.000000000000000000 ) ) ;
#7368=CARTESIAN_POINT ( 'NONE',  ( -32.01814843081343298, 233.1823905683720284, -16.75240474999999307 ) ) ;
#7369=CARTESIAN_POINT ( 'NONE',  ( -42.88789093042844058, 402.9323905683720568, -9.489475012073734561 ) ) ;
#7371=CARTESIAN_POINT ( 'NONE',  ( -8.685887942688720997, 346.9948905765656377, -2.449293598294705724E-15 ) ) ;
#7373=CARTESIAN_POINT ( 'NONE',  ( -19.19641293061497223, 297.3073905683720568, 14.20200298773971426 ) ) ;
#7375=CARTESIAN_POINT ( 'NONE',  ( -22.27502019258948707, 458.4948905683720568, 15.47720386886985189 ) ) ;
#7378=DIRECTION ( 'NONE',  ( -1.191790137725560488E-16, 1.000000000000000000, -0.000000000000000000 ) ) ;
#7383=CARTESIAN_POINT ( 'NONE',  ( -24.70764059509558308, 534.4323905601785327, -19.99999999999999289 ) ) ;
#7384=CARTESIAN_POINT ( 'NONE',  ( -35.09675569278794427, 351.9948905683720000, -15.47720386886985544 ) ) ;
#7386=CARTESIAN_POINT ( 'NONE',  ( -19.19641293061499709, 507.3073905683720568, 14.20200298773971426 ) ) ;
#7388=CARTESIAN_POINT ( 'NONE',  ( -42.82802356641965957, 380.7448905765656377, -14.14213562373094746 ) ) ;
#7392=CARTESIAN_POINT ( 'NONE',  ( -42.88789093042844769, 454.8073905683720000, 9.489475012073736337 ) ) ;
#7393=ORIENTED_EDGE ( 'NONE', *, *, #17887, .T. ) ;
#7394=CARTESIAN_POINT ( 'NONE',  ( -44.16309181155857999, 464.4948905683720000, 6.410867750099241924 ) ) ;
#7397=CARTESIAN_POINT ( 'NONE',  ( -32.66413529028188378, 409.8073905765656377, -19.99999999999999289 ) ) ;
#7399=CARTESIAN_POINT ( 'NONE',  ( -28.68588794268874054, 573.2448905601785327, 0.000000000000000000 ) ) ;
#7402=CARTESIAN_POINT ( 'NONE',  ( -36.33955658999049376, 260.1198905765655809, -18.47759065022572855 ) ) ;
#7403=CARTESIAN_POINT ( 'NONE',  ( -8.685887942688642838, 432.5573905601784759, -3.978247347592952732 ) ) ;
#7405=CARTESIAN_POINT ( 'NONE',  ( -22.27502019258947641, 282.2448905683720568, -15.47720386886985544 ) ) ;
#7406=CARTESIAN_POINT ( 'NONE',  ( -11.73070664223723547, 253.1823905601785043, -11.32908994701042715 ) ) ;
#7408=CARTESIAN_POINT ( 'NONE',  ( -22.27502019258948707, 448.4948905683720568, 15.47720386886985189 ) ) ;
#7409=CARTESIAN_POINT ( 'NONE',  ( -44.16309181155855867, 264.7448905683720000, -6.410867750099231266 ) ) ;
#7411=DIRECTION ( 'NONE',  ( -1.191790137725560488E-16, 1.000000000000000000, -0.000000000000000000 ) ) ;
#7413=CARTESIAN_POINT ( 'NONE',  ( -25.35362745456399480, 478.1823905683720568, 16.75240474999998952 ) ) ;
#7415=ORIENTED_EDGE ( 'NONE', *, *, #11556, .F. ) ;
#7416=CARTESIAN_POINT ( 'NONE',  ( -8.685887942688742314, 526.9948905765655809, -2.449293598294705724E-15 ) ) ;
#7417=CARTESIAN_POINT ( 'NONE',  ( -25.35362745456396638, 236.6823905683720284, 16.75240474999998952 ) ) ;
#7420=CARTESIAN_POINT ( 'NONE',  ( -28.68588794268872633, 464.4948905765656377, 19.99999999999999289 ) ) ;
#7421=CARTESIAN_POINT ( 'NONE',  ( -14.54375231895776999, 390.9948905601784759, 14.14213562373094568 ) ) ;
#7423=CARTESIAN_POINT ( 'NONE',  ( -28.68588794268870146, 232.8698905683720284, -16.75240474999999307 ) ) ;
#7424=CARTESIAN_POINT ( 'NONE',  ( -13.20868407381887799, 510.9948905683721136, -6.410867750099233042 ) ) ;
#7426=CARTESIAN_POINT ( 'NONE',  ( -35.09675569278793006, 251.9948905683720568, -15.47720386886985544 ) ) ;
#7427=CARTESIAN_POINT ( 'NONE',  ( -11.93348319268872260, 340.0573905683720000, 3.332260488124728415 ) ) ;
#7430=CARTESIAN_POINT ( 'NONE',  ( -10.20829729246297823, 306.3698905765655809, 7.653668647301790529 ) ) ;
#7431=CARTESIAN_POINT ( 'NONE',  ( -25.35362745456399480, 391.0573905683720568, -16.75240474999999307 ) ) ;
#7434=CARTESIAN_POINT ( 'NONE',  ( -45.64106924314018698, 386.3073905601785327, -11.32908994701042715 ) ) ;
#7437=CYLINDRICAL_SURFACE ( 'NONE', #21190, 19.99999999999999645 ) ;
#7440=CARTESIAN_POINT ( 'NONE',  ( -40.53162694259545873, 514.1198905683720568, -11.84573899990672707 ) ) ;
#7443=CARTESIAN_POINT ( 'NONE',  ( -13.20868407381885312, 300.9948905683720568, -6.410867750099233042 ) ) ;
#7444=ORIENTED_EDGE ( 'NONE', *, *, #635, .F. ) ;
#7445=CARTESIAN_POINT ( 'NONE',  ( -40.53162694259543741, 335.1198905683720568, 11.84573899990672885 ) ) ;
#7446=CARTESIAN_POINT ( 'NONE',  ( -40.53162694259543741, 352.6198905683720000, -11.84573899990672707 ) ) ;
#7447=CARTESIAN_POINT ( 'NONE',  ( -42.82802356641965247, 293.2448905765655809, 14.14213562373094923 ) ) ;
#7448=LINE ( 'NONE', #4222, #18282 ) ;
#7449=CARTESIAN_POINT ( 'NONE',  ( -14.48388495494898365, 237.9323905683720000, 9.489475012073731008 ) ) ;
#7450=CARTESIAN_POINT ( 'NONE',  ( -42.82802356641963826, 204.8142847187655491, 5.000000000000000000 ) ) ;
#7451=CARTESIAN_POINT ( 'NONE',  ( -38.17536295476246266, 393.8073905683720000, -14.20200298773971426 ) ) ;
#7452=EDGE_CURVE ( 'NONE', #19877, #13421, #11662, .T. ) ;
#7455=LINE ( 'NONE', #6154, #3562 ) ;
#7456=CARTESIAN_POINT ( 'NONE',  ( -19.19641293061498999, 437.3073905683720000, 14.20200298773971426 ) ) ;
#7458=CARTESIAN_POINT ( 'NONE',  ( -14.54375231895777532, 440.9948905601784759, 14.14213562373094568 ) ) ;
#7462=ORIENTED_EDGE ( 'NONE', *, *, #21349, .T. ) ;
#7464=CARTESIAN_POINT ( 'NONE',  ( -40.01497788969912506, 318.8073905601784759, 16.95518130045146776 ) ) ;
#7465=CARTESIAN_POINT ( 'NONE',  ( -11.93348319268871727, 308.5573905683719431, 3.332260488124728415 ) ) ;
#7466=CARTESIAN_POINT ( 'NONE',  ( -22.27502019258947641, 368.4948905683720568, 15.47720386886985189 ) ) ;
#7469=CARTESIAN_POINT ( 'NONE',  ( -14.54375231895779130, 528.2448905765656946, -14.14213562373094746 ) ) ;
#7470=CARTESIAN_POINT ( 'NONE',  ( -32.01814843081345430, 406.0573905683720000, 16.75240474999999307 ) ) ;
#7471=CARTESIAN_POINT ( 'NONE',  ( -11.93348319268870839, 250.6823905683720852, -3.332260488124732856 ) ) ;
#7472=CARTESIAN_POINT ( 'NONE',  ( -28.68588794268872277, 411.3698905683720568, -16.75240474999999307 ) ) ;
#7473=CARTESIAN_POINT ( 'NONE',  ( -42.82802356641965957, 350.7448905765655809, -14.14213562373094746 ) ) ;
#7474=CARTESIAN_POINT ( 'NONE',  ( -24.70764059509555466, 324.4323905601784190, -19.99999999999999289 ) ) ;
#7475=CARTESIAN_POINT ( 'NONE',  ( -32.01814843081344009, 301.6823905683720568, -16.75240474999999307 ) ) ;
#7477=CARTESIAN_POINT ( 'NONE',  ( -44.16309181155857999, 465.9948905683720000, 6.410867750099241924 ) ) ;
#7481=EDGE_CURVE ( 'NONE', #7137, #14447, #20730, .T. ) ;
#7482=VECTOR ( 'NONE', #9007, 1000.000000000000000 ) ;
#7483=CARTESIAN_POINT ( 'NONE',  ( -25.35362745456399125, 362.5573905683720568, -16.75240474999999307 ) ) ;
#7484=CARTESIAN_POINT ( 'NONE',  ( -8.685887942688719221, 332.2448905601784759, -2.449293598294705724E-15 ) ) ;
#7486=CARTESIAN_POINT ( 'NONE',  ( -10.20829729246300310, 512.8698905601785327, -7.653668647301794969 ) ) ;
#7487=CARTESIAN_POINT ( 'NONE',  ( -28.68588794268871212, 341.3698905683720000, -16.75240474999999307 ) ) ;
#7490=CARTESIAN_POINT ( 'NONE',  ( -16.84014894278200458, 507.6198905683720000, 11.84573899990672530 ) ) ;
#7494=EDGE_CURVE ( 'NONE', #13587, #18118, #2131, .T. ) ;
#7495=CARTESIAN_POINT ( 'NONE',  ( -44.16309181155857999, 414.7448905683720568, -6.410867750099231266 ) ) ;
#7498=CARTESIAN_POINT ( 'NONE',  ( -22.27502019258949773, 460.7448905683720568, -15.47720386886985544 ) ) ;
#7500=CARTESIAN_POINT ( 'NONE',  ( -16.84014894278200103, 467.6198905683720000, 11.84573899990672530 ) ) ;
#7502=AXIS2_PLACEMENT_3D ( 'NONE', #7399, #2765, #12500 ) ;
#7503=CARTESIAN_POINT ( 'NONE',  ( -32.66413529028188378, 404.1823905765656946, 19.99999999999999289 ) ) ;
#7504=CARTESIAN_POINT ( 'NONE',  ( -8.685887942688742314, 573.2448905601785327, 2.449293598294706119E-15 ) ) ;
#7505=CARTESIAN_POINT ( 'NONE',  ( -14.54375231895777176, 368.2448905765656377, -14.14213562373094746 ) ) ;
#7510=CARTESIAN_POINT ( 'NONE',  ( -48.68588794268878672, 237.5573905601784475, 3.978247347592954952 ) ) ;
#7512=CARTESIAN_POINT ( 'NONE',  ( -44.16309181155855867, 275.9948905683720000, 6.410867750099241924 ) ) ;
#7513=CARTESIAN_POINT ( 'NONE',  ( -24.70764059509554755, 244.4323905601784759, -19.99999999999999289 ) ) ;
#7514=CARTESIAN_POINT ( 'NONE',  ( -24.70764059509554755, 364.8073905765656377, 19.99999999999998934 ) ) ;
#7515=CARTESIAN_POINT ( 'NONE',  ( -22.27502019258948351, 428.4948905683720568, 15.47720386886985189 ) ) ;
#7516=CARTESIAN_POINT ( 'NONE',  ( -28.68588794268871922, 399.4948905765656377, -19.99999999999999289 ) ) ;
#7517=CARTESIAN_POINT ( 'NONE',  ( -44.16309181155855157, 245.9948905683720284, 6.410867750099241924 ) ) ;
#7519=CARTESIAN_POINT ( 'NONE',  ( -8.685887942688742314, 573.2448905601785327, 2.449293598294706119E-15 ) ) ;
#7520=ORIENTED_EDGE ( 'NONE', *, *, #401, .F. ) ;
#7521=CARTESIAN_POINT ( 'NONE',  ( -42.88789093042844769, 484.4323905683720000, -9.489475012073734561 ) ) ;
#7523=LINE ( 'NONE', #4294, #1756 ) ;
#7524=CARTESIAN_POINT ( 'NONE',  ( -32.01814843081343298, 241.6823905683720568, -16.75240474999999307 ) ) ;
#7525=ORIENTED_EDGE ( 'NONE', *, *, #115, .T. ) ;
#7526=CARTESIAN_POINT ( 'NONE',  ( -25.35362745456401257, 521.0573905683719431, -16.75240474999999307 ) ) ;
#7527=DIRECTION ( 'NONE',  ( -1.000000000000000000, 0.000000000000000000, 0.000000000000000000 ) ) ;
#7528=CARTESIAN_POINT ( 'NONE',  ( -47.16347859291445843, 462.6198905765655809, 7.653668647301805628 ) ) ;
#7529=CARTESIAN_POINT ( 'NONE',  ( -14.54375231895776466, 350.9948905601784759, 14.14213562373094568 ) ) ;
#7530=CYLINDRICAL_SURFACE ( 'NONE', #2878, 19.99999999999999645 ) ;
#7531=CARTESIAN_POINT ( 'NONE',  ( -31.59713164724962198, 223.9102039777117454, -17.88048509134786812 ) ) ;
#7533=CARTESIAN_POINT ( 'NONE',  ( -22.27502019258949417, 508.4948905683720568, 15.47720386886985189 ) ) ;
#7535=CARTESIAN_POINT ( 'NONE',  ( -22.27502019258946220, 256.9948905683720568, 15.47720386886985189 ) ) ;
#7536=CARTESIAN_POINT ( 'NONE',  ( -45.43829269268870519, 335.0573905683720568, -3.332260488124726194 ) ) ;
#7537=CARTESIAN_POINT ( 'NONE',  ( -47.16347859291445843, 467.8698905601784759, 7.653668647301805628 ) ) ;
#7538=CARTESIAN_POINT ( 'NONE',  ( -32.66413529028186247, 304.1823905765655809, 19.99999999999999289 ) ) ;
#7540=CARTESIAN_POINT ( 'NONE',  ( -28.68588794268871567, 386.3698905683720568, 16.75240474999999307 ) ) ;
#7541=ADVANCED_FACE ( 'NONE', ( #2667 ), #12294, .T. ) ;
#7542=CARTESIAN_POINT ( 'NONE',  ( -8.685887942688728103, 422.2448905601784759, -2.449293598294705724E-15 ) ) ;
#7543=CARTESIAN_POINT ( 'NONE',  ( -47.16347859291444422, 377.8698905601784190, 7.653668647301805628 ) ) ;
#7547=ORIENTED_EDGE ( 'NONE', *, *, #16367, .F. ) ;
#7548=ORIENTED_EDGE ( 'NONE', *, *, #20195, .T. ) ;
#7549=CARTESIAN_POINT ( 'NONE',  ( -25.35362745456399836, 498.1823905683720000, 16.75240474999998952 ) ) ;
#7550=CARTESIAN_POINT ( 'NONE',  ( -8.685887942688980345, 296.6823905765654104, 3.978247347593800054 ) ) ;
#7552=CARTESIAN_POINT ( 'NONE',  ( -22.27502019258947996, 312.2448905683720000, -15.47720386886985544 ) ) ;
#7554=CARTESIAN_POINT ( 'NONE',  ( -14.48388495494899431, 327.9323905683720568, 9.489475012073732785 ) ) ;
#7555=CARTESIAN_POINT ( 'NONE',  ( -44.16309181155856578, 344.4948905683720000, 6.410867750099241924 ) ) ;
#7556=CARTESIAN_POINT ( 'NONE',  ( -40.01497788969912506, 293.5573905765656377, 16.95518130045146776 ) ) ;
#7558=CARTESIAN_POINT ( 'NONE',  ( -42.88789093042841927, 244.8073905683720568, 9.489475012073734561 ) ) ;
#7559=CARTESIAN_POINT ( 'NONE',  ( -19.19641293061498999, 401.9323905683720000, -14.20200298773971603 ) ) ;
#7561=EDGE_CURVE ( 'NONE', #1608, #3040, #15660, .T. ) ;
#7564=CARTESIAN_POINT ( 'NONE',  ( -10.20829729246297291, 242.8698905601785043, -7.653668647301794969 ) ) ;
#7565=CARTESIAN_POINT ( 'NONE',  ( -42.88789093042844769, 452.9323905683720568, -9.489475012073736337 ) ) ;
#7567=CARTESIAN_POINT ( 'NONE',  ( -48.68588794268871567, 437.2448905601785327, 0.000000000000000000 ) ) ;
#7573=CARTESIAN_POINT ( 'NONE',  ( -48.68588794268870146, 327.2448905601785327, 0.000000000000000000 ) ) ;
#7575=EDGE_CURVE ( 'NONE', #15608, #19602, #846, .T. ) ;
#7576=CARTESIAN_POINT ( 'NONE',  ( -11.93348319268872260, 370.6823905683719431, -3.332260488124732856 ) ) ;
#7577=DIRECTION ( 'NONE',  ( -1.191790137725560488E-16, 1.000000000000000000, -0.000000000000000000 ) ) ;
#7578=CARTESIAN_POINT ( 'NONE',  ( -32.66413529028189799, 524.1823905765656946, 19.99999999999999289 ) ) ;
#7579=CARTESIAN_POINT ( 'NONE',  ( -13.20868407381886378, 408.2448905683720568, 6.410867750099229490 ) ) ;
#7580=CARTESIAN_POINT ( 'NONE',  ( -44.16309181155855867, 234.7448905683720000, -6.410867750099231266 ) ) ;
#7581=CARTESIAN_POINT ( 'NONE',  ( -25.35362745456398770, 406.6823905683719431, 16.75240474999998952 ) ) ;
#7582=CARTESIAN_POINT ( 'NONE',  ( -36.33955658999050797, 350.1198905765656377, -18.47759065022572855 ) ) ;
#7584=CARTESIAN_POINT ( 'NONE',  ( -32.01814843081344009, 306.0573905683720000, 16.75240474999999307 ) ) ;
#7585=CARTESIAN_POINT ( 'NONE',  ( -22.27502019258949773, 452.2448905683720000, -15.47720386886985544 ) ) ;
#7590=CARTESIAN_POINT ( 'NONE',  ( -38.17536295476244845, 376.9323905683719431, 14.20200298773971781 ) ) ;
#7591=CARTESIAN_POINT ( 'NONE',  ( -13.20868407381887799, 509.4948905683720568, -6.410867750099233042 ) ) ;
#7592=CARTESIAN_POINT ( 'NONE',  ( -14.54375231895778420, 510.9948905601784190, 14.14213562373094568 ) ) ;
#7593=CARTESIAN_POINT ( 'NONE',  ( -35.09675569278793716, 321.9948905683720568, -15.47720386886985544 ) ) ;
#7595=CARTESIAN_POINT ( 'NONE',  ( -38.17536295476246977, 502.3073905683720568, -14.20200298773971426 ) ) ;
#7597=CARTESIAN_POINT ( 'NONE',  ( -48.68588794268872277, 457.2448905601784759, 0.000000000000000000 ) ) ;
#7598=CARTESIAN_POINT ( 'NONE',  ( -13.20868407381886733, 420.9948905683720000, -6.410867750099233042 ) ) ;
#7599=CARTESIAN_POINT ( 'NONE',  ( -40.01497788969911795, 233.5573905765656093, 16.95518130045146776 ) ) ;
#7600=CARTESIAN_POINT ( 'NONE',  ( -14.54375231895778953, 518.2448905765656946, -14.14213562373094746 ) ) ;
#7601=CARTESIAN_POINT ( 'NONE',  ( -38.17536295476246977, 462.3073905683720568, -14.20200298773971426 ) ) ;
#7603=CARTESIAN_POINT ( 'NONE',  ( -14.48388495494901029, 457.9323905683720000, 9.489475012073731008 ) ) ;
#7604=( BOUNDED_CURVE ( )  B_SPLINE_CURVE ( 2, ( #12707, #4790, #16386, #8132, #12813, #17569, #2868, #21348, #17781, #9451, #6092, #3073, #16068, #11386, #19509, #20925, #6516 ),
 .UNSPECIFIED., .F., .T. ) 
 B_SPLINE_CURVE_WITH_KNOTS ( ( 3, 2, 2, 2, 2, 2, 2, 2, 3 ),
 ( 0.3750000000000001665, 0.3769531250000001665, 0.3789062500000001665, 0.3808593750000001665, 0.3828125000000001665, 0.3847656250000001665, 0.3867187500000001665, 0.3886718750000001665, 0.3906250000000001665 ),
 .UNSPECIFIED. ) 
 CURVE ( )  GEOMETRIC_REPRESENTATION_ITEM ( )  RATIONAL_B_SPLINE_CURVE ( ( 0.9999999999999983347, 0.9807852804032320959, 1.000000000000000000, 0.9807852804032304306, 1.000000000000000000, 0.9807852804032304306, 1.000000000000000000, 0.9807852804032304306, 1.000000000000000000, 0.9807852804032304306, 1.000000000000000000, 0.9807852804032304306, 1.000000000000000000, 0.9807852804032304306, 1.000000000000000000, 0.9807852804032287652, 1.000000000000001554 ) ) 
 REPRESENTATION_ITEM ( '' )  );
#7607=CARTESIAN_POINT ( 'NONE',  ( -32.66413529028188378, 394.1823905765655809, 19.99999999999999289 ) ) ;
#7608=CARTESIAN_POINT ( 'NONE',  ( -28.68588794268870501, 279.4948905765656377, -19.99999999999999289 ) ) ;
#7611=CARTESIAN_POINT ( 'NONE',  ( -14.54375231895778242, 485.7448905765656377, 14.14213562373094568 ) ) ;
#7615=CARTESIAN_POINT ( 'NONE',  ( -36.33955658999049376, 255.3698905601785043, -18.47759065022572855 ) ) ;
#7616=CARTESIAN_POINT ( 'NONE',  ( -43.03936164446626833, 223.9102039777117454, 11.81008090239473773 ) ) ;
#7617=ADVANCED_FACE ( 'NONE', ( #10765, #19211 ), #1061, .F. ) ;
#7619=CARTESIAN_POINT ( 'NONE',  ( -32.66413529028186247, 255.0573905601785043, -19.99999999999999289 ) ) ;
#7620=CARTESIAN_POINT ( 'NONE',  ( -17.35679799567828852, 365.4323905765656377, 16.95518130045146421 ) ) ;
#7621=CARTESIAN_POINT ( 'NONE',  ( -42.88789093042844058, 434.4323905683720568, -9.489475012073736337 ) ) ;
#7622=CARTESIAN_POINT ( 'NONE',  ( -11.73070664223723547, 266.0573905765656377, 11.32908994701042005 ) ) ;
#7624=CARTESIAN_POINT ( 'NONE',  ( -45.43829269268869808, 245.3698905683720568, 0.000000000000000000 ) ) ;
#7627=CARTESIAN_POINT ( 'NONE',  ( -28.68588794268869790, 223.9102039777116602, 0.000000000000000000 ) ) ;
#7628=ORIENTED_EDGE ( 'NONE', *, *, #9300, .T. ) ;
#7629=CARTESIAN_POINT ( 'NONE',  ( -42.88789093042844769, 464.4323905683720000, -9.489475012073734561 ) ) ;
#7630=EDGE_CURVE ( 'NONE', #15821, #15878, #20511, .T. ) ;
#7634=CARTESIAN_POINT ( 'NONE',  ( -48.68588794268870856, 367.2448905601784759, 0.000000000000000000 ) ) ;
#7635=CARTESIAN_POINT ( 'NONE',  ( -22.27502019258946220, 246.9948905683720284, 15.47720386886985189 ) ) ;
#7637=CARTESIAN_POINT ( 'NONE',  ( -14.48388495494901562, 517.9323905683720568, 9.489475012073731008 ) ) ;
#7640=CARTESIAN_POINT ( 'NONE',  ( -24.70764059509556532, 464.8073905765656377, 19.99999999999998934 ) ) ;
#7642=CARTESIAN_POINT ( 'NONE',  ( -45.64106924314017277, 282.9323905765656377, 11.32908994701042538 ) ) ;
#7645=CARTESIAN_POINT ( 'NONE',  ( -28.68588794268869435, 227.8698905683720284, 16.75240474999999307 ) ) ;
#7646=CARTESIAN_POINT ( 'NONE',  ( -8.685887942688735208, 466.9948905765656377, -2.449293598294705724E-15 ) ) ;
#7647=CARTESIAN_POINT ( 'NONE',  ( -35.09675569278793006, 221.9948905683720284, -15.47720386886985544 ) ) ;
#7648=CARTESIAN_POINT ( 'NONE',  ( -38.17536295476245556, 343.8073905683720000, -14.20200298773971426 ) ) ;
#7650=CARTESIAN_POINT ( 'NONE',  ( -36.33955658999050797, 319.1198905601784759, 18.47759065022572500 ) ) ;
#7652=CARTESIAN_POINT ( 'NONE',  ( -38.17536295476244135, 316.9323905683719431, 14.20200298773971781 ) ) ;
#7653=CARTESIAN_POINT ( 'NONE',  ( -32.01814843081344719, 376.0573905683720000, 16.75240474999999307 ) ) ;
#7655=CARTESIAN_POINT ( 'NONE',  ( -14.54375231895777354, 393.4948905601784190, -14.14213562373094746 ) ) ;
#7657=EDGE_LOOP ( 'NONE', ( #5080, #13093, #3961, #3253 ) ) ;
#7659=CARTESIAN_POINT ( 'NONE',  ( -45.43829269268871940, 505.0573905683721136, -3.332260488124726194 ) ) ;
#7662=CARTESIAN_POINT ( 'NONE',  ( -38.17536295476244845, 303.8073905683720000, -14.20200298773971426 ) ) ;
#7664=CARTESIAN_POINT ( 'NONE',  ( -42.88789093042843348, 332.9323905683720568, -9.489475012073736337 ) ) ;
#7666=CARTESIAN_POINT ( 'NONE',  ( -17.35679799567828141, 265.4323905765656377, 16.95518130045146421 ) ) ;
#7667=CARTESIAN_POINT ( 'NONE',  ( -8.685887942688742314, 573.2448905601785327, 2.449293598294706119E-15 ) ) ;
#7669=CARTESIAN_POINT ( 'NONE',  ( -40.53162694259542320, 242.6198905683720284, -11.84573899990672707 ) ) ;
#7670=CYLINDRICAL_SURFACE ( 'NONE', #19821, 19.99999999999999645 ) ;
#7671=( BOUNDED_CURVE ( )  B_SPLINE_CURVE ( 2, ( #19014, #18901, #20861, #4198, #10673, #9274, #10784, #19128, #974, #17606, #2369, #5812, #12420, #5704, #7537, #20750, #14276 ),
 .UNSPECIFIED., .F., .T. ) 
 B_SPLINE_CURVE_WITH_KNOTS ( ( 3, 2, 2, 2, 2, 2, 2, 2, 3 ),
 ( 0.2031250000000001665, 0.2050781250000001665, 0.2070312500000001665, 0.2089843750000001665, 0.2109375000000001665, 0.2128906250000001943, 0.2148437500000001943, 0.2167968750000001943, 0.2187500000000001943 ),
 .UNSPECIFIED. ) 
 CURVE ( )  GEOMETRIC_REPRESENTATION_ITEM ( )  RATIONAL_B_SPLINE_CURVE ( ( 0.9999999999999983347, 0.9807852804032320959, 1.000000000000000000, 0.9807852804032304306, 1.000000000000000000, 0.9807852804032304306, 1.000000000000000000, 0.9807852804032304306, 1.000000000000000000, 0.9807852804032304306, 1.000000000000000000, 0.9807852804032304306, 1.000000000000000000, 0.9807852804032304306, 1.000000000000000000, 0.9807852804032285432, 1.000000000000001998 ) ) 
 REPRESENTATION_ITEM ( '' )  );
#7672=CARTESIAN_POINT ( 'NONE',  ( -35.09675569278795848, 407.2448905683720568, 15.47720386886985366 ) ) ;
#7676=CARTESIAN_POINT ( 'NONE',  ( -36.33955658999049376, 245.3698905601785043, -18.47759065022572855 ) ) ;
#7677=CARTESIAN_POINT ( 'NONE',  ( -28.68588794268872277, 436.3698905683720000, 16.75240474999999307 ) ) ;
#7679=CARTESIAN_POINT ( 'NONE',  ( -8.685887942688731655, 452.5573905601784759, -3.978247347593165895 ) ) ;
#7680=ORIENTED_EDGE ( 'NONE', *, *, #3878, .T. ) ;
#7681=ORIENTED_EDGE ( 'NONE', *, *, #13784, .F. ) ;
#7682=ORIENTED_EDGE ( 'NONE', *, *, #8792, .F. ) ;
#7684=CARTESIAN_POINT ( 'NONE',  ( -8.685887942688719221, 332.2448905601784759, -2.449293598294705724E-15 ) ) ;
#7686=CARTESIAN_POINT ( 'NONE',  ( -14.48388495494899963, 369.4323905683719431, 9.489475012073731008 ) ) ;
#7687=DIRECTION ( 'NONE',  ( -1.000000000000000000, 0.000000000000000000, 0.000000000000000000 ) ) ;
#7688=CARTESIAN_POINT ( 'NONE',  ( -10.20829729246300310, 496.3698905765655809, 7.653668647301790529 ) ) ;
#7689=CARTESIAN_POINT ( 'NONE',  ( -25.35362745456398414, 386.6823905683720568, 16.75240474999998952 ) ) ;
#7690=CARTESIAN_POINT ( 'NONE',  ( -44.16309181155855157, 235.9948905683720284, 6.410867750099241924 ) ) ;
#7691=AXIS2_PLACEMENT_3D ( 'NONE', #17213, #18399, #10487 ) ;
#7692=CARTESIAN_POINT ( 'NONE',  ( -35.09675569278795138, 411.9948905683720000, -15.47720386886985544 ) ) ;
#7693=CARTESIAN_POINT ( 'NONE',  ( -45.64106924314017988, 322.9323905765655809, 11.32908994701042715 ) ) ;
#7695=CARTESIAN_POINT ( 'NONE',  ( -25.35362745456398414, 301.0573905683720568, -16.75240474999999307 ) ) ;
#7696=CARTESIAN_POINT ( 'NONE',  ( -11.93348319268873148, 450.3698905683720000, -2.051577885510841163E-15 ) ) ;
#7697=CARTESIAN_POINT ( 'NONE',  ( -11.73070664223725856, 461.3073905601784759, 11.32908994701042005 ) ) ;
#7698=CARTESIAN_POINT ( 'NONE',  ( -11.73070664223724791, 371.3073905601784759, 11.32908994701042005 ) ) ;
#7699=CARTESIAN_POINT ( 'NONE',  ( -28.68588794268874054, 573.2448905601785327, 0.000000000000000000 ) ) ;
#7702=CARTESIAN_POINT ( 'NONE',  ( -22.27502019258948707, 362.2448905683720000, -15.47720386886985544 ) ) ;
#7703=CARTESIAN_POINT ( 'NONE',  ( -25.35362745456400901, 511.0573905683720568, -16.75240474999999307 ) ) ;
#7705=CARTESIAN_POINT ( 'NONE',  ( -45.64106924314020119, 516.3073905601784190, -11.32908994701042715 ) ) ;
#7706=CARTESIAN_POINT ( 'NONE',  ( -28.68588794268871212, 331.3698905683720000, -16.75240474999999307 ) ) ;
#7712=CARTESIAN_POINT ( 'NONE',  ( -40.53162694259544452, 414.1198905683720000, -11.84573899990672707 ) ) ;
#7713=CARTESIAN_POINT ( 'NONE',  ( -38.17536295476246977, 452.3073905683720568, -14.20200298773971426 ) ) ;
#7715=CARTESIAN_POINT ( 'NONE',  ( -32.01814843081345430, 461.6823905683720568, -16.75240474999999307 ) ) ;
#7718=CARTESIAN_POINT ( 'NONE',  ( -42.82802356641966668, 410.7448905765656377, -14.14213562373094746 ) ) ;
#7721=CYLINDRICAL_SURFACE ( 'NONE', #5638, 19.99999999999999645 ) ;
#7725=CARTESIAN_POINT ( 'NONE',  ( -8.685887942688710339, 256.9948905765655809, -2.449293598294705724E-15 ) ) ;
#7727=CARTESIAN_POINT ( 'NONE',  ( -21.03221929538689849, 240.3698905601784759, 18.47759065022572500 ) ) ;
#7729=CARTESIAN_POINT ( 'NONE',  ( -11.93348319268872793, 420.3698905683720568, -2.051577885510841163E-15 ) ) ;
#7730=CARTESIAN_POINT ( 'NONE',  ( -36.33955658999050797, 385.3698905601785327, -18.47759065022572855 ) ) ;
#7731=CARTESIAN_POINT ( 'NONE',  ( -22.27502019258946220, 248.4948905683720284, 15.47720386886985189 ) ) ;
#7733=EDGE_LOOP ( 'NONE', ( #17900, #17198, #20759, #7762 ) ) ;
#7735=CARTESIAN_POINT ( 'NONE',  ( -28.68588794268872277, 457.8698905683720000, 16.75240474999999307 ) ) ;
#7736=CARTESIAN_POINT ( 'NONE',  ( -48.68588794268869435, 231.6823905765656377, -3.978247347593158345 ) ) ;
#7739=CARTESIAN_POINT ( 'NONE',  ( -24.70764059509556887, 524.8073905765658083, 19.99999999999998934 ) ) ;
#7740=CARTESIAN_POINT ( 'NONE',  ( -25.35362745456397704, 231.0573905683720568, -16.75240474999999307 ) ) ;
#7742=CARTESIAN_POINT ( 'NONE',  ( -28.68588794268873343, 526.3698905683720568, 16.75240474999999307 ) ) ;
#7744=CARTESIAN_POINT ( 'NONE',  ( -48.68588794268872277, 471.6823905765656377, -3.978247347593158345 ) ) ;
#7747=CARTESIAN_POINT ( 'NONE',  ( -47.16347859291443001, 241.3698905765656093, -7.653668647301793193 ) ) ;
#7748=CARTESIAN_POINT ( 'NONE',  ( -35.09675569278793716, 227.2448905683720568, 15.47720386886985366 ) ) ;
#7750=CARTESIAN_POINT ( 'NONE',  ( -11.93348319268870661, 228.5573905683720568, 3.332260488124728415 ) ) ;
#7751=CARTESIAN_POINT ( 'NONE',  ( -16.84014894278198682, 321.6198905683720568, -11.84573899990672707 ) ) ;
#7753=CARTESIAN_POINT ( 'NONE',  ( -43.68588794268869435, 193.9102039777116602, 0.000000000000000000 ) ) ;
#7754=CARTESIAN_POINT ( 'NONE',  ( -40.01497788969913216, 378.8073905601785327, 16.95518130045146776 ) ) ;
#7756=CARTESIAN_POINT ( 'NONE',  ( -22.27502019258947996, 302.2448905683720000, -15.47720386886985544 ) ) ;
#7757=ADVANCED_FACE ( 'NONE', ( #11518 ), #21152, .T. ) ;
#7758=CARTESIAN_POINT ( 'NONE',  ( -11.93348319268872260, 378.8698905683720000, -2.051577885510841163E-15 ) ) ;
#7759=CARTESIAN_POINT ( 'NONE',  ( -22.27502019258950483, 522.2448905683720568, -15.47720386886985544 ) ) ;
#7760=CARTESIAN_POINT ( 'NONE',  ( -8.685887942688722774, 382.5573905601784759, -3.978247347593165895 ) ) ;
#7761=CARTESIAN_POINT ( 'NONE',  ( -45.64106924314016567, 231.0573905765656093, -11.32908994701042538 ) ) ;
#7762=ORIENTED_EDGE ( 'NONE', *, *, #662, .F. ) ;
#7764=CARTESIAN_POINT ( 'NONE',  ( -32.01814843081346140, 493.1823905683721136, -16.75240474999999307 ) ) ;
#7766=ORIENTED_EDGE ( 'NONE', *, *, #16765, .F. ) ;
#7767=ADVANCED_FACE ( 'NONE', ( #9885 ), #5022, .T. ) ;
#7768=CARTESIAN_POINT ( 'NONE',  ( -45.43829269268870519, 305.3698905683720568, 0.000000000000000000 ) ) ;
#7769=CARTESIAN_POINT ( 'NONE',  ( -25.35362745456398770, 321.0573905683720568, -16.75240474999999307 ) ) ;
#7770=CARTESIAN_POINT ( 'NONE',  ( -32.66413529028186247, 269.8073905765655809, -19.99999999999999289 ) ) ;
#7771=CARTESIAN_POINT ( 'NONE',  ( -24.70764059509557242, 474.4323905601785327, -19.99999999999999289 ) ) ;
#7773=CARTESIAN_POINT ( 'NONE',  ( -25.35362745456398414, 388.1823905683720568, 16.75240474999998952 ) ) ;
#7776=CARTESIAN_POINT ( 'NONE',  ( -28.68588794268870146, 244.7448905601785043, -19.99999999999999289 ) ) ;
#7777=CARTESIAN_POINT ( 'NONE',  ( -44.16309181155857289, 444.4948905683720568, 6.410867750099241924 ) ) ;
#7780=CARTESIAN_POINT ( 'NONE',  ( -42.82802356641967378, 455.9948905601784759, -14.14213562373094746 ) ) ;
#7783=EDGE_LOOP ( 'NONE', ( #4867, #14941, #21257, #569 ) ) ;
#7785=CARTESIAN_POINT ( 'NONE',  ( -45.64106924314017988, 326.3073905601785327, -11.32908994701042715 ) ) ;
#7786=CARTESIAN_POINT ( 'NONE',  ( -39.89451704885674843, 223.9102039777116318, -12.46781227845250584 ) ) ;
#7787=CARTESIAN_POINT ( 'NONE',  ( -14.48388495494899963, 361.3073905683720568, -9.489475012073734561 ) ) ;
#7789=CARTESIAN_POINT ( 'NONE',  ( -14.54375231895778420, 495.7448905765656377, 14.14213562373094568 ) ) ;
#7790=CARTESIAN_POINT ( 'NONE',  ( -14.48388495494900496, 389.8073905683721136, -9.489475012073736337 ) ) ;
#7791=CARTESIAN_POINT ( 'NONE',  ( -25.35362745456397349, 222.5573905683720568, -16.75240474999999307 ) ) ;
#7792=CARTESIAN_POINT ( 'NONE',  ( -16.84014894278199748, 410.1198905683720000, -11.84573899990672707 ) ) ;
#7794=CARTESIAN_POINT ( 'NONE',  ( -32.66413529028187668, 329.8073905765655809, -19.99999999999999289 ) ) ;
#7796=CARTESIAN_POINT ( 'NONE',  ( -11.93348319268871371, 299.1823905683720000, -3.332260488124732856 ) ) ;
#7797=CARTESIAN_POINT ( 'NONE',  ( -35.09675569278795848, 463.4948905683720000, -15.47720386886985544 ) ) ;
#7798=CARTESIAN_POINT ( 'NONE',  ( -47.16347859291445843, 457.8698905601785327, 7.653668647301805628 ) ) ;
#7799=CARTESIAN_POINT ( 'NONE',  ( -32.66413529028186957, 369.4323905601784190, 19.99999999999999289 ) ) ;
#7802=CARTESIAN_POINT ( 'NONE',  ( -28.68588794268871212, 367.8698905683720000, 16.75240474999999307 ) ) ;
#7803=CARTESIAN_POINT ( 'NONE',  ( -11.93348319268873858, 498.5573905683720568, 3.332260488124728415 ) ) ;
#7804=CARTESIAN_POINT ( 'NONE',  ( -8.685887942688740537, 511.9323905601785327, 3.978247347593161010 ) ) ;
#7805=CARTESIAN_POINT ( 'NONE',  ( -44.16309181155855867, 314.4948905683720000, 6.410867750099241924 ) ) ;
#7808=CARTESIAN_POINT ( 'NONE',  ( -24.70764059509557953, 524.4323905601783053, -19.99999999999999289 ) ) ;
#7813=CARTESIAN_POINT ( 'NONE',  ( -19.19641293061498999, 431.9323905683719431, -14.20200298773971603 ) ) ;
#7814=CARTESIAN_POINT ( 'NONE',  ( -24.70764059509555111, 394.8073905765655809, 19.99999999999998934 ) ) ;
#7815=CARTESIAN_POINT ( 'NONE',  ( -28.68588794268872277, 436.3698905683720000, 16.75240474999999307 ) ) ;
#7816=EDGE_LOOP ( 'NONE', ( #7444, #9473, #10207, #9619 ) ) ;
#7817=CARTESIAN_POINT ( 'NONE',  ( -40.53162694259545162, 462.6198905683720000, -11.84573899990672707 ) ) ;
#7820=CARTESIAN_POINT ( 'NONE',  ( -24.70764059509556532, 389.1823905765656377, -19.99999999999999289 ) ) ;
#7824=CARTESIAN_POINT ( 'NONE',  ( -24.70764059509553334, 254.8073905765656093, 19.99999999999998934 ) ) ;
#7827=CARTESIAN_POINT ( 'NONE',  ( -32.66413529028185536, 255.0573905601785043, -19.99999999999999289 ) ) ;
#7828=CARTESIAN_POINT ( 'NONE',  ( -36.33955658999050797, 345.3698905601784759, -18.47759065022572855 ) ) ;
#7831=CARTESIAN_POINT ( 'NONE',  ( -40.53162694259544452, 426.6198905683720000, 11.84573899990672885 ) ) ;
#7832=CARTESIAN_POINT ( 'NONE',  ( -8.685887942688887975, 266.6823905765656377, 3.978247347593586447 ) ) ;
#7833=CARTESIAN_POINT ( 'NONE',  ( -22.27502019258947286, 242.2448905683720000, -15.47720386886985544 ) ) ;
#7838=CARTESIAN_POINT ( 'NONE',  ( -25.35362745456399480, 468.1823905683720568, 16.75240474999998952 ) ) ;
#7839=CARTESIAN_POINT ( 'NONE',  ( -28.68588794268869790, 234.4948905765656377, 19.99999999999999289 ) ) ;
#7842=CARTESIAN_POINT ( 'NONE',  ( -40.53162694259545873, 534.1198905683720568, -11.84573899990672707 ) ) ;
#7844=CARTESIAN_POINT ( 'NONE',  ( -25.35362745456400191, 526.6823905683720568, 16.75240474999998952 ) ) ;
#7848=CARTESIAN_POINT ( 'NONE',  ( -14.54375231895778064, 448.2448905765656377, -14.14213562373094746 ) ) ;
#7849=CARTESIAN_POINT ( 'NONE',  ( -8.685887942688720997, 352.2448905601784759, -2.449293598294705724E-15 ) ) ;
#7850=CARTESIAN_POINT ( 'NONE',  ( -48.68588794268870146, 281.9948905765656377, 0.000000000000000000 ) ) ;
#7851=CARTESIAN_POINT ( 'NONE',  ( -8.685887942688708563, 236.9948905765656377, -2.449293598294705724E-15 ) ) ;
#7852=FACE_OUTER_BOUND ( 'NONE', #18272, .T. ) ;
#7853=CARTESIAN_POINT ( 'NONE',  ( -12.66381623556490332, 223.9102039777117454, 12.07890426730769029 ) ) ;
#7854=CARTESIAN_POINT ( 'NONE',  ( -22.27502019258945865, 226.9948905683720284, 15.47720386886985189 ) ) ;
#7855=CARTESIAN_POINT ( 'NONE',  ( -16.84014894278197971, 309.1198905683720000, 11.84573899990672530 ) ) ;
#7857=CARTESIAN_POINT ( 'NONE',  ( -8.685887942688729879, 442.2448905601785327, -2.449293598294705724E-15 ) ) ;
#7859=CARTESIAN_POINT ( 'NONE',  ( -45.43829269268870519, 305.3698905683720568, 0.000000000000000000 ) ) ;
#7860=CARTESIAN_POINT ( 'NONE',  ( -45.43829269268870519, 374.1823905683720568, 3.332260488124734632 ) ) ;
#7861=CARTESIAN_POINT ( 'NONE',  ( -14.48388495494901562, 519.4323905683719431, 9.489475012073731008 ) ) ;
#7862=CARTESIAN_POINT ( 'NONE',  ( -24.70764059509556176, 374.4323905601784759, -19.99999999999999289 ) ) ;
#7863=CARTESIAN_POINT ( 'NONE',  ( -10.20829729246299067, 402.8698905601784759, -7.653668647301794969 ) ) ;
#7865=CARTESIAN_POINT ( 'NONE',  ( -32.01814843081346140, 487.5573905683720568, 16.75240474999999307 ) ) ;
#7867=CARTESIAN_POINT ( 'NONE',  ( -16.84014894278197616, 277.6198905683720568, 11.84573899990672530 ) ) ;
#7868=EDGE_LOOP ( 'NONE', ( #17975, #13322, #20241, #1477 ) ) ;
#7869=CARTESIAN_POINT ( 'NONE',  ( -22.27502019258947641, 282.2448905683720568, -15.47720386886985544 ) ) ;
#7870=CARTESIAN_POINT ( 'NONE',  ( -14.48388495494899253, 317.9323905683720000, 9.489475012073732785 ) ) ;
#7871=CARTESIAN_POINT ( 'NONE',  ( -14.54375231895775933, 268.2448905765656377, -14.14213562373094746 ) ) ;
#7872=CARTESIAN_POINT ( 'NONE',  ( -21.03221929538693757, 474.1198905601784759, -18.47759065022572855 ) ) ;
#7873=CARTESIAN_POINT ( 'NONE',  ( -35.09675569278793006, 231.9948905683720284, -15.47720386886985544 ) ) ;
#7874=CARTESIAN_POINT ( 'NONE',  ( -42.88789093042843348, 376.3073905683720000, 9.489475012073736337 ) ) ;
#7877=EDGE_CURVE ( 'NONE', #10847, #1235, #13886, .T. ) ;
#7881=CARTESIAN_POINT ( 'NONE',  ( -13.20868407381886733, 438.2448905683720000, 6.410867750099229490 ) ) ;
#7884=CARTESIAN_POINT ( 'NONE',  ( -42.82802356641966668, 435.9948905601784759, -14.14213562373094746 ) ) ;
#7889=CARTESIAN_POINT ( 'NONE',  ( -21.03221929538691981, 324.1198905601784759, -18.47759065022572855 ) ) ;
#7891=CARTESIAN_POINT ( 'NONE',  ( -22.27502019258947641, 348.4948905683720000, 15.47720386886985189 ) ) ;
#7892=CARTESIAN_POINT ( 'NONE',  ( -42.82802356641967378, 500.7448905765656946, -14.14213562373094746 ) ) ;
#7893=CARTESIAN_POINT ( 'NONE',  ( -40.53162694259544452, 392.6198905683720568, -11.84573899990672707 ) ) ;
#7895=CARTESIAN_POINT ( 'NONE',  ( -13.20868407381886200, 379.4948905683720000, -6.410867750099233042 ) ) ;
#7896=AXIS2_PLACEMENT_3D ( 'NONE', #6518, #17784, #3075 ) ;
#7897=CARTESIAN_POINT ( 'NONE',  ( -24.70764059509555821, 329.1823905765656377, -19.99999999999999289 ) ) ;
#7898=CARTESIAN_POINT ( 'NONE',  ( -35.09675569278793716, 281.9948905683720000, -15.47720386886985544 ) ) ;
#7900=CARTESIAN_POINT ( 'NONE',  ( -45.43829269268871229, 435.6823905683720568, 3.332260488124734632 ) ) ;
#7902=CARTESIAN_POINT ( 'NONE',  ( -47.16347859291444422, 367.8698905601784759, 7.653668647301805628 ) ) ;
#7904=FACE_OUTER_BOUND ( 'NONE', #19346, .T. ) ;
#7905=CARTESIAN_POINT ( 'NONE',  ( -19.19641293061498288, 341.9323905683720568, -14.20200298773971603 ) ) ;
#7906=CARTESIAN_POINT ( 'NONE',  ( -28.68588794268873343, 511.3698905683720000, -16.75240474999999307 ) ) ;
#7907=CARTESIAN_POINT ( 'NONE',  ( -42.82802356641968089, 508.4948905601784759, 14.14213562373094923 ) ) ;
#7908=CARTESIAN_POINT ( 'NONE',  ( -19.19641293061497933, 327.3073905683720568, 14.20200298773971426 ) ) ;
#7910=CARTESIAN_POINT ( 'NONE',  ( -32.66413529028189089, 525.0573905601785327, -19.99999999999999289 ) ) ;
#7913=( BOUNDED_CURVE ( )  B_SPLINE_CURVE ( 2, ( #4334, #9189, #10915, #20781, #999, #17318, #7676, #4110, #7776, #5947, #15815, #20666, #19158, #9409, #7564, #16025, #20885 ),
 .UNSPECIFIED., .F., .T. ) 
 B_SPLINE_CURVE_WITH_KNOTS ( ( 3, 2, 2, 2, 2, 2, 2, 2, 3 ),
 ( 0.9062500000000001110, 0.9082031250000001110, 0.9101562500000001110, 0.9121093750000001110, 0.9140625000000001110, 0.9160156250000001110, 0.9179687500000001110, 0.9199218750000001110, 0.9218750000000001110 ),
 .UNSPECIFIED. ) 
 CURVE ( )  GEOMETRIC_REPRESENTATION_ITEM ( )  RATIONAL_B_SPLINE_CURVE ( ( 0.9999999999999988898, 0.9807852804032315408, 1.000000000000000000, 0.9807852804032304306, 1.000000000000000000, 0.9807852804032304306, 1.000000000000000000, 0.9807852804032304306, 1.000000000000000000, 0.9807852804032304306, 1.000000000000000000, 0.9807852804032304306, 1.000000000000000000, 0.9807852804032304306, 1.000000000000000000, 0.9807852804032293204, 1.000000000000001110 ) ) 
 REPRESENTATION_ITEM ( '' )  );
#7914=CARTESIAN_POINT ( 'NONE',  ( -25.35362745456399836, 422.5573905683721136, -16.75240474999999307 ) ) ;
#7916=LINE ( 'NONE', #3069, #15233 ) ;
#7917=CARTESIAN_POINT ( 'NONE',  ( -16.84014894278200103, 450.1198905683720568, -11.84573899990672707 ) ) ;
#7919=CARTESIAN_POINT ( 'NONE',  ( -25.35362745456400191, 451.0573905683719431, -16.75240474999999307 ) ) ;
#7922=CARTESIAN_POINT ( 'NONE',  ( -32.66413529028187668, 379.8073905765656377, -19.99999999999999289 ) ) ;
#7926=CARTESIAN_POINT ( 'NONE',  ( -40.01497788969911795, 253.5573905765656093, 16.95518130045146776 ) ) ;
#7927=CARTESIAN_POINT ( 'NONE',  ( -40.53162694259545873, 516.6198905683720568, 11.84573899990672885 ) ) ;
#7929=CARTESIAN_POINT ( 'NONE',  ( -8.685887942688530927, 252.5573905601784475, -3.978247347592740013 ) ) ;
#7930=CARTESIAN_POINT ( 'NONE',  ( -8.685887942688728103, 422.2448905601784759, -2.449293598294705724E-15 ) ) ;
#7931=CARTESIAN_POINT ( 'NONE',  ( -11.93348319268872970, 430.0573905683721136, 3.332260488124728415 ) ) ;
#7932=CARTESIAN_POINT ( 'NONE',  ( -17.35679799567827786, 265.4323905765656377, 16.95518130045146421 ) ) ;
#7934=CARTESIAN_POINT ( 'NONE',  ( -11.93348319268870661, 240.3698905683720568, -2.051577885510841163E-15 ) ) ;
#7935=ORIENTED_EDGE ( 'NONE', *, *, #10844, .T. ) ;
#7937=EDGE_LOOP ( 'NONE', ( #13340, #16672, #10855, #14834 ) ) ;
#7938=CARTESIAN_POINT ( 'NONE',  ( -38.17536295476246266, 466.9323905683721136, 14.20200298773971781 ) ) ;
#7939=CARTESIAN_POINT ( 'NONE',  ( -45.43829269268873361, 533.8698905683720568, 0.000000000000000000 ) ) ;
#7941=CARTESIAN_POINT ( 'NONE',  ( -8.685887942688742314, 573.2448905601785327, 2.449293598294706119E-15 ) ) ;
#7942=CARTESIAN_POINT ( 'NONE',  ( -11.93348319268874214, 530.0573905683720568, 3.332260488124728415 ) ) ;
#7944=CARTESIAN_POINT ( 'NONE',  ( -35.09675569278797269, 525.7448905683720568, 15.47720386886985366 ) ) ;
#7948=CARTESIAN_POINT ( 'NONE',  ( -42.82802356641966668, 440.7448905765656377, -14.14213562373094746 ) ) ;
#7950=CARTESIAN_POINT ( 'NONE',  ( -13.20868407381885845, 339.4948905683720568, -6.410867750099233042 ) ) ;
#7951=CARTESIAN_POINT ( 'NONE',  ( -8.685887942688733432, 456.9948905765656377, -2.449293598294705724E-15 ) ) ;
#7956=CARTESIAN_POINT ( 'NONE',  ( -25.35362745456396638, 236.6823905683720284, 16.75240474999998952 ) ) ;
#7958=CARTESIAN_POINT ( 'NONE',  ( -14.48388495494899253, 319.4323905683720568, 9.489475012073732785 ) ) ;
#7959=CARTESIAN_POINT ( 'NONE',  ( -45.64106924314018698, 446.3073905601784190, -11.32908994701042538 ) ) ;
#7960=CARTESIAN_POINT ( 'NONE',  ( -8.685887942688728103, 416.9948905765656377, -2.449293598294705724E-15 ) ) ;
#7961=CARTESIAN_POINT ( 'NONE',  ( -16.84014894278197971, 299.1198905683720000, 11.84573899990672530 ) ) ;
#7964=CARTESIAN_POINT ( 'NONE',  ( -45.43829269268870519, 364.1823905683720568, 3.332260488124734632 ) ) ;
#7966=CARTESIAN_POINT ( 'NONE',  ( -11.93348319268874214, 530.3698905683720568, -2.051577885510841163E-15 ) ) ;
#7967=CARTESIAN_POINT ( 'NONE',  ( -10.20829729246298712, 372.8698905601784759, -7.653668647301794969 ) ) ;
#7969=ORIENTED_EDGE ( 'NONE', *, *, #17936, .T. ) ;
#7970=CARTESIAN_POINT ( 'NONE',  ( -35.09675569278795848, 493.4948905683720568, -15.47720386886985544 ) ) ;
#7972=CARTESIAN_POINT ( 'NONE',  ( -14.48388495494898898, 287.9323905683720000, 9.489475012073732785 ) ) ;
#7975=ADVANCED_FACE ( 'NONE', ( #5486 ), #16970, .T. ) ;
#7976=CARTESIAN_POINT ( 'NONE',  ( -28.68588794268870856, 292.8698905683720568, -16.75240474999999307 ) ) ;
#7977=CARTESIAN_POINT ( 'NONE',  ( -44.16309181155857289, 333.2448905683720568, -6.410867750099231266 ) ) ;
#7978=CARTESIAN_POINT ( 'NONE',  ( -47.16347859291443001, 262.6198905765655809, 7.653668647301805628 ) ) ;
#7979=CARTESIAN_POINT ( 'NONE',  ( -32.66413529028188378, 475.0573905601785327, -19.99999999999999289 ) ) ;
#7982=CARTESIAN_POINT ( 'NONE',  ( -18.66797547166049753, 223.9102039777116602, -17.31025331282116397 ) ) ;
#7983=CARTESIAN_POINT ( 'NONE',  ( -28.68588794268871567, 377.8698905683720000, 16.75240474999999307 ) ) ;
#7985=CARTESIAN_POINT ( 'NONE',  ( -48.68588794268857356, 461.6823905765656377, -3.978247347593530936 ) ) ;
#7987=CARTESIAN_POINT ( 'NONE',  ( -45.43829269268871940, 413.8698905683720568, 0.000000000000000000 ) ) ;
#7990=CARTESIAN_POINT ( 'NONE',  ( -48.68588794268871567, 417.2448905601784759, 0.000000000000000000 ) ) ;
#7992=VERTEX_POINT ( 'NONE', #749 ) ;
#7994=CARTESIAN_POINT ( 'NONE',  ( -24.70764059509555466, 314.4323905601784190, -19.99999999999999289 ) ) ;
#7995=CYLINDRICAL_SURFACE ( 'NONE', #20096, 19.99999999999999645 ) ;
#7997=CARTESIAN_POINT ( 'NONE',  ( -45.43829269268871229, 345.0573905683720568, -3.332260488124726638 ) ) ;
#7998=CARTESIAN_POINT ( 'NONE',  ( -47.16347859291445843, 501.3698905765655809, -7.653668647301793193 ) ) ;
#7999=CARTESIAN_POINT ( 'NONE',  ( -40.53162694259543741, 382.6198905683720568, -11.84573899990672707 ) ) ;
#8001=CARTESIAN_POINT ( 'NONE',  ( -25.35362745456399480, 381.0573905683719431, -16.75240474999999307 ) ) ;
#8002=CARTESIAN_POINT ( 'NONE',  ( -47.16347859291444422, 331.3698905765656377, -7.653668647301793193 ) ) ;
#8003=CARTESIAN_POINT ( 'NONE',  ( -47.16347859291445133, 426.6198905601785327, -7.653668647301793193 ) ) ;
#8004=CARTESIAN_POINT ( 'NONE',  ( -45.43829269268870519, 283.5573905683721136, -3.332260488124726638 ) ) ;
#8005=CARTESIAN_POINT ( 'NONE',  ( -45.43829269268871229, 435.0573905683720568, -3.332260488124726194 ) ) ;
#8011=CARTESIAN_POINT ( 'NONE',  ( -32.01814843081344719, 353.1823905683720568, -16.75240474999999307 ) ) ;
#8012=CARTESIAN_POINT ( 'NONE',  ( -28.68588794268872633, 486.3698905683720568, 16.75240474999999307 ) ) ;
#8014=CARTESIAN_POINT ( 'NONE',  ( -47.16347859291445843, 477.8698905601784759, 7.653668647301805628 ) ) ;
#8015=CARTESIAN_POINT ( 'NONE',  ( -28.68588794268870856, 316.3698905683720568, 16.75240474999999307 ) ) ;
#8023=CARTESIAN_POINT ( 'NONE',  ( -22.27502019258949417, 412.2448905683720568, -15.47720386886985544 ) ) ;
#8024=CARTESIAN_POINT ( 'NONE',  ( -8.685887942688726326, 396.9948905765656377, -2.449293598294705724E-15 ) ) ;
#8025=CARTESIAN_POINT ( 'NONE',  ( -25.35362745456399125, 446.6823905683720568, 16.75240474999998952 ) ) ;
#8026=CARTESIAN_POINT ( 'NONE',  ( -32.01814843081344719, 446.0573905683720000, 16.75240474999999307 ) ) ;
#8029=B_SPLINE_CURVE_WITH_KNOTS ( 'NONE', 1,
 ( #10172, #8551 ),
 .UNSPECIFIED., .F., .F.,
 ( 2, 2 ),
 ( 0.000000000000000000, 1.000000000000000000 ),
 .UNSPECIFIED. ) ;
#8031=CARTESIAN_POINT ( 'NONE',  ( -47.16347859291444422, 381.3698905765656377, -7.653668647301793193 ) ) ;
#8033=CARTESIAN_POINT ( 'NONE',  ( -40.01497788969914637, 390.4323905765656377, -16.95518130045146421 ) ) ;
#8035=VECTOR ( 'NONE', #8463, 1000.000000000000000 ) ;
#8037=CARTESIAN_POINT ( 'NONE',  ( -28.68588794268872988, 497.8698905683720568, 16.75240474999999307 ) ) ;
#8039=LINE ( 'NONE', #19517, #13895 ) ;
#8040=CARTESIAN_POINT ( 'NONE',  ( -8.685887942689062058, 521.9323905601784190, 3.978247347593932837 ) ) ;
#8041=CARTESIAN_POINT ( 'NONE',  ( -40.53162694259544452, 414.1198905683720000, -11.84573899990672707 ) ) ;
#8042=CYLINDRICAL_SURFACE ( 'NONE', #13009, 19.99999999999999645 ) ;
#8043=( BOUNDED_CURVE ( )  B_SPLINE_CURVE ( 2, ( #14854, #20028, #18182, #11699, #6604, #18291, #3478, #8444, #11479, #253, #5204, #18077, #19814, #21328, #11800, #3379, #18397 ),
 .UNSPECIFIED., .F., .T. ) 
 B_SPLINE_CURVE_WITH_KNOTS ( ( 3, 2, 2, 2, 2, 2, 2, 2, 3 ),
 ( 0.06250000000000005551, 0.06445312500000009714, 0.06640625000000015266, 0.06835937500000019429, 0.07031250000000024980, 0.07226562500000029143, 0.07421875000000033307, 0.07617187500000038858, 0.07812500000000043021 ),
 .UNSPECIFIED. ) 
 CURVE ( )  GEOMETRIC_REPRESENTATION_ITEM ( )  RATIONAL_B_SPLINE_CURVE ( ( 0.9999999999999994449, 0.9807852804032309857, 1.000000000000000000, 0.9807852804032304306, 1.000000000000000000, 0.9807852804032304306, 1.000000000000000000, 0.9807852804032304306, 1.000000000000000000, 0.9807852804032304306, 1.000000000000000000, 0.9807852804032304306, 1.000000000000000000, 0.9807852804032304306, 1.000000000000000000, 0.9807852804032262117, 1.000000000000004219 ) ) 
 REPRESENTATION_ITEM ( '' )  );
#8044=CARTESIAN_POINT ( 'NONE',  ( -28.68588794268869790, 222.8698905683720284, -16.75240474999999307 ) ) ;
#8045=ORIENTED_EDGE ( 'NONE', *, *, #5512, .F. ) ;
#8048=CARTESIAN_POINT ( 'NONE',  ( -40.53162694259545162, 456.6198905683720568, 11.84573899990672885 ) ) ;
#8049=CARTESIAN_POINT ( 'NONE',  ( -28.68588794268869435, 224.4948905765656377, 19.99999999999999289 ) ) ;
#8052=CARTESIAN_POINT ( 'NONE',  ( -48.68588794268873698, 573.2448905601785327, 0.000000000000000000 ) ) ;
#8053=CARTESIAN_POINT ( 'NONE',  ( -25.35362745456400191, 528.1823905683719431, 16.75240474999998952 ) ) ;
#8056=CARTESIAN_POINT ( 'NONE',  ( -25.35362745456400901, 511.0573905683718863, -16.75240474999999307 ) ) ;
#8058=CARTESIAN_POINT ( 'NONE',  ( -45.64106924314020119, 451.0573905765656377, -11.32908994701042715 ) ) ;
#8062=CARTESIAN_POINT ( 'NONE',  ( -11.73070664223723547, 237.9323905765656093, -11.32908994701042538 ) ) ;
#8065=CARTESIAN_POINT ( 'NONE',  ( -32.01814843081343298, 231.6823905683720568, -16.75240474999999307 ) ) ;
#8066=CARTESIAN_POINT ( 'NONE',  ( -44.16309181155855867, 315.9948905683720568, 6.410867750099241924 ) ) ;
#8068=CARTESIAN_POINT ( 'NONE',  ( -8.685887942688712116, 271.9323905601785327, 3.978247347593161010 ) ) ;
#8070=CARTESIAN_POINT ( 'NONE',  ( -40.53162694259543031, 316.6198905683720568, 11.84573899990672885 ) ) ;
#8071=EDGE_CURVE ( 'NONE', #11409, #15181, #20634, .T. ) ;
#8072=CARTESIAN_POINT ( 'NONE',  ( -32.01814843081346140, 517.5573905683720568, 16.75240474999999307 ) ) ;
#8073=CARTESIAN_POINT ( 'NONE',  ( -8.685887942688722774, 362.2448905601784190, -2.449293598294705724E-15 ) ) ;
#8074=CARTESIAN_POINT ( 'NONE',  ( -42.82802356641965247, 315.9948905601784759, -14.14213562373094746 ) ) ;
#8075=ORIENTED_EDGE ( 'NONE', *, *, #18160, .T. ) ;
#8076=CARTESIAN_POINT ( 'NONE',  ( -28.68588794268872633, 477.8698905683720568, 16.75240474999999307 ) ) ;
#8078=DIRECTION ( 'NONE',  ( -1.000000000000000000, 0.000000000000000000, 0.000000000000000000 ) ) ;
#8079=CARTESIAN_POINT ( 'NONE',  ( -35.09675569278793716, 271.9948905683720000, -15.47720386886985544 ) ) ;
#8080=ORIENTED_EDGE ( 'NONE', *, *, #10844, .F. ) ;
#8081=CARTESIAN_POINT ( 'NONE',  ( -19.19641293061497578, 291.9323905683720568, -14.20200298773971603 ) ) ;
#8082=CARTESIAN_POINT ( 'NONE',  ( -40.53162694259543031, 312.6198905683720000, -11.84573899990672707 ) ) ;
#8083=CARTESIAN_POINT ( 'NONE',  ( -45.64106924314017988, 272.9323905765655809, 11.32908994701042715 ) ) ;
#8086=CARTESIAN_POINT ( 'NONE',  ( -44.16309181155857289, 374.7448905683720568, -6.410867750099231266 ) ) ;
#8091=CARTESIAN_POINT ( 'NONE',  ( -22.27502019258948351, 426.9948905683720568, 15.47720386886985189 ) ) ;
#8093=CARTESIAN_POINT ( 'NONE',  ( -28.68588794268874054, 573.2448905601785327, 0.000000000000000000 ) ) ;
#8094=ORIENTED_EDGE ( 'NONE', *, *, #3408, .F. ) ;
#8095=CARTESIAN_POINT ( 'NONE',  ( -14.54375231895777709, 423.4948905601784759, -14.14213562373094746 ) ) ;
#8098=CARTESIAN_POINT ( 'NONE',  ( -17.35679799567828852, 355.4323905765656377, 16.95518130045146421 ) ) ;
#8099=CARTESIAN_POINT ( 'NONE',  ( -36.33955658999050087, 315.3698905601784759, -18.47759065022572855 ) ) ;
#8100=CARTESIAN_POINT ( 'NONE',  ( -42.82802356641963826, 205.4725094246604442, -5.000000000000000888 ) ) ;
#8101=CARTESIAN_POINT ( 'NONE',  ( -14.48388495494899786, 351.3073905683720568, -9.489475012073734561 ) ) ;
#8102=CARTESIAN_POINT ( 'NONE',  ( -32.66413529028189799, 504.1823905765656946, 19.99999999999999289 ) ) ;
#8103=CARTESIAN_POINT ( 'NONE',  ( -22.27502019258947996, 376.9948905683720568, 15.47720386886985189 ) ) ;
#8104=CARTESIAN_POINT ( 'NONE',  ( -48.68588794268853803, 311.6823905765655809, -3.978247347593583783 ) ) ;
#8105=CARTESIAN_POINT ( 'NONE',  ( -42.88789093042844058, 394.8073905683720000, 9.489475012073734561 ) ) ;
#8107=CARTESIAN_POINT ( 'NONE',  ( -17.35679799567829562, 318.5573905765656377, -16.95518130045146421 ) ) ;
#8109=CARTESIAN_POINT ( 'NONE',  ( -42.88789093042842637, 292.9323905683720568, -9.489475012073734561 ) ) ;
#8111=CARTESIAN_POINT ( 'NONE',  ( -22.27502019258949417, 432.2448905683720000, -15.47720386886985544 ) ) ;
#8115=CARTESIAN_POINT ( 'NONE',  ( -48.68588794268870146, 317.2448905601784759, 0.000000000000000000 ) ) ;
#8117=CARTESIAN_POINT ( 'NONE',  ( -11.93348319268872260, 350.6823905683720000, -3.332260488124732856 ) ) ;
#8118=CARTESIAN_POINT ( 'NONE',  ( -19.19641293061500065, 490.4323905683720000, -14.20200298773971603 ) ) ;
#8120=CARTESIAN_POINT ( 'NONE',  ( -40.01497788969915348, 495.6823905601784759, -16.95518130045146421 ) ) ;
#8121=CARTESIAN_POINT ( 'NONE',  ( -22.27502019258947996, 310.7448905683720000, -15.47720386886985544 ) ) ;
#8126=CARTESIAN_POINT ( 'NONE',  ( -45.43829269268871940, 405.3698905683720000, 0.000000000000000000 ) ) ;
#8129=CARTESIAN_POINT ( 'NONE',  ( -44.16309181155857289, 444.4948905683720568, 6.410867750099241924 ) ) ;
#8130=CARTESIAN_POINT ( 'NONE',  ( -28.68588794268872633, 441.3698905683720000, -16.75240474999999307 ) ) ;
#8132=CARTESIAN_POINT ( 'NONE',  ( -45.64106924314018698, 416.3073905601785327, -11.32908994701042538 ) ) ;
#8133=CARTESIAN_POINT ( 'NONE',  ( -48.68588794268871567, 392.3073905765656377, 3.978247347593168115 ) ) ;
#8135=CYLINDRICAL_SURFACE ( 'NONE', #11303, 19.99999999999999645 ) ;
#8138=CARTESIAN_POINT ( 'NONE',  ( -16.84014894278200103, 489.1198905683720000, 11.84573899990672530 ) ) ;
#8141=CARTESIAN_POINT ( 'NONE',  ( -48.68588794268885067, 417.5573905601784759, 3.978247347592849259 ) ) ;
#8143=CARTESIAN_POINT ( 'NONE',  ( -19.19641293061498999, 411.9323905683720000, -14.20200298773971603 ) ) ;
#8144=CARTESIAN_POINT ( 'NONE',  ( -28.68588794268870146, 264.4948905765656377, 19.99999999999999289 ) ) ;
#8146=CARTESIAN_POINT ( 'NONE',  ( -19.19641293061497223, 231.9323905683720000, -14.20200298773971603 ) ) ;
#8150=CARTESIAN_POINT ( 'NONE',  ( -28.68588794268871922, 424.4948905765656377, 19.99999999999999289 ) ) ;
#8152=CARTESIAN_POINT ( 'NONE',  ( -45.43829269268871940, 435.6823905683720568, 3.332260488124734632 ) ) ;
#8153=CARTESIAN_POINT ( 'NONE',  ( -48.68588794268869435, 221.6823905765656662, -3.978247347593158345 ) ) ;
#8155=CARTESIAN_POINT ( 'NONE',  ( -43.67497163690818240, 210.1113231631601082, 0.6580207156766563203 ) ) ;
#8156=CARTESIAN_POINT ( 'NONE',  ( -25.35362745456396283, 226.6823905683720284, 16.75240474999998952 ) ) ;
#8158=CARTESIAN_POINT ( 'NONE',  ( -40.53162694259545162, 502.6198905683720568, -11.84573899990672707 ) ) ;
#8161=CARTESIAN_POINT ( 'NONE',  ( -17.35679799567830273, 445.4323905765656377, 16.95518130045146421 ) ) ;
#8162=CARTESIAN_POINT ( 'NONE',  ( -14.54375231895776288, 298.2448905765656377, -14.14213562373094746 ) ) ;
#8166=CARTESIAN_POINT ( 'NONE',  ( -8.685887942688713892, 292.2448905601784759, -2.449293598294705724E-15 ) ) ;
#8168=CARTESIAN_POINT ( 'NONE',  ( -34.34829387991847227, 223.9102039777116886, 19.24951607415172461 ) ) ;
#8172=CARTESIAN_POINT ( 'NONE',  ( -32.01814843081344009, 327.5573905683720568, 16.75240474999999307 ) ) ;
#8174=CARTESIAN_POINT ( 'NONE',  ( -36.33955658999050087, 269.1198905601784759, 18.47759065022572500 ) ) ;
#8175=CARTESIAN_POINT ( 'NONE',  ( -8.685887942688717445, 322.2448905601784759, -2.449293598294705724E-15 ) ) ;
#8176=CARTESIAN_POINT ( 'NONE',  ( -40.53162694259543031, 286.6198905683720000, 11.84573899990672885 ) ) ;
#8177=CARTESIAN_POINT ( 'NONE',  ( -25.35362745456401257, 532.5573905683720568, -16.75240474999999307 ) ) ;
#8178=CARTESIAN_POINT ( 'NONE',  ( -42.82802356641965957, 358.4948905601785327, 14.14213562373094923 ) ) ;
#8180=LINE ( 'NONE', #16534, #9089 ) ;
#8182=CARTESIAN_POINT ( 'NONE',  ( -40.53162694259545162, 484.1198905683720000, -11.84573899990672707 ) ) ;
#8184=CARTESIAN_POINT ( 'NONE',  ( -22.27502019258946575, 276.9948905683720000, 15.47720386886985189 ) ) ;
#8186=LINE ( 'NONE', #11146, #19021 ) ;
#8187=CARTESIAN_POINT ( 'NONE',  ( -45.43829269268870519, 275.0573905683720568, -3.332260488124726638 ) ) ;
#8188=CARTESIAN_POINT ( 'NONE',  ( -45.43829269268869808, 265.0573905683720568, -3.332260488124726638 ) ) ;
#8190=CARTESIAN_POINT ( 'NONE',  ( -8.685887942688708563, 237.3073905765656662, -3.978247347593165895 ) ) ;
#8191=CARTESIAN_POINT ( 'NONE',  ( -8.685887942688605534, 472.5573905601784759, -3.978247347592846594 ) ) ;
#8192=CARTESIAN_POINT ( 'NONE',  ( -32.01814843081343298, 226.0573905683720568, 16.75240474999999307 ) ) ;
#8193=CARTESIAN_POINT ( 'NONE',  ( -32.01814843081343298, 266.0573905683720568, 16.75240474999999307 ) ) ;
#8195=CARTESIAN_POINT ( 'NONE',  ( -28.68588794268871922, 382.8698905683720000, -16.75240474999999307 ) ) ;
#8198=CARTESIAN_POINT ( 'NONE',  ( -28.68588794268872988, 459.4948905765656377, -19.99999999999999289 ) ) ;
#8202=CARTESIAN_POINT ( 'NONE',  ( -32.01814843081345430, 426.0573905683720568, 16.75240474999999307 ) ) ;
#8203=DIRECTION ( 'NONE',  ( -1.191790137725560488E-16, 1.000000000000000000, -0.000000000000000000 ) ) ;
#8205=CARTESIAN_POINT ( 'NONE',  ( -40.01497788969913927, 418.8073905601785896, 16.95518130045146776 ) ) ;
#8210=CARTESIAN_POINT ( 'NONE',  ( -24.70764059509554755, 354.8073905765656377, 19.99999999999998934 ) ) ;
#8211=CARTESIAN_POINT ( 'NONE',  ( -11.73070664223724258, 303.1823905601784759, -11.32908994701042715 ) ) ;
#8213=CARTESIAN_POINT ( 'NONE',  ( -42.88789093042843348, 334.4323905683721136, -9.489475012073734561 ) ) ;
#8214=CARTESIAN_POINT ( 'NONE',  ( -28.68588794268872988, 479.4948905765656377, -19.99999999999999289 ) ) ;
#8215=CARTESIAN_POINT ( 'NONE',  ( -11.93348319268872260, 368.8698905683720000, -2.051577885510841163E-15 ) ) ;
#8216=CARTESIAN_POINT ( 'NONE',  ( -40.01497788969913216, 310.4323905765656377, -16.95518130045146421 ) ) ;
#8217=CARTESIAN_POINT ( 'NONE',  ( -38.17536295476246266, 392.3073905683720568, -14.20200298773971426 ) ) ;
#8218=EDGE_CURVE ( 'NONE', #7167, #1107, #7216, .T. ) ;
#8219=CARTESIAN_POINT ( 'NONE',  ( -47.16347859291443712, 311.3698905765656377, -7.653668647301793193 ) ) ;
#8221=CARTESIAN_POINT ( 'NONE',  ( -40.53162694259543031, 295.1198905683720000, 11.84573899990672885 ) ) ;
#8222=FACE_OUTER_BOUND ( 'NONE', #9416, .T. ) ;
#8223=CARTESIAN_POINT ( 'NONE',  ( -42.88789093042844058, 434.4323905683720568, -9.489475012073736337 ) ) ;
#8227=CARTESIAN_POINT ( 'NONE',  ( -47.16347859291445133, 447.8698905601785327, 7.653668647301805628 ) ) ;
#8228=CARTESIAN_POINT ( 'NONE',  ( -42.88789093042843348, 344.4323905683720000, -9.489475012073736337 ) ) ;
#8229=CARTESIAN_POINT ( 'NONE',  ( -38.17536295476246977, 492.3073905683720000, -14.20200298773971426 ) ) ;
#8231=CARTESIAN_POINT ( 'NONE',  ( -28.68588794268873343, 494.7448905601785327, -19.99999999999999289 ) ) ;
#8232=CARTESIAN_POINT ( 'NONE',  ( -35.09675569278793716, 311.9948905683720568, -15.47720386886985544 ) ) ;
#8235=CARTESIAN_POINT ( 'NONE',  ( -31.26501780185373391, 205.1437886375728965, 0.000000000000000000 ) ) ;
#8236=ORIENTED_EDGE ( 'NONE', *, *, #15232, .F. ) ;
#8238=CARTESIAN_POINT ( 'NONE',  ( -44.16309181155857999, 404.7448905683720568, -6.410867750099231266 ) ) ;
#8239=CARTESIAN_POINT ( 'NONE',  ( -48.68588794268870856, 377.2448905601784759, 0.000000000000000000 ) ) ;
#8240=CARTESIAN_POINT ( 'NONE',  ( -40.53162694259544452, 422.6198905683720000, -11.84573899990672707 ) ) ;
#8241=CARTESIAN_POINT ( 'NONE',  ( -16.84014894278200103, 450.1198905683720568, -11.84573899990672707 ) ) ;
#8243=CARTESIAN_POINT ( 'NONE',  ( -11.73070664223724968, 401.3073905601784190, 11.32908994701042005 ) ) ;
#8245=CARTESIAN_POINT ( 'NONE',  ( -21.03221929538691271, 375.1198905765656377, 18.47759065022572500 ) ) ;
#8250=CARTESIAN_POINT ( 'NONE',  ( -38.17536295476246977, 503.8073905683721136, -14.20200298773971426 ) ) ;
#8253=CARTESIAN_POINT ( 'NONE',  ( -28.68588794268872988, 519.7448905601784190, 19.99999999999999289 ) ) ;
#8255=CARTESIAN_POINT ( 'NONE',  ( -42.88789093042844058, 404.4323905683721136, -9.489475012073736337 ) ) ;
#8257=CARTESIAN_POINT ( 'NONE',  ( -42.88789093042841927, 224.4323905683720000, -9.489475012073736337 ) ) ;
#8259=CARTESIAN_POINT ( 'NONE',  ( -48.68588794268871567, 421.9948905765656377, 0.000000000000000000 ) ) ;
#8261=CARTESIAN_POINT ( 'NONE',  ( -40.53162694259544452, 434.1198905683720000, -11.84573899990672707 ) ) ;
#8262=CARTESIAN_POINT ( 'NONE',  ( -13.20868407381887977, 528.2448905683720568, 6.410867750099229490 ) ) ;
#8265=CARTESIAN_POINT ( 'NONE',  ( -28.68588794268873698, 532.8698905683719431, -16.75240474999999307 ) ) ;
#8266=VERTEX_POINT ( 'NONE', #4715 ) ;
#8267=CARTESIAN_POINT ( 'NONE',  ( -16.84014894278200813, 500.1198905683720000, -11.84573899990672707 ) ) ;
#8268=CARTESIAN_POINT ( 'NONE',  ( -8.685887942688848895, 491.9323905601785327, 3.978247347593427907 ) ) ;
#8270=CARTESIAN_POINT ( 'NONE',  ( -45.64106924314019409, 442.9323905765656377, 11.32908994701042715 ) ) ;
#8272=CARTESIAN_POINT ( 'NONE',  ( -21.03221929538690560, 330.3698905601784759, 18.47759065022572500 ) ) ;
#8273=LINE ( 'NONE', #14797, #135 ) ;
#8279=CARTESIAN_POINT ( 'NONE',  ( -45.43829269268869808, 305.6823905683719431, 3.332260488124734632 ) ) ;
#8281=CARTESIAN_POINT ( 'NONE',  ( -10.20829729246297646, 272.8698905601784759, -7.653668647301794969 ) ) ;
#8282=CARTESIAN_POINT ( 'NONE',  ( -47.16347859291445133, 412.6198905765656377, 7.653668647301805628 ) ) ;
#8283=CARTESIAN_POINT ( 'NONE',  ( -22.27502019258947996, 292.2448905683720000, -15.47720386886985544 ) ) ;
#8286=CARTESIAN_POINT ( 'NONE',  ( -11.93348319268873858, 510.3698905683720000, -2.051577885510841163E-15 ) ) ;
#8288=CARTESIAN_POINT ( 'NONE',  ( -21.03221929538692336, 374.1198905601785327, -18.47759065022572855 ) ) ;
#8290=AXIS2_PLACEMENT_3D ( 'NONE', #532, #5269, #18670 ) ;
#8291=CARTESIAN_POINT ( 'NONE',  ( -14.54375231895776466, 313.4948905601784759, -14.14213562373094746 ) ) ;
#8293=CARTESIAN_POINT ( 'NONE',  ( -19.19641293061499354, 461.9323905683720568, -14.20200298773971603 ) ) ;
#8295=CARTESIAN_POINT ( 'NONE',  ( -38.17536295476244845, 272.3073905683720000, -14.20200298773971426 ) ) ;
#8298=CARTESIAN_POINT ( 'NONE',  ( -22.27502019258946575, 278.4948905683720000, 15.47720386886985189 ) ) ;
#8300=EDGE_CURVE ( 'NONE', #8848, #16774, #18538, .T. ) ;
#8301=CARTESIAN_POINT ( 'NONE',  ( -42.82802356641964536, 240.7448905765656093, -14.14213562373094746 ) ) ;
#8304=CARTESIAN_POINT ( 'NONE',  ( -21.03221929538690560, 224.1198905601785043, -18.47759065022572855 ) ) ;
#8306=CARTESIAN_POINT ( 'NONE',  ( -45.43829269268869098, 263.5573905683720568, -3.332260488124726194 ) ) ;
#8307=CARTESIAN_POINT ( 'NONE',  ( -14.48388495494899963, 369.4323905683720000, 9.489475012073732785 ) ) ;
#8309=AXIS2_PLACEMENT_3D ( 'NONE', #5625, #12235, #6923 ) ;
#8311=CARTESIAN_POINT ( 'NONE',  ( -22.27502019258948351, 416.9948905683720000, 15.47720386886985189 ) ) ;
#8314=CARTESIAN_POINT ( 'NONE',  ( -47.16347859291445133, 426.6198905601785327, -7.653668647301793193 ) ) ;
#8319=CARTESIAN_POINT ( 'NONE',  ( -48.68588794268873698, 573.2448905601785327, 0.000000000000000000 ) ) ;
#8320=CARTESIAN_POINT ( 'NONE',  ( -42.82802356641965247, 308.4948905601784759, 14.14213562373094923 ) ) ;
#8322=CARTESIAN_POINT ( 'NONE',  ( -35.09675569278794427, 353.4948905683720000, -15.47720386886985544 ) ) ;
#8325=CARTESIAN_POINT ( 'NONE',  ( -10.20829729246300133, 487.6198905765656377, -7.653668647301794969 ) ) ;
#8326=CARTESIAN_POINT ( 'NONE',  ( -16.84014894278198682, 367.6198905683720000, 11.84573899990672530 ) ) ;
#8327=CARTESIAN_POINT ( 'NONE',  ( -40.53162694259544452, 395.1198905683720000, 11.84573899990672885 ) ) ;
#8328=CARTESIAN_POINT ( 'NONE',  ( -42.82802356641965247, 313.2448905765656377, 14.14213562373094923 ) ) ;
#8330=CARTESIAN_POINT ( 'NONE',  ( -32.01814843081343298, 266.0573905683720568, 16.75240474999999307 ) ) ;
#8331=CARTESIAN_POINT ( 'NONE',  ( -17.35679799567829917, 440.6823905601785327, 16.95518130045146421 ) ) ;
#8332=CARTESIAN_POINT ( 'NONE',  ( -11.93348319268872970, 440.0573905683720000, 3.332260488124728415 ) ) ;
#8333=CARTESIAN_POINT ( 'NONE',  ( -8.685887942688722774, 356.9948905765655809, -2.449293598294705724E-15 ) ) ;
#8334=CARTESIAN_POINT ( 'NONE',  ( -8.685887942689104690, 501.9323905601783622, 3.978247347594039418 ) ) ;
#8335=CYLINDRICAL_SURFACE ( 'NONE', #10912, 19.99999999999999645 ) ;
#8338=CARTESIAN_POINT ( 'NONE',  ( -14.48388495494899786, 341.3073905683720568, -9.489475012073736337 ) ) ;
#8339=CARTESIAN_POINT ( 'NONE',  ( -32.01814843081346140, 491.6823905683720000, -16.75240474999999307 ) ) ;
#8341=ORIENTED_EDGE ( 'NONE', *, *, #19545, .T. ) ;
#8342=CARTESIAN_POINT ( 'NONE',  ( -48.68588794268872277, 487.2448905601784759, 0.000000000000000000 ) ) ;
#8343=CARTESIAN_POINT ( 'NONE',  ( -45.43829269268869808, 303.5573905683720568, -3.332260488124726194 ) ) ;
#8348=CARTESIAN_POINT ( 'NONE',  ( -25.35362745456399480, 402.5573905683720568, -16.75240474999999307 ) ) ;
#8349=CARTESIAN_POINT ( 'NONE',  ( -45.64106924314017988, 376.3073905601784190, -11.32908994701042538 ) ) ;
#8351=CARTESIAN_POINT ( 'NONE',  ( -25.35362745456399836, 421.0573905683720000, -16.75240474999999307 ) ) ;
#8352=CARTESIAN_POINT ( 'NONE',  ( -25.35362745456398059, 262.5573905683720000, -16.75240474999999307 ) ) ;
#8353=CARTESIAN_POINT ( 'NONE',  ( -16.84014894278199748, 437.6198905683720000, 11.84573899990672530 ) ) ;
#8356=CARTESIAN_POINT ( 'NONE',  ( -8.685887942688720997, 356.6823905765656377, 3.978247347593161010 ) ) ;
#8358=CARTESIAN_POINT ( 'NONE',  ( -10.20829729246297468, 262.8698905601785327, -7.653668647301794969 ) ) ;
#8359=CARTESIAN_POINT ( 'NONE',  ( -42.82802356641966668, 430.7448905765656377, -14.14213562373094746 ) ) ;
#8362=CARTESIAN_POINT ( 'NONE',  ( -14.48388495494901562, 499.4323905683720000, 9.489475012073732785 ) ) ;
#8365=DIRECTION ( 'NONE',  ( -1.191790137725560488E-16, 1.000000000000000000, -0.000000000000000000 ) ) ;
#8366=CARTESIAN_POINT ( 'NONE',  ( -21.03221929538691626, 420.3698905601784759, 18.47759065022572500 ) ) ;
#8367=CARTESIAN_POINT ( 'NONE',  ( -16.84014894278199392, 409.1198905683720000, 11.84573899990672530 ) ) ;
#8368=CARTESIAN_POINT ( 'NONE',  ( -32.66413529028185536, 264.1823905765656946, 19.99999999999999289 ) ) ;
#8370=CARTESIAN_POINT ( 'NONE',  ( -40.53162694259542320, 226.6198905683720000, 11.84573899990672885 ) ) ;
#8371=CARTESIAN_POINT ( 'NONE',  ( -22.27502019258947641, 366.9948905683720568, 15.47720386886985189 ) ) ;
#8373=ORIENTED_EDGE ( 'NONE', *, *, #14403, .T. ) ;
#8374=CARTESIAN_POINT ( 'NONE',  ( -22.27502019258950483, 530.7448905683720568, -15.47720386886985544 ) ) ;
#8376=CARTESIAN_POINT ( 'NONE',  ( -32.01814843081345430, 453.1823905683720568, -16.75240474999999307 ) ) ;
#8377=CARTESIAN_POINT ( 'NONE',  ( -38.17536295476247687, 532.3073905683719431, -14.20200298773971426 ) ) ;
#8379=CARTESIAN_POINT ( 'NONE',  ( -48.68588794268872988, 531.6823905765655809, -3.978247347593157901 ) ) ;
#8380=CARTESIAN_POINT ( 'NONE',  ( -16.84014894278200458, 490.1198905683720000, -11.84573899990672707 ) ) ;
#8382=CARTESIAN_POINT ( 'NONE',  ( -16.84014894278200813, 510.1198905683720568, -11.84573899990672707 ) ) ;
#8384=CARTESIAN_POINT ( 'NONE',  ( -10.20829729246299422, 427.6198905765656377, -7.653668647301794969 ) ) ;
#8385=CARTESIAN_POINT ( 'NONE',  ( -48.68588794268870856, 361.9948905765655809, 0.000000000000000000 ) ) ;
#8386=CARTESIAN_POINT ( 'NONE',  ( -47.16347859291443001, 251.3698905765656093, -7.653668647301793193 ) ) ;
#8391=CYLINDRICAL_SURFACE ( 'NONE', #20109, 19.99999999999999645 ) ;
#8392=CARTESIAN_POINT ( 'NONE',  ( -8.685887942688703234, 223.9102039777117170, -1.743609257155848136 ) ) ;
#8393=CARTESIAN_POINT ( 'NONE',  ( -44.16309181155855867, 295.9948905683720000, 6.410867750099241924 ) ) ;
#8394=CARTESIAN_POINT ( 'NONE',  ( -8.685887942688742314, 532.2448905601784190, -2.449293598294705724E-15 ) ) ;
#8395=CARTESIAN_POINT ( 'NONE',  ( -40.01497788969912506, 278.8073905601785327, 16.95518130045146776 ) ) ;
#8397=CARTESIAN_POINT ( 'NONE',  ( -44.16309181155856578, 284.7448905683720568, -6.410867750099231266 ) ) ;
#8400=CARTESIAN_POINT ( 'NONE',  ( -22.27502019258950128, 512.2448905683720568, -15.47720386886985544 ) ) ;
#8404=CARTESIAN_POINT ( 'NONE',  ( -45.43829269268871940, 475.0573905683720000, -3.332260488124726194 ) ) ;
#8405=B_SPLINE_CURVE_WITH_KNOTS ( 'NONE', 3,
 ( #1529, #8100, #14729, #6482, #3885, #5191, #20439, #18383, #18804, #16780, #11788, #7121, #16990, #237, #6806, #10259, #20123, #13534, #3572, #660 ),
 .UNSPECIFIED., .F., .F.,
 ( 4, 2, 2, 2, 2, 2, 2, 2, 2, 4 ),
 ( 0.007875367097399143743, 0.008859169463295337929, 0.009842971829191532115, 0.01082677419508772804, 0.01181057656098392222, 0.01279437892688011641, 0.01377818129277631060, 0.01476198365867250478, 0.01525388484162060188, 0.01574578602456869897 ),
 .UNSPECIFIED. ) ;
#8406=CARTESIAN_POINT ( 'NONE',  ( -48.68588794268858067, 411.6823905765655240, -3.978247347593477201 ) ) ;
#8407=CARTESIAN_POINT ( 'NONE',  ( -32.01814843081343298, 266.0573905683720568, 16.75240474999999307 ) ) ;
#8408=ORIENTED_EDGE ( 'NONE', *, *, #10736, .F. ) ;
#8409=CARTESIAN_POINT ( 'NONE',  ( -14.54375231895776466, 335.7448905765655809, 14.14213562373094568 ) ) ;
#8410=CARTESIAN_POINT ( 'NONE',  ( -45.43829269268869808, 235.0573905683720568, -3.332260488124726638 ) ) ;
#8412=CARTESIAN_POINT ( 'NONE',  ( -10.20829729246297291, 246.3698905765656093, 7.653668647301790529 ) ) ;
#8413=CARTESIAN_POINT ( 'NONE',  ( 15.48595089668572555, 220.7569358267784025, 2.447515658234522107 ) ) ;
#8415=CARTESIAN_POINT ( 'NONE',  ( -19.19641293061497578, 260.4323905683720000, -14.20200298773971603 ) ) ;
#8416=EDGE_CURVE ( 'NONE', #12168, #4317, #15527, .T. ) ;
#8418=CARTESIAN_POINT ( 'NONE',  ( -45.43829269268870519, 365.0573905683720568, -3.332260488124726194 ) ) ;
#8421=CARTESIAN_POINT ( 'NONE',  ( -28.68588794268871922, 416.3698905683720568, 16.75240474999999307 ) ) ;
#8422=CARTESIAN_POINT ( 'NONE',  ( -32.66413529028186957, 339.8073905765656377, -19.99999999999999289 ) ) ;
#8424=CARTESIAN_POINT ( 'NONE',  ( -42.82802356641966668, 408.4948905601784759, 14.14213562373094923 ) ) ;
#8429=CARTESIAN_POINT ( 'NONE',  ( -40.53162694259545873, 534.1198905683720568, -11.84573899990672707 ) ) ;
#8430=CARTESIAN_POINT ( 'NONE',  ( -45.64106924314017988, 306.3073905601784190, -11.32908994701042715 ) ) ;
#8433=( BOUNDED_CURVE ( )  B_SPLINE_CURVE ( 2, ( #17775, #14543, #12806, #12914, #21129, #17980, #4683, #1140, #3068, #11173, #1342, #7599, #6087, #9652, #21237, #9759, #4582 ),
 .UNSPECIFIED., .F., .T. ) 
 B_SPLINE_CURVE_WITH_KNOTS ( ( 3, 2, 2, 2, 2, 2, 2, 2, 3 ),
 ( 0.9218750000000001110, 0.9238281250000001110, 0.9257812500000001110, 0.9277343750000001110, 0.9296875000000001110, 0.9316406250000001110, 0.9335937500000001110, 0.9355468750000001110, 0.9375000000000001110 ),
 .UNSPECIFIED. ) 
 CURVE ( )  GEOMETRIC_REPRESENTATION_ITEM ( )  RATIONAL_B_SPLINE_CURVE ( ( 0.9999999999999988898, 0.9807852804032315408, 1.000000000000000000, 0.9807852804032304306, 1.000000000000000000, 0.9807852804032304306, 1.000000000000000000, 0.9807852804032304306, 1.000000000000000000, 0.9807852804032304306, 1.000000000000000000, 0.9807852804032304306, 1.000000000000000000, 0.9807852804032304306, 1.000000000000000000, 0.9807852804032293204, 1.000000000000001110 ) ) 
 REPRESENTATION_ITEM ( '' )  );
#8435=CARTESIAN_POINT ( 'NONE',  ( -16.84014894278198682, 321.6198905683720568, -11.84573899990672707 ) ) ;
#8436=CARTESIAN_POINT ( 'NONE',  ( -32.01814843081344719, 356.0573905683719431, 16.75240474999999307 ) ) ;
#8437=CARTESIAN_POINT ( 'NONE',  ( -16.84014894278199037, 360.1198905683720000, -11.84573899990672707 ) ) ;
#8438=CARTESIAN_POINT ( 'NONE',  ( -45.64106924314017988, 302.9323905765655809, 11.32908994701042715 ) ) ;
#8440=CARTESIAN_POINT ( 'NONE',  ( -42.88789093042842637, 274.8073905683720000, 9.489475012073734561 ) ) ;
#8441=CARTESIAN_POINT ( 'NONE',  ( -40.01497788969913927, 438.8073905601784190, 16.95518130045146776 ) ) ;
#8442=CARTESIAN_POINT ( 'NONE',  ( -42.88789093042844058, 426.3073905683720568, 9.489475012073736337 ) ) ;
#8443=CARTESIAN_POINT ( 'NONE',  ( -28.68588794268874054, 573.2448905601785327, 0.000000000000000000 ) ) ;
#8444=CARTESIAN_POINT ( 'NONE',  ( -32.66413529028189089, 515.0573905601785327, -19.99999999999999289 ) ) ;
#8445=CARTESIAN_POINT ( 'NONE',  ( -8.685887942688742314, 573.2448905601785327, 2.449293598294706119E-15 ) ) ;
#8447=CARTESIAN_POINT ( 'NONE',  ( -25.35362745456397704, 328.1823905683720568, 16.75240474999998952 ) ) ;
#8448=CARTESIAN_POINT ( 'NONE',  ( -14.48388495494901029, 477.9323905683721136, 9.489475012073732785 ) ) ;
#8449=ORIENTED_EDGE ( 'NONE', *, *, #5505, .F. ) ;
#8450=CARTESIAN_POINT ( 'NONE',  ( -40.01497788969914637, 478.8073905601784759, 16.95518130045146776 ) ) ;
#8451=CARTESIAN_POINT ( 'NONE',  ( -35.09675569278793716, 301.9948905683720568, -15.47720386886985544 ) ) ;
#8452=ORIENTED_EDGE ( 'NONE', *, *, #17251, .F. ) ;
#8456=CARTESIAN_POINT ( 'NONE',  ( -32.01814843081344719, 413.1823905683719431, -16.75240474999999307 ) ) ;
#8457=CARTESIAN_POINT ( 'NONE',  ( -8.685887942688868435, 481.9323905601784759, 3.978247347593479866 ) ) ;
#8458=CARTESIAN_POINT ( 'NONE',  ( -45.64106924314017988, 382.9323905765656377, 11.32908994701042538 ) ) ;
#8459=CARTESIAN_POINT ( 'NONE',  ( -19.19641293061498999, 417.3073905683720568, 14.20200298773971426 ) ) ;
#8460=CARTESIAN_POINT ( 'NONE',  ( -45.43829269268869808, 265.3698905683720000, 0.000000000000000000 ) ) ;
#8461=CARTESIAN_POINT ( 'NONE',  ( -40.53162694259544452, 422.6198905683720000, -11.84573899990672707 ) ) ;
#8463=DIRECTION ( 'NONE',  ( -1.191790137725560488E-16, 1.000000000000000000, -0.000000000000000000 ) ) ;
#8465=CARTESIAN_POINT ( 'NONE',  ( -32.66413529028187668, 359.8073905765656946, -19.99999999999999289 ) ) ;
#8466=CARTESIAN_POINT ( 'NONE',  ( -8.685887942688712116, 272.2448905601784759, -2.449293598294705724E-15 ) ) ;
#8468=CARTESIAN_POINT ( 'NONE',  ( -32.01814843081344719, 331.6823905683720000, -16.75240474999999307 ) ) ;
#8470=CARTESIAN_POINT ( 'NONE',  ( -45.43829269268872650, 505.3698905683721136, 0.000000000000000000 ) ) ;
#8473=CARTESIAN_POINT ( 'NONE',  ( -8.685887942688742314, 573.2448905601785327, 2.449293598294706119E-15 ) ) ;
#8475=CARTESIAN_POINT ( 'NONE',  ( -35.09675569278795138, 387.2448905683720000, 15.47720386886985366 ) ) ;
#8476=CARTESIAN_POINT ( 'NONE',  ( -21.03221929538693757, 468.8698905765656377, -18.47759065022572855 ) ) ;
#8478=CARTESIAN_POINT ( 'NONE',  ( -32.01814843081343298, 227.5573905683720568, 16.75240474999999307 ) ) ;
#8479=CARTESIAN_POINT ( 'NONE',  ( -13.20868407381886023, 368.2448905683720000, 6.410867750099229490 ) ) ;
#8481=CARTESIAN_POINT ( 'NONE',  ( -38.17536295476246977, 515.4323905683720568, 14.20200298773971781 ) ) ;
#8483=CARTESIAN_POINT ( 'NONE',  ( -32.01814843081344719, 437.5573905683720000, 16.75240474999999307 ) ) ;
#8484=CARTESIAN_POINT ( 'NONE',  ( -22.27502019258950483, 530.7448905683720568, -15.47720386886985544 ) ) ;
#8487=CARTESIAN_POINT ( 'NONE',  ( -35.09675569278795848, 491.9948905683720568, -15.47720386886985544 ) ) ;
#8489=CARTESIAN_POINT ( 'NONE',  ( -32.01814843081346140, 506.0573905683719431, 16.75240474999999307 ) ) ;
#8491=CARTESIAN_POINT ( 'NONE',  ( -11.73070664223725501, 426.0573905765656377, 11.32908994701042005 ) ) ;
#8494=CARTESIAN_POINT ( 'NONE',  ( -48.68588794268861619, 486.9323905601785896, -3.978247347593425243 ) ) ;
#8496=( BOUNDED_CURVE ( )  B_SPLINE_CURVE ( 2, ( #1599, #19759, #13172, #4942, #19440, #18132, #4624, #16002, #1824, #13391, #3537, #8500, #5469, #6665, #6877, #5359, #10015 ),
 .UNSPECIFIED., .F., .T. ) 
 B_SPLINE_CURVE_WITH_KNOTS ( ( 3, 2, 2, 2, 2, 2, 2, 2, 3 ),
 ( 0.9375000000000001110, 0.9394531250000001110, 0.9414062500000001110, 0.9433593750000001110, 0.9453125000000001110, 0.9472656250000001110, 0.9492187500000001110, 0.9511718750000001110, 0.9531250000000001110 ),
 .UNSPECIFIED. ) 
 CURVE ( )  GEOMETRIC_REPRESENTATION_ITEM ( )  RATIONAL_B_SPLINE_CURVE ( ( 0.9999999999999988898, 0.9807852804032315408, 1.000000000000000000, 0.9807852804032304306, 1.000000000000000000, 0.9807852804032304306, 1.000000000000000000, 0.9807852804032304306, 1.000000000000000000, 0.9807852804032304306, 1.000000000000000000, 0.9807852804032304306, 1.000000000000000000, 0.9807852804032304306, 1.000000000000000000, 0.9807852804032293204, 1.000000000000001110 ) ) 
 REPRESENTATION_ITEM ( '' )  );
#8498=DIRECTION ( 'NONE',  ( -1.191790137725560488E-16, 1.000000000000000000, -0.000000000000000000 ) ) ;
#8499=CARTESIAN_POINT ( 'NONE',  ( -25.35362745456398414, 302.5573905683720000, -16.75240474999999307 ) ) ;
#8500=CARTESIAN_POINT ( 'NONE',  ( -17.35679799567828141, 233.8073905601784759, -16.95518130045146421 ) ) ;
#8501=CARTESIAN_POINT ( 'NONE',  ( -17.35679799567828852, 263.8073905601784759, -16.95518130045146421 ) ) ;
#8503=CARTESIAN_POINT ( 'NONE',  ( -16.84014894278198327, 291.6198905683720000, -11.84573899990672707 ) ) ;
#8504=ORIENTED_EDGE ( 'NONE', *, *, #11734, .T. ) ;
#8505=CARTESIAN_POINT ( 'NONE',  ( -14.54375231895775578, 270.9948905601784759, 14.14213562373094568 ) ) ;
#8506=CARTESIAN_POINT ( 'NONE',  ( -45.43829269268872650, 505.0573905683720568, -3.332260488124726638 ) ) ;
#8510=CARTESIAN_POINT ( 'NONE',  ( -13.20868407381887089, 459.7448905683720568, 6.410867750099229490 ) ) ;
#8511=CARTESIAN_POINT ( 'NONE',  ( -8.685887942688726326, 406.9948905765656377, -2.449293598294705724E-15 ) ) ;
#8512=CARTESIAN_POINT ( 'NONE',  ( -16.84014894278197616, 257.6198905683720568, 11.84573899990672530 ) ) ;
#8513=ORIENTED_EDGE ( 'NONE', *, *, #14518, .F. ) ;
#8514=CARTESIAN_POINT ( 'NONE',  ( -42.82802356641965957, 333.2448905765656377, 14.14213562373094923 ) ) ;
#8516=CARTESIAN_POINT ( 'NONE',  ( -22.27502019258946220, 238.4948905683720284, 15.47720386886985189 ) ) ;
#8518=CARTESIAN_POINT ( 'NONE',  ( -42.82802356641964536, 243.2448905765656093, 14.14213562373094923 ) ) ;
#8520=CARTESIAN_POINT ( 'NONE',  ( -28.68588794268869435, 229.7448905601785043, 19.99999999999999289 ) ) ;
#8521=CARTESIAN_POINT ( 'NONE',  ( -45.43829269268870519, 273.8698905683720000, 0.000000000000000000 ) ) ;
#8522=CARTESIAN_POINT ( 'NONE',  ( -11.93348319268872260, 360.0573905683719431, 3.332260488124728415 ) ) ;
#8524=CARTESIAN_POINT ( 'NONE',  ( -21.03221929538694113, 504.1198905601784759, -18.47759065022572855 ) ) ;
#8526=CARTESIAN_POINT ( 'NONE',  ( -40.53162694259544452, 395.1198905683720000, 11.84573899990672885 ) ) ;
#8527=CARTESIAN_POINT ( 'NONE',  ( -14.54375231895776821, 338.2448905765656377, -14.14213562373094746 ) ) ;
#8529=CARTESIAN_POINT ( 'NONE',  ( -48.68588794268871567, 406.9323905601784759, -3.978247347593158345 ) ) ;
#8534=CARTESIAN_POINT ( 'NONE',  ( -13.20868407381887977, 520.9948905683720568, -6.410867750099233042 ) ) ;
#8535=CARTESIAN_POINT ( 'NONE',  ( -40.01497788969913216, 285.6823905601784759, -16.95518130045146421 ) ) ;
#8538=CARTESIAN_POINT ( 'NONE',  ( -38.17536295476244135, 326.9323905683720568, 14.20200298773971781 ) ) ;
#8540=CARTESIAN_POINT ( 'NONE',  ( -11.93348319268872082, 358.8698905683720000, -2.051577885510841163E-15 ) ) ;
#8541=CARTESIAN_POINT ( 'NONE',  ( -11.93348319268872260, 369.1823905683720000, -3.332260488124732856 ) ) ;
#8543=CARTESIAN_POINT ( 'NONE',  ( -21.03221929538690205, 295.1198905765656377, 18.47759065022572500 ) ) ;
#8545=CARTESIAN_POINT ( 'NONE',  ( -14.48388495494898542, 257.9323905683720000, 9.489475012073731008 ) ) ;
#8546=CARTESIAN_POINT ( 'NONE',  ( -8.685887942688735208, 466.9948905765656377, -2.449293598294705724E-15 ) ) ;
#8548=CARTESIAN_POINT ( 'NONE',  ( -38.17536295476246266, 413.8073905683719431, -14.20200298773971426 ) ) ;
#8549=EDGE_CURVE ( 'NONE', #18118, #20734, #3759, .T. ) ;
#8551=CARTESIAN_POINT ( 'NONE',  ( -48.68588794268872988, 537.2448905601785327, 0.000000000000000000 ) ) ;
#8552=CARTESIAN_POINT ( 'NONE',  ( -8.685887942688902186, 381.9323905601784759, 3.978247347593586447 ) ) ;
#8553=CARTESIAN_POINT ( 'NONE',  ( -24.70764059509555466, 410.0573905601784759, 19.99999999999998934 ) ) ;
#8554=CARTESIAN_POINT ( 'NONE',  ( -19.19641293061498288, 321.9323905683720000, -14.20200298773971603 ) ) ;
#8555=CARTESIAN_POINT ( 'NONE',  ( -11.93348319268873325, 458.8698905683720000, -2.051577885510841163E-15 ) ) ;
#8557=CARTESIAN_POINT ( 'NONE',  ( -10.20829729246299777, 462.8698905601785327, -7.653668647301794969 ) ) ;
#8558=CARTESIAN_POINT ( 'NONE',  ( -14.48388495494899075, 297.9323905683720000, 9.489475012073732785 ) ) ;
#8562=CARTESIAN_POINT ( 'NONE',  ( -8.685887942688719221, 342.5573905601785327, -3.978247347593165895 ) ) ;
#8563=CARTESIAN_POINT ( 'NONE',  ( -35.09675569278794427, 383.4948905683720000, -15.47720386886985544 ) ) ;
#8566=CARTESIAN_POINT ( 'NONE',  ( -38.17536295476246266, 422.3073905683720568, -14.20200298773971426 ) ) ;
#8567=CARTESIAN_POINT ( 'NONE',  ( -22.27502019258946575, 268.4948905683720000, 15.47720386886985189 ) ) ;
#8568=CARTESIAN_POINT ( 'NONE',  ( -28.68588794268871922, 426.3698905683720568, 16.75240474999999307 ) ) ;
#8569=CARTESIAN_POINT ( 'NONE',  ( -10.20829729246299067, 401.6198905601784759, 7.653668647301790529 ) ) ;
#8570=CARTESIAN_POINT ( 'NONE',  ( -17.35679799567829917, 358.5573905765655809, -16.95518130045146421 ) ) ;
#8572=CYLINDRICAL_SURFACE ( 'NONE', #6117, 19.99999999999999645 ) ;
#8573=CARTESIAN_POINT ( 'NONE',  ( -35.09675569278794427, 331.9948905683720000, -15.47720386886985544 ) ) ;
#8574=DIRECTION ( 'NONE',  ( -1.191790137725560488E-16, 1.000000000000000000, -0.000000000000000000 ) ) ;
#8575=CARTESIAN_POINT ( 'NONE',  ( -19.19641293061499354, 478.8073905683720568, 14.20200298773971426 ) ) ;
#8576=CARTESIAN_POINT ( 'NONE',  ( -48.68588794268880804, 432.3073905765656377, 3.978247347592954952 ) ) ;
#8578=CARTESIAN_POINT ( 'NONE',  ( -8.685887942688449215, 302.5573905601784759, -3.978247347592526850 ) ) ;
#8579=CARTESIAN_POINT ( 'NONE',  ( -38.17536295476244845, 386.9323905683721136, 14.20200298773971781 ) ) ;
#8581=CARTESIAN_POINT ( 'NONE',  ( -24.70764059509558308, 524.4323905601785327, -19.99999999999999289 ) ) ;
#8582=CARTESIAN_POINT ( 'NONE',  ( -32.01814843081344719, 366.0573905683720000, 16.75240474999999307 ) ) ;
#8585=CARTESIAN_POINT ( 'NONE',  ( -38.17536295476247687, 532.3073905683719431, -14.20200298773971426 ) ) ;
#8587=CARTESIAN_POINT ( 'NONE',  ( -42.88789093042845479, 514.8073905683720568, 9.489475012073736337 ) ) ;
#8589=CARTESIAN_POINT ( 'NONE',  ( -48.68588794268880804, 427.5573905601784190, 3.978247347592954952 ) ) ;
#8590=CARTESIAN_POINT ( 'NONE',  ( -13.20868407381887621, 489.4948905683720568, -6.410867750099233042 ) ) ;
#8592=CARTESIAN_POINT ( 'NONE',  ( -35.09675569278795848, 481.9948905683720000, -15.47720386886985544 ) ) ;
#8593=CARTESIAN_POINT ( 'NONE',  ( -42.82802356641967378, 488.4948905601784759, 14.14213562373094923 ) ) ;
#8594=CARTESIAN_POINT ( 'NONE',  ( -32.66413529028188378, 419.8073905765655809, -19.99999999999999289 ) ) ;
#8597=CARTESIAN_POINT ( 'NONE',  ( -24.70764059509556887, 439.1823905765655809, -19.99999999999999289 ) ) ;
#8600=CARTESIAN_POINT ( 'NONE',  ( -32.66413529028188378, 494.1823905765655240, 19.99999999999999289 ) ) ;
#8601=CARTESIAN_POINT ( 'NONE',  ( -40.53162694259543031, 296.6198905683720000, 11.84573899990672885 ) ) ;
#8603=CARTESIAN_POINT ( 'NONE',  ( -45.43829269268871940, 445.3698905683720000, 0.000000000000000000 ) ) ;
#8605=CARTESIAN_POINT ( 'NONE',  ( -45.43829269268869808, 295.0573905683720000, -3.332260488124726194 ) ) ;
#8607=CARTESIAN_POINT ( 'NONE',  ( -17.35679799567831694, 533.8073905601784190, -16.95518130045146421 ) ) ;
#8608=CARTESIAN_POINT ( 'NONE',  ( -28.68588794268873343, 502.8698905683719431, -16.75240474999999307 ) ) ;
#8609=AXIS2_PLACEMENT_3D ( 'NONE', #14428, #9951, #19588 ) ;
#8612=CARTESIAN_POINT ( 'NONE',  ( -22.27502019258949062, 468.4948905683720000, 15.47720386886985189 ) ) ;
#8614=CARTESIAN_POINT ( 'NONE',  ( -45.43829269268869098, 263.5573905683720568, -3.332260488124726194 ) ) ;
#8617=CARTESIAN_POINT ( 'NONE',  ( -48.68588794268887199, 332.3073905765655240, 3.978247347592742678 ) ) ;
#8619=CARTESIAN_POINT ( 'NONE',  ( -19.19641293061496867, 268.8073905683720568, 14.20200298773971426 ) ) ;
#8620=CARTESIAN_POINT ( 'NONE',  ( -8.685887942688717445, 306.9948905765655809, -2.449293598294705724E-15 ) ) ;
#8622=CARTESIAN_POINT ( 'NONE',  ( -32.01814843081343298, 237.5573905683720568, 16.75240474999999307 ) ) ;
#8623=CARTESIAN_POINT ( 'NONE',  ( -47.16347859291443712, 307.8698905601784759, 7.653668647301805628 ) ) ;
#8624=CYLINDRICAL_SURFACE ( 'NONE', #15641, 19.99999999999999645 ) ;
#8625=CARTESIAN_POINT ( 'NONE',  ( -22.27502019258947641, 260.7448905683720000, -15.47720386886985544 ) ) ;
#8626=CARTESIAN_POINT ( 'NONE',  ( -45.43829269268871229, 355.3698905683720568, 0.000000000000000000 ) ) ;
#8629=CARTESIAN_POINT ( 'NONE',  ( -32.01814843081345430, 406.0573905683720000, 16.75240474999999307 ) ) ;
#8630=CARTESIAN_POINT ( 'NONE',  ( -48.68588794268872277, 507.2448905601785327, 0.000000000000000000 ) ) ;
#8631=VECTOR ( 'NONE', #13456, 1000.000000000000000 ) ;
#8632=CARTESIAN_POINT ( 'NONE',  ( -11.73070664223725501, 403.1823905601785327, -11.32908994701042715 ) ) ;
#8634=EDGE_LOOP ( 'NONE', ( #19790, #9893, #15765, #6610 ) ) ;
#8638=CARTESIAN_POINT ( 'NONE',  ( -14.48388495494901740, 519.4323905683720568, 9.489475012073732785 ) ) ;
#8639=CARTESIAN_POINT ( 'NONE',  ( -8.685887942688712116, 281.9323905601784759, 3.978247347593161010 ) ) ;
#8640=CARTESIAN_POINT ( 'NONE',  ( -48.68588794268870146, 321.9948905765655809, 0.000000000000000000 ) ) ;
#8641=CARTESIAN_POINT ( 'NONE',  ( -42.88789093042842637, 316.3073905683721136, 9.489475012073734561 ) ) ;
#8642=VERTEX_POINT ( 'NONE', #1043 ) ;
#8643=CARTESIAN_POINT ( 'NONE',  ( -38.17536295476244845, 365.4323905683720000, 14.20200298773971781 ) ) ;
#8644=CARTESIAN_POINT ( 'NONE',  ( -38.17536295476244845, 375.4323905683720000, 14.20200298773971781 ) ) ;
#8646=CARTESIAN_POINT ( 'NONE',  ( -32.66413529028186957, 299.8073905765656377, -19.99999999999999289 ) ) ;
#8649=CARTESIAN_POINT ( 'NONE',  ( -28.68588794268869790, 256.3698905683720000, 16.75240474999999307 ) ) ;
#8650=CARTESIAN_POINT ( 'NONE',  ( -42.87301415892787304, 204.0033847496196984, 4.870997244581528385 ) ) ;
#8652=CARTESIAN_POINT ( 'NONE',  ( -38.17536295476246266, 423.8073905683720568, -14.20200298773971426 ) ) ;
#8655=CARTESIAN_POINT ( 'NONE',  ( -48.68588794268871567, 411.9948905765656377, 0.000000000000000000 ) ) ;
#8659=CARTESIAN_POINT ( 'NONE',  ( -40.53162694259543741, 336.6198905683720000, 11.84573899990672885 ) ) ;
#8660=CARTESIAN_POINT ( 'NONE',  ( -16.84014894278200103, 467.6198905683720000, 11.84573899990672530 ) ) ;
#8662=CARTESIAN_POINT ( 'NONE',  ( -40.01497788969914637, 468.8073905601785327, 16.95518130045146776 ) ) ;
#8663=CARTESIAN_POINT ( 'NONE',  ( -11.93348319268871194, 288.8698905683720568, -2.051577885510841163E-15 ) ) ;
#8665=CARTESIAN_POINT ( 'NONE',  ( -8.685887942688720997, 346.9948905765656377, -2.449293598294705724E-15 ) ) ;
#8668=CARTESIAN_POINT ( 'NONE',  ( -17.35679799567828852, 340.6823905601785896, 16.95518130045146421 ) ) ;
#8669=CARTESIAN_POINT ( 'NONE',  ( -45.43829269268869808, 294.1823905683720000, 3.332260488124734632 ) ) ;
#8670=CARTESIAN_POINT ( 'NONE',  ( -16.84014894278199037, 389.1198905683720568, 11.84573899990672530 ) ) ;
#8671=CARTESIAN_POINT ( 'NONE',  ( -45.64106924314017277, 296.3073905601784190, -11.32908994701042538 ) ) ;
#8672=DIRECTION ( 'NONE',  ( -1.191790137725560488E-16, 1.000000000000000000, -0.000000000000000000 ) ) ;
#8673=CARTESIAN_POINT ( 'NONE',  ( -14.48388495494900496, 419.8073905683720000, -9.489475012073736337 ) ) ;
#8674=CARTESIAN_POINT ( 'NONE',  ( -22.27502019258946220, 258.4948905683720568, 15.47720386886985189 ) ) ;
#8675=CARTESIAN_POINT ( 'NONE',  ( -11.93348319268872793, 419.1823905683720568, -3.332260488124732856 ) ) ;
#8676=PRODUCT_CONTEXT ( 'NONE', #20085, 'mechanical' ) ;
#8677=CARTESIAN_POINT ( 'NONE',  ( -28.68588794268871567, 369.4948905765656377, -19.99999999999999289 ) ) ;
#8679=CARTESIAN_POINT ( 'NONE',  ( -19.19641293061497933, 330.4323905683720568, -14.20200298773971603 ) ) ;
#8680=CARTESIAN_POINT ( 'NONE',  ( -14.54375231895778597, 488.2448905765656377, -14.14213562373094746 ) ) ;
#8681=CARTESIAN_POINT ( 'NONE',  ( -25.35362745456399480, 468.1823905683721136, 16.75240474999998952 ) ) ;
#8682=EDGE_CURVE ( 'NONE', #3367, #19032, #19244, .T. ) ;
#8683=CARTESIAN_POINT ( 'NONE',  ( -8.685887942688729879, 436.9948905765656377, -2.449293598294705724E-15 ) ) ;
#8689=CARTESIAN_POINT ( 'NONE',  ( -19.19641293061498644, 388.8073905683720568, 14.20200298773971426 ) ) ;
#8691=CARTESIAN_POINT ( 'NONE',  ( -40.01497788969916058, 535.6823905601784190, -16.95518130045146421 ) ) ;
#8692=CARTESIAN_POINT ( 'NONE',  ( -14.48388495494899608, 347.9323905683720000, 9.489475012073732785 ) ) ;
#8694=CARTESIAN_POINT ( 'NONE',  ( -42.88789093042845479, 522.9323905683720568, -9.489475012073736337 ) ) ;
#8696=CARTESIAN_POINT ( 'NONE',  ( -8.685887942688719221, 351.9323905601784759, 3.978247347593161010 ) ) ;
#8697=CARTESIAN_POINT ( 'NONE',  ( -45.43829269268873361, 513.8698905683720568, 0.000000000000000000 ) ) ;
#8701=CARTESIAN_POINT ( 'NONE',  ( -38.17536295476246266, 475.4323905683720568, 14.20200298773971781 ) ) ;
#8703=CARTESIAN_POINT ( 'NONE',  ( -16.84014894278200103, 487.6198905683720000, 11.84573899990672530 ) ) ;
#8705=CARTESIAN_POINT ( 'NONE',  ( -48.68588794268871567, 431.9948905765656377, 0.000000000000000000 ) ) ;
#8706=CARTESIAN_POINT ( 'NONE',  ( -32.66413529028188378, 474.1823905765655809, 19.99999999999999289 ) ) ;
#8708=CARTESIAN_POINT ( 'NONE',  ( -14.54375231895778420, 483.4948905601784759, -14.14213562373094746 ) ) ;
#8713=CARTESIAN_POINT ( 'NONE',  ( -44.16309181155856578, 294.7448905683720568, -6.410867750099231266 ) ) ;
#8715=CARTESIAN_POINT ( 'NONE',  ( -40.53162694259544452, 446.6198905683720568, 11.84573899990672885 ) ) ;
#8718=CARTESIAN_POINT ( 'NONE',  ( -11.93348319268871194, 270.0573905683719431, 3.332260488124728415 ) ) ;
#8721=CARTESIAN_POINT ( 'NONE',  ( -14.48388495494901562, 511.3073905683720568, -9.489475012073734561 ) ) ;
#8723=CARTESIAN_POINT ( 'NONE',  ( -32.01814843081346140, 457.5573905683720000, 16.75240474999999307 ) ) ;
#8724=FACE_OUTER_BOUND ( 'NONE', #15376, .T. ) ;
#8725=CARTESIAN_POINT ( 'NONE',  ( -14.48388495494898898, 269.8073905683720000, -9.489475012073736337 ) ) ;
#8728=CYLINDRICAL_SURFACE ( 'NONE', #1785, 19.99999999999999645 ) ;
#8729=CARTESIAN_POINT ( 'NONE',  ( -28.68588794268870501, 272.8698905683720000, -16.75240474999999307 ) ) ;
#8730=CARTESIAN_POINT ( 'NONE',  ( -10.20829729246299955, 476.3698905765656377, 7.653668647301790529 ) ) ;
#8732=CARTESIAN_POINT ( 'NONE',  ( -13.20868407381884602, 249.7448905683720000, 6.410867750099229490 ) ) ;
#8733=CARTESIAN_POINT ( 'NONE',  ( -40.01497788969914637, 420.4323905765656377, -16.95518130045146421 ) ) ;
#8734=CARTESIAN_POINT ( 'NONE',  ( -21.03221929538689494, 230.3698905601784759, 18.47759065022572500 ) ) ;
#8736=CARTESIAN_POINT ( 'NONE',  ( -16.84014894278197616, 250.1198905683720284, -11.84573899990672707 ) ) ;
#8737=CARTESIAN_POINT ( 'NONE',  ( -19.19641293061498644, 351.9323905683720568, -14.20200298773971603 ) ) ;
#8742=CARTESIAN_POINT ( 'NONE',  ( -13.20868407381886556, 409.4948905683720000, -6.410867750099233042 ) ) ;
#8744=CARTESIAN_POINT ( 'NONE',  ( -8.685887942688543362, 337.3073905765656377, -3.978247347592740013 ) ) ;
#8745=( BOUNDED_CURVE ( )  B_SPLINE_CURVE ( 2, ( #6956, #13677, #7059, #16820, #3715, #10199, #18740, #15516, #10623, #12260, #2010, #13579, #15309, #20268, #15200, #8578, #17239 ),
 .UNSPECIFIED., .F., .T. ) 
 B_SPLINE_CURVE_WITH_KNOTS ( ( 3, 2, 2, 2, 2, 2, 2, 2, 3 ),
 ( 0.7187500000000002220, 0.7207031250000002220, 0.7226562500000002220, 0.7246093750000002220, 0.7265625000000002220, 0.7285156250000003331, 0.7304687500000003331, 0.7324218750000003331, 0.7343750000000003331 ),
 .UNSPECIFIED. ) 
 CURVE ( )  GEOMETRIC_REPRESENTATION_ITEM ( )  RATIONAL_B_SPLINE_CURVE ( ( 0.9999999999999977796, 0.9807852804032326510, 1.000000000000000000, 0.9807852804032304306, 1.000000000000000000, 0.9807852804032304306, 1.000000000000000000, 0.9807852804032304306, 1.000000000000000000, 0.9807852804032304306, 1.000000000000000000, 0.9807852804032304306, 1.000000000000000000, 0.9807852804032304306, 1.000000000000000000, 0.9807852804032270999, 1.000000000000003331 ) ) 
 REPRESENTATION_ITEM ( '' )  );
#8746=CARTESIAN_POINT ( 'NONE',  ( -21.03221929538691271, 400.3698905601785327, 18.47759065022572500 ) ) ;
#8748=CARTESIAN_POINT ( 'NONE',  ( -11.73070664223724791, 347.9323905765655809, -11.32908994701042538 ) ) ;
#8749=VERTEX_POINT ( 'NONE', #19090 ) ;
#8751=CARTESIAN_POINT ( 'NONE',  ( -45.43829269268872650, 525.6823905683719431, 3.332260488124734632 ) ) ;
#8752=CARTESIAN_POINT ( 'NONE',  ( -45.64106924314017988, 286.3073905601785327, -11.32908994701042715 ) ) ;
#8754=VECTOR ( 'NONE', #9255, 1000.000000000000000 ) ;
#8755=CARTESIAN_POINT ( 'NONE',  ( -40.53162694259543031, 314.1198905683720568, -11.84573899990672707 ) ) ;
#8757=CARTESIAN_POINT ( 'NONE',  ( -22.27502019258947286, 336.9948905683720000, 15.47720386886985189 ) ) ;
#8759=CARTESIAN_POINT ( 'NONE',  ( -25.35362745456399125, 361.0573905683720000, -16.75240474999999307 ) ) ;
#8760=CARTESIAN_POINT ( 'NONE',  ( -47.16347859291443712, 291.3698905765655809, -7.653668647301793193 ) ) ;
#8762=CARTESIAN_POINT ( 'NONE',  ( -22.27502019258947641, 270.7448905683720568, -15.47720386886985544 ) ) ;
#8763=CARTESIAN_POINT ( 'NONE',  ( -42.83955070047271363, 204.4880047785818249, 4.967744786903340426 ) ) ;
#8764=CARTESIAN_POINT ( 'NONE',  ( -11.93348319268872615, 410.0573905683720000, 3.332260488124728415 ) ) ;
#8767=CARTESIAN_POINT ( 'NONE',  ( -48.68588794268878672, 502.3073905765656946, 3.978247347593009131 ) ) ;
#8769=CARTESIAN_POINT ( 'NONE',  ( -45.43829269268870519, 335.0573905683720568, -3.332260488124726194 ) ) ;
#8770=CARTESIAN_POINT ( 'NONE',  ( -13.20868407381887266, 459.4948905683720568, -6.410867750099233042 ) ) ;
#8772=CARTESIAN_POINT ( 'NONE',  ( -14.54375231895777887, 470.9948905601784759, 14.14213562373094568 ) ) ;
#8773=CARTESIAN_POINT ( 'NONE',  ( -16.84014894278197616, 277.6198905683720568, 11.84573899990672530 ) ) ;
#8778=CARTESIAN_POINT ( 'NONE',  ( -47.16347859291444422, 336.6198905601784759, -7.653668647301793193 ) ) ;
#8779=CARTESIAN_POINT ( 'NONE',  ( -42.88789093042842637, 304.8073905683720000, 9.489475012073736337 ) ) ;
#8781=CARTESIAN_POINT ( 'NONE',  ( -32.01814843081344719, 387.5573905683719431, 16.75240474999999307 ) ) ;
#8782=CARTESIAN_POINT ( 'NONE',  ( -14.54375231895776110, 293.4948905601785327, -14.14213562373094746 ) ) ;
#8783=CARTESIAN_POINT ( 'NONE',  ( -8.685887942688740537, 516.9948905765655809, -2.449293598294705724E-15 ) ) ;
#8784=CARTESIAN_POINT ( 'NONE',  ( -44.16309181155857999, 403.2448905683720568, -6.410867750099231266 ) ) ;
#8785=CARTESIAN_POINT ( 'NONE',  ( -22.27502019258947641, 262.2448905683720000, -15.47720386886985544 ) ) ;
#8786=CARTESIAN_POINT ( 'NONE',  ( -28.68588794268871922, 416.3698905683720568, 16.75240474999999307 ) ) ;
#8788=CARTESIAN_POINT ( 'NONE',  ( -48.68588794268870856, 372.3073905765656377, 3.978247347593168115 ) ) ;
#8790=CARTESIAN_POINT ( 'NONE',  ( -40.53162694259543741, 335.1198905683720568, 11.84573899990672885 ) ) ;
#8791=CARTESIAN_POINT ( 'NONE',  ( -13.20868407381887444, 480.9948905683720000, -6.410867750099233042 ) ) ;
#8792=EDGE_CURVE ( 'NONE', #13236, #14199, #14024, .T. ) ;
#8796=CARTESIAN_POINT ( 'NONE',  ( -11.93348319268872260, 380.0573905683721136, 3.332260488124728415 ) ) ;
#8798=CARTESIAN_POINT ( 'NONE',  ( -28.68588794268872988, 519.7448905601784190, 19.99999999999999289 ) ) ;
#8799=CARTESIAN_POINT ( 'NONE',  ( -14.48388495494899786, 339.8073905683720568, -9.489475012073736337 ) ) ;
#8801=CARTESIAN_POINT ( 'NONE',  ( -19.19641293061500065, 500.4323905683721136, -14.20200298773971603 ) ) ;
#8803=CARTESIAN_POINT ( 'NONE',  ( -21.03221929538690915, 350.3698905601784759, 18.47759065022572500 ) ) ;
#8807=CARTESIAN_POINT ( 'NONE',  ( -22.27502019258949773, 480.7448905683720568, -15.47720386886985544 ) ) ;
#8808=ORIENTED_EDGE ( 'NONE', *, *, #11864, .F. ) ;
#8809=CARTESIAN_POINT ( 'NONE',  ( -11.93348319268873681, 489.1823905683720568, -3.332260488124732856 ) ) ;
#8811=CARTESIAN_POINT ( 'NONE',  ( -17.35679799567830628, 418.5573905765656377, -16.95518130045146421 ) ) ;
#8812=CARTESIAN_POINT ( 'NONE',  ( -42.82802356641967378, 473.2448905765655809, 14.14213562373094923 ) ) ;
#8814=CARTESIAN_POINT ( 'NONE',  ( -47.16347859291445843, 486.6198905601784759, -7.653668647301793193 ) ) ;
#8815=CARTESIAN_POINT ( 'NONE',  ( -40.01497788969914637, 483.5573905765655809, 16.95518130045146776 ) ) ;
#8816=CARTESIAN_POINT ( 'NONE',  ( -42.82802356641964536, 260.7448905765656377, -14.14213562373094746 ) ) ;
#8819=CARTESIAN_POINT ( 'NONE',  ( -45.43829269268869808, 275.6823905683720568, 3.332260488124734632 ) ) ;
#8821=CARTESIAN_POINT ( 'NONE',  ( -21.03221929538690915, 365.1198905765656377, 18.47759065022572500 ) ) ;
#8822=CARTESIAN_POINT ( 'NONE',  ( -19.19641293061498999, 438.8073905683720000, 14.20200298773971426 ) ) ;
#8824=CARTESIAN_POINT ( 'NONE',  ( -28.68588794268870146, 267.8698905683720000, 16.75240474999999307 ) ) ;
#8826=CARTESIAN_POINT ( 'NONE',  ( -8.685887942688887975, 271.9323905601784759, 3.978247347593586447 ) ) ;
#8827=CARTESIAN_POINT ( 'NONE',  ( -13.20868407381887444, 480.9948905683720000, -6.410867750099233042 ) ) ;
#8829=CARTESIAN_POINT ( 'NONE',  ( -47.16347859291445133, 411.3698905765656377, -7.653668647301793193 ) ) ;
#8830=CARTESIAN_POINT ( 'NONE',  ( -42.88789093042841927, 264.8073905683721136, 9.489475012073736337 ) ) ;
#8833=CARTESIAN_POINT ( 'NONE',  ( -38.17536295476244845, 273.8073905683720000, -14.20200298773971426 ) ) ;
#8834=CARTESIAN_POINT ( 'NONE',  ( -36.33955658999052929, 483.8698905765656377, 18.47759065022572500 ) ) ;
#8836=CARTESIAN_POINT ( 'NONE',  ( -37.54166915975687857, 223.9102039777117454, -14.57737010498150276 ) ) ;
#8837=CARTESIAN_POINT ( 'NONE',  ( -16.84014894278197616, 251.6198905683720284, -11.84573899990672707 ) ) ;
#8838=CARTESIAN_POINT ( 'NONE',  ( -42.88789093042845479, 524.4323905683720568, -9.489475012073736337 ) ) ;
#8839=CARTESIAN_POINT ( 'NONE',  ( -40.01497788969913216, 373.5573905765656377, 16.95518130045146776 ) ) ;
#8840=CARTESIAN_POINT ( 'NONE',  ( -32.01814843081343298, 256.0573905683720000, 16.75240474999999307 ) ) ;
#8841=CARTESIAN_POINT ( 'NONE',  ( -14.48388495494899786, 351.3073905683721136, -9.489475012073736337 ) ) ;
#8842=CARTESIAN_POINT ( 'NONE',  ( -47.16347859291445843, 506.6198905601784190, -7.653668647301793193 ) ) ;
#8844=CARTESIAN_POINT ( 'NONE',  ( -35.09675569278795138, 401.9948905683720568, -15.47720386886985544 ) ) ;
#8846=CARTESIAN_POINT ( 'NONE',  ( -45.64106924314019409, 398.1823905601784759, 11.32908994701042715 ) ) ;
#8848=VERTEX_POINT ( 'NONE', #3185 ) ;
#8849=CARTESIAN_POINT ( 'NONE',  ( -40.01497788969913927, 350.4323905765655809, -16.95518130045146421 ) ) ;
#8850=VERTEX_POINT ( 'NONE', #17989 ) ;
#8851=ORIENTED_EDGE ( 'NONE', *, *, #9944, .F. ) ;
#8852=CARTESIAN_POINT ( 'NONE',  ( -45.43829269268871940, 505.6823905683720568, 3.332260488124734632 ) ) ;
#8853=CARTESIAN_POINT ( 'NONE',  ( -47.16347859291443712, 286.6198905601784759, -7.653668647301793193 ) ) ;
#8854=CARTESIAN_POINT ( 'NONE',  ( -42.82802356641965247, 320.7448905765656377, -14.14213562373094746 ) ) ;
#8856=CARTESIAN_POINT ( 'NONE',  ( -16.84014894278198327, 329.1198905683720568, 11.84573899990672530 ) ) ;
#8857=VERTEX_POINT ( 'NONE', #17882 ) ;
#8858=CARTESIAN_POINT ( 'NONE',  ( -19.19641293061498288, 347.3073905683720568, 14.20200298773971426 ) ) ;
#8859=CARTESIAN_POINT ( 'NONE',  ( -40.53162694259543741, 365.1198905683720000, 11.84573899990672885 ) ) ;
#8861=CARTESIAN_POINT ( 'NONE',  ( -40.01497788969913216, 290.4323905765656377, -16.95518130045146421 ) ) ;
#8862=CARTESIAN_POINT ( 'NONE',  ( -24.70764059509556176, 394.4323905601784190, -19.99999999999999289 ) ) ;
#8863=CARTESIAN_POINT ( 'NONE',  ( -19.19641293061496867, 250.4323905683720284, -14.20200298773971603 ) ) ;
#8864=CARTESIAN_POINT ( 'NONE',  ( -48.68588794268860198, 226.9323905601784759, -3.978247347593371508 ) ) ;
#8865=CARTESIAN_POINT ( 'NONE',  ( -35.09675569278795848, 417.2448905683720568, 15.47720386886985366 ) ) ;
#8868=CARTESIAN_POINT ( 'NONE',  ( -10.20829729246300310, 506.3698905765656946, 7.653668647301790529 ) ) ;
#8869=( BOUNDED_CURVE ( )  B_SPLINE_CURVE ( 2, ( #16793, #4199, #12312, #5813, #18902, #1080, #11801, #13437, #12421, #4087, #19016, #10674, #10785, #18398, #9163, #15787, #975 ),
 .UNSPECIFIED., .F., .T. ) 
 B_SPLINE_CURVE_WITH_KNOTS ( ( 3, 2, 2, 2, 2, 2, 2, 2, 3 ),
 ( 0.5468750000000003331, 0.5488281250000003331, 0.5507812500000002220, 0.5527343750000002220, 0.5546875000000002220, 0.5566406250000002220, 0.5585937500000002220, 0.5605468750000001110, 0.5625000000000001110 ),
 .UNSPECIFIED. ) 
 CURVE ( )  GEOMETRIC_REPRESENTATION_ITEM ( )  RATIONAL_B_SPLINE_CURVE ( ( 0.9999999999999966693, 0.9807852804032337612, 1.000000000000000000, 0.9807852804032304306, 1.000000000000000000, 0.9807852804032304306, 1.000000000000000000, 0.9807852804032304306, 1.000000000000000000, 0.9807852804032304306, 1.000000000000000000, 0.9807852804032304306, 1.000000000000000000, 0.9807852804032304306, 1.000000000000000000, 0.9807852804032293204, 1.000000000000001110 ) ) 
 REPRESENTATION_ITEM ( '' )  );
#8871=CARTESIAN_POINT ( 'NONE',  ( -40.53162694259543031, 324.1198905683720568, -11.84573899990672707 ) ) ;
#8872=CARTESIAN_POINT ( 'NONE',  ( -14.48388495494901029, 459.8073905683720000, -9.489475012073736337 ) ) ;
#8874=CARTESIAN_POINT ( 'NONE',  ( -8.685887942688733432, 462.2448905601784759, -2.449293598294705724E-15 ) ) ;
#8875=CARTESIAN_POINT ( 'NONE',  ( -32.01814843081344009, 281.6823905683720568, -16.75240474999999307 ) ) ;
#8878=CARTESIAN_POINT ( 'NONE',  ( -35.09675569278795848, 453.4948905683720568, -15.47720386886985544 ) ) ;
#8881=CARTESIAN_POINT ( 'NONE',  ( -40.01497788969913927, 345.6823905601784759, -16.95518130045146421 ) ) ;
#8882=CARTESIAN_POINT ( 'NONE',  ( -25.35362745456398414, 291.0573905683720000, -16.75240474999999307 ) ) ;
#8883=ADVANCED_FACE ( 'NONE', ( #3295 ), #58, .T. ) ;
#8884=AXIS2_PLACEMENT_3D ( 'NONE', #16549, #14718, #11448 ) ;
#8885=CARTESIAN_POINT ( 'NONE',  ( -32.01814843081344719, 383.1823905683720000, -16.75240474999999307 ) ) ;
#8886=CARTESIAN_POINT ( 'NONE',  ( -10.20829729246297113, 231.6198905601785043, 7.653668647301790529 ) ) ;
#8887=CARTESIAN_POINT ( 'NONE',  ( -17.35679799567831694, 518.5573905765655809, -16.95518130045146421 ) ) ;
#8888=CARTESIAN_POINT ( 'NONE',  ( -28.68588794268871922, 406.3698905683720000, 16.75240474999999307 ) ) ;
#8889=CARTESIAN_POINT ( 'NONE',  ( -11.93348319268870839, 250.0573905683720000, 3.332260488124728415 ) ) ;
#8890=CARTESIAN_POINT ( 'NONE',  ( -44.16309181155857999, 423.2448905683720568, -6.410867750099231266 ) ) ;
#8892=CARTESIAN_POINT ( 'NONE',  ( -11.73070664223724968, 337.9323905765655809, -11.32908994701042715 ) ) ;
#8894=CARTESIAN_POINT ( 'NONE',  ( -22.27502019258947286, 316.9948905683720568, 15.47720386886985189 ) ) ;
#8895=CARTESIAN_POINT ( 'NONE',  ( -44.16309181155858710, 484.7448905683720568, -6.410867750099231266 ) ) ;
#8897=CARTESIAN_POINT ( 'NONE',  ( -17.35679799567827430, 225.4323905765656093, 16.95518130045146421 ) ) ;
#8899=CARTESIAN_POINT ( 'NONE',  ( -40.53162694259543741, 386.6198905683720568, 11.84573899990672885 ) ) ;
#8901=CARTESIAN_POINT ( 'NONE',  ( -42.82802356641968089, 518.4948905601785327, 14.14213562373094923 ) ) ;
#8902=CARTESIAN_POINT ( 'NONE',  ( -25.35362745456398770, 341.0573905683720000, -16.75240474999999307 ) ) ;
#8904=CARTESIAN_POINT ( 'NONE',  ( -40.53162694259545162, 502.6198905683720568, -11.84573899990672707 ) ) ;
#8906=CARTESIAN_POINT ( 'NONE',  ( -41.29049502611874090, 223.9102039777116033, -11.05440166866015694 ) ) ;
#8908=EDGE_CURVE ( 'NONE', #16932, #1213, #5154, .T. ) ;
#8910=CARTESIAN_POINT ( 'NONE',  ( -40.01497788969916058, 520.4323905765656946, -16.95518130045146421 ) ) ;
#8911=CARTESIAN_POINT ( 'NONE',  ( -11.93348319268873325, 458.5573905683720568, 3.332260488124728415 ) ) ;
#8913=CARTESIAN_POINT ( 'NONE',  ( -42.88789093042844769, 494.8073905683720000, 9.489475012073734561 ) ) ;
#8914=CARTESIAN_POINT ( 'NONE',  ( -8.685887942688708563, 252.2448905601784475, -2.449293598294705724E-15 ) ) ;
#8915=CARTESIAN_POINT ( 'NONE',  ( -48.68588794268871567, 412.3073905765655809, 3.978247347593168115 ) ) ;
#8921=CARTESIAN_POINT ( 'NONE',  ( -21.03221929538693047, 434.1198905601784759, -18.47759065022572855 ) ) ;
#8923=CARTESIAN_POINT ( 'NONE',  ( -11.93348319268871194, 280.0573905683720568, 3.332260488124728415 ) ) ;
#8925=CARTESIAN_POINT ( 'NONE',  ( -45.64106924314017277, 258.1823905601784759, 11.32908994701042715 ) ) ;
#8926=CARTESIAN_POINT ( 'NONE',  ( -28.68588794268872277, 437.8698905683720568, 16.75240474999999307 ) ) ;
#8928=CARTESIAN_POINT ( 'NONE',  ( -14.48388495494898898, 271.3073905683720568, -9.489475012073736337 ) ) ;
#8930=CARTESIAN_POINT ( 'NONE',  ( -48.68588794268861619, 481.6823905765655809, -3.978247347593425243 ) ) ;
#8932=CARTESIAN_POINT ( 'NONE',  ( -14.48388495494901029, 489.4323905683720000, 9.489475012073731008 ) ) ;
#8933=ORIENTED_EDGE ( 'NONE', *, *, #16446, .F. ) ;
#8934=CARTESIAN_POINT ( 'NONE',  ( -28.68588794268874054, 573.2448905601785327, 0.000000000000000000 ) ) ;
#8935=CARTESIAN_POINT ( 'NONE',  ( -19.19641293061496867, 237.3073905683720284, 14.20200298773971426 ) ) ;
#8936=ADVANCED_FACE ( 'NONE', ( #4906 ), #14663, .T. ) ;
#8940=CARTESIAN_POINT ( 'NONE',  ( -48.68588794268872277, 481.9948905765656377, 0.000000000000000000 ) ) ;
#8941=CARTESIAN_POINT ( 'NONE',  ( -48.68588794268870856, 387.2448905601784759, 0.000000000000000000 ) ) ;
#8942=CARTESIAN_POINT ( 'NONE',  ( -19.52302674270934801, 223.9102039777117454, -17.65796940415495087 ) ) ;
#8944=CARTESIAN_POINT ( 'NONE',  ( -11.93348319268874036, 520.3698905683720568, -2.051577885510841163E-15 ) ) ;
#8945=CARTESIAN_POINT ( 'NONE',  ( -8.685887942688724550, 376.9948905765655809, -2.449293598294705724E-15 ) ) ;
#8946=CARTESIAN_POINT ( 'NONE',  ( -45.43829269268869098, 243.5573905683720000, -3.332260488124726194 ) ) ;
#8947=CARTESIAN_POINT ( 'NONE',  ( -13.20868407381885845, 340.9948905683720000, -6.410867750099233042 ) ) ;
#8949=CARTESIAN_POINT ( 'NONE',  ( -28.68588794268870856, 319.7448905601785327, 19.99999999999999289 ) ) ;
#8951=VECTOR ( 'NONE', #17207, 1000.000000000000000 ) ;
#8953=CARTESIAN_POINT ( 'NONE',  ( -44.16309181155857999, 403.2448905683720568, -6.410867750099231266 ) ) ;
#8954=CARTESIAN_POINT ( 'NONE',  ( -42.88789093042845479, 534.4323905683719431, -9.489475012073734561 ) ) ;
#8955=CARTESIAN_POINT ( 'NONE',  ( -36.33955658999051508, 379.1198905601784759, 18.47759065022572500 ) ) ;
#8958=EDGE_LOOP ( 'NONE', ( #15207, #15586 ) ) ;
#8959=ORIENTED_EDGE ( 'NONE', *, *, #12797, .F. ) ;
#8960=CARTESIAN_POINT ( 'NONE',  ( -42.88789093042845479, 506.3073905683720568, 9.489475012073736337 ) ) ;
#8962=ORIENTED_EDGE ( 'NONE', *, *, #662, .T. ) ;
#8964=CARTESIAN_POINT ( 'NONE',  ( -13.20868407381885490, 310.9948905683720568, -6.410867750099233042 ) ) ;
#8966=CARTESIAN_POINT ( 'NONE',  ( -11.93348319268872260, 348.5573905683720000, 3.332260488124728415 ) ) ;
#8967=CARTESIAN_POINT ( 'NONE',  ( -38.17536295476244845, 345.4323905683719431, 14.20200298773971781 ) ) ;
#8968=CARTESIAN_POINT ( 'NONE',  ( -42.82802356641965247, 280.7448905765655809, -14.14213562373094746 ) ) ;
#8970=CARTESIAN_POINT ( 'NONE',  ( -40.53162694259542320, 252.6198905683720284, -11.84573899990672707 ) ) ;
#8972=CARTESIAN_POINT ( 'NONE',  ( -32.01814843081345430, 397.5573905683721136, 16.75240474999999307 ) ) ;
#8974=CARTESIAN_POINT ( 'NONE',  ( -10.20829729246298356, 352.8698905601784759, -7.653668647301794969 ) ) ;
#8977=CARTESIAN_POINT ( 'NONE',  ( -35.09675569278794427, 317.2448905683720000, 15.47720386886985366 ) ) ;
#8978=CARTESIAN_POINT ( 'NONE',  ( -45.43829269268872650, 453.8698905683720000, 0.000000000000000000 ) ) ;
#8980=CARTESIAN_POINT ( 'NONE',  ( -32.66413529028189089, 459.4323905601784759, 19.99999999999999289 ) ) ;
#8981=CARTESIAN_POINT ( 'NONE',  ( -44.16309181155856578, 283.2448905683720568, -6.410867750099231266 ) ) ;
#8988=CARTESIAN_POINT ( 'NONE',  ( -32.01814843081344009, 301.6823905683720568, -16.75240474999999307 ) ) ;
#8989=CARTESIAN_POINT ( 'NONE',  ( -25.35362745456399125, 362.5573905683720568, -16.75240474999999307 ) ) ;
#8991=CARTESIAN_POINT ( 'NONE',  ( -8.685887942688546914, 372.5573905601784190, -3.978247347592740013 ) ) ;
#8992=CARTESIAN_POINT ( 'NONE',  ( -28.68588794268872988, 514.4948905765655809, 19.99999999999999289 ) ) ;
#8993=CARTESIAN_POINT ( 'NONE',  ( -19.19641293061498644, 397.3073905683720000, 14.20200298773971426 ) ) ;
#8994=CARTESIAN_POINT ( 'NONE',  ( -38.17536295476244135, 233.8073905683720284, -14.20200298773971426 ) ) ;
#8995=CARTESIAN_POINT ( 'NONE',  ( -42.88789093042844058, 404.8073905683721136, 9.489475012073734561 ) ) ;
#8997=CARTESIAN_POINT ( 'NONE',  ( -48.68588794268870856, 352.3073905765656377, 3.978247347593168115 ) ) ;
#8999=CARTESIAN_POINT ( 'NONE',  ( -14.48388495494899075, 297.9323905683720000, 9.489475012073731008 ) ) ;
#9000=CARTESIAN_POINT ( 'NONE',  ( -16.84014894278200103, 461.6198905683720568, -11.84573899990672707 ) ) ;
#9001=CARTESIAN_POINT ( 'NONE',  ( -8.685887942688886199, 461.9323905601784190, 3.978247347593533600 ) ) ;
#9004=EDGE_CURVE ( 'NONE', #17095, #19877, #10381, .T. ) ;
#9005=STYLED_ITEM('',(#21442),#12085);
#9006=CARTESIAN_POINT ( 'NONE',  ( -22.27502019258947641, 368.4948905683720568, 15.47720386886985189 ) ) ;
#9007=DIRECTION ( 'NONE',  ( -1.191790137725560488E-16, 1.000000000000000000, -0.000000000000000000 ) ) ;
#9008=CARTESIAN_POINT ( 'NONE',  ( -24.70764059509556887, 520.0573905601784190, 19.99999999999998934 ) ) ;
#9009=CARTESIAN_POINT ( 'NONE',  ( -38.17536295476244845, 335.4323905683720000, 14.20200298773971781 ) ) ;
#9010=ORIENTED_EDGE ( 'NONE', *, *, #12854, .F. ) ;
#9011=CARTESIAN_POINT ( 'NONE',  ( -11.93348319268873858, 509.1823905683719431, -3.332260488124732856 ) ) ;
#9013=CARTESIAN_POINT ( 'NONE',  ( -40.84173908167358036, 223.9102039777116033, -11.54621117671109864 ) ) ;
#9014=CARTESIAN_POINT ( 'NONE',  ( -11.73070664223724080, 316.0573905765655809, 11.32908994701042005 ) ) ;
#9015=B_SPLINE_CURVE_WITH_KNOTS ( 'NONE', 3,
 ( #19976, #8392, #13060, #15124, #306, #5155, #18348, #4826, #19646, #13170 ),
 .UNSPECIFIED., .F., .F.,
 ( 4, 2, 2, 2, 4 ),
 ( 0.5000000000000000000, 0.5416256048145712265, 0.5832512096291423420, 0.6248768144437135685, 0.6665024192582847951 ),
 .UNSPECIFIED. ) ;
#9017=CARTESIAN_POINT ( 'NONE',  ( -17.35679799567831694, 518.5573905765655809, -16.95518130045146421 ) ) ;
#9018=CARTESIAN_POINT ( 'NONE',  ( -40.53162694259545162, 455.1198905683720568, 11.84573899990672885 ) ) ;
#9019=ORIENTED_EDGE ( 'NONE', *, *, #11734, .F. ) ;
#9020=CARTESIAN_POINT ( 'NONE',  ( -28.68588794268872633, 476.3698905683720568, 16.75240474999999307 ) ) ;
#9022=CARTESIAN_POINT ( 'NONE',  ( -45.64106924314019409, 412.9323905765655809, 11.32908994701042715 ) ) ;
#9024=CARTESIAN_POINT ( 'NONE',  ( -24.70764059509554045, 300.0573905601784759, 19.99999999999998934 ) ) ;
#9025=DIRECTION ( 'NONE',  ( -1.000000000000000000, 0.000000000000000000, 0.000000000000000000 ) ) ;
#9026=DIRECTION ( 'NONE',  ( -1.000000000000000000, 0.000000000000000000, 0.000000000000000000 ) ) ;
#9027=CARTESIAN_POINT ( 'NONE',  ( -40.01497788969912506, 260.4323905765656377, -16.95518130045146421 ) ) ;
#9029=CARTESIAN_POINT ( 'NONE',  ( -11.93348319268871371, 280.6823905683720000, -3.332260488124732856 ) ) ;
#9030=EDGE_CURVE ( 'NONE', #3989, #19427, #489, .T. ) ;
#9031=CARTESIAN_POINT ( 'NONE',  ( -40.01497788969911795, 258.8073905601784759, 16.95518130045146776 ) ) ;
#9034=CARTESIAN_POINT ( 'NONE',  ( -14.48388495494900496, 439.4323905683720000, 9.489475012073732785 ) ) ;
#9036=CARTESIAN_POINT ( 'NONE',  ( -38.17536295476243424, 266.9323905683720000, 14.20200298773971781 ) ) ;
#9037=ORIENTED_EDGE ( 'NONE', *, *, #12205, .F. ) ;
#9038=CARTESIAN_POINT ( 'NONE',  ( -10.20829729246299955, 477.6198905765656377, -7.653668647301794969 ) ) ;
#9040=VERTEX_POINT ( 'NONE', #16814 ) ;
#9041=CARTESIAN_POINT ( 'NONE',  ( -28.68588794268872633, 487.8698905683720568, 16.75240474999999307 ) ) ;
#9044=CARTESIAN_POINT ( 'NONE',  ( -14.48388495494898365, 247.9323905683720284, 9.489475012073732785 ) ) ;
#9047=CARTESIAN_POINT ( 'NONE',  ( -28.68588794268872988, 469.4948905765656377, -19.99999999999999289 ) ) ;
#9049=DIRECTION ( 'NONE',  ( -1.191790137725560488E-16, 1.000000000000000000, -0.000000000000000000 ) ) ;
#9050=CARTESIAN_POINT ( 'NONE',  ( -33.72690641870477180, 223.9102039777116886, -17.05470716272690979 ) ) ;
#9052=CARTESIAN_POINT ( 'NONE',  ( -28.68588794268873343, 512.8698905683719431, -16.75240474999999307 ) ) ;
#9053=CARTESIAN_POINT ( 'NONE',  ( -42.82802356641965957, 373.2448905765656377, 14.14213562373094923 ) ) ;
#9055=CARTESIAN_POINT ( 'NONE',  ( -25.35362745456397704, 241.0573905683720284, -16.75240474999999307 ) ) ;
#9057=CARTESIAN_POINT ( 'NONE',  ( -16.84014894278198327, 329.1198905683720568, 11.84573899990672530 ) ) ;
#9058=CARTESIAN_POINT ( 'NONE',  ( -45.64106924314017277, 318.1823905601784759, 11.32908994701042538 ) ) ;
#9059=CARTESIAN_POINT ( 'NONE',  ( -21.03221929538690205, 275.1198905765655809, 18.47759065022572500 ) ) ;
#9060=CARTESIAN_POINT ( 'NONE',  ( -45.43829269268871229, 373.8698905683720000, 0.000000000000000000 ) ) ;
#9061=PLANE ( 'NONE',  #13972 ) ;
#9063=CARTESIAN_POINT ( 'NONE',  ( -8.685887942688726326, 392.2448905601784759, -2.449293598294705724E-15 ) ) ;
#9065=CARTESIAN_POINT ( 'NONE',  ( -36.33955658999050797, 350.1198905765656377, -18.47759065022572855 ) ) ;
#9067=VERTEX_POINT ( 'NONE', #12146 ) ;
#9068=CARTESIAN_POINT ( 'NONE',  ( -38.17536295476246977, 516.9323905683720568, 14.20200298773971781 ) ) ;
#9071=CARTESIAN_POINT ( 'NONE',  ( -16.84014894278197971, 299.1198905683720000, 11.84573899990672530 ) ) ;
#9073=CARTESIAN_POINT ( 'NONE',  ( -25.35362745456397704, 336.6823905683720568, 16.75240474999998952 ) ) ;
#9075=CARTESIAN_POINT ( 'NONE',  ( -11.93348319268872260, 338.5573905683720568, 3.332260488124728859 ) ) ;
#9076=CARTESIAN_POINT ( 'NONE',  ( -10.20829729246297646, 277.6198905765655809, -7.653668647301794969 ) ) ;
#9077=CARTESIAN_POINT ( 'NONE',  ( -42.82802356641966668, 395.9948905601784759, -14.14213562373094746 ) ) ;
#9078=CARTESIAN_POINT ( 'NONE',  ( -13.20868407381884779, 239.4948905683720284, -6.410867750099233042 ) ) ;
#9081=CARTESIAN_POINT ( 'NONE',  ( -45.43829269268871940, 395.3698905683720000, 0.000000000000000000 ) ) ;
#9083=CARTESIAN_POINT ( 'NONE',  ( -8.685887942688738761, 506.9948905765655240, -2.449293598294705724E-15 ) ) ;
#9086=CARTESIAN_POINT ( 'NONE',  ( -11.93348319268872970, 439.1823905683720000, -3.332260488124732856 ) ) ;
#9088=CARTESIAN_POINT ( 'NONE',  ( -28.68588794268872277, 439.7448905601784759, 19.99999999999999289 ) ) ;
#9089=VECTOR ( 'NONE', #16649, 1000.000000000000000 ) ;
#9092=VERTEX_POINT ( 'NONE', #3813 ) ;
#9095=CARTESIAN_POINT ( 'NONE',  ( -10.20829729246298001, 322.8698905601784759, -7.653668647301794969 ) ) ;
#9097=CARTESIAN_POINT ( 'NONE',  ( -16.84014894278198327, 300.1198905683720000, -11.84573899990672707 ) ) ;
#9098=CARTESIAN_POINT ( 'NONE',  ( -13.20868407381886023, 369.7448905683720568, 6.410867750099229490 ) ) ;
#9099=CARTESIAN_POINT ( 'NONE',  ( -48.68588794268871567, 391.9948905765656377, 0.000000000000000000 ) ) ;
#9100=CARTESIAN_POINT ( 'NONE',  ( -16.84014894278199392, 400.1198905683720000, -11.84573899990672707 ) ) ;
#9101=CARTESIAN_POINT ( 'NONE',  ( -28.68588794268869790, 247.8698905683720000, 16.75240474999999307 ) ) ;
#9102=CARTESIAN_POINT ( 'NONE',  ( -45.43829269268871940, 403.5573905683721136, -3.332260488124726638 ) ) ;
#9103=CARTESIAN_POINT ( 'NONE',  ( -47.16347859291444422, 341.3698905765655809, -7.653668647301793193 ) ) ;
#9105=CARTESIAN_POINT ( 'NONE',  ( -40.53162694259543031, 305.1198905683720000, 11.84573899990672885 ) ) ;
#9106=( LENGTH_UNIT ( ) NAMED_UNIT ( * ) SI_UNIT ( .MILLI., .METRE. ) );
#9107=CARTESIAN_POINT ( 'NONE',  ( -44.16309181155857999, 455.9948905683720000, 6.410867750099241924 ) ) ;
#9108=CARTESIAN_POINT ( 'NONE',  ( -42.82802356641968089, 513.2448905765656946, 14.14213562373094923 ) ) ;
#9110=CARTESIAN_POINT ( 'NONE',  ( -8.685887942688733432, 456.9948905765656377, -2.449293598294705724E-15 ) ) ;
#9112=CARTESIAN_POINT ( 'NONE',  ( -16.84014894278198682, 369.1198905683720000, 11.84573899990672530 ) ) ;
#9114=CARTESIAN_POINT ( 'NONE',  ( -17.35679799567831338, 513.8073905601785327, -16.95518130045146421 ) ) ;
#9115=CARTESIAN_POINT ( 'NONE',  ( -40.53162694259543741, 352.6198905683720000, -11.84573899990672707 ) ) ;
#9117=CARTESIAN_POINT ( 'NONE',  ( -13.20868407381887799, 509.4948905683720568, -6.410867750099233042 ) ) ;
#9120=CARTESIAN_POINT ( 'NONE',  ( -13.20868407381886911, 430.9948905683720568, -6.410867750099233042 ) ) ;
#9122=CARTESIAN_POINT ( 'NONE',  ( -10.20829729246300488, 517.6198905765656946, -7.653668647301794969 ) ) ;
#9123=CARTESIAN_POINT ( 'NONE',  ( -42.88789093042844769, 472.9323905683720000, -9.489475012073736337 ) ) ;
#9125=CARTESIAN_POINT ( 'NONE',  ( -35.09675569278796559, 475.7448905683720568, 15.47720386886985366 ) ) ;
#9126=CARTESIAN_POINT ( 'NONE',  ( -21.03221929538689849, 250.3698905601785043, 18.47759065022572500 ) ) ;
#9127=CARTESIAN_POINT ( 'NONE',  ( -24.70764059509555466, 394.8073905765655809, 19.99999999999998934 ) ) ;
#9136=CARTESIAN_POINT ( 'NONE',  ( -42.88789093042842637, 286.3073905683720000, 9.489475012073736337 ) ) ;
#9137=CARTESIAN_POINT ( 'NONE',  ( -36.33955658999050087, 259.1198905601784759, 18.47759065022572500 ) ) ;
#9139=CARTESIAN_POINT ( 'NONE',  ( -19.19641293061498999, 428.8073905683720000, 14.20200298773971426 ) ) ;
#9141=CARTESIAN_POINT ( 'NONE',  ( -16.84014894278197616, 259.1198905683720568, 11.84573899990672530 ) ) ;
#9145=CARTESIAN_POINT ( 'NONE',  ( -32.01814843081345430, 483.1823905683720000, -16.75240474999999307 ) ) ;
#9148=CARTESIAN_POINT ( 'NONE',  ( -25.35362745456397704, 241.0573905683720284, -16.75240474999999307 ) ) ;
#9150=CARTESIAN_POINT ( 'NONE',  ( -38.17536295476247687, 522.3073905683720568, -14.20200298773971426 ) ) ;
#9153=CARTESIAN_POINT ( 'NONE',  ( -45.64106924314020119, 462.9323905765655809, 11.32908994701042715 ) ) ;
#9155=CARTESIAN_POINT ( 'NONE',  ( -28.68588794268870146, 284.4948905765656377, 19.99999999999999289 ) ) ;
#9156=CARTESIAN_POINT ( 'NONE',  ( -14.54375231895778064, 453.4948905601784759, -14.14213562373094746 ) ) ;
#9158=CARTESIAN_POINT ( 'NONE',  ( -16.84014894278200458, 509.1198905683720568, 11.84573899990672530 ) ) ;
#9160=CARTESIAN_POINT ( 'NONE',  ( -40.53162694259542320, 245.1198905683720284, 11.84573899990672885 ) ) ;
#9161=CARTESIAN_POINT ( 'NONE',  ( -28.68588794268871212, 342.8698905683720000, -16.75240474999999307 ) ) ;
#9163=CARTESIAN_POINT ( 'NONE',  ( -47.16347859291444422, 357.8698905601784759, 7.653668647301805628 ) ) ;
#9165=CARTESIAN_POINT ( 'NONE',  ( -13.20868407381886200, 388.2448905683720000, 6.410867750099229490 ) ) ;
#9166=CARTESIAN_POINT ( 'NONE',  ( -44.16309181155859420, 534.7448905683720568, -6.410867750099231266 ) ) ;
#9167=CARTESIAN_POINT ( 'NONE',  ( -8.685887942688724550, 391.9323905601784759, 3.978247347593161010 ) ) ;
#9169=CARTESIAN_POINT ( 'NONE',  ( -17.35679799567828141, 228.5573905765656093, -16.95518130045146421 ) ) ;
#9172=CARTESIAN_POINT ( 'NONE',  ( -45.43829269268872650, 515.0573905683720568, -3.332260488124726194 ) ) ;
#9173=DIRECTION ( 'NONE',  ( -1.191790137725560488E-16, 1.000000000000000000, -0.000000000000000000 ) ) ;
#9174=ORIENTED_EDGE ( 'NONE', *, *, #9004, .T. ) ;
#9176=CARTESIAN_POINT ( 'NONE',  ( -13.20868407381885135, 309.7448905683720568, 6.410867750099229490 ) ) ;
#9178=CARTESIAN_POINT ( 'NONE',  ( -42.88789093042843348, 344.8073905683719431, 9.489475012073736337 ) ) ;
#9179=CARTESIAN_POINT ( 'NONE',  ( -40.53162694259543741, 355.1198905683720568, 11.84573899990672885 ) ) ;
#9180=CARTESIAN_POINT ( 'NONE',  ( -17.35679799567828496, 285.4323905765656377, 16.95518130045146421 ) ) ;
#9181=CARTESIAN_POINT ( 'NONE',  ( -28.68588794268873343, 499.4948905765656377, -19.99999999999999289 ) ) ;
#9182=CARTESIAN_POINT ( 'NONE',  ( -16.84014894278197261, 247.6198905683720284, 11.84573899990672530 ) ) ;
#9183=CARTESIAN_POINT ( 'NONE',  ( -19.81321358049341086, 224.0162454934389586, -17.97266195050653081 ) ) ;
#9184=( BOUNDED_CURVE ( )  B_SPLINE_CURVE ( 2, ( #6498, #6106, #1658, #9356, #12718, #255, #10972, #12614, #13227, #9747, #31, #17965, #11482, #17581, #8227, #21330, #14856 ),
 .UNSPECIFIED., .F., .T. ) 
 B_SPLINE_CURVE_WITH_KNOTS ( ( 3, 2, 2, 2, 2, 2, 2, 2, 3 ),
 ( 0.2656250000000002220, 0.2675781250000002220, 0.2695312500000001665, 0.2714843750000001665, 0.2734375000000001110, 0.2753906250000001110, 0.2773437500000001110, 0.2792968750000000555, 0.2812500000000000555 ),
 .UNSPECIFIED. ) 
 CURVE ( )  GEOMETRIC_REPRESENTATION_ITEM ( )  RATIONAL_B_SPLINE_CURVE ( ( 0.9999999999999977796, 0.9807852804032326510, 1.000000000000000000, 0.9807852804032304306, 1.000000000000000000, 0.9807852804032304306, 1.000000000000000000, 0.9807852804032304306, 1.000000000000000000, 0.9807852804032304306, 1.000000000000000000, 0.9807852804032304306, 1.000000000000000000, 0.9807852804032304306, 1.000000000000000000, 0.9807852804032298755, 1.000000000000000444 ) ) 
 REPRESENTATION_ITEM ( '' )  );
#9185=CARTESIAN_POINT ( 'NONE',  ( -14.48388495494900496, 401.3073905683720568, -9.489475012073736337 ) ) ;
#9189=CARTESIAN_POINT ( 'NONE',  ( -48.68588794268860198, 246.9323905601784475, -3.978247347593371508 ) ) ;
#9190=AXIS2_PLACEMENT_3D ( 'NONE', #19919, #19699, #3480 ) ;
#9191=CARTESIAN_POINT ( 'NONE',  ( -19.19641293061498999, 447.3073905683720568, 14.20200298773971426 ) ) ;
#9192=ORIENTED_EDGE ( 'NONE', *, *, #19162, .T. ) ;
#9193=CARTESIAN_POINT ( 'NONE',  ( -47.16347859291445133, 437.8698905601784759, 7.653668647301805628 ) ) ;
#9198=CARTESIAN_POINT ( 'NONE',  ( -11.73070664223724080, 321.3073905601784759, 11.32908994701042005 ) ) ;
#9199=CARTESIAN_POINT ( 'NONE',  ( -19.19641293061498288, 361.9323905683720568, -14.20200298773971603 ) ) ;
#9202=CARTESIAN_POINT ( 'NONE',  ( -14.54375231895778953, 518.2448905765656946, -14.14213562373094746 ) ) ;
#9203=CARTESIAN_POINT ( 'NONE',  ( -11.93348319268872615, 409.1823905683720568, -3.332260488124732856 ) ) ;
#9204=CARTESIAN_POINT ( 'NONE',  ( -42.88789093042841927, 244.4323905683720284, -9.489475012073736337 ) ) ;
#9206=CARTESIAN_POINT ( 'NONE',  ( -28.68588794268871567, 396.3698905683720000, 16.75240474999999307 ) ) ;
#9210=CARTESIAN_POINT ( 'NONE',  ( -11.73070664223724968, 347.9323905765655809, -11.32908994701042715 ) ) ;
#9212=CARTESIAN_POINT ( 'NONE',  ( -38.17536295476244135, 305.4323905683720000, 14.20200298773971781 ) ) ;
#9213=CARTESIAN_POINT ( 'NONE',  ( -14.48388495494901029, 461.3073905683720568, -9.489475012073736337 ) ) ;
#9219=CARTESIAN_POINT ( 'NONE',  ( -14.48388495494900141, 371.3073905683720568, -9.489475012073736337 ) ) ;
#9220=CARTESIAN_POINT ( 'NONE',  ( -40.53162694259545162, 495.1198905683720000, 11.84573899990672885 ) ) ;
#9221=CARTESIAN_POINT ( 'NONE',  ( -10.20829729246300310, 502.8698905601784759, -7.653668647301794969 ) ) ;
#9222=CARTESIAN_POINT ( 'NONE',  ( -38.17536295476244135, 325.4323905683720000, 14.20200298773971781 ) ) ;
#9226=CARTESIAN_POINT ( 'NONE',  ( -13.20868407381887621, 508.2448905683720568, 6.410867750099229490 ) ) ;
#9230=CARTESIAN_POINT ( 'NONE',  ( -22.27502019258949417, 432.2448905683720000, -15.47720386886985544 ) ) ;
#9233=CARTESIAN_POINT ( 'NONE',  ( -19.19641293061499354, 467.3073905683721136, 14.20200298773971426 ) ) ;
#9235=CARTESIAN_POINT ( 'NONE',  ( -11.93348319268873325, 458.5573905683720568, 3.332260488124728859 ) ) ;
#9236=CARTESIAN_POINT ( 'NONE',  ( -48.68588794268878672, 247.5573905601784759, 3.978247347592954952 ) ) ;
#9239=CARTESIAN_POINT ( 'NONE',  ( -14.54375231895777532, 408.2448905765655809, -14.14213562373094746 ) ) ;
#9244=VECTOR ( 'NONE', #1849, 1000.000000000000000 ) ;
#9247=CARTESIAN_POINT ( 'NONE',  ( -24.70764059509555466, 344.4323905601784759, -19.99999999999999289 ) ) ;
#9248=CARTESIAN_POINT ( 'NONE',  ( -17.35679799567828496, 253.8073905601785043, -16.95518130045146421 ) ) ;
#9249=CARTESIAN_POINT ( 'NONE',  ( -28.68588794268871922, 404.4948905765656377, 19.99999999999999289 ) ) ;
#9250=CARTESIAN_POINT ( 'NONE',  ( -28.68588794268871922, 427.8698905683720568, 16.75240474999999307 ) ) ;
#9252=CARTESIAN_POINT ( 'NONE',  ( -35.09675569278793716, 247.2448905683720000, 15.47720386886985366 ) ) ;
#9255=DIRECTION ( 'NONE',  ( -1.191790137725560488E-16, 1.000000000000000000, -0.000000000000000000 ) ) ;
#9256=ORIENTED_EDGE ( 'NONE', *, *, #20274, .T. ) ;
#9257=CARTESIAN_POINT ( 'NONE',  ( -11.93348319268873325, 460.6823905683720568, -3.332260488124732856 ) ) ;
#9260=CARTESIAN_POINT ( 'NONE',  ( -35.09675569278793006, 231.9948905683720284, -15.47720386886985544 ) ) ;
#9261=VERTEX_POINT ( 'NONE', #19065 ) ;
#9262=CARTESIAN_POINT ( 'NONE',  ( -11.93348319268874036, 518.5573905683720568, 3.332260488124728859 ) ) ;
#9264=CARTESIAN_POINT ( 'NONE',  ( -32.66413529028189089, 464.1823905765656377, 19.99999999999999289 ) ) ;
#9266=CYLINDRICAL_SURFACE ( 'NONE', #9424, 19.99999999999999645 ) ;
#9270=CARTESIAN_POINT ( 'NONE',  ( -11.93348319268873858, 510.6823905683720000, -3.332260488124732856 ) ) ;
#9271=CARTESIAN_POINT ( 'NONE',  ( -13.68588794268869435, 193.9102039777116602, 1.836970198721029983E-15 ) ) ;
#9272=CARTESIAN_POINT ( 'NONE',  ( -28.68588794268870146, 231.3698905683720284, -16.75240474999999307 ) ) ;
#9273=CARTESIAN_POINT ( 'NONE',  ( -16.84014894278198327, 339.1198905683720568, 11.84573899990672530 ) ) ;
#9274=CARTESIAN_POINT ( 'NONE',  ( -17.35679799567830273, 470.6823905601784759, 16.95518130045146421 ) ) ;
#9277=CARTESIAN_POINT ( 'NONE',  ( -35.09675569278794427, 381.9948905683720568, -15.47720386886985544 ) ) ;
#9278=CARTESIAN_POINT ( 'NONE',  ( -47.06209031768872819, 536.3073905642752379, 0.000000000000000000 ) ) ;
#9279=CARTESIAN_POINT ( 'NONE',  ( -10.20829729246298889, 391.6198905601784759, 7.653668647301790529 ) ) ;
#9284=CARTESIAN_POINT ( 'NONE',  ( -42.88789093042845479, 514.4323905683720568, -9.489475012073736337 ) ) ;
#9287=CARTESIAN_POINT ( 'NONE',  ( -44.16309181155856578, 294.7448905683720568, -6.410867750099231266 ) ) ;
#9289=CARTESIAN_POINT ( 'NONE',  ( -42.88789093042842637, 324.8073905683720000, 9.489475012073736337 ) ) ;
#9291=CARTESIAN_POINT ( 'NONE',  ( -47.16347859291443712, 272.6198905765655809, 7.653668647301805628 ) ) ;
#9293=CARTESIAN_POINT ( 'NONE',  ( -11.93348319268870661, 248.5573905683719715, 3.332260488124728859 ) ) ;
#9295=CARTESIAN_POINT ( 'NONE',  ( -13.20868407381886378, 390.9948905683720568, -6.410867750099233042 ) ) ;
#9300=EDGE_CURVE ( 'NONE', #7992, #13900, #6529, .T. ) ;
#9301=CARTESIAN_POINT ( 'NONE',  ( -38.17536295476245556, 445.4323905683720568, 14.20200298773971781 ) ) ;
#9303=CARTESIAN_POINT ( 'NONE',  ( -47.16347859291445843, 456.6198905601784759, -7.653668647301793193 ) ) ;
#9305=ORIENTED_EDGE ( 'NONE', *, *, #12363, .T. ) ;
#9307=CARTESIAN_POINT ( 'NONE',  ( -48.68588794268870146, 317.5573905601784759, 3.978247347593168115 ) ) ;
#9309=CARTESIAN_POINT ( 'NONE',  ( -45.43829269268871229, 365.0573905683720568, -3.332260488124726638 ) ) ;
#9311=CARTESIAN_POINT ( 'NONE',  ( -8.685887942688738761, 496.9948905765655809, -2.449293598294705724E-15 ) ) ;
#9312=CARTESIAN_POINT ( 'NONE',  ( -13.20868407381886378, 389.4948905683720000, -6.410867750099233042 ) ) ;
#9313=CARTESIAN_POINT ( 'NONE',  ( -22.27502019258947286, 242.2448905683720000, -15.47720386886985544 ) ) ;
#9314=CARTESIAN_POINT ( 'NONE',  ( -13.20868407381886556, 409.4948905683720000, -6.410867750099233042 ) ) ;
#9315=( BOUNDED_CURVE ( )  B_SPLINE_CURVE ( 2, ( #12304, #5915, #10560, #18894, #2576, #1073, #12413, #4080, #20854, #19006, #10666, #2683, #9156, #12526, #15779, #13828, #17285 ),
 .UNSPECIFIED., .F., .T. ) 
 B_SPLINE_CURVE_WITH_KNOTS ( ( 3, 2, 2, 2, 2, 2, 2, 2, 3 ),
 ( 0.2500000000000002220, 0.2519531250000002220, 0.2539062500000002220, 0.2558593750000002220, 0.2578125000000002220, 0.2597656250000002220, 0.2617187500000002220, 0.2636718750000002220, 0.2656250000000002220 ),
 .UNSPECIFIED. ) 
 CURVE ( )  GEOMETRIC_REPRESENTATION_ITEM ( )  RATIONAL_B_SPLINE_CURVE ( ( 0.9999999999999977796, 0.9807852804032326510, 1.000000000000000000, 0.9807852804032304306, 1.000000000000000000, 0.9807852804032304306, 1.000000000000000000, 0.9807852804032304306, 1.000000000000000000, 0.9807852804032304306, 1.000000000000000000, 0.9807852804032304306, 1.000000000000000000, 0.9807852804032304306, 1.000000000000000000, 0.9807852804032282101, 1.000000000000002220 ) ) 
 REPRESENTATION_ITEM ( '' )  );
#9316=CARTESIAN_POINT ( 'NONE',  ( -24.70764059509554755, 334.8073905765656377, 19.99999999999998934 ) ) ;
#9318=CARTESIAN_POINT ( 'NONE',  ( -13.20868407381885135, 308.2448905683720000, 6.410867750099229490 ) ) ;
#9320=CARTESIAN_POINT ( 'NONE',  ( -14.48388495494900852, 451.3073905683721136, -9.489475012073736337 ) ) ;
#9324=CARTESIAN_POINT ( 'NONE',  ( -45.43829269268871229, 365.3698905683720568, 0.000000000000000000 ) ) ;
#9325=CARTESIAN_POINT ( 'NONE',  ( -19.19641293061500065, 500.4323905683721136, -14.20200298773971603 ) ) ;
#9326=CARTESIAN_POINT ( 'NONE',  ( -8.685887942688740537, 502.5573905601785896, -3.978247347593165895 ) ) ;
#9327=CARTESIAN_POINT ( 'NONE',  ( -25.35362745456398770, 321.0573905683720568, -16.75240474999999307 ) ) ;
#9329=CARTESIAN_POINT ( 'NONE',  ( -47.16347859291446554, 526.6198905601784190, -7.653668647301793193 ) ) ;
#9330=ORIENTED_EDGE ( 'NONE', *, *, #14142, .F. ) ;
#9332=CARTESIAN_POINT ( 'NONE',  ( -38.17536295476246266, 423.8073905683720568, -14.20200298773971426 ) ) ;
#9335=CARTESIAN_POINT ( 'NONE',  ( -22.27502019258948707, 436.9948905683720568, 15.47720386886985189 ) ) ;
#9337=CARTESIAN_POINT ( 'NONE',  ( -22.27502019258949773, 470.7448905683720568, -15.47720386886985544 ) ) ;
#9342=CARTESIAN_POINT ( 'NONE',  ( -8.685887942688726326, 397.3073905765656946, -3.978247347593165895 ) ) ;
#9343=CARTESIAN_POINT ( 'NONE',  ( -14.54375231895776110, 278.2448905765655809, -14.14213562373094746 ) ) ;
#9346=CARTESIAN_POINT ( 'NONE',  ( -48.68588794268871567, 441.9948905765656377, 0.000000000000000000 ) ) ;
#9353=CARTESIAN_POINT ( 'NONE',  ( -38.88879370254166190, 223.9102039777117170, 16.61907291475590043 ) ) ;
#9355=CARTESIAN_POINT ( 'NONE',  ( -10.20829729246297291, 241.6198905601784759, 7.653668647301790529 ) ) ;
#9356=CARTESIAN_POINT ( 'NONE',  ( -11.73070664223725679, 451.3073905601784759, 11.32908994701042005 ) ) ;
#9357=CARTESIAN_POINT ( 'NONE',  ( -28.68588794268872277, 422.8698905683720568, -16.75240474999999307 ) ) ;
#9360=CARTESIAN_POINT ( 'NONE',  ( -16.84014894278197261, 249.1198905683720284, 11.84573899990672530 ) ) ;
#9362=ORIENTED_EDGE ( 'NONE', *, *, #4137, .F. ) ;
#9363=ORIENTED_EDGE ( 'NONE', *, *, #5300, .T. ) ;
#9364=CARTESIAN_POINT ( 'NONE',  ( -40.01497788969915348, 480.4323905765656377, -16.95518130045146421 ) ) ;
#9365=ORIENTED_EDGE ( 'NONE', *, *, #15650, .T. ) ;
#9366=CARTESIAN_POINT ( 'NONE',  ( -35.09675569278796559, 467.2448905683720568, 15.47720386886985366 ) ) ;
#9367=CARTESIAN_POINT ( 'NONE',  ( -24.70764059509554755, 229.1823905765656377, -19.99999999999999289 ) ) ;
#9368=VECTOR ( 'NONE', #2876, 1000.000000000000000 ) ;
#9371=CARTESIAN_POINT ( 'NONE',  ( -8.685887942688722774, 362.2448905601784190, -2.449293598294705724E-15 ) ) ;
#9373=CARTESIAN_POINT ( 'NONE',  ( -19.19641293061499709, 517.3073905683720568, 14.20200298773971426 ) ) ;
#9374=DIRECTION ( 'NONE',  ( -1.191790137725560488E-16, 1.000000000000000000, -0.000000000000000000 ) ) ;
#9375=CARTESIAN_POINT ( 'NONE',  ( -17.35679799567830983, 458.5573905765656377, -16.95518130045146421 ) ) ;
#9380=CARTESIAN_POINT ( 'NONE',  ( -11.73821085826490851, 223.9102039777117739, 10.74164566205277715 ) ) ;
#9381=CARTESIAN_POINT ( 'NONE',  ( -13.20868407381884424, 228.2448905683720568, 6.410867750099229490 ) ) ;
#9382=CARTESIAN_POINT ( 'NONE',  ( -38.17536295476244845, 313.8073905683720000, -14.20200298773971426 ) ) ;
#9386=CARTESIAN_POINT ( 'NONE',  ( -28.68588794268870856, 317.8698905683720000, 16.75240474999999307 ) ) ;
#9387=CARTESIAN_POINT ( 'NONE',  ( -42.88789093042843348, 374.8073905683720568, 9.489475012073736337 ) ) ;
#9388=CARTESIAN_POINT ( 'NONE',  ( -14.48388495494901740, 529.4323905683720568, 9.489475012073731008 ) ) ;
#9389=CARTESIAN_POINT ( 'NONE',  ( -32.66413529028188378, 395.0573905601784190, -19.99999999999999289 ) ) ;
#9393=CARTESIAN_POINT ( 'NONE',  ( -42.88789093042844769, 496.3073905683720568, 9.489475012073736337 ) ) ;
#9396=CARTESIAN_POINT ( 'NONE',  ( -45.43829269268870519, 295.0573905683720000, -3.332260488124726638 ) ) ;
#9397=CARTESIAN_POINT ( 'NONE',  ( -32.01814843081344009, 321.6823905683720568, -16.75240474999999307 ) ) ;
#9400=CARTESIAN_POINT ( 'NONE',  ( -11.73070664223723547, 266.0573905765655809, 11.32908994701042005 ) ) ;
#9403=CARTESIAN_POINT ( 'NONE',  ( -40.53162694259544452, 394.1198905683720000, -11.84573899990672707 ) ) ;
#9404=DIRECTION ( 'NONE',  ( -1.000000000000000000, 0.000000000000000000, 0.000000000000000000 ) ) ;
#9405=CARTESIAN_POINT ( 'NONE',  ( -28.68588794268874054, 573.2448905601785327, 0.000000000000000000 ) ) ;
#9409=CARTESIAN_POINT ( 'NONE',  ( -11.73070664223723547, 243.1823905601784759, -11.32908994701042538 ) ) ;
#9410=CARTESIAN_POINT ( 'NONE',  ( -16.84014894278199748, 447.6198905683720568, 11.84573899990672530 ) ) ;
#9413=CARTESIAN_POINT ( 'NONE',  ( -11.73070664223725679, 451.3073905601785327, 11.32908994701042005 ) ) ;
#9414=ORIENTED_EDGE ( 'NONE', *, *, #16475, .T. ) ;
#9416=EDGE_LOOP ( 'NONE', ( #17216, #3491, #18222, #8373 ) ) ;
#9417=CARTESIAN_POINT ( 'NONE',  ( -21.03221929538690560, 320.3698905601785327, 18.47759065022572500 ) ) ;
#9419=CARTESIAN_POINT ( 'NONE',  ( -45.43829269268871229, 355.0573905683720568, -3.332260488124726638 ) ) ;
#9420=DIRECTION ( 'NONE',  ( 1.000000000000000000, 0.000000000000000000, 0.000000000000000000 ) ) ;
#9421=CARTESIAN_POINT ( 'NONE',  ( -11.73070664223726389, 506.0573905765656377, 11.32908994701042005 ) ) ;
#9422=CARTESIAN_POINT ( 'NONE',  ( -14.48388495494900141, 379.8073905683720568, -9.489475012073736337 ) ) ;
#9424=AXIS2_PLACEMENT_3D ( 'NONE', #4617, #3000, #2901 ) ;
#9425=CARTESIAN_POINT ( 'NONE',  ( -11.93348319268872615, 399.1823905683720568, -3.332260488124732856 ) ) ;
#9427=CARTESIAN_POINT ( 'NONE',  ( -45.64106924314018698, 331.0573905765655809, -11.32908994701042715 ) ) ;
#9429=CARTESIAN_POINT ( 'NONE',  ( -13.20868407381885490, 309.4948905683720568, -6.410867750099233042 ) ) ;
#9430=CARTESIAN_POINT ( 'NONE',  ( -25.35362745456399125, 448.1823905683719431, 16.75240474999998952 ) ) ;
#9434=CARTESIAN_POINT ( 'NONE',  ( -35.09675569278795138, 377.2448905683720000, 15.47720386886985366 ) ) ;
#9435=CARTESIAN_POINT ( 'NONE',  ( -14.48388495494901740, 499.8073905683720568, -9.489475012073736337 ) ) ;
#9437=CARTESIAN_POINT ( 'NONE',  ( -48.68588794268872277, 496.9323905601784759, -3.978247347593158345 ) ) ;
#9438=CARTESIAN_POINT ( 'NONE',  ( -11.93348319268871727, 319.1823905683720568, -3.332260488124732856 ) ) ;
#9439=EDGE_CURVE ( 'NONE', #10338, #2613, #17725, .T. ) ;
#9443=( BOUNDED_CURVE ( )  B_SPLINE_CURVE ( 2, ( #1950, #10146, #6894, #11982, #539, #8733, #15358, #7106, #13726, #20316, #18147, #16544, #1729, #1319, #17145, #5556, #9519 ),
 .UNSPECIFIED., .F., .T. ) 
 B_SPLINE_CURVE_WITH_KNOTS ( ( 3, 2, 2, 2, 2, 2, 2, 2, 3 ),
 ( 0.3437500000000001110, 0.3457031250000001110, 0.3476562500000001110, 0.3496093750000001110, 0.3515625000000001110, 0.3535156250000001110, 0.3554687500000001110, 0.3574218750000001110, 0.3593750000000001110 ),
 .UNSPECIFIED. ) 
 CURVE ( )  GEOMETRIC_REPRESENTATION_ITEM ( )  RATIONAL_B_SPLINE_CURVE ( ( 0.9999999999999988898, 0.9807852804032315408, 1.000000000000000000, 0.9807852804032304306, 1.000000000000000000, 0.9807852804032304306, 1.000000000000000000, 0.9807852804032304306, 1.000000000000000000, 0.9807852804032304306, 1.000000000000000000, 0.9807852804032304306, 1.000000000000000000, 0.9807852804032304306, 1.000000000000000000, 0.9807852804032293204, 1.000000000000001110 ) ) 
 REPRESENTATION_ITEM ( '' )  );
#9445=CARTESIAN_POINT ( 'NONE',  ( -45.43829269268871940, 415.6823905683720568, 3.332260488124734632 ) ) ;
#9447=CARTESIAN_POINT ( 'NONE',  ( -35.09675569278795848, 451.9948905683720000, -15.47720386886985544 ) ) ;
#9449=CARTESIAN_POINT ( 'NONE',  ( -16.84014894278199748, 457.6198905683720568, 11.84573899990672530 ) ) ;
#9451=CARTESIAN_POINT ( 'NONE',  ( -24.70764059509556532, 414.4323905601784759, -19.99999999999999289 ) ) ;
#9454=CARTESIAN_POINT ( 'NONE',  ( -48.68588794268870856, 382.3073905765656377, 3.978247347593168115 ) ) ;
#9455=CARTESIAN_POINT ( 'NONE',  ( -48.68588794268860909, 281.6823905765656377, -3.978247347593371508 ) ) ;
#9456=DIRECTION ( 'NONE',  ( -1.191790137725560488E-16, 1.000000000000000000, -0.000000000000000000 ) ) ;
#9461=CARTESIAN_POINT ( 'NONE',  ( -11.73070664223723547, 253.1823905601785043, -11.32908994701042538 ) ) ;
#9463=CARTESIAN_POINT ( 'NONE',  ( -16.84014894278199748, 431.6198905683720000, -11.84573899990672707 ) ) ;
#9465=CARTESIAN_POINT ( 'NONE',  ( -28.68588794268870146, 242.8698905683720568, -16.75240474999999307 ) ) ;
#9466=ORIENTED_EDGE ( 'NONE', *, *, #16976, .T. ) ;
#9470=CARTESIAN_POINT ( 'NONE',  ( -42.88789093042844769, 456.3073905683720000, 9.489475012073734561 ) ) ;
#9471=CARTESIAN_POINT ( 'NONE',  ( -24.70764059509554045, 219.1823905765656377, -19.99999999999999289 ) ) ;
#9473=ORIENTED_EDGE ( 'NONE', *, *, #6048, .F. ) ;
#9475=CARTESIAN_POINT ( 'NONE',  ( -14.48388495494898365, 229.8073905683720000, -9.489475012073736337 ) ) ;
#9477=CARTESIAN_POINT ( 'NONE',  ( -35.09675569278796559, 531.9948905683720568, -15.47720386886985544 ) ) ;
#9479=CARTESIAN_POINT ( 'NONE',  ( -32.66413529028188378, 439.8073905765656946, -19.99999999999999289 ) ) ;
#9482=CARTESIAN_POINT ( 'NONE',  ( -32.66413529028185536, 239.8073905765656377, -19.99999999999999289 ) ) ;
#9483=ADVANCED_FACE ( 'NONE', ( #3050 ), #21111, .T. ) ;
#9484=CARTESIAN_POINT ( 'NONE',  ( -14.54375231895775755, 290.9948905601784759, 14.14213562373094568 ) ) ;
#9486=CARTESIAN_POINT ( 'NONE',  ( -8.685887942688713892, 223.9102039777116886, 2.449293598294704541E-15 ) ) ;
#9487=CARTESIAN_POINT ( 'NONE',  ( -32.01814843081343298, 221.6823905683720000, -16.75240474999999307 ) ) ;
#9488=CARTESIAN_POINT ( 'NONE',  ( -14.48388495494899431, 321.3073905683720000, -9.489475012073736337 ) ) ;
#9489=CARTESIAN_POINT ( 'NONE',  ( -13.68588794268873698, 548.2448905601784190, 0.000000000000000000 ) ) ;
#9490=CARTESIAN_POINT ( 'NONE',  ( -45.64106924314017988, 378.1823905601785327, 11.32908994701042538 ) ) ;
#9491=CARTESIAN_POINT ( 'NONE',  ( -25.35362745456397349, 308.1823905683719431, 16.75240474999998952 ) ) ;
#9492=CARTESIAN_POINT ( 'NONE',  ( -16.84014894278199037, 387.6198905683720568, 11.84573899990672530 ) ) ;
#9493=CARTESIAN_POINT ( 'NONE',  ( -13.20868407381887977, 520.9948905683720568, -6.410867750099233042 ) ) ;
#9494=CARTESIAN_POINT ( 'NONE',  ( -21.03221929538690915, 360.3698905601784759, 18.47759065022572500 ) ) ;
#9495=CARTESIAN_POINT ( 'NONE',  ( -42.82802356641966668, 405.9948905601785327, -14.14213562373094746 ) ) ;
#9497=CARTESIAN_POINT ( 'NONE',  ( -35.09675569278795848, 483.4948905683720000, -15.47720386886985544 ) ) ;
#9499=CARTESIAN_POINT ( 'NONE',  ( -32.01814843081344009, 286.0573905683720568, 16.75240474999999307 ) ) ;
#9501=CARTESIAN_POINT ( 'NONE',  ( -13.20868407381885135, 290.9948905683720000, -6.410867750099233042 ) ) ;
#9502=CARTESIAN_POINT ( 'NONE',  ( -32.01814843081344719, 331.6823905683720000, -16.75240474999999307 ) ) ;
#9503=CARTESIAN_POINT ( 'NONE',  ( -8.685887942688710339, 256.6823905765656377, 3.978247347593161010 ) ) ;
#9504=CARTESIAN_POINT ( 'NONE',  ( -8.685887942688726326, 392.2448905601784759, -2.449293598294705724E-15 ) ) ;
#9505=CARTESIAN_POINT ( 'NONE',  ( -25.35362745456396283, 226.6823905683720284, 16.75240474999998952 ) ) ;
#9506=CARTESIAN_POINT ( 'NONE',  ( -14.48388495494899963, 379.4323905683721136, 9.489475012073732785 ) ) ;
#9508=CARTESIAN_POINT ( 'NONE',  ( -8.685887942688736985, 492.2448905601785327, -2.449293598294705724E-15 ) ) ;
#9509=CARTESIAN_POINT ( 'NONE',  ( -36.33955658999052929, 510.1198905765655809, -18.47759065022572855 ) ) ;
#9510=CARTESIAN_POINT ( 'NONE',  ( -25.35362745456400191, 451.0573905683719431, -16.75240474999999307 ) ) ;
#9513=CARTESIAN_POINT ( 'NONE',  ( -14.54375231895777532, 430.9948905601784759, 14.14213562373094568 ) ) ;
#9517=CARTESIAN_POINT ( 'NONE',  ( -47.16347859291444422, 352.6198905765656377, 7.653668647301805628 ) ) ;
#9518=CARTESIAN_POINT ( 'NONE',  ( -24.70764059509554755, 320.0573905601784759, 19.99999999999998934 ) ) ;
#9519=CARTESIAN_POINT ( 'NONE',  ( -8.685887942688728103, 416.9948905765656377, -2.449293598294705724E-15 ) ) ;
#9520=CARTESIAN_POINT ( 'NONE',  ( -45.43829269268871229, 345.3698905683720568, 0.000000000000000000 ) ) ;
#9521=CYLINDRICAL_SURFACE ( 'NONE', #1433, 19.99999999999999645 ) ;
#9522=CARTESIAN_POINT ( 'NONE',  ( -24.70764059509556887, 504.8073905765656377, 19.99999999999998934 ) ) ;
#9523=CARTESIAN_POINT ( 'NONE',  ( -19.19641293061498999, 390.4323905683720568, -14.20200298773971603 ) ) ;
#9524=CARTESIAN_POINT ( 'NONE',  ( -42.88789093042841927, 224.4323905683720000, -9.489475012073736337 ) ) ;
#9525=CARTESIAN_POINT ( 'NONE',  ( -19.19641293061498644, 390.4323905683721136, -14.20200298773971603 ) ) ;
#9526=CARTESIAN_POINT ( 'NONE',  ( -10.20829729246298179, 327.6198905765656377, -7.653668647301794969 ) ) ;
#9527=CARTESIAN_POINT ( 'NONE',  ( -32.66413529028187668, 425.0573905601784759, -19.99999999999999289 ) ) ;
#9528=CARTESIAN_POINT ( 'NONE',  ( -16.84014894278197971, 287.6198905683720000, 11.84573899990672530 ) ) ;
#9530=CARTESIAN_POINT ( 'NONE',  ( -11.93348319268872970, 440.6823905683721136, -3.332260488124732856 ) ) ;
#9531=CARTESIAN_POINT ( 'NONE',  ( -28.68588794268870501, 284.7448905601784759, -19.99999999999999289 ) ) ;
#9532=CARTESIAN_POINT ( 'NONE',  ( -24.70764059509554755, 370.0573905601783622, 19.99999999999998934 ) ) ;
#9534=CARTESIAN_POINT ( 'NONE',  ( -28.68588794268871212, 347.8698905683720568, 16.75240474999999307 ) ) ;
#9535=CARTESIAN_POINT ( 'NONE',  ( -28.68588794268872988, 496.3698905683720568, 16.75240474999999307 ) ) ;
#9536=CARTESIAN_POINT ( 'NONE',  ( -24.70764059509557953, 514.4323905601785327, -19.99999999999999289 ) ) ;
#9537=CARTESIAN_POINT ( 'NONE',  ( -40.53162694259543741, 332.6198905683720000, -11.84573899990672707 ) ) ;
#9546=CARTESIAN_POINT ( 'NONE',  ( -44.16309181155857289, 415.9948905683720000, 6.410867750099241924 ) ) ;
#9547=CYLINDRICAL_SURFACE ( 'NONE', #15931, 5.000000000000001776 ) ;
#9548=CARTESIAN_POINT ( 'NONE',  ( -42.88789093042844058, 434.8073905683720568, 9.489475012073736337 ) ) ;
#9550=CARTESIAN_POINT ( 'NONE',  ( -19.19641293061499709, 470.4323905683719431, -14.20200298773971603 ) ) ;
#9553=CARTESIAN_POINT ( 'NONE',  ( -32.66413529028187668, 384.1823905765655809, 19.99999999999999289 ) ) ;
#9557=CARTESIAN_POINT ( 'NONE',  ( -11.73070664223723369, 256.0573905765656377, 11.32908994701042005 ) ) ;
#9562=CARTESIAN_POINT ( 'NONE',  ( -8.685887942688543362, 342.5573905601784190, -3.978247347592740013 ) ) ;
#9564=CARTESIAN_POINT ( 'NONE',  ( -44.16309181155857289, 425.9948905683720568, 6.410867750099241924 ) ) ;
#9566=( BOUNDED_CURVE ( )  B_SPLINE_CURVE ( 2, ( #5439, #12153, #15625, #18630, #812, #8897, #2107, #10410, #594, #17137, #12039 ),
 .UNSPECIFIED., .F., .T. ) 
 B_SPLINE_CURVE_WITH_KNOTS ( ( 3, 2, 2, 2, 2, 3 ),
 ( 0.9531250000000001110, 0.9550781250000001110, 0.9570312500000001110, 0.9589843750000000000, 0.9609375000000000000, 0.9627616638092109103 ),
 .UNSPECIFIED. ) 
 CURVE ( )  GEOMETRIC_REPRESENTATION_ITEM ( )  RATIONAL_B_SPLINE_CURVE ( ( 0.9999999999999988898, 0.9807852804032315408, 1.000000000000000000, 0.9807852804032304306, 1.000000000000000000, 0.9807852804032304306, 1.000000000000000000, 0.9807852804032304306, 1.000000000000000000, 0.9820539924006078669, 0.9976301173658341792 ) ) 
 REPRESENTATION_ITEM ( '' )  );
#9567=CARTESIAN_POINT ( 'NONE',  ( -22.27502019258947286, 252.2448905683720284, -15.47720386886985544 ) ) ;
#9571=ORIENTED_EDGE ( 'NONE', *, *, #12310, .F. ) ;
#9572=CARTESIAN_POINT ( 'NONE',  ( -32.01814843081345430, 463.1823905683720000, -16.75240474999999307 ) ) ;
#9573=CARTESIAN_POINT ( 'NONE',  ( -40.01497788969912506, 220.4323905765656093, -16.95518130045146421 ) ) ;
#9577=CARTESIAN_POINT ( 'NONE',  ( -20.29730442459490547, 220.5357903062123626, -14.50085278415678403 ) ) ;
#9578=ORIENTED_EDGE ( 'NONE', *, *, #13647, .F. ) ;
#9579=CARTESIAN_POINT ( 'NONE',  ( -42.88789093042845479, 532.9323905683720568, -9.489475012073734561 ) ) ;
#9582=CARTESIAN_POINT ( 'NONE',  ( -36.33955658999052218, 443.8698905765656377, 18.47759065022572500 ) ) ;
#9585=CARTESIAN_POINT ( 'NONE',  ( -14.48388495494899786, 339.8073905683720000, -9.489475012073734561 ) ) ;
#9588=CARTESIAN_POINT ( 'NONE',  ( -40.01497788969912506, 288.8073905601785327, 16.95518130045146776 ) ) ;
#9590=CARTESIAN_POINT ( 'NONE',  ( -42.88789093042841927, 232.9323905683720000, -9.489475012073736337 ) ) ;
#9591=CARTESIAN_POINT ( 'NONE',  ( -25.35362745456397349, 308.1823905683719431, 16.75240474999998952 ) ) ;
#9594=CARTESIAN_POINT ( 'NONE',  ( -14.48388495494899075, 309.4323905683720568, 9.489475012073732785 ) ) ;
#9595=CARTESIAN_POINT ( 'NONE',  ( -14.48388495494900141, 369.8073905683720000, -9.489475012073736337 ) ) ;
#9596=CARTESIAN_POINT ( 'NONE',  ( -25.35362745456399836, 518.1823905683720568, 16.75240474999998952 ) ) ;
#9597=CARTESIAN_POINT ( 'NONE',  ( -8.685887942688724550, 372.2448905601784759, -2.449293598294705724E-15 ) ) ;
#9600=CARTESIAN_POINT ( 'NONE',  ( -19.19641293061499709, 481.9323905683720000, -14.20200298773971603 ) ) ;
#9601=DIRECTION ( 'NONE',  ( -1.000000000000000000, 0.000000000000000000, 0.000000000000000000 ) ) ;
#9602=CARTESIAN_POINT ( 'NONE',  ( -13.20868407381885135, 279.4948905683720000, -6.410867750099233042 ) ) ;
#9604=CARTESIAN_POINT ( 'NONE',  ( -25.35362745456396993, 278.1823905683720000, 16.75240474999998952 ) ) ;
#9605=CARTESIAN_POINT ( 'NONE',  ( -19.19641293061498288, 320.4323905683720568, -14.20200298773971603 ) ) ;
#9606=CARTESIAN_POINT ( 'NONE',  ( -22.27502019258946220, 258.4948905683720568, 15.47720386886985189 ) ) ;
#9608=CARTESIAN_POINT ( 'NONE',  ( -28.68588794268869790, 254.4948905765656093, 19.99999999999999289 ) ) ;
#9610=CARTESIAN_POINT ( 'NONE',  ( -32.01814843081343298, 236.0573905683720568, 16.75240474999999307 ) ) ;
#9612=CARTESIAN_POINT ( 'NONE',  ( -35.09675569278795138, 377.2448905683720000, 15.47720386886985366 ) ) ;
#9616=CARTESIAN_POINT ( 'NONE',  ( -36.33955658999050087, 270.1198905765655809, -18.47759065022572855 ) ) ;
#9617=CARTESIAN_POINT ( 'NONE',  ( -16.84014894278199392, 427.6198905683720000, 11.84573899990672530 ) ) ;
#9619=ORIENTED_EDGE ( 'NONE', *, *, #11793, .T. ) ;
#9620=CARTESIAN_POINT ( 'NONE',  ( -28.68588794268871922, 419.7448905601784759, 19.99999999999999289 ) ) ;
#9621=EDGE_CURVE ( 'NONE', #6799, #13531, #6918, .T. ) ;
#9624=CARTESIAN_POINT ( 'NONE',  ( -36.33955658999051508, 353.8698905765656377, 18.47759065022572500 ) ) ;
#9625=CARTESIAN_POINT ( 'NONE',  ( -48.68588794268870146, 307.2448905601784759, 0.000000000000000000 ) ) ;
#9627=CARTESIAN_POINT ( 'NONE',  ( -14.48388495494899608, 339.4323905683720000, 9.489475012073731008 ) ) ;
#9628=CARTESIAN_POINT ( 'NONE',  ( -17.35679799567831338, 508.5573905765655240, -16.95518130045146421 ) ) ;
#9629=CARTESIAN_POINT ( 'NONE',  ( -35.09675569278795138, 375.7448905683720000, 15.47720386886985366 ) ) ;
#9630=CARTESIAN_POINT ( 'NONE',  ( -11.93348319268870661, 230.6823905683720284, -3.332260488124732856 ) ) ;
#9631=CARTESIAN_POINT ( 'NONE',  ( -32.01814843081344719, 386.0573905683720000, 16.75240474999999307 ) ) ;
#9633=CARTESIAN_POINT ( 'NONE',  ( -42.82802356641965957, 330.7448905765655809, -14.14213562373094746 ) ) ;
#9635=CARTESIAN_POINT ( 'NONE',  ( -40.53162694259543031, 282.6198905683720000, -11.84573899990672707 ) ) ;
#9637=CARTESIAN_POINT ( 'NONE',  ( -14.48388495494900852, 441.3073905683720568, -9.489475012073736337 ) ) ;
#9641=CARTESIAN_POINT ( 'NONE',  ( -48.68588794268872277, 501.9948905765656377, 0.000000000000000000 ) ) ;
#9642=CARTESIAN_POINT ( 'NONE',  ( -45.43829269268871229, 355.3698905683720568, 0.000000000000000000 ) ) ;
#9643=CARTESIAN_POINT ( 'NONE',  ( -40.53162694259545873, 505.1198905683720568, 11.84573899990672885 ) ) ;
#9644=CARTESIAN_POINT ( 'NONE',  ( -11.73070664223726034, 481.3073905601785896, 11.32908994701042005 ) ) ;
#9645=CARTESIAN_POINT ( 'NONE',  ( -45.43829269268870519, 323.8698905683720000, 0.000000000000000000 ) ) ;
#9648=CARTESIAN_POINT ( 'NONE',  ( -48.68588794268871567, 526.9323905601785327, -3.978247347593212080 ) ) ;
#9649=VERTEX_POINT ( 'NONE', #13542 ) ;
#9651=CARTESIAN_POINT ( 'NONE',  ( -19.19641293061498644, 401.9323905683720000, -14.20200298773971603 ) ) ;
#9652=CARTESIAN_POINT ( 'NONE',  ( -45.64106924314016567, 232.9323905765656093, 11.32908994701042538 ) ) ;
#9654=CARTESIAN_POINT ( 'NONE',  ( -11.93348319268873148, 448.8698905683720000, -2.051577885510841163E-15 ) ) ;
#9655=CARTESIAN_POINT ( 'NONE',  ( -11.93348319268873148, 448.5573905683720000, 3.332260488124728859 ) ) ;
#9657=CARTESIAN_POINT ( 'NONE',  ( -28.68588794268871567, 384.4948905765656377, 19.99999999999999289 ) ) ;
#9658=DIRECTION ( 'NONE',  ( -1.000000000000000000, 0.000000000000000000, 0.000000000000000000 ) ) ;
#9659=CARTESIAN_POINT ( 'NONE',  ( -28.68588794268871922, 389.4948905765656377, -19.99999999999999289 ) ) ;
#9662=CARTESIAN_POINT ( 'NONE',  ( -22.27502019258950128, 492.2448905683720000, -15.47720386886985544 ) ) ;
#9665=CARTESIAN_POINT ( 'NONE',  ( -21.03221929538690915, 254.1198905601784759, -18.47759065022572855 ) ) ;
#9666=CARTESIAN_POINT ( 'NONE',  ( -32.66413529028186957, 345.0573905601784759, -19.99999999999999289 ) ) ;
#9667=CARTESIAN_POINT ( 'NONE',  ( -35.09675569278795138, 413.4948905683720000, -15.47720386886985544 ) ) ;
#9668=CARTESIAN_POINT ( 'NONE',  ( -32.66413529028186957, 385.0573905601784759, -19.99999999999999289 ) ) ;
#9669=CIRCLE ( 'NONE', #3809, 15.00000000000000000 ) ;
#9670=CARTESIAN_POINT ( 'NONE',  ( -19.19641293061496867, 238.8073905683720000, 14.20200298773971426 ) ) ;
#9671=VERTEX_POINT ( 'NONE', #5403 ) ;
#9675=CARTESIAN_POINT ( 'NONE',  ( -13.20868407381887266, 460.9948905683720000, -6.410867750099233042 ) ) ;
#9676=CARTESIAN_POINT ( 'NONE',  ( -11.73070664223723192, 236.0573905765656093, 11.32908994701042005 ) ) ;
#9678=VERTEX_POINT ( 'NONE', #20023 ) ;
#9679=CARTESIAN_POINT ( 'NONE',  ( -48.68588794268872988, 521.9948905765656946, 0.000000000000000000 ) ) ;
#9680=CARTESIAN_POINT ( 'NONE',  ( -16.84014894278200813, 529.1198905683720568, 11.84573899990672530 ) ) ;
#9682=CARTESIAN_POINT ( 'NONE',  ( -40.53162694259545873, 505.1198905683720568, 11.84573899990672885 ) ) ;
#9685=CARTESIAN_POINT ( 'NONE',  ( -47.16347859291445843, 451.3698905765656377, -7.653668647301793193 ) ) ;
#9688=CARTESIAN_POINT ( 'NONE',  ( -28.68588794268870856, 336.3698905683720000, 16.75240474999999307 ) ) ;
#9689=CARTESIAN_POINT ( 'NONE',  ( -28.68588794268874054, 573.2448905601785327, 0.000000000000000000 ) ) ;
#9694=CARTESIAN_POINT ( 'NONE',  ( -38.17536295476244135, 232.3073905683720568, -14.20200298773971426 ) ) ;
#9695=CARTESIAN_POINT ( 'NONE',  ( -25.35362745456397704, 318.1823905683720568, 16.75240474999998952 ) ) ;
#9696=CARTESIAN_POINT ( 'NONE',  ( -48.68588794268865882, 446.9323905601784190, -3.978247347593264927 ) ) ;
#9697=CARTESIAN_POINT ( 'NONE',  ( -42.82802356641964536, 265.9948905601784759, -14.14213562373094746 ) ) ;
#9699=CARTESIAN_POINT ( 'NONE',  ( -32.01814843081344009, 317.5573905683720568, 16.75240474999999307 ) ) ;
#9702=CARTESIAN_POINT ( 'NONE',  ( -40.53162694259545873, 526.6198905683720568, 11.84573899990672885 ) ) ;
#9703=CARTESIAN_POINT ( 'NONE',  ( -36.33955658999051508, 369.1198905601785327, 18.47759065022572500 ) ) ;
#9707=CARTESIAN_POINT ( 'NONE',  ( -19.19641293061499354, 478.8073905683720568, 14.20200298773971426 ) ) ;
#9708=CARTESIAN_POINT ( 'NONE',  ( -45.43829269268870519, 273.8698905683720000, 0.000000000000000000 ) ) ;
#9711=CARTESIAN_POINT ( 'NONE',  ( -16.84014894278197616, 279.1198905683720568, 11.84573899990672530 ) ) ;
#9712=CARTESIAN_POINT ( 'NONE',  ( -44.16309181155856578, 313.2448905683720000, -6.410867750099231266 ) ) ;
#9713=CARTESIAN_POINT ( 'NONE',  ( -16.84014894278197616, 259.1198905683720568, 11.84573899990672530 ) ) ;
#9714=CARTESIAN_POINT ( 'NONE',  ( -40.01497788969912506, 273.5573905765656377, 16.95518130045146776 ) ) ;
#9715=CARTESIAN_POINT ( 'NONE',  ( -42.82802356641967378, 475.9948905601784759, -14.14213562373094746 ) ) ;
#9718=CARTESIAN_POINT ( 'NONE',  ( -42.88789093042843348, 374.4323905683720000, -9.489475012073736337 ) ) ;
#9721=CARTESIAN_POINT ( 'NONE',  ( -13.20868407381886911, 429.4948905683720568, -6.410867750099233042 ) ) ;
#9724=CARTESIAN_POINT ( 'NONE',  ( -32.66413529028188378, 425.0573905601784759, -19.99999999999999289 ) ) ;
#9727=ORIENTED_EDGE ( 'NONE', *, *, #15379, .F. ) ;
#9729=CARTESIAN_POINT ( 'NONE',  ( -40.01497788969913216, 305.6823905601784190, -16.95518130045146421 ) ) ;
#9732=CARTESIAN_POINT ( 'NONE',  ( -38.17536295476244845, 336.9323905683720568, 14.20200298773971781 ) ) ;
#9733=CARTESIAN_POINT ( 'NONE',  ( -32.66413529028189799, 509.8073905765655809, -19.99999999999999289 ) ) ;
#9734=CARTESIAN_POINT ( 'NONE',  ( -11.93348319268872260, 379.1823905683721136, -3.332260488124732856 ) ) ;
#9736=CARTESIAN_POINT ( 'NONE',  ( -25.35362745456398414, 386.6823905683720000, 16.75240474999998952 ) ) ;
#9737=CARTESIAN_POINT ( 'NONE',  ( -47.16347859291443712, 322.6198905765655809, 7.653668647301805628 ) ) ;
#9739=CARTESIAN_POINT ( 'NONE',  ( -14.48388495494899075, 279.8073905683720000, -9.489475012073734561 ) ) ;
#9741=CARTESIAN_POINT ( 'NONE',  ( -35.09675569278795138, 443.4948905683720568, -15.47720386886985544 ) ) ;
#9743=LINE ( 'NONE', #4670, #10948 ) ;
#9745=FACE_OUTER_BOUND ( 'NONE', #7783, .T. ) ;
#9747=CARTESIAN_POINT ( 'NONE',  ( -32.66413529028187668, 449.4323905601785327, 19.99999999999999289 ) ) ;
#9748=CARTESIAN_POINT ( 'NONE',  ( -42.88789093042843348, 356.3073905683720000, 9.489475012073736337 ) ) ;
#9749=CARTESIAN_POINT ( 'NONE',  ( -45.43829269268871940, 484.1823905683720000, 3.332260488124734632 ) ) ;
#9751=CARTESIAN_POINT ( 'NONE',  ( -14.54375231895778420, 483.4948905601784759, -14.14213562373094746 ) ) ;
#9752=CARTESIAN_POINT ( 'NONE',  ( -19.19641293061497933, 310.4323905683720568, -14.20200298773971603 ) ) ;
#9758=CARTESIAN_POINT ( 'NONE',  ( -32.01814843081344719, 407.5573905683720568, 16.75240474999999307 ) ) ;
#9759=CARTESIAN_POINT ( 'NONE',  ( -48.68588794268878672, 232.3073905765656377, 3.978247347592954952 ) ) ;
#9760=CARTESIAN_POINT ( 'NONE',  ( -19.19641293061498999, 447.3073905683720568, 14.20200298773971426 ) ) ;
#9761=CARTESIAN_POINT ( 'NONE',  ( -14.48388495494901029, 449.8073905683720000, -9.489475012073734561 ) ) ;
#9763=CARTESIAN_POINT ( 'NONE',  ( -47.16347859291445133, 392.6198905765655809, 7.653668647301805628 ) ) ;
#9765=CARTESIAN_POINT ( 'NONE',  ( -32.66413529028185536, 265.0573905601784759, -19.99999999999999289 ) ) ;
#9768=CARTESIAN_POINT ( 'NONE',  ( -11.93348319268873681, 490.3698905683720568, -2.051577885510841163E-15 ) ) ;
#9770=CARTESIAN_POINT ( 'NONE',  ( -10.20829729246299777, 462.8698905601785327, -7.653668647301794969 ) ) ;
#9771=CARTESIAN_POINT ( 'NONE',  ( -47.16347859291446554, 517.8698905601785327, 7.653668647301805628 ) ) ;
#9773=CARTESIAN_POINT ( 'NONE',  ( -16.84014894278199748, 411.6198905683720568, -11.84573899990672707 ) ) ;
#9774=CARTESIAN_POINT ( 'NONE',  ( -8.685887942688605534, 467.3073905765656946, -3.978247347592846594 ) ) ;
#9775=CARTESIAN_POINT ( 'NONE',  ( -22.27502019258945865, 228.4948905683720284, 15.47720386886985189 ) ) ;
#9779=CARTESIAN_POINT ( 'NONE',  ( -44.16309181155857289, 445.9948905683720568, 6.410867750099241924 ) ) ;
#9780=CARTESIAN_POINT ( 'NONE',  ( -45.64106924314017277, 222.9323905765656093, 11.32908994701042715 ) ) ;
#9783=CARTESIAN_POINT ( 'NONE',  ( -45.64106924314020119, 522.9323905765655809, 11.32908994701042538 ) ) ;
#9784=CARTESIAN_POINT ( 'NONE',  ( -13.20868407381884602, 229.4948905683720284, -6.410867750099233042 ) ) ;
#9785=AXIS2_PLACEMENT_3D ( 'NONE', #6601, #13222, #19810 ) ;
#9786=ORIENTED_EDGE ( 'NONE', *, *, #7575, .T. ) ;
#9787=CARTESIAN_POINT ( 'NONE',  ( -38.17536295476246977, 505.4323905683720568, 14.20200298773971781 ) ) ;
#9789=CARTESIAN_POINT ( 'NONE',  ( -48.68588794268872277, 451.6823905765656377, -3.978247347593158345 ) ) ;
#9790=CARTESIAN_POINT ( 'NONE',  ( -21.03221929538691626, 298.8698905765656377, -18.47759065022572855 ) ) ;
#9795=CARTESIAN_POINT ( 'NONE',  ( -24.70764059509554045, 290.0573905601784759, 19.99999999999998934 ) ) ;
#9797=DIRECTION ( 'NONE',  ( -1.191790137725560488E-16, 1.000000000000000000, -0.000000000000000000 ) ) ;
#9798=CARTESIAN_POINT ( 'NONE',  ( -40.53162694259543031, 316.6198905683720568, 11.84573899990672885 ) ) ;
#9799=CARTESIAN_POINT ( 'NONE',  ( -28.68588794268870146, 269.7448905601784759, 19.99999999999999289 ) ) ;
#9801=AXIS2_PLACEMENT_3D ( 'NONE', #8093, #8203, #14830 ) ;
#9802=CARTESIAN_POINT ( 'NONE',  ( -38.17536295476244845, 293.8073905683720568, -14.20200298773971426 ) ) ;
#9803=CARTESIAN_POINT ( 'NONE',  ( -40.53162694259545873, 524.1198905683720568, -11.84573899990672707 ) ) ;
#9804=CARTESIAN_POINT ( 'NONE',  ( -48.68588794268870856, 357.5573905601784759, 3.978247347593168115 ) ) ;
#9805=ADVANCED_FACE ( 'NONE', ( #6712 ), #7127, .F. ) ;
#9808=CARTESIAN_POINT ( 'NONE',  ( -42.88789093042844769, 494.4323905683720000, -9.489475012073736337 ) ) ;
#9810=CARTESIAN_POINT ( 'NONE',  ( -22.27502019258947641, 280.7448905683720568, -15.47720386886985544 ) ) ;
#9811=EDGE_LOOP ( 'NONE', ( #11096, #20731, #233, #2023 ) ) ;
#9812=CARTESIAN_POINT ( 'NONE',  ( -25.35362745456397349, 288.1823905683720000, 16.75240474999998952 ) ) ;
#9813=CARTESIAN_POINT ( 'NONE',  ( -19.19641293061497223, 261.9323905683720568, -14.20200298773971603 ) ) ;
#9814=CARTESIAN_POINT ( 'NONE',  ( -42.82802356641964536, 253.2448905765656377, 14.14213562373094923 ) ) ;
#9816=CARTESIAN_POINT ( 'NONE',  ( -16.84014894278197616, 230.1198905683720000, -11.84573899990672707 ) ) ;
#9817=CARTESIAN_POINT ( 'NONE',  ( -11.93348319268871194, 269.1823905683720000, -3.332260488124732856 ) ) ;
#9818=CARTESIAN_POINT ( 'NONE',  ( -42.88789093042843348, 386.3073905683720000, 9.489475012073736337 ) ) ;
#9823=CARTESIAN_POINT ( 'NONE',  ( -38.17536295476246266, 422.3073905683720568, -14.20200298773971426 ) ) ;
#9826=CARTESIAN_POINT ( 'NONE',  ( -32.66413529028188378, 429.4323905601785896, 19.99999999999999289 ) ) ;
#9833=CARTESIAN_POINT ( 'NONE',  ( -21.03221929538691626, 304.1198905601785327, -18.47759065022572855 ) ) ;
#9835=CARTESIAN_POINT ( 'NONE',  ( -45.43829269268871229, 335.0573905683720568, -3.332260488124726638 ) ) ;
#9836=CARTESIAN_POINT ( 'NONE',  ( -8.685887942688738761, 487.3073905765656377, -3.978247347593165895 ) ) ;
#9837=CARTESIAN_POINT ( 'NONE',  ( -44.16309181155857289, 373.2448905683720000, -6.410867750099231266 ) ) ;
#9838=CARTESIAN_POINT ( 'NONE',  ( -21.25395633610896695, 222.1412455016266279, -15.05426537146665389 ) ) ;
#9839=CARTESIAN_POINT ( 'NONE',  ( -42.88789093042843348, 382.9323905683720000, -9.489475012073734561 ) ) ;
#9840=CARTESIAN_POINT ( 'NONE',  ( -11.73070664223724613, 307.9323905765656946, -11.32908994701042715 ) ) ;
#9842=CARTESIAN_POINT ( 'NONE',  ( -11.93348319268871194, 288.8698905683720568, -2.051577885510841163E-15 ) ) ;
#9844=CARTESIAN_POINT ( 'NONE',  ( -32.01814843081345430, 437.5573905683720000, 16.75240474999999307 ) ) ;
#9848=CARTESIAN_POINT ( 'NONE',  ( -45.43829269268873361, 535.3698905683720568, 0.000000000000000000 ) ) ;
#9849=CARTESIAN_POINT ( 'NONE',  ( -11.93348319268871904, 350.3698905683720568, -2.051577885510841163E-15 ) ) ;
#9850=CARTESIAN_POINT ( 'NONE',  ( -14.48388495494901385, 487.9323905683719431, 9.489475012073732785 ) ) ;
#9851=ORIENTED_EDGE ( 'NONE', *, *, #6160, .F. ) ;
#9852=CARTESIAN_POINT ( 'NONE',  ( -42.82802356641967378, 488.4948905601784759, 14.14213562373094923 ) ) ;
#9853=CARTESIAN_POINT ( 'NONE',  ( -42.88789093042842637, 294.8073905683720000, 9.489475012073736337 ) ) ;
#9855=CARTESIAN_POINT ( 'NONE',  ( -8.685887942688809815, 346.6823905765656377, 3.978247347593374172 ) ) ;
#9860=CARTESIAN_POINT ( 'NONE',  ( -32.01814843081344719, 397.5573905683720568, 16.75240474999999307 ) ) ;
#9863=CARTESIAN_POINT ( 'NONE',  ( -44.16309181155857999, 433.2448905683720000, -6.410867750099231266 ) ) ;
#9864=CARTESIAN_POINT ( 'NONE',  ( -35.09675569278795138, 441.9948905683720568, -15.47720386886985544 ) ) ;
#9867=CARTESIAN_POINT ( 'NONE',  ( -10.20829729246298712, 376.3698905765656377, 7.653668647301790529 ) ) ;
#9868=DIRECTION ( 'NONE',  ( 0.000000000000000000, 0.000000000000000000, 1.000000000000000000 ) ) ;
#9870=CARTESIAN_POINT ( 'NONE',  ( -48.68588794268862330, 431.6823905765655240, -3.978247347593371508 ) ) ;
#9871=CARTESIAN_POINT ( 'NONE',  ( -40.01497788969915348, 490.4323905765656377, -16.95518130045146421 ) ) ;
#9872=CARTESIAN_POINT ( 'NONE',  ( -11.93348319268873858, 500.6823905683720568, -3.332260488124732856 ) ) ;
#9873=ADVANCED_FACE ( 'NONE', ( #354 ), #2601, .T. ) ;
#9877=( BOUNDED_CURVE ( )  B_SPLINE_CURVE ( 2, ( #1927, #6977, #6870, #18451, #3636, #10219, #10322, #16842, #2029, #8597, #15332, #13599, #516, #1248, #19199, #2654, #17465 ),
 .UNSPECIFIED., .F., .T. ) 
 B_SPLINE_CURVE_WITH_KNOTS ( ( 3, 2, 2, 2, 2, 2, 2, 2, 3 ),
 ( 0.2812500000000000555, 0.2832031250000000555, 0.2851562500000000555, 0.2871093750000000555, 0.2890625000000001110, 0.2910156250000001110, 0.2929687500000001110, 0.2949218750000001110, 0.2968750000000001110 ),
 .UNSPECIFIED. ) 
 CURVE ( )  GEOMETRIC_REPRESENTATION_ITEM ( )  RATIONAL_B_SPLINE_CURVE ( ( 0.9999999999999994449, 0.9807852804032309857, 1.000000000000000000, 0.9807852804032304306, 1.000000000000000000, 0.9807852804032304306, 1.000000000000000000, 0.9807852804032304306, 1.000000000000000000, 0.9807852804032304306, 1.000000000000000000, 0.9807852804032304306, 1.000000000000000000, 0.9807852804032304306, 1.000000000000000000, 0.9807852804032293204, 1.000000000000001110 ) ) 
 REPRESENTATION_ITEM ( '' )  );
#9878=EDGE_CURVE ( 'NONE', #18296, #4322, #7448, .T. ) ;
#9879=VECTOR ( 'NONE', #5098, 1000.000000000000000 ) ;
#9880=CARTESIAN_POINT ( 'NONE',  ( -38.17536295476245556, 416.9323905683720568, 14.20200298773971781 ) ) ;
#9881=CARTESIAN_POINT ( 'NONE',  ( -42.82802356641967378, 470.7448905765655809, -14.14213562373094746 ) ) ;
#9882=CARTESIAN_POINT ( 'NONE',  ( -38.17536295476244135, 223.8073905683720284, -14.20200298773971426 ) ) ;
#9885=FACE_OUTER_BOUND ( 'NONE', #3091, .T. ) ;
#9887=CARTESIAN_POINT ( 'NONE',  ( -14.48388495494901029, 451.3073905683720568, -9.489475012073734561 ) ) ;
#9888=CARTESIAN_POINT ( 'NONE',  ( -35.09675569278796559, 531.9948905683720568, -15.47720386886985544 ) ) ;
#9889=EDGE_CURVE ( 'NONE', #13531, #13961, #10952, .T. ) ;
#9892=CARTESIAN_POINT ( 'NONE',  ( -16.84014894278197616, 230.1198905683720000, -11.84573899990672707 ) ) ;
#9893=ORIENTED_EDGE ( 'NONE', *, *, #6691, .F. ) ;
#9894=CARTESIAN_POINT ( 'NONE',  ( -13.20868407381887621, 508.2448905683720568, 6.410867750099229490 ) ) ;
#9896=VECTOR ( 'NONE', #19232, 1000.000000000000000 ) ;
#9897=CARTESIAN_POINT ( 'NONE',  ( -17.35679799567830273, 435.4323905765656377, 16.95518130045146421 ) ) ;
#9899=CARTESIAN_POINT ( 'NONE',  ( -40.01497788969912506, 250.4323905765656377, -16.95518130045146421 ) ) ;
#9900=CARTESIAN_POINT ( 'NONE',  ( -42.82802356641967378, 453.2448905765656377, 14.14213562373094923 ) ) ;
#9903=VECTOR ( 'NONE', #11725, 1000.000000000000000 ) ;
#9905=CARTESIAN_POINT ( 'NONE',  ( -11.73070664223726389, 496.0573905765656946, 11.32908994701042005 ) ) ;
#9906=CARTESIAN_POINT ( 'NONE',  ( -44.16309181155855867, 305.9948905683720568, 6.410867750099241924 ) ) ;
#9908=CARTESIAN_POINT ( 'NONE',  ( -36.33955658999050087, 275.3698905601784759, -18.47759065022572855 ) ) ;
#9909=CARTESIAN_POINT ( 'NONE',  ( -48.68588794268885067, 412.3073905765655809, 3.978247347592849259 ) ) ;
#9910=CARTESIAN_POINT ( 'NONE',  ( -28.68588794268870856, 292.8698905683720568, -16.75240474999999307 ) ) ;
#9912=CARTESIAN_POINT ( 'NONE',  ( -22.27502019258950128, 502.2448905683720568, -15.47720386886985544 ) ) ;
#9913=CARTESIAN_POINT ( 'NONE',  ( -17.35679799567829207, 360.6823905601785327, 16.95518130045146421 ) ) ;
#9917=CARTESIAN_POINT ( 'NONE',  ( -44.16309181155857999, 475.9948905683720000, 6.410867750099241924 ) ) ;
#9918=CARTESIAN_POINT ( 'NONE',  ( -28.68588794268874054, 573.2448905601785327, 0.000000000000000000 ) ) ;
#9919=CARTESIAN_POINT ( 'NONE',  ( -14.48388495494898720, 277.9323905683720000, 9.489475012073732785 ) ) ;
#9922=CARTESIAN_POINT ( 'NONE',  ( -13.20868407381884957, 289.7448905683720568, 6.410867750099229490 ) ) ;
#9923=CARTESIAN_POINT ( 'NONE',  ( -32.01814843081343298, 263.1823905683720000, -16.75240474999999307 ) ) ;
#9924=CARTESIAN_POINT ( 'NONE',  ( -45.64106924314017277, 251.0573905765656093, -11.32908994701042715 ) ) ;
#9925=CARTESIAN_POINT ( 'NONE',  ( -14.54375231895775045, 230.9948905601784759, 14.14213562373094568 ) ) ;
#9926=CARTESIAN_POINT ( 'NONE',  ( -17.35679799567828496, 258.5573905765656377, -16.95518130045146421 ) ) ;
#9927=CARTESIAN_POINT ( 'NONE',  ( -25.35362745456396993, 276.6823905683720000, 16.75240474999998952 ) ) ;
#9928=CARTESIAN_POINT ( 'NONE',  ( -38.17536295476244845, 386.9323905683721136, 14.20200298773971781 ) ) ;
#9931=CARTESIAN_POINT ( 'NONE',  ( -21.03221929538693402, 458.8698905765656377, -18.47759065022572855 ) ) ;
#9933=CARTESIAN_POINT ( 'NONE',  ( -13.20868407381886556, 418.2448905683720568, 6.410867750099229490 ) ) ;
#9934=CARTESIAN_POINT ( 'NONE',  ( -42.82802356641968089, 508.4948905601784759, 14.14213562373094923 ) ) ;
#9935=ORIENTED_EDGE ( 'NONE', *, *, #12335, .T. ) ;
#9936=CARTESIAN_POINT ( 'NONE',  ( -11.73070664223725501, 431.3073905601785327, 11.32908994701042005 ) ) ;
#9941=CARTESIAN_POINT ( 'NONE',  ( -45.64106924314017988, 352.9323905765656946, 11.32908994701042538 ) ) ;
#9942=CARTESIAN_POINT ( 'NONE',  ( -10.20829729246297823, 302.8698905601784759, -7.653668647301794969 ) ) ;
#9944=EDGE_CURVE ( 'NONE', #4208, #6694, #2495, .T. ) ;
#9945=CARTESIAN_POINT ( 'NONE',  ( -44.16309181155857289, 344.7448905683720568, -6.410867750099231266 ) ) ;
#9947=CARTESIAN_POINT ( 'NONE',  ( -48.68588794268872277, 491.6823905765656946, -3.978247347593158345 ) ) ;
#9948=CARTESIAN_POINT ( 'NONE',  ( -11.93348319268872260, 369.1823905683720000, -3.332260488124732856 ) ) ;
#9949=CARTESIAN_POINT ( 'NONE',  ( -22.27502019258949062, 380.7448905683720000, -15.47720386886985544 ) ) ;
#9950=CARTESIAN_POINT ( 'NONE',  ( -10.20829729246297823, 296.3698905765655809, 7.653668647301790529 ) ) ;
#9951=DIRECTION ( 'NONE',  ( -1.191790137725560488E-16, 1.000000000000000000, -0.000000000000000000 ) ) ;
#9952=CARTESIAN_POINT ( 'NONE',  ( -28.68588794268870856, 291.3698905683720568, -16.75240474999999307 ) ) ;
#9953=CARTESIAN_POINT ( 'NONE',  ( -48.68588794268869435, 237.2448905601785043, 0.000000000000000000 ) ) ;
#9954=CARTESIAN_POINT ( 'NONE',  ( -38.17536295476246266, 443.8073905683720568, -14.20200298773971426 ) ) ;
#9957=CARTESIAN_POINT ( 'NONE',  ( -11.73070664223724080, 283.1823905601784759, -11.32908994701042538 ) ) ;
#9958=EDGE_CURVE ( 'NONE', #14145, #19311, #18919, .T. ) ;
#9960=CARTESIAN_POINT ( 'NONE',  ( -48.68588794268869435, 267.2448905601784759, 0.000000000000000000 ) ) ;
#9962=CARTESIAN_POINT ( 'NONE',  ( -44.16309181155856578, 345.9948905683720000, 6.410867750099241924 ) ) ;
#9963=CARTESIAN_POINT ( 'NONE',  ( -19.19641293061499709, 480.4323905683720568, -14.20200298773971603 ) ) ;
#9964=ORIENTED_EDGE ( 'NONE', *, *, #1555, .F. ) ;
#9965=CARTESIAN_POINT ( 'NONE',  ( -17.35679799567830983, 483.8073905601784190, -16.95518130045146421 ) ) ;
#9966=CARTESIAN_POINT ( 'NONE',  ( -35.09675569278794427, 305.7448905683720568, 15.47720386886985366 ) ) ;
#9968=DIRECTION ( 'NONE',  ( 0.000000000000000000, 0.000000000000000000, 1.000000000000000000 ) ) ;
#9969=ORIENTED_EDGE ( 'NONE', *, *, #1134, .F. ) ;
#9972=CARTESIAN_POINT ( 'NONE',  ( -19.19641293061498644, 408.8073905683720568, 14.20200298773971426 ) ) ;
#9974=CARTESIAN_POINT ( 'NONE',  ( -21.03221929538691271, 385.1198905765656377, 18.47759065022572500 ) ) ;
#9975=CARTESIAN_POINT ( 'NONE',  ( -13.20868407381886556, 418.2448905683720568, 6.410867750099229490 ) ) ;
#9976=CARTESIAN_POINT ( 'NONE',  ( -19.19641293061499354, 450.4323905683720000, -14.20200298773971603 ) ) ;
#9978=LINE ( 'NONE', #166, #12745 ) ;
#9979=CARTESIAN_POINT ( 'NONE',  ( -32.66413529028187668, 364.1823905765656377, 19.99999999999999289 ) ) ;
#9981=CARTESIAN_POINT ( 'NONE',  ( -42.82802356641964536, 265.9948905601784759, -14.14213562373094746 ) ) ;
#9982=CARTESIAN_POINT ( 'NONE',  ( -17.35679799567831338, 488.5573905765655809, -16.95518130045146421 ) ) ;
#9983=CARTESIAN_POINT ( 'NONE',  ( -28.68588794268873343, 502.8698905683719431, -16.75240474999999307 ) ) ;
#9986=CARTESIAN_POINT ( 'NONE',  ( -25.35362745456399836, 412.5573905683719431, -16.75240474999999307 ) ) ;
#9988=CARTESIAN_POINT ( 'NONE',  ( -11.93348319268870839, 240.0573905683720000, 3.332260488124728415 ) ) ;
#9989=CARTESIAN_POINT ( 'NONE',  ( -11.93348319268872260, 358.5573905683720000, 3.332260488124728415 ) ) ;
#9991=CARTESIAN_POINT ( 'NONE',  ( -45.43829269268872650, 533.5573905683720568, -3.332260488124726194 ) ) ;
#9993=CARTESIAN_POINT ( 'NONE',  ( -11.93348319268873148, 450.6823905683720568, -3.332260488124732856 ) ) ;
#9994=CARTESIAN_POINT ( 'NONE',  ( -40.53162694259545873, 532.6198905683720568, -11.84573899990672707 ) ) ;
#9997=CARTESIAN_POINT ( 'NONE',  ( -21.03221929538691626, 430.3698905601784759, 18.47759065022572500 ) ) ;
#9998=CARTESIAN_POINT ( 'NONE',  ( -28.68588794268872633, 486.3698905683720568, 16.75240474999999307 ) ) ;
#9999=EDGE_CURVE ( 'NONE', #313, #11409, #1307, .T. ) ;
#10001=CARTESIAN_POINT ( 'NONE',  ( -14.48388495494901385, 497.9323905683720568, 9.489475012073731008 ) ) ;
#10003=EDGE_CURVE ( 'NONE', #16434, #1235, #4742, .T. ) ;
#10004=CARTESIAN_POINT ( 'NONE',  ( -45.64106924314019409, 432.9323905765656946, 11.32908994701042715 ) ) ;
#10005=CARTESIAN_POINT ( 'NONE',  ( -40.01497788969913216, 300.4323905765656377, -16.95518130045146421 ) ) ;
#10006=CARTESIAN_POINT ( 'NONE',  ( -48.68588794268869435, 251.9948905765656093, 0.000000000000000000 ) ) ;
#10007=CARTESIAN_POINT ( 'NONE',  ( -21.03221929538691981, 455.1198905765655809, 18.47759065022572500 ) ) ;
#10010=( BOUNDED_CURVE ( )  B_SPLINE_CURVE ( 2, ( #17104, #8864, #13862, #18814, #3995, #2713, #12558, #19153, #4328, #17833, #2603, #9183, #14503, #4542, #7982 ),
 .UNSPECIFIED., .F., .T. ) 
 B_SPLINE_CURVE_WITH_KNOTS ( ( 3, 2, 2, 2, 2, 2, 2, 3 ),
 ( 0.9687500000000001110, 0.9707031250000001110, 0.9726562500000001110, 0.9746093750000000000, 0.9765625000000000000, 0.9785156250000000000, 0.9791718336226143959, 0.9791727248540345041 ),
 .UNSPECIFIED. ) 
 CURVE ( )  GEOMETRIC_REPRESENTATION_ITEM ( )  RATIONAL_B_SPLINE_CURVE ( ( 0.9999999999999988898, 0.9807852804032315408, 1.000000000000000000, 0.9807852804032304306, 1.000000000000000000, 0.9807852804032304306, 1.000000000000000000, 0.9807852804032304306, 1.000000000000000000, 0.9807852804032304306, 1.000000000000000000, 0.9935442612835747589, 0.9914265054520787768, 0.9914265054520787768, 0.9914265054520787768 ) ) 
 REPRESENTATION_ITEM ( '' )  );
#10012=CARTESIAN_POINT ( 'NONE',  ( -24.70764059509556532, 494.8073905765656377, 19.99999999999998934 ) ) ;
#10013=CARTESIAN_POINT ( 'NONE',  ( -11.93348319268871371, 300.3698905683720568, -2.051577885510841163E-15 ) ) ;
#10015=CARTESIAN_POINT ( 'NONE',  ( -8.685887942688706786, 232.2448905601785043, -2.449293598294705724E-15 ) ) ;
#10016=CARTESIAN_POINT ( 'NONE',  ( -45.64106924314017277, 266.3073905601784190, -11.32908994701042715 ) ) ;
#10018=CARTESIAN_POINT ( 'NONE',  ( -28.68588794268870146, 287.8698905683720568, 16.75240474999999307 ) ) ;
#10020=CARTESIAN_POINT ( 'NONE',  ( -21.03221929538694468, 534.1198905601785327, -18.47759065022572855 ) ) ;
#10021=CARTESIAN_POINT ( 'NONE',  ( -45.43829269268872650, 505.6823905683720568, 3.332260488124734632 ) ) ;
#10022=AXIS2_PLACEMENT_3D ( 'NONE', #189, #15109, #6968 ) ;
#10023=CARTESIAN_POINT ( 'NONE',  ( -8.685887942688616192, 227.3073905765656377, -3.978247347592952732 ) ) ;
#10025=CARTESIAN_POINT ( 'NONE',  ( -45.43829269268871940, 475.6823905683720000, 3.332260488124734632 ) ) ;
#10027=CARTESIAN_POINT ( 'NONE',  ( -13.20868407381884779, 259.4948905683720568, -6.410867750099233042 ) ) ;
#10030=CARTESIAN_POINT ( 'NONE',  ( -11.93348319268870661, 240.0573905683720000, 3.332260488124728859 ) ) ;
#10031=CARTESIAN_POINT ( 'NONE',  ( -45.64106924314017277, 242.9323905765656377, 11.32908994701042715 ) ) ;
#10034=CARTESIAN_POINT ( 'NONE',  ( -10.20829729246297113, 231.6198905601785043, 7.653668647301790529 ) ) ;
#10036=CARTESIAN_POINT ( 'NONE',  ( -45.43829269268869808, 263.8698905683720000, 0.000000000000000000 ) ) ;
#10037=CARTESIAN_POINT ( 'NONE',  ( -28.68588794268871567, 352.8698905683720568, -16.75240474999999307 ) ) ;
#10041=CARTESIAN_POINT ( 'NONE',  ( -45.43829269268871229, 423.5573905683720000, -3.332260488124726194 ) ) ;
#10042=CARTESIAN_POINT ( 'NONE',  ( -47.16347859291444422, 341.3698905765655809, -7.653668647301793193 ) ) ;
#10044=CARTESIAN_POINT ( 'NONE',  ( -17.35679799567829917, 410.6823905601784759, 16.95518130045146421 ) ) ;
#10045=ORIENTED_EDGE ( 'NONE', *, *, #19227, .T. ) ;
#10049=CARTESIAN_POINT ( 'NONE',  ( -25.35362745456401257, 522.5573905683720568, -16.75240474999999307 ) ) ;
#10050=CARTESIAN_POINT ( 'NONE',  ( -36.33955658999050797, 309.1198905601785327, 18.47759065022572500 ) ) ;
#10053=CARTESIAN_POINT ( 'NONE',  ( -11.93348319268871727, 330.6823905683721136, -3.332260488124732856 ) ) ;
#10055=CARTESIAN_POINT ( 'NONE',  ( -25.35362745456398059, 356.6823905683720568, 16.75240474999998952 ) ) ;
#10056=CARTESIAN_POINT ( 'NONE',  ( -32.01814843081344719, 361.6823905683721136, -16.75240474999999307 ) ) ;
#10057=CARTESIAN_POINT ( 'NONE',  ( -42.82802356641965247, 303.2448905765656377, 14.14213562373094923 ) ) ;
#10060=CARTESIAN_POINT ( 'NONE',  ( -14.48388495494898720, 267.9323905683720568, 9.489475012073731008 ) ) ;
#10062=CARTESIAN_POINT ( 'NONE',  ( -13.20868407381886556, 419.7448905683720000, 6.410867750099229490 ) ) ;
#10064=CARTESIAN_POINT ( 'NONE',  ( -8.685887942688738761, 502.2448905601784190, -2.449293598294705724E-15 ) ) ;
#10065=CARTESIAN_POINT ( 'NONE',  ( -8.685887942688712116, 276.9948905765656377, -2.449293598294705724E-15 ) ) ;
#10067=CARTESIAN_POINT ( 'NONE',  ( -25.35362745456397704, 338.1823905683720000, 16.75240474999998952 ) ) ;
#10068=CARTESIAN_POINT ( 'NONE',  ( -42.88789093042844769, 484.8073905683720000, 9.489475012073736337 ) ) ;
#10069=AXIS2_PLACEMENT_3D ( 'NONE', #19554, #19657, #9601 ) ;
#10072=CARTESIAN_POINT ( 'NONE',  ( -21.03221929538692336, 480.3698905601784759, 18.47759065022572500 ) ) ;
#10073=CARTESIAN_POINT ( 'NONE',  ( -44.16309181155856578, 303.2448905683720000, -6.410867750099231266 ) ) ;
#10078=ADVANCED_FACE ( 'NONE', ( #14608 ), #2817, .T. ) ;
#10079=CARTESIAN_POINT ( 'NONE',  ( -42.88789093042844058, 404.4323905683721136, -9.489475012073734561 ) ) ;
#10080=CARTESIAN_POINT ( 'NONE',  ( -17.35679799567829917, 445.4323905765656377, 16.95518130045146421 ) ) ;
#10081=CARTESIAN_POINT ( 'NONE',  ( -36.33955658999051508, 383.8698905765656377, 18.47759065022572500 ) ) ;
#10082=CARTESIAN_POINT ( 'NONE',  ( -44.16309181155857289, 424.4948905683720568, 6.410867750099241924 ) ) ;
#10083=CARTESIAN_POINT ( 'NONE',  ( -25.35362745456396993, 268.1823905683720000, 16.75240474999998952 ) ) ;
#10084=CARTESIAN_POINT ( 'NONE',  ( -32.01814843081344719, 436.0573905683720568, 16.75240474999999307 ) ) ;
#10087=CARTESIAN_POINT ( 'NONE',  ( -48.68588794268870856, 371.9948905765655809, 0.000000000000000000 ) ) ;
#10089=CARTESIAN_POINT ( 'NONE',  ( -48.68588794268869435, 267.2448905601784759, 0.000000000000000000 ) ) ;
#10090=CARTESIAN_POINT ( 'NONE',  ( -45.43829269268871229, 333.8698905683720000, 0.000000000000000000 ) ) ;
#10092=CARTESIAN_POINT ( 'NONE',  ( -16.84014894278200458, 491.6198905683720000, -11.84573899990672707 ) ) ;
#10097=CARTESIAN_POINT ( 'NONE',  ( -38.17536295476246266, 403.8073905683721136, -14.20200298773971426 ) ) ;
#10100=CARTESIAN_POINT ( 'NONE',  ( 8.313338196759850973, 218.8819358349711024, 2.050088646935358305 ) ) ;
#10101=CARTESIAN_POINT ( 'NONE',  ( -35.09675569278794427, 361.9948905683720568, -15.47720386886985544 ) ) ;
#10103=CARTESIAN_POINT ( 'NONE',  ( -38.17536295476247687, 522.3073905683721705, -14.20200298773971426 ) ) ;
#10105=CARTESIAN_POINT ( 'NONE',  ( -19.19641293061498999, 448.8073905683721136, 14.20200298773971426 ) ) ;
#10106=CARTESIAN_POINT ( 'NONE',  ( -19.19641293061499709, 517.3073905683720568, 14.20200298773971426 ) ) ;
#10109=CARTESIAN_POINT ( 'NONE',  ( -14.54375231895779130, 528.2448905765656946, -14.14213562373094746 ) ) ;
#10110=CARTESIAN_POINT ( 'NONE',  ( -38.17536295476246266, 485.4323905683720000, 14.20200298773971781 ) ) ;
#10113=CARTESIAN_POINT ( 'NONE',  ( -11.93348319268873858, 509.1823905683720000, -3.332260488124732856 ) ) ;
#10115=CARTESIAN_POINT ( 'NONE',  ( -8.685887942688729879, 427.3073905765655809, -3.978247347593165895 ) ) ;
#10116=CARTESIAN_POINT ( 'NONE',  ( -28.68588794268871567, 359.4948905765656377, -19.99999999999999289 ) ) ;
#10117=CARTESIAN_POINT ( 'NONE',  ( -32.66413529028185536, 249.8073905765656662, -19.99999999999999289 ) ) ;
#10119=CARTESIAN_POINT ( 'NONE',  ( -28.68588794268874054, 573.2448905601785327, 0.000000000000000000 ) ) ;
#10123=CARTESIAN_POINT ( 'NONE',  ( -42.99819559747531628, 202.9232509211816478, -4.491669896562675568 ) ) ;
#10124=CARTESIAN_POINT ( 'NONE',  ( -19.19641293061497933, 301.9323905683720000, -14.20200298773971603 ) ) ;
#10125=CARTESIAN_POINT ( 'NONE',  ( -14.54375231895778775, 530.9948905601784190, 14.14213562373094568 ) ) ;
#10126=CARTESIAN_POINT ( 'NONE',  ( -21.03221929538690205, 270.3698905601784759, 18.47759065022572500 ) ) ;
#10128=CARTESIAN_POINT ( 'NONE',  ( -40.53162694259543031, 296.6198905683720000, 11.84573899990672885 ) ) ;
#10132=CARTESIAN_POINT ( 'NONE',  ( -28.68588794268872988, 497.8698905683720568, 16.75240474999999307 ) ) ;
#10134=ORIENTED_EDGE ( 'NONE', *, *, #7452, .T. ) ;
#10135=CARTESIAN_POINT ( 'NONE',  ( -42.88789093042844769, 466.3073905683720568, 9.489475012073736337 ) ) ;
#10136=DIRECTION ( 'NONE',  ( -1.191790137725560488E-16, 1.000000000000000000, -0.000000000000000000 ) ) ;
#10137=CARTESIAN_POINT ( 'NONE',  ( -44.16309181155855157, 264.4948905683720000, 6.410867750099241924 ) ) ;
#10139=VERTEX_POINT ( 'NONE', #4846 ) ;
#10140=( BOUNDED_CURVE ( )  B_SPLINE_CURVE ( 2, ( #15042, #226, #8842, #18477, #6689, #5179, #11775, #10151, #16767, #1954, #8524, #16871, #15149, #6898, #20111, #10247, #5280 ),
 .UNSPECIFIED., .F., .T. ) 
 B_SPLINE_CURVE_WITH_KNOTS ( ( 3, 2, 2, 2, 2, 2, 2, 2, 3 ),
 ( 0.09375000000000008327, 0.09570312500000012490, 0.09765625000000018041, 0.09960937500000022204, 0.1015625000000002776, 0.1035156250000003192, 0.1054687500000003608, 0.1074218750000004163, 0.1093750000000004580 ),
 .UNSPECIFIED. ) 
 CURVE ( )  GEOMETRIC_REPRESENTATION_ITEM ( )  RATIONAL_B_SPLINE_CURVE ( ( 0.9999999999999992228, 0.9807852804032312077, 1.000000000000000000, 0.9807852804032304306, 1.000000000000000000, 0.9807852804032304306, 1.000000000000000000, 0.9807852804032304306, 1.000000000000000000, 0.9807852804032304306, 1.000000000000000000, 0.9807852804032304306, 1.000000000000000000, 0.9807852804032304306, 1.000000000000000000, 0.9807852804032258787, 1.000000000000004441 ) ) 
 REPRESENTATION_ITEM ( '' )  );
#10141=DIRECTION ( 'NONE',  ( -1.191790137725560488E-16, 1.000000000000000000, -0.000000000000000000 ) ) ;
#10142=EDGE_CURVE ( 'NONE', #12371, #368, #3512, .T. ) ;
#10143=CARTESIAN_POINT ( 'NONE',  ( -19.19641293061496512, 248.8073905683720284, 14.20200298773971426 ) ) ;
#10145=CARTESIAN_POINT ( 'NONE',  ( -10.20829729246297291, 247.6198905765656377, -7.653668647301794969 ) ) ;
#10146=CARTESIAN_POINT ( 'NONE',  ( -48.68588794268862330, 421.6823905765655240, -3.978247347593371508 ) ) ;
#10147=CARTESIAN_POINT ( 'NONE',  ( -17.35679799567828496, 233.8073905601784475, -16.95518130045146421 ) ) ;
#10148=CARTESIAN_POINT ( 'NONE',  ( -38.17536295476244135, 262.3073905683720568, -14.20200298773971426 ) ) ;
#10150=CARTESIAN_POINT ( 'NONE',  ( -28.68588794268871212, 357.8698905683720568, 16.75240474999999307 ) ) ;
#10151=CARTESIAN_POINT ( 'NONE',  ( -32.66413529028188378, 505.0573905601785327, -19.99999999999999289 ) ) ;
#10152=CARTESIAN_POINT ( 'NONE',  ( -40.53162694259544452, 412.6198905683720568, -11.84573899990672707 ) ) ;
#10154=ORIENTED_EDGE ( 'NONE', *, *, #12715, .T. ) ;
#10155=CARTESIAN_POINT ( 'NONE',  ( -42.82802356641966668, 415.9948905601785327, -14.14213562373094746 ) ) ;
#10156=ORIENTED_EDGE ( 'NONE', *, *, #4472, .F. ) ;
#10158=EDGE_LOOP ( 'NONE', ( #17743, #13848, #13399, #15746 ) ) ;
#10159=CARTESIAN_POINT ( 'NONE',  ( -44.16309181155859420, 534.7448905683720568, -6.410867750099231266 ) ) ;
#10160=CARTESIAN_POINT ( 'NONE',  ( -28.68588794268870501, 284.7448905601784759, -19.99999999999999289 ) ) ;
#10163=CARTESIAN_POINT ( 'NONE',  ( -35.09675569278794427, 333.4948905683720568, -15.47720386886985544 ) ) ;
#10164=ORIENTED_EDGE ( 'NONE', *, *, #16908, .F. ) ;
#10165=CARTESIAN_POINT ( 'NONE',  ( -35.09675569278795138, 355.7448905683720568, 15.47720386886985366 ) ) ;
#10166=CARTESIAN_POINT ( 'NONE',  ( -28.68588794268871212, 366.3698905683720568, 16.75240474999999307 ) ) ;
#10167=CARTESIAN_POINT ( 'NONE',  ( -48.68588794268870146, 311.9948905765655809, 0.000000000000000000 ) ) ;
#10169=CARTESIAN_POINT ( 'NONE',  ( -11.93348319268870839, 258.8698905683720000, -2.051577885510841163E-15 ) ) ;
#10170=CARTESIAN_POINT ( 'NONE',  ( -44.16309181155857999, 424.7448905683720000, -6.410867750099231266 ) ) ;
#10171=CARTESIAN_POINT ( 'NONE',  ( -8.685887942688712116, 266.9948905765656377, -2.449293598294705724E-15 ) ) ;
#10172=CARTESIAN_POINT ( 'NONE',  ( -45.43829269268873361, 535.3698905683720568, 0.000000000000000000 ) ) ;
#10173=CARTESIAN_POINT ( 'NONE',  ( -48.68588794268885067, 407.5573905601785327, 3.978247347592849259 ) ) ;
#10174=CARTESIAN_POINT ( 'NONE',  ( -19.19641293061497933, 318.8073905683720568, 14.20200298773971426 ) ) ;
#10175=CARTESIAN_POINT ( 'NONE',  ( -32.01814843081346140, 476.0573905683720000, 16.75240474999999307 ) ) ;
#10177=CARTESIAN_POINT ( 'NONE',  ( -17.35679799567830628, 470.6823905601784759, 16.95518130045146421 ) ) ;
#10178=CARTESIAN_POINT ( 'NONE',  ( -22.27502019258947996, 300.7448905683720568, -15.47720386886985544 ) ) ;
#10179=CARTESIAN_POINT ( 'NONE',  ( -24.70764059509554755, 344.8073905765656377, 19.99999999999998934 ) ) ;
#10182=CARTESIAN_POINT ( 'NONE',  ( -45.64106924314018698, 348.1823905601784190, 11.32908994701042715 ) ) ;
#10183=CARTESIAN_POINT ( 'NONE',  ( -38.17536295476246266, 393.8073905683720000, -14.20200298773971426 ) ) ;
#10185=DIRECTION ( 'NONE',  ( -1.000000000000000000, 0.000000000000000000, 0.000000000000000000 ) ) ;
#10186=CARTESIAN_POINT ( 'NONE',  ( -16.84014894278199392, 427.6198905683720000, 11.84573899990672530 ) ) ;
#10187=CARTESIAN_POINT ( 'NONE',  ( -45.43829269268869098, 255.6823905683720000, 3.332260488124734632 ) ) ;
#10188=CARTESIAN_POINT ( 'NONE',  ( -28.68588794268872277, 431.3698905683720000, -16.75240474999999307 ) ) ;
#10191=CARTESIAN_POINT ( 'NONE',  ( -8.685887942688722774, 366.6823905765656946, 3.978247347593161010 ) ) ;
#10193=DIRECTION ( 'NONE',  ( -1.000000000000000000, 0.000000000000000000, 0.000000000000000000 ) ) ;
#10194=CARTESIAN_POINT ( 'NONE',  ( -38.17536295476245556, 332.3073905683720000, -14.20200298773971426 ) ) ;
#10196=CARTESIAN_POINT ( 'NONE',  ( -14.48388495494901385, 471.3073905683720568, -9.489475012073736337 ) ) ;
#10198=CARTESIAN_POINT ( 'NONE',  ( -11.73070664223726212, 463.1823905601784759, -11.32908994701042538 ) ) ;
#10199=CARTESIAN_POINT ( 'NONE',  ( -40.01497788969913216, 305.6823905601784190, -16.95518130045146421 ) ) ;
#10201=CARTESIAN_POINT ( 'NONE',  ( -42.88789093042843348, 384.4323905683720000, -9.489475012073736337 ) ) ;
#10203=CARTESIAN_POINT ( 'NONE',  ( -47.16347859291446554, 536.6198905601784190, -7.653668647301793193 ) ) ;
#10204=CARTESIAN_POINT ( 'NONE',  ( -42.88789093042843348, 372.9323905683720568, -9.489475012073736337 ) ) ;
#10205=ORIENTED_EDGE ( 'NONE', *, *, #10517, .F. ) ;
#10206=CARTESIAN_POINT ( 'NONE',  ( -32.01814843081346851, 531.6823905683719431, -16.75240474999999307 ) ) ;
#10207=ORIENTED_EDGE ( 'NONE', *, *, #14481, .T. ) ;
#10208=CARTESIAN_POINT ( 'NONE',  ( -35.09675569278797269, 525.7448905683720568, 15.47720386886985366 ) ) ;
#10210=CARTESIAN_POINT ( 'NONE',  ( -17.35679799567831694, 528.5573905765656946, -16.95518130045146421 ) ) ;
#10211=CARTESIAN_POINT ( 'NONE',  ( -16.84014894278200458, 480.1198905683720000, -11.84573899990672707 ) ) ;
#10213=CARTESIAN_POINT ( 'NONE',  ( -14.48388495494901029, 487.9323905683719431, 9.489475012073731008 ) ) ;
#10216=CARTESIAN_POINT ( 'NONE',  ( -47.16347859291445133, 421.3698905765656377, -7.653668647301793193 ) ) ;
#10219=CARTESIAN_POINT ( 'NONE',  ( -40.01497788969914637, 440.4323905765656946, -16.95518130045146421 ) ) ;
#10221=CARTESIAN_POINT ( 'NONE',  ( -45.64106924314018698, 436.3073905601784759, -11.32908994701042538 ) ) ;
#10222=CARTESIAN_POINT ( 'NONE',  ( -28.68588794268872988, 494.4948905765656377, 19.99999999999999289 ) ) ;
#10223=CARTESIAN_POINT ( 'NONE',  ( -11.93348319268871549, 300.0573905683720568, 3.332260488124728415 ) ) ;
#10227=CARTESIAN_POINT ( 'NONE',  ( -16.84014894278200103, 441.6198905683720568, -11.84573899990672707 ) ) ;
#10228=CARTESIAN_POINT ( 'NONE',  ( -8.685887942688738761, 496.9948905765655809, -2.449293598294705724E-15 ) ) ;
#10229=CARTESIAN_POINT ( 'NONE',  ( -13.20868407381885135, 290.9948905683720000, -6.410867750099233042 ) ) ;
#10231=CARTESIAN_POINT ( 'NONE',  ( -38.17536295476246977, 506.9323905683720000, 14.20200298773971781 ) ) ;
#10234=CARTESIAN_POINT ( 'NONE',  ( -22.27502019258949773, 472.2448905683720568, -15.47720386886985544 ) ) ;
#10236=CARTESIAN_POINT ( 'NONE',  ( -44.16309181155855157, 254.4948905683720568, 6.410867750099241924 ) ) ;
#10237=ORIENTED_EDGE ( 'NONE', *, *, #4464, .T. ) ;
#10241=CARTESIAN_POINT ( 'NONE',  ( -40.53162694259542320, 234.1198905683720000, -11.84573899990672707 ) ) ;
#10243=CARTESIAN_POINT ( 'NONE',  ( -36.33955658999049376, 225.3698905601784759, -18.47759065022572855 ) ) ;
#10244=CARTESIAN_POINT ( 'NONE',  ( -38.17536295476244845, 272.3073905683720000, -14.20200298773971426 ) ) ;
#10245=CARTESIAN_POINT ( 'NONE',  ( -13.20868407381886023, 360.9948905683720568, -6.410867750099233042 ) ) ;
#10247=CARTESIAN_POINT ( 'NONE',  ( -8.685887942688374608, 502.5573905601784759, -3.978247347592287486 ) ) ;
#10249=CARTESIAN_POINT ( 'NONE',  ( -14.48388495494900496, 407.9323905683720000, 9.489475012073732785 ) ) ;
#10250=CARTESIAN_POINT ( 'NONE',  ( -11.73070664223724791, 337.9323905765655809, -11.32908994701042538 ) ) ;
#10251=( BOUNDED_CURVE ( )  B_SPLINE_CURVE ( 2, ( #9083, #18924, #8868, #18499, #18605, #17002, #3790, #18817, #4109, #13652, #3689, #7030, #17317, #10380, #3898, #8767, #13759 ),
 .UNSPECIFIED., .F., .T. ) 
 B_SPLINE_CURVE_WITH_KNOTS ( ( 3, 2, 2, 2, 2, 2, 2, 2, 3 ),
 ( 0.07812500000000043021, 0.08007812500000038858, 0.08203125000000034694, 0.08398437500000030531, 0.08593750000000024980, 0.08789062500000020817, 0.08984375000000016653, 0.09179687500000012490, 0.09375000000000008327 ),
 .UNSPECIFIED. ) 
 CURVE ( )  GEOMETRIC_REPRESENTATION_ITEM ( )  RATIONAL_B_SPLINE_CURVE ( ( 0.9999999999999957812, 0.9807852804032346494, 1.000000000000000000, 0.9807852804032304306, 1.000000000000000000, 0.9807852804032304306, 1.000000000000000000, 0.9807852804032304306, 1.000000000000000000, 0.9807852804032304306, 1.000000000000000000, 0.9807852804032304306, 1.000000000000000000, 0.9807852804032304306, 1.000000000000000000, 0.9807852804032296534, 1.000000000000000888 ) ) 
 REPRESENTATION_ITEM ( '' )  );
#10252=CARTESIAN_POINT ( 'NONE',  ( -21.03221929538691626, 410.3698905601784759, 18.47759065022572500 ) ) ;
#10253=ORIENTED_EDGE ( 'NONE', *, *, #2893, .F. ) ;
#10255=ORIENTED_EDGE ( 'NONE', *, *, #20031, .T. ) ;
#10257=CARTESIAN_POINT ( 'NONE',  ( -16.84014894278201169, 531.6198905683720568, -11.84573899990672707 ) ) ;
#10258=CARTESIAN_POINT ( 'NONE',  ( -10.20829729246297646, 282.8698905601784759, -7.653668647301794969 ) ) ;
#10259=CARTESIAN_POINT ( 'NONE',  ( -43.66427838156418773, 210.0786766341574889, -0.8210443013742924068 ) ) ;
#10261=CARTESIAN_POINT ( 'NONE',  ( -25.35362745456397704, 328.1823905683720568, 16.75240474999998952 ) ) ;
#10264=CARTESIAN_POINT ( 'NONE',  ( -44.16309181155856578, 354.4948905683720000, 6.410867750099241924 ) ) ;
#10266=CARTESIAN_POINT ( 'NONE',  ( -25.35362745456398059, 366.6823905683720568, 16.75240474999998952 ) ) ;
#10269=CARTESIAN_POINT ( 'NONE',  ( -24.70764059509555466, 309.1823905765656377, -19.99999999999999289 ) ) ;
#10270=DIRECTION ( 'NONE',  ( -1.191790137725560488E-16, 1.000000000000000000, -0.000000000000000000 ) ) ;
#10271=CARTESIAN_POINT ( 'NONE',  ( -42.88789093042842637, 272.9323905683721136, -9.489475012073734561 ) ) ;
#10272=CARTESIAN_POINT ( 'NONE',  ( -43.37470026482864682, 201.1699573972601343, 3.051950158715579065 ) ) ;
#10273=CARTESIAN_POINT ( 'NONE',  ( -28.68588794268872277, 412.8698905683720568, -16.75240474999999307 ) ) ;
#10274=DIRECTION ( 'NONE',  ( -1.191790137725560488E-16, 1.000000000000000000, -0.000000000000000000 ) ) ;
#10275=CARTESIAN_POINT ( 'NONE',  ( -24.70764059509555821, 354.4323905601784759, -19.99999999999999289 ) ) ;
#10276=CARTESIAN_POINT ( 'NONE',  ( -24.70764059509553690, 274.8073905765656377, 19.99999999999998934 ) ) ;
#10279=CARTESIAN_POINT ( 'NONE',  ( -16.84014894278198682, 331.6198905683720000, -11.84573899990672707 ) ) ;
#10280=CARTESIAN_POINT ( 'NONE',  ( -25.35362745456399125, 456.6823905683720000, 16.75240474999998952 ) ) ;
#10282=CARTESIAN_POINT ( 'NONE',  ( -10.20829729246299777, 471.6198905601784759, 7.653668647301790529 ) ) ;
#10283=CARTESIAN_POINT ( 'NONE',  ( -13.20868407381885135, 279.4948905683720000, -6.410867750099233042 ) ) ;
#10284=DIRECTION ( 'NONE',  ( -1.000000000000000000, 0.000000000000000000, 0.000000000000000000 ) ) ;
#10287=CARTESIAN_POINT ( 'NONE',  ( -28.68588794268871212, 344.7448905601784759, -19.99999999999999289 ) ) ;
#10288=CARTESIAN_POINT ( 'NONE',  ( -22.27502019258949062, 392.2448905683720568, -15.47720386886985544 ) ) ;
#10289=CARTESIAN_POINT ( 'NONE',  ( -8.685887942688706786, 232.2448905601785043, -2.449293598294705724E-15 ) ) ;
#10290=CARTESIAN_POINT ( 'NONE',  ( -8.685887942688726326, 386.9948905765655809, -2.449293598294705724E-15 ) ) ;
#10291=CARTESIAN_POINT ( 'NONE',  ( -16.84014894278199748, 420.1198905683720000, -11.84573899990672707 ) ) ;
#10292=CARTESIAN_POINT ( 'NONE',  ( -45.43829269268869098, 265.6823905683720568, 3.332260488124734632 ) ) ;
#10293=CARTESIAN_POINT ( 'NONE',  ( -11.93348319268872793, 418.8698905683720568, -2.051577885510841163E-15 ) ) ;
#10294=CARTESIAN_POINT ( 'NONE',  ( -11.73070664223724791, 356.0573905765655809, 11.32908994701042005 ) ) ;
#10295=CARTESIAN_POINT ( 'NONE',  ( -48.68588794268853803, 276.9323905601784759, -3.978247347593583783 ) ) ;
#10296=CARTESIAN_POINT ( 'NONE',  ( -22.27502019258948351, 320.7448905683720000, -15.47720386886985544 ) ) ;
#10297=CARTESIAN_POINT ( 'NONE',  ( -36.33955658999052218, 490.1198905765656377, -18.47759065022572855 ) ) ;
#10298=CARTESIAN_POINT ( 'NONE',  ( -40.53162694259545162, 486.6198905683720000, 11.84573899990672885 ) ) ;
#10302=CARTESIAN_POINT ( 'NONE',  ( -19.19641293061498999, 391.9323905683720000, -14.20200298773971603 ) ) ;
#10304=CARTESIAN_POINT ( 'NONE',  ( -28.68588794268873698, 524.7448905601785327, -19.99999999999999289 ) ) ;
#10305=CARTESIAN_POINT ( 'NONE',  ( -14.48388495494899963, 359.8073905683720000, -9.489475012073736337 ) ) ;
#10308=CARTESIAN_POINT ( 'NONE',  ( -28.68588794268873343, 526.3698905683720568, 16.75240474999999307 ) ) ;
#10309=VERTEX_POINT ( 'NONE', #13516 ) ;
#10310=CARTESIAN_POINT ( 'NONE',  ( -8.685887942688720997, 352.2448905601784759, -2.449293598294705724E-15 ) ) ;
#10311=CARTESIAN_POINT ( 'NONE',  ( -25.35362745456401257, 521.0573905683720568, -16.75240474999999307 ) ) ;
#10313=CARTESIAN_POINT ( 'NONE',  ( -14.54375231895778597, 493.4948905601784759, -14.14213562373094746 ) ) ;
#10314=CARTESIAN_POINT ( 'NONE',  ( -28.68588794268872633, 476.3698905683720568, 16.75240474999999307 ) ) ;
#10316=CARTESIAN_POINT ( 'NONE',  ( -11.93348319268873681, 488.8698905683720568, -2.051577885510841163E-15 ) ) ;
#10317=CARTESIAN_POINT ( 'NONE',  ( -11.73070664223726212, 491.3073905601784759, 11.32908994701042005 ) ) ;
#10318=EDGE_CURVE ( 'NONE', #16131, #19239, #1434, .T. ) ;
#10319=CARTESIAN_POINT ( 'NONE',  ( -42.82802356641966668, 433.2448905765656377, 14.14213562373094923 ) ) ;
#10320=CARTESIAN_POINT ( 'NONE',  ( -10.20829729246297823, 297.6198905765656377, -7.653668647301794969 ) ) ;
#10322=CARTESIAN_POINT ( 'NONE',  ( -36.33955658999051508, 440.1198905765656377, -18.47759065022572855 ) ) ;
#10328=CARTESIAN_POINT ( 'NONE',  ( -22.27502019258946930, 298.4948905683720568, 15.47720386886985189 ) ) ;
#10330=CARTESIAN_POINT ( 'NONE',  ( -16.84014894278199748, 449.1198905683720568, 11.84573899990672530 ) ) ;
#10332=CARTESIAN_POINT ( 'NONE',  ( -32.01814843081344009, 277.5573905683720000, 16.75240474999999307 ) ) ;
#10334=CARTESIAN_POINT ( 'NONE',  ( -17.35679799567827786, 270.6823905601785327, 16.95518130045146421 ) ) ;
#10335=EDGE_CURVE ( 'NONE', #15878, #19602, #9443, .T. ) ;
#10336=CARTESIAN_POINT ( 'NONE',  ( -19.19641293061499709, 498.8073905683720568, 14.20200298773971426 ) ) ;
#10338=VERTEX_POINT ( 'NONE', #7171 ) ;
#10339=CARTESIAN_POINT ( 'NONE',  ( -35.09675569278796559, 467.2448905683720568, 15.47720386886985366 ) ) ;
#10341=CARTESIAN_POINT ( 'NONE',  ( -14.48388495494898542, 257.9323905683720568, 9.489475012073732785 ) ) ;
#10344=EDGE_CURVE ( 'NONE', #8850, #6325, #17039, .T. ) ;
#10345=CARTESIAN_POINT ( 'NONE',  ( -32.01814843081343298, 267.5573905683720000, 16.75240474999999307 ) ) ;
#10346=CARTESIAN_POINT ( 'NONE',  ( -36.33955658999052218, 490.1198905765656377, -18.47759065022572855 ) ) ;
#10347=CARTESIAN_POINT ( 'NONE',  ( -21.03221929538691271, 390.3698905601785327, 18.47759065022572500 ) ) ;
#10348=CARTESIAN_POINT ( 'NONE',  ( -28.68588794268869790, 247.8698905683720000, 16.75240474999999307 ) ) ;
#10350=CARTESIAN_POINT ( 'NONE',  ( -21.03221929538690915, 234.1198905601784475, -18.47759065022572855 ) ) ;
#10351=CARTESIAN_POINT ( 'NONE',  ( -40.53162694259542320, 242.6198905683720284, -11.84573899990672707 ) ) ;
#10352=CARTESIAN_POINT ( 'NONE',  ( -16.84014894278199037, 361.6198905683720000, -11.84573899990672707 ) ) ;
#10355=CARTESIAN_POINT ( 'NONE',  ( -13.20868407381886556, 399.4948905683720000, -6.410867750099233042 ) ) ;
#10357=CARTESIAN_POINT ( 'NONE',  ( -32.66413529028188378, 409.4323905601784759, 19.99999999999999289 ) ) ;
#10359=CARTESIAN_POINT ( 'NONE',  ( -28.68588794268871567, 349.4948905765656377, -19.99999999999999289 ) ) ;
#10362=FACE_OUTER_BOUND ( 'NONE', #18220, .T. ) ;
#10363=CARTESIAN_POINT ( 'NONE',  ( -36.33955658999050797, 289.1198905601785327, 18.47759065022572500 ) ) ;
#10364=CARTESIAN_POINT ( 'NONE',  ( -10.20829729246298001, 317.6198905765655809, -7.653668647301794969 ) ) ;
#10365=EDGE_CURVE ( 'NONE', #6110, #1587, #2258, .T. ) ;
#10366=CARTESIAN_POINT ( 'NONE',  ( -45.43829269268870519, 315.0573905683720000, -3.332260488124726638 ) ) ;
#10368=EDGE_LOOP ( 'NONE', ( #10154, #19681, #13910, #2429, #19114, #4473, #6305, #20890, #6083, #10984, #18278, #17772, #677, #19368, #17509, #18584, #3234, #9578, #10491, #21159, #8080, #12909, #4704, #15875, #4009, #9851, #13426, #20219, #16305, #5398, #4654, #9362, #16733, #9037, #9727, #6374, #13656, #5188, #1505, #10553, #1664, #10654, #5873, #7547, #14755, #7520, #8449, #20839, #19401, #21342, #16406, #1578, #19393, #21286, #20458, #9571, #12622, #8045, #10574, #8933, #3483, #3936, #6015, #2883, #13842 ) ) ;
#10369=CARTESIAN_POINT ( 'NONE',  ( -32.01814843081344719, 341.6823905683720000, -16.75240474999999307 ) ) ;
#10370=CARTESIAN_POINT ( 'NONE',  ( -16.84014894278198682, 357.6198905683720000, 11.84573899990672530 ) ) ;
#10371=AXIS2_PLACEMENT_3D ( 'NONE', #2252, #10136, #2144 ) ;
#10372=CARTESIAN_POINT ( 'NONE',  ( -10.20829729246297646, 276.3698905765656377, 7.653668647301790529 ) ) ;
#10375=CARTESIAN_POINT ( 'NONE',  ( -28.68588794268870146, 266.3698905683720000, 16.75240474999999307 ) ) ;
#10376=CARTESIAN_POINT ( 'NONE',  ( -10.20829729246299777, 466.3698905765656377, 7.653668647301790529 ) ) ;
#10378=CARTESIAN_POINT ( 'NONE',  ( -13.20868407381886556, 410.9948905683720000, -6.410867750099233042 ) ) ;
#10380=CARTESIAN_POINT ( 'NONE',  ( -45.64106924314020119, 502.9323905765656946, 11.32908994701042538 ) ) ;
#10381=( BOUNDED_CURVE ( )  B_SPLINE_CURVE ( 2, ( #17131, #10295, #20262, #18420, #16709, #15408, #16918, #5227, #7054, #20161, #13778, #6843, #2100, #5432, #18312, #12033, #8466 ),
 .UNSPECIFIED., .F., .T. ) 
 B_SPLINE_CURVE_WITH_KNOTS ( ( 3, 2, 2, 2, 2, 2, 2, 2, 3 ),
 ( 0.8125000000000002220, 0.8144531250000002220, 0.8164062500000002220, 0.8183593750000002220, 0.8203125000000002220, 0.8222656250000002220, 0.8242187500000002220, 0.8261718750000002220, 0.8281250000000002220 ),
 .UNSPECIFIED. ) 
 CURVE ( )  GEOMETRIC_REPRESENTATION_ITEM ( )  RATIONAL_B_SPLINE_CURVE ( ( 0.9999999999999977796, 0.9807852804032326510, 1.000000000000000000, 0.9807852804032304306, 1.000000000000000000, 0.9807852804032304306, 1.000000000000000000, 0.9807852804032304306, 1.000000000000000000, 0.9807852804032304306, 1.000000000000000000, 0.9807852804032304306, 1.000000000000000000, 0.9807852804032304306, 1.000000000000000000, 0.9807852804032282101, 1.000000000000002220 ) ) 
 REPRESENTATION_ITEM ( '' )  );
#10383=CARTESIAN_POINT ( 'NONE',  ( -35.09675569278794427, 285.7448905683720568, 15.47720386886985366 ) ) ;
#10384=CARTESIAN_POINT ( 'NONE',  ( -28.68588794268871212, 322.8698905683720000, -16.75240474999999307 ) ) ;
#10385=CARTESIAN_POINT ( 'NONE',  ( -11.93348319268873503, 468.8698905683720000, -2.051577885510841163E-15 ) ) ;
#10387=CARTESIAN_POINT ( 'NONE',  ( -48.68588794268872277, 466.9323905601785327, -3.978247347593158345 ) ) ;
#10388=CARTESIAN_POINT ( 'NONE',  ( -16.84014894278197971, 287.6198905683720000, 11.84573899990672530 ) ) ;
#10393=CARTESIAN_POINT ( 'NONE',  ( -47.16347859291444422, 337.8698905601785327, 7.653668647301805628 ) ) ;
#10394=CARTESIAN_POINT ( 'NONE',  ( -16.84014894278197971, 307.6198905683720000, 11.84573899990672530 ) ) ;
#10395=CARTESIAN_POINT ( 'NONE',  ( -35.09675569278795138, 377.2448905683720000, 15.47720386886985366 ) ) ;
#10397=CARTESIAN_POINT ( 'NONE',  ( -47.16347859291446554, 522.6198905765655809, 7.653668647301805628 ) ) ;
#10398=CARTESIAN_POINT ( 'NONE',  ( -32.01814843081345430, 411.6823905683720568, -16.75240474999999307 ) ) ;
#10399=CARTESIAN_POINT ( 'NONE',  ( -32.01814843081343298, 267.5573905683720000, 16.75240474999999307 ) ) ;
#10401=CARTESIAN_POINT ( 'NONE',  ( -22.27502019258948351, 416.9948905683720000, 15.47720386886985189 ) ) ;
#10404=CARTESIAN_POINT ( 'NONE',  ( -42.82802356641965957, 370.7448905765656377, -14.14213562373094746 ) ) ;
#10406=CARTESIAN_POINT ( 'NONE',  ( -44.16309181155855867, 324.4948905683720568, 6.410867750099241924 ) ) ;
#10407=CARTESIAN_POINT ( 'NONE',  ( -32.01814843081346140, 477.5573905683720568, 16.75240474999999307 ) ) ;
#10410=CARTESIAN_POINT ( 'NONE',  ( -24.70764059509552979, 224.8073905765656662, 19.99999999999998934 ) ) ;
#10411=CARTESIAN_POINT ( 'NONE',  ( -11.93348319268872260, 380.6823905683720568, -3.332260488124732856 ) ) ;
#10413=CARTESIAN_POINT ( 'NONE',  ( -36.33955658999052929, 535.3698905601784190, -18.47759065022572855 ) ) ;
#10414=CARTESIAN_POINT ( 'NONE',  ( -22.27502019258947286, 336.9948905683720000, 15.47720386886985189 ) ) ;
#10416=CARTESIAN_POINT ( 'NONE',  ( -13.20868407381887799, 518.2448905683720568, 6.410867750099229490 ) ) ;
#10418=CARTESIAN_POINT ( 'NONE',  ( -14.54375231895776821, 353.4948905601785327, -14.14213562373094746 ) ) ;
#10421=CARTESIAN_POINT ( 'NONE',  ( -42.82802356641965247, 290.7448905765655809, -14.14213562373094746 ) ) ;
#10422=CARTESIAN_POINT ( 'NONE',  ( -42.82802356641967378, 495.9948905601784759, -14.14213562373094746 ) ) ;
#10423=CARTESIAN_POINT ( 'NONE',  ( -45.43829269268871940, 483.5573905683720000, -3.332260488124726194 ) ) ;
#10426=CARTESIAN_POINT ( 'NONE',  ( -35.09675569278796559, 495.7448905683720000, 15.47720386886985366 ) ) ;
#10427=CARTESIAN_POINT ( 'NONE',  ( -17.35679799567830273, 490.6823905601784190, 16.95518130045146421 ) ) ;
#10428=CARTESIAN_POINT ( 'NONE',  ( -10.20829729246299244, 417.6198905765656377, -7.653668647301794969 ) ) ;
#10430=CARTESIAN_POINT ( 'NONE',  ( -8.685887942688736985, 486.9948905765656377, -2.449293598294705724E-15 ) ) ;
#10431=CARTESIAN_POINT ( 'NONE',  ( -8.685887942688738761, 506.9948905765655240, -2.449293598294705724E-15 ) ) ;
#10432=CARTESIAN_POINT ( 'NONE',  ( -8.685887942688848895, 486.6823905765656946, 3.978247347593427907 ) ) ;
#10433=DIRECTION ( 'NONE',  ( -1.191790137725560488E-16, 1.000000000000000000, -0.000000000000000000 ) ) ;
#10437=CARTESIAN_POINT ( 'NONE',  ( -14.48388495494899075, 281.3073905683720000, -9.489475012073736337 ) ) ;
#10438=CARTESIAN_POINT ( 'NONE',  ( -17.35679799567827786, 250.6823905601785043, 16.95518130045146421 ) ) ;
#10440=CARTESIAN_POINT ( 'NONE',  ( -13.20868407381887089, 440.9948905683720568, -6.410867750099233042 ) ) ;
#10442=CARTESIAN_POINT ( 'NONE',  ( -19.19641293061497223, 278.8073905683720000, 14.20200298773971426 ) ) ;
#10445=CARTESIAN_POINT ( 'NONE',  ( -32.01814843081345430, 493.1823905683721136, -16.75240474999999307 ) ) ;
#10450=CARTESIAN_POINT ( 'NONE',  ( -11.93348319268871016, 268.8698905683720000, -2.051577885510841163E-15 ) ) ;
#10454=CARTESIAN_POINT ( 'NONE',  ( -28.68588794268872633, 484.4948905765656377, 19.99999999999999289 ) ) ;
#10455=CARTESIAN_POINT ( 'NONE',  ( -40.01497788969913216, 388.8073905601784759, 16.95518130045146776 ) ) ;
#10456=CARTESIAN_POINT ( 'NONE',  ( -22.27502019258947286, 242.2448905683720000, -15.47720386886985544 ) ) ;
#10457=CARTESIAN_POINT ( 'NONE',  ( -42.88789093042845479, 514.4323905683720568, -9.489475012073736337 ) ) ;
#10459=CARTESIAN_POINT ( 'NONE',  ( -44.16309181155855867, 243.2448905683720000, -6.410867750099231266 ) ) ;
#10460=CARTESIAN_POINT ( 'NONE',  ( -32.01814843081344719, 357.5573905683720000, 16.75240474999999307 ) ) ;
#10462=CARTESIAN_POINT ( 'NONE',  ( -32.66413529028186247, 279.4323905601785327, 19.99999999999999289 ) ) ;
#10464=CARTESIAN_POINT ( 'NONE',  ( -11.93348319268872615, 409.1823905683720568, -3.332260488124732856 ) ) ;
#10466=CARTESIAN_POINT ( 'NONE',  ( -24.70764059509556887, 414.4323905601785327, -19.99999999999999289 ) ) ;
#10467=EDGE_LOOP ( 'NONE', ( #17949, #14537, #1110, #12379, #19960, #13877, #13590 ) ) ;
#10471=CARTESIAN_POINT ( 'NONE',  ( -22.27502019258950483, 532.2448905683720568, -15.47720386886985544 ) ) ;
#10472=CARTESIAN_POINT ( 'NONE',  ( -10.20829729246297646, 292.8698905601784759, -7.653668647301794969 ) ) ;
#10476=CARTESIAN_POINT ( 'NONE',  ( -16.84014894278198682, 331.6198905683720000, -11.84573899990672707 ) ) ;
#10477=CARTESIAN_POINT ( 'NONE',  ( -11.93348319268872260, 349.1823905683720000, -3.332260488124732856 ) ) ;
#10478=CARTESIAN_POINT ( 'NONE',  ( -14.48388495494900141, 369.8073905683720000, -9.489475012073734561 ) ) ;
#10481=CARTESIAN_POINT ( 'NONE',  ( -28.68588794268870146, 284.4948905765656377, 19.99999999999999289 ) ) ;
#10483=CARTESIAN_POINT ( 'NONE',  ( -44.16309181155856578, 273.2448905683720568, -6.410867750099231266 ) ) ;
#10484=CARTESIAN_POINT ( 'NONE',  ( -32.01814843081345430, 427.5573905683720000, 16.75240474999999307 ) ) ;
#10487=DIRECTION ( 'NONE',  ( -1.000000000000000000, 0.000000000000000000, 0.000000000000000000 ) ) ;
#10489=CARTESIAN_POINT ( 'NONE',  ( -40.53162694259543031, 326.6198905683720568, 11.84573899990672885 ) ) ;
#10490=CARTESIAN_POINT ( 'NONE',  ( -19.19641293061498999, 457.3073905683720568, 14.20200298773971426 ) ) ;
#10491=ORIENTED_EDGE ( 'NONE', *, *, #7877, .F. ) ;
#10492=CARTESIAN_POINT ( 'NONE',  ( -24.70764059509556176, 460.0573905601784759, 19.99999999999998934 ) ) ;
#10493=CARTESIAN_POINT ( 'NONE',  ( -40.53162694259543031, 285.1198905683720568, 11.84573899990672885 ) ) ;
#10495=ORIENTED_EDGE ( 'NONE', *, *, #4464, .F. ) ;
#10496=CARTESIAN_POINT ( 'NONE',  ( -28.68588794268870856, 339.7448905601784759, 19.99999999999999289 ) ) ;
#10497=CARTESIAN_POINT ( 'NONE',  ( -25.35362745456399125, 448.1823905683720000, 16.75240474999998952 ) ) ;
#10499=FACE_OUTER_BOUND ( 'NONE', #20414, .T. ) ;
#10500=CARTESIAN_POINT ( 'NONE',  ( -17.35679799567829562, 343.8073905601785327, -16.95518130045146421 ) ) ;
#10501=CARTESIAN_POINT ( 'NONE',  ( -35.09675569278793716, 291.9948905683720000, -15.47720386886985544 ) ) ;
#10502=CARTESIAN_POINT ( 'NONE',  ( -40.53162694259543741, 376.6198905683720568, 11.84573899990672885 ) ) ;
#10503=CARTESIAN_POINT ( 'NONE',  ( -8.685887942688738761, 512.2448905601784190, -2.449293598294705724E-15 ) ) ;
#10504=CARTESIAN_POINT ( 'NONE',  ( -36.33955658999052929, 520.1198905765655809, -18.47759065022572855 ) ) ;
#10505=CARTESIAN_POINT ( 'NONE',  ( -13.20868407381886378, 398.2448905683720568, 6.410867750099229490 ) ) ;
#10506=CARTESIAN_POINT ( 'NONE',  ( -22.27502019258947286, 232.2448905683720000, -15.47720386886985544 ) ) ;
#10507=CARTESIAN_POINT ( 'NONE',  ( -38.17536295476245556, 435.4323905683720568, 14.20200298773971781 ) ) ;
#10508=CARTESIAN_POINT ( 'NONE',  ( -36.33955658999051508, 333.8698905765656377, 18.47759065022572500 ) ) ;
#10510=CARTESIAN_POINT ( 'NONE',  ( -38.17536295476244845, 322.3073905683720568, -14.20200298773971426 ) ) ;
#10511=CARTESIAN_POINT ( 'NONE',  ( -25.35362745456400546, 482.5573905683720000, -16.75240474999999307 ) ) ;
#10515=CARTESIAN_POINT ( 'NONE',  ( -45.43829269268870519, 385.6823905683720000, 3.332260488124734632 ) ) ;
#10517=EDGE_CURVE ( 'NONE', #15177, #20201, #19386, .T. ) ;
#10518=CARTESIAN_POINT ( 'NONE',  ( -48.68588794268872988, 526.9323905601785327, -3.978247347593158345 ) ) ;
#10519=CARTESIAN_POINT ( 'NONE',  ( -44.16309181155856578, 344.4948905683720000, 6.410867750099241924 ) ) ;
#10521=CARTESIAN_POINT ( 'NONE',  ( -13.20868407381887799, 499.4948905683720568, -6.410867750099233042 ) ) ;
#10523=CARTESIAN_POINT ( 'NONE',  ( -39.39453070547082802, 223.9102039777117170, -12.89991794593033525 ) ) ;
#10525=CARTESIAN_POINT ( 'NONE',  ( -48.68588794268860909, 291.6823905765655809, -3.978247347593371508 ) ) ;
#10526=CARTESIAN_POINT ( 'NONE',  ( -47.16347859291446554, 521.3698905765655809, -7.653668647301793193 ) ) ;
#10527=CARTESIAN_POINT ( 'NONE',  ( -16.84014894278200458, 470.1198905683720568, -11.84573899990672707 ) ) ;
#10529=CARTESIAN_POINT ( 'NONE',  ( -14.48388495494901385, 489.8073905683720568, -9.489475012073734561 ) ) ;
#10530=CARTESIAN_POINT ( 'NONE',  ( -10.20829729246297291, 251.6198905601784759, 7.653668647301790529 ) ) ;
#10532=CARTESIAN_POINT ( 'NONE',  ( -14.54375231895777176, 405.7448905765656377, 14.14213562373094568 ) ) ;
#10533=CARTESIAN_POINT ( 'NONE',  ( -47.16347859291445843, 472.6198905765656377, 7.653668647301805628 ) ) ;
#10535=CARTESIAN_POINT ( 'NONE',  ( -21.03221929538693757, 484.1198905601785327, -18.47759065022572855 ) ) ;
#10539=DIRECTION ( 'NONE',  ( -1.000000000000000000, 0.000000000000000000, 0.000000000000000000 ) ) ;
#10542=CARTESIAN_POINT ( 'NONE',  ( -14.48388495494898898, 271.3073905683720568, -9.489475012073736337 ) ) ;
#10543=CARTESIAN_POINT ( 'NONE',  ( -48.68588794268869435, 246.9323905601784759, -3.978247347593158345 ) ) ;
#10544=CARTESIAN_POINT ( 'NONE',  ( -28.68588794268871212, 364.4948905765656377, 19.99999999999999289 ) ) ;
#10546=CARTESIAN_POINT ( 'NONE',  ( -22.27502019258948707, 438.4948905683720568, 15.47720386886985189 ) ) ;
#10547=CARTESIAN_POINT ( 'NONE',  ( -45.64106924314017988, 331.0573905765655809, -11.32908994701042538 ) ) ;
#10548=CARTESIAN_POINT ( 'NONE',  ( -25.35362745456396993, 278.1823905683720000, 16.75240474999998952 ) ) ;
#10552=CARTESIAN_POINT ( 'NONE',  ( -25.35362745456400901, 492.5573905683721136, -16.75240474999999307 ) ) ;
#10553=ORIENTED_EDGE ( 'NONE', *, *, #13854, .F. ) ;
#10554=CARTESIAN_POINT ( 'NONE',  ( -28.68588794268874054, 573.2448905601785327, 0.000000000000000000 ) ) ;
#10555=CARTESIAN_POINT ( 'NONE',  ( -11.93348319268870661, 248.8698905683720000, -2.051577885510841163E-15 ) ) ;
#10556=ORIENTED_EDGE ( 'NONE', *, *, #16983, .T. ) ;
#10558=CARTESIAN_POINT ( 'NONE',  ( -40.01497788969915348, 490.4323905765655809, -16.95518130045146421 ) ) ;
#10559=CARTESIAN_POINT ( 'NONE',  ( -32.66413529028186957, 389.4323905601784759, 19.99999999999999289 ) ) ;
#10560=CARTESIAN_POINT ( 'NONE',  ( -47.16347859291445843, 456.6198905601784759, -7.653668647301793193 ) ) ;
#10561=CARTESIAN_POINT ( 'NONE',  ( -16.84014894278196905, 229.1198905683720000, 11.84573899990672530 ) ) ;
#10562=CARTESIAN_POINT ( 'NONE',  ( -32.01814843081346851, 523.1823905683720568, -16.75240474999999307 ) ) ;
#10564=CARTESIAN_POINT ( 'NONE',  ( -14.48388495494898365, 247.9323905683720284, 9.489475012073732785 ) ) ;
#10565=CARTESIAN_POINT ( 'NONE',  ( -40.53162694259543741, 344.1198905683720568, -11.84573899990672707 ) ) ;
#10566=CARTESIAN_POINT ( 'NONE',  ( -21.03221929538690560, 320.3698905601785327, 18.47759065022572500 ) ) ;
#10568=CARTESIAN_POINT ( 'NONE',  ( -16.84014894278199392, 400.1198905683720000, -11.84573899990672707 ) ) ;
#10569=CARTESIAN_POINT ( 'NONE',  ( -45.64106924314017277, 322.9323905765655809, 11.32908994701042538 ) ) ;
#10570=CARTESIAN_POINT ( 'NONE',  ( -17.35679799567829562, 380.6823905601784759, 16.95518130045146421 ) ) ;
#10572=EDGE_LOOP ( 'NONE', ( #16853, #10237, #15794, #12099 ) ) ;
#10573=DIRECTION ( 'NONE',  ( -1.000000000000000000, 0.000000000000000000, 0.000000000000000000 ) ) ;
#10574=ORIENTED_EDGE ( 'NONE', *, *, #18795, .F. ) ;
#10576=CARTESIAN_POINT ( 'NONE',  ( -45.43829269268872650, 505.3698905683721136, 0.000000000000000000 ) ) ;
#10577=CARTESIAN_POINT ( 'NONE',  ( -8.685887942688717445, 316.9948905765655809, -2.449293598294705724E-15 ) ) ;
#10579=CARTESIAN_POINT ( 'NONE',  ( -16.84014894278197971, 309.1198905683720000, 11.84573899990672530 ) ) ;
#10580=ORIENTED_EDGE ( 'NONE', *, *, #2055, .F. ) ;
#10581=CARTESIAN_POINT ( 'NONE',  ( -45.43829269268870519, 354.1823905683721136, 3.332260488124734632 ) ) ;
#10582=CARTESIAN_POINT ( 'NONE',  ( -45.43829269268871229, 353.8698905683720568, 0.000000000000000000 ) ) ;
#10585=CARTESIAN_POINT ( 'NONE',  ( -40.01497788969912506, 283.5573905765655809, 16.95518130045146776 ) ) ;
#10586=CARTESIAN_POINT ( 'NONE',  ( -40.01497788969915348, 500.4323905765656377, -16.95518130045146421 ) ) ;
#10587=CARTESIAN_POINT ( 'NONE',  ( -42.88789093042841927, 242.9323905683720000, -9.489475012073734561 ) ) ;
#10588=CARTESIAN_POINT ( 'NONE',  ( -14.54375231895777887, 465.7448905765655809, 14.14213562373094568 ) ) ;
#10589=CARTESIAN_POINT ( 'NONE',  ( -45.43829269268871229, 405.0573905683721136, -3.332260488124726194 ) ) ;
#10591=CARTESIAN_POINT ( 'NONE',  ( -48.68588794268870146, 277.2448905601784759, 0.000000000000000000 ) ) ;
#10592=CARTESIAN_POINT ( 'NONE',  ( -21.03221929538692336, 354.1198905601785327, -18.47759065022572855 ) ) ;
#10594=CARTESIAN_POINT ( 'NONE',  ( -14.48388495494899431, 311.3073905683720568, -9.489475012073736337 ) ) ;
#10595=CARTESIAN_POINT ( 'NONE',  ( -40.53162694259545162, 465.1198905683720568, 11.84573899990672885 ) ) ;
#10597=CARTESIAN_POINT ( 'NONE',  ( -21.03221929538692336, 470.3698905601784759, 18.47759065022572500 ) ) ;
#10598=CARTESIAN_POINT ( 'NONE',  ( -35.09675569278794427, 285.7448905683720568, 15.47720386886985366 ) ) ;
#10602=CARTESIAN_POINT ( 'NONE',  ( -48.68588794268887199, 337.5573905601784190, 3.978247347592742678 ) ) ;
#10606=CARTESIAN_POINT ( 'NONE',  ( -32.66413529028187668, 345.0573905601784759, -19.99999999999999289 ) ) ;
#10607=CARTESIAN_POINT ( 'NONE',  ( -32.01814843081344009, 306.0573905683720000, 16.75240474999999307 ) ) ;
#10609=CARTESIAN_POINT ( 'NONE',  ( -35.09675569278795138, 393.4948905683720000, -15.47720386886985544 ) ) ;
#10611=CARTESIAN_POINT ( 'NONE',  ( -47.16347859291446554, 521.3698905765655809, -7.653668647301793193 ) ) ;
#10612=CARTESIAN_POINT ( 'NONE',  ( -42.88789093042844058, 394.8073905683720000, 9.489475012073736337 ) ) ;
#10613=CARTESIAN_POINT ( 'NONE',  ( -13.20868407381884602, 249.7448905683720000, 6.410867750099229490 ) ) ;
#10614=CARTESIAN_POINT ( 'NONE',  ( -22.27502019258949417, 410.7448905683720568, -15.47720386886985544 ) ) ;
#10617=CARTESIAN_POINT ( 'NONE',  ( -42.82802356641965957, 340.7448905765655809, -14.14213562373094746 ) ) ;
#10619=CARTESIAN_POINT ( 'NONE',  ( -11.93348319268871549, 308.5573905683719431, 3.332260488124728859 ) ) ;
#10620=CARTESIAN_POINT ( 'NONE',  ( -13.20868407381887444, 470.9948905683720000, -6.410867750099233042 ) ) ;
#10621=CARTESIAN_POINT ( 'NONE',  ( -14.54375231895778597, 515.7448905765655809, 14.14213562373094568 ) ) ;
#10623=CARTESIAN_POINT ( 'NONE',  ( -28.68588794268870856, 304.7448905601785327, -19.99999999999999289 ) ) ;
#10624=CARTESIAN_POINT ( 'NONE',  ( -22.27502019258949062, 392.2448905683720568, -15.47720386886985544 ) ) ;
#10626=CARTESIAN_POINT ( 'NONE',  ( -11.73070664223726922, 523.1823905601784190, -11.32908994701042715 ) ) ;
#10627=CARTESIAN_POINT ( 'NONE',  ( -35.09675569278795138, 335.7448905683720568, 15.47720386886985366 ) ) ;
#10628=ORIENTED_EDGE ( 'NONE', *, *, #4648, .F. ) ;
#10629=CARTESIAN_POINT ( 'NONE',  ( -44.16309181155857999, 504.4948905683720568, 6.410867750099241924 ) ) ;
#10631=CARTESIAN_POINT ( 'NONE',  ( -10.20829729246298356, 352.8698905601784759, -7.653668647301794969 ) ) ;
#10635=CARTESIAN_POINT ( 'NONE',  ( -24.70764059509557953, 519.1823905765655809, -19.99999999999999289 ) ) ;
#10636=CARTESIAN_POINT ( 'NONE',  ( -28.68588794268872633, 466.3698905683720000, 16.75240474999999307 ) ) ;
#10638=CARTESIAN_POINT ( 'NONE',  ( -19.19641293061499354, 477.3073905683720000, 14.20200298773971426 ) ) ;
#10640=CARTESIAN_POINT ( 'NONE',  ( -40.01497788969913927, 403.5573905765656946, 16.95518130045146776 ) ) ;
#10643=CARTESIAN_POINT ( 'NONE',  ( -48.68588794268872988, 531.9948905765656946, 0.000000000000000000 ) ) ;
#10644=FACE_OUTER_BOUND ( 'NONE', #11489, .T. ) ;
#10646=CARTESIAN_POINT ( 'NONE',  ( -45.43829269268869808, 285.0573905683720000, -3.332260488124726194 ) ) ;
#10648=CARTESIAN_POINT ( 'NONE',  ( -42.82802356641964536, 245.9948905601784759, -14.14213562373094746 ) ) ;
#10649=CARTESIAN_POINT ( 'NONE',  ( -40.01497788969913927, 403.5573905765656946, 16.95518130045146776 ) ) ;
#10650=CARTESIAN_POINT ( 'NONE',  ( -44.16309181155857999, 444.7448905683720000, -6.410867750099231266 ) ) ;
#10651=CARTESIAN_POINT ( 'NONE',  ( -10.20829729246298179, 327.6198905765656377, -7.653668647301794969 ) ) ;
#10652=CARTESIAN_POINT ( 'NONE',  ( -40.53162694259543031, 276.6198905683720568, 11.84573899990672885 ) ) ;
#10653=ORIENTED_EDGE ( 'NONE', *, *, #2752, .T. ) ;
#10654=ORIENTED_EDGE ( 'NONE', *, *, #7630, .F. ) ;
#10655=CARTESIAN_POINT ( 'NONE',  ( -19.19641293061499709, 481.9323905683720000, -14.20200298773971603 ) ) ;
#10659=CARTESIAN_POINT ( 'NONE',  ( -48.68588794268843145, 366.9323905601784190, -3.978247347593797389 ) ) ;
#10660=CARTESIAN_POINT ( 'NONE',  ( -11.93348319268870839, 248.5573905683719715, 3.332260488124728415 ) ) ;
#10664=CARTESIAN_POINT ( 'NONE',  ( -48.68588794268872277, 471.9948905765656377, 0.000000000000000000 ) ) ;
#10665=CARTESIAN_POINT ( 'NONE',  ( -8.685887942688539809, 307.3073905765654672, -3.978247347592740013 ) ) ;
#10666=CARTESIAN_POINT ( 'NONE',  ( -21.03221929538693402, 454.1198905601784759, -18.47759065022572855 ) ) ;
#10667=CARTESIAN_POINT ( 'NONE',  ( -13.20868407381884602, 230.9948905683720284, -6.410867750099233042 ) ) ;
#10668=ADVANCED_FACE ( 'NONE', ( #4977 ), #7995, .T. ) ;
#10669=CARTESIAN_POINT ( 'NONE',  ( -38.17536295476247687, 523.8073905683720568, -14.20200298773971426 ) ) ;
#10671=CARTESIAN_POINT ( 'NONE',  ( -19.19641293061496867, 247.3073905683720284, 14.20200298773971426 ) ) ;
#10672=CARTESIAN_POINT ( 'NONE',  ( -45.43829269268870519, 335.6823905683720568, 3.332260488124734632 ) ) ;
#10673=CARTESIAN_POINT ( 'NONE',  ( -14.54375231895777887, 470.9948905601784759, 14.14213562373094568 ) ) ;
#10674=CARTESIAN_POINT ( 'NONE',  ( -40.01497788969913216, 358.8073905601784190, 16.95518130045146776 ) ) ;
#10675=AXIS2_PLACEMENT_3D ( 'NONE', #1974, #13430, #18494 ) ;
#10676=CARTESIAN_POINT ( 'NONE',  ( -38.17536295476244845, 375.4323905683720568, 14.20200298773971781 ) ) ;
#10677=DIRECTION ( 'NONE',  ( 1.000000000000000000, 0.000000000000000000, -0.000000000000000000 ) ) ;
#10678=CARTESIAN_POINT ( 'NONE',  ( -28.68588794268871567, 389.7448905601785327, 19.99999999999999289 ) ) ;
#10679=ORIENTED_EDGE ( 'NONE', *, *, #453, .T. ) ;
#10680=FACE_OUTER_BOUND ( 'NONE', #20761, .T. ) ;
#10683=CARTESIAN_POINT ( 'NONE',  ( -14.48388495494901562, 509.4323905683719431, 9.489475012073732785 ) ) ;
#10686=CARTESIAN_POINT ( 'NONE',  ( -11.93348319268871549, 310.6823905683720568, -3.332260488124732856 ) ) ;
#10688=CARTESIAN_POINT ( 'NONE',  ( -19.19641293061498644, 350.4323905683720000, -14.20200298773971603 ) ) ;
#10689=CARTESIAN_POINT ( 'NONE',  ( -28.68588794268871567, 351.3698905683720568, -16.75240474999999307 ) ) ;
#10690=CARTESIAN_POINT ( 'NONE',  ( -21.03221929538691271, 278.8698905765656377, -18.47759065022572855 ) ) ;
#10692=CARTESIAN_POINT ( 'NONE',  ( -22.27502019258947286, 240.7448905683720000, -15.47720386886985544 ) ) ;
#10693=CARTESIAN_POINT ( 'NONE',  ( -17.35679799567830273, 465.4323905765656946, 16.95518130045146421 ) ) ;
#10695=CARTESIAN_POINT ( 'NONE',  ( -22.27502019258949062, 402.2448905683720568, -15.47720386886985544 ) ) ;
#10696=DIRECTION ( 'NONE',  ( -1.000000000000000000, 0.000000000000000000, 0.000000000000000000 ) ) ;
#10697=CARTESIAN_POINT ( 'NONE',  ( -28.68588794268871567, 354.7448905601784759, -19.99999999999999289 ) ) ;
#10700=CARTESIAN_POINT ( 'NONE',  ( -22.27502019258949773, 460.7448905683720568, -15.47720386886985544 ) ) ;
#10702=CARTESIAN_POINT ( 'NONE',  ( -28.68588794268872277, 449.7448905601784759, 19.99999999999999289 ) ) ;
#10705=ORIENTED_EDGE ( 'NONE', *, *, #13688, .F. ) ;
#10708=CARTESIAN_POINT ( 'NONE',  ( -32.66413529028186957, 325.0573905601785327, -19.99999999999999289 ) ) ;
#10709=CARTESIAN_POINT ( 'NONE',  ( -22.27502019258946930, 306.9948905683720568, 15.47720386886985189 ) ) ;
#10710=CARTESIAN_POINT ( 'NONE',  ( -11.93348319268872260, 360.0573905683720000, 3.332260488124728859 ) ) ;
#10711=CARTESIAN_POINT ( 'NONE',  ( -11.73070664223724080, 293.1823905601784759, -11.32908994701042538 ) ) ;
#10714=CARTESIAN_POINT ( 'NONE',  ( -14.54375231895778775, 525.7448905765655809, 14.14213562373094568 ) ) ;
#10715=CARTESIAN_POINT ( 'NONE',  ( -45.43829269268871229, 403.5573905683720000, -3.332260488124726194 ) ) ;
#10716=CARTESIAN_POINT ( 'NONE',  ( -16.84014894278197616, 231.6198905683720000, -11.84573899990672707 ) ) ;
#10718=CARTESIAN_POINT ( 'NONE',  ( -45.43829269268871940, 404.1823905683719431, 3.332260488124734632 ) ) ;
#10720=CARTESIAN_POINT ( 'NONE',  ( -48.68588794268870856, 351.9948905765656377, 0.000000000000000000 ) ) ;
#10722=CARTESIAN_POINT ( 'NONE',  ( -45.43829269268870519, 314.1823905683720000, 3.332260488124734632 ) ) ;
#10725=CARTESIAN_POINT ( 'NONE',  ( -38.17536295476246266, 456.9323905683720000, 14.20200298773971781 ) ) ;
#10727=CARTESIAN_POINT ( 'NONE',  ( -48.68588794268873698, 573.2448905601785327, 0.000000000000000000 ) ) ;
#10731=CARTESIAN_POINT ( 'NONE',  ( -44.16309181155856578, 365.9948905683720568, 6.410867750099241924 ) ) ;
#10734=CARTESIAN_POINT ( 'NONE',  ( -48.68588794268872277, 507.5573905601784759, 3.978247347593168115 ) ) ;
#10735=CARTESIAN_POINT ( 'NONE',  ( -13.20868407381885667, 348.2448905683720000, 6.410867750099229490 ) ) ;
#10736=EDGE_CURVE ( 'NONE', #20528, #20871, #8405, .T. ) ;
#10738=CARTESIAN_POINT ( 'NONE',  ( -14.48388495494901562, 507.9323905683720568, 9.489475012073732785 ) ) ;
#10741=CARTESIAN_POINT ( 'NONE',  ( -22.27502019258948351, 418.4948905683720000, 15.47720386886985189 ) ) ;
#10742=CARTESIAN_POINT ( 'NONE',  ( -14.54375231895776110, 288.2448905765656377, -14.14213562373094746 ) ) ;
#10744=CARTESIAN_POINT ( 'NONE',  ( -28.68588794268872988, 471.3698905683720568, -16.75240474999999307 ) ) ;
#10746=CARTESIAN_POINT ( 'NONE',  ( -38.17536295476246977, 462.3073905683720568, -14.20200298773971426 ) ) ;
#10747=CARTESIAN_POINT ( 'NONE',  ( -45.43280446313950449, 223.9102039777116602, 0.4287796227366179602 ) ) ;
#10748=CARTESIAN_POINT ( 'NONE',  ( -11.73070664223725146, 396.0573905765655809, 11.32908994701042005 ) ) ;
#10751=CARTESIAN_POINT ( 'NONE',  ( -32.66413529028186957, 369.8073905765655240, -19.99999999999999289 ) ) ;
#10756=CARTESIAN_POINT ( 'NONE',  ( -47.16347859291443001, 237.8698905601784759, 7.653668647301805628 ) ) ;
#10757=CARTESIAN_POINT ( 'NONE',  ( -42.82802356641964536, 205.1437886375728965, -5.000000000000001776 ) ) ;
#10758=CARTESIAN_POINT ( 'NONE',  ( -38.17536295476244845, 273.8073905683720000, -14.20200298773971426 ) ) ;
#10760=CARTESIAN_POINT ( 'NONE',  ( -32.01814843081345430, 417.5573905683720568, 16.75240474999999307 ) ) ;
#10761=CARTESIAN_POINT ( 'NONE',  ( -36.33955658999050797, 330.1198905765655809, -18.47759065022572855 ) ) ;
#10762=CARTESIAN_POINT ( 'NONE',  ( -28.68588794268870146, 277.8698905683720000, 16.75240474999999307 ) ) ;
#10765=FACE_BOUND ( 'NONE', #20844, .T. ) ;
#10766=EDGE_LOOP ( 'NONE', ( #6861, #13181, #5500, #2707 ) ) ;
#10767=CARTESIAN_POINT ( 'NONE',  ( -42.88789093042844769, 474.4323905683721136, -9.489475012073734561 ) ) ;
#10768=ORIENTED_EDGE ( 'NONE', *, *, #3976, .T. ) ;
#10769=CARTESIAN_POINT ( 'NONE',  ( -21.03221929538692336, 364.1198905601785327, -18.47759065022572855 ) ) ;
#10770=CARTESIAN_POINT ( 'NONE',  ( -11.93348319268870839, 239.1823905683720284, -3.332260488124732856 ) ) ;
#10772=CARTESIAN_POINT ( 'NONE',  ( -32.01814843081346140, 531.6823905683719431, -16.75240474999999307 ) ) ;
#10773=CARTESIAN_POINT ( 'NONE',  ( -48.68588794268870856, 347.2448905601784759, 0.000000000000000000 ) ) ;
#10774=CARTESIAN_POINT ( 'NONE',  ( -8.685887942688735208, 466.9948905765656377, -2.449293598294705724E-15 ) ) ;
#10777=CARTESIAN_POINT ( 'NONE',  ( -25.77425622588650000, 223.9102039777116318, -18.75905995620974309 ) ) ;
#10779=CARTESIAN_POINT ( 'NONE',  ( -11.93348319268873858, 510.0573905683720000, 3.332260488124728415 ) ) ;
#10780=CARTESIAN_POINT ( 'NONE',  ( -48.68588794268872988, 517.2448905601785327, 0.000000000000000000 ) ) ;
#10781=CARTESIAN_POINT ( 'NONE',  ( -13.20868407381884602, 238.2448905683720000, 6.410867750099229490 ) ) ;
#10783=CARTESIAN_POINT ( 'NONE',  ( -19.19641293061498288, 341.9323905683720568, -14.20200298773971603 ) ) ;
#10784=CARTESIAN_POINT ( 'NONE',  ( -21.03221929538692336, 470.3698905601784759, 18.47759065022572500 ) ) ;
#10785=CARTESIAN_POINT ( 'NONE',  ( -42.82802356641965957, 358.4948905601785327, 14.14213562373094923 ) ) ;
#10786=CARTESIAN_POINT ( 'NONE',  ( -38.17536295476246266, 392.3073905683720568, -14.20200298773971426 ) ) ;
#10789=CARTESIAN_POINT ( 'NONE',  ( -36.33955658999051508, 389.1198905601784759, 18.47759065022572500 ) ) ;
#10795=CARTESIAN_POINT ( 'NONE',  ( -11.93348319268873858, 500.6823905683720568, -3.332260488124732856 ) ) ;
#10796=CYLINDRICAL_SURFACE ( 'NONE', #11109, 19.99999999999999645 ) ;
#10797=ORIENTED_EDGE ( 'NONE', *, *, #520, .T. ) ;
#10798=CARTESIAN_POINT ( 'NONE',  ( -28.68588794268870856, 312.8698905683720000, -16.75240474999999307 ) ) ;
#10801=CARTESIAN_POINT ( 'NONE',  ( -11.93348319268872260, 338.5573905683720568, 3.332260488124728415 ) ) ;
#10802=CARTESIAN_POINT ( 'NONE',  ( -40.53162694259543741, 342.6198905683720000, -11.84573899990672707 ) ) ;
#10804=CARTESIAN_POINT ( 'NONE',  ( -17.35679799567828141, 275.4323905765656377, 16.95518130045146421 ) ) ;
#10806=CARTESIAN_POINT ( 'NONE',  ( -19.19641293061496512, 247.3073905683720284, 14.20200298773971426 ) ) ;
#10808=CARTESIAN_POINT ( 'NONE',  ( -14.48388495494900496, 399.4323905683720568, 9.489475012073732785 ) ) ;
#10813=CARTESIAN_POINT ( 'NONE',  ( -38.17536295476246977, 452.3073905683720568, -14.20200298773971426 ) ) ;
#10815=CARTESIAN_POINT ( 'NONE',  ( -40.01497788969913927, 438.8073905601784190, 16.95518130045146776 ) ) ;
#10817=AXIS2_PLACEMENT_3D ( 'NONE', #18907, #13741, #2375 ) ;
#10819=CARTESIAN_POINT ( 'NONE',  ( -32.66413529028186957, 339.4323905601784190, 19.99999999999999289 ) ) ;
#10823=CARTESIAN_POINT ( 'NONE',  ( -21.03221929538690560, 330.3698905601784759, 18.47759065022572500 ) ) ;
#10825=CARTESIAN_POINT ( 'NONE',  ( -11.93348319268872260, 370.3698905683720568, -2.051577885510841163E-15 ) ) ;
#10826=CARTESIAN_POINT ( 'NONE',  ( -45.64106924314016567, 228.1823905601784759, 11.32908994701042538 ) ) ;
#10827=CARTESIAN_POINT ( 'NONE',  ( -48.68588794268872988, 531.9948905765656946, 0.000000000000000000 ) ) ;
#10828=CARTESIAN_POINT ( 'NONE',  ( -14.48388495494900496, 409.8073905683720568, -9.489475012073736337 ) ) ;
#10829=CARTESIAN_POINT ( 'NONE',  ( -40.53162694259542320, 246.6198905683720284, 11.84573899990672885 ) ) ;
#10830=CARTESIAN_POINT ( 'NONE',  ( -16.84014894278199392, 400.1198905683720000, -11.84573899990672707 ) ) ;
#10832=( BOUNDED_CURVE ( )  B_SPLINE_CURVE ( 2, ( #2547, #5888, #6311, #19302, #16070, #11183, #12817, #10751, #938, #15859, #14240, #15751, #7505, #19408, #17464, #14349, #20714 ),
 .UNSPECIFIED., .F., .T. ) 
 B_SPLINE_CURVE_WITH_KNOTS ( ( 3, 2, 2, 2, 2, 2, 2, 2, 3 ),
 ( 0.5000000000000002220, 0.5019531250000002220, 0.5039062500000002220, 0.5058593750000002220, 0.5078125000000002220, 0.5097656250000002220, 0.5117187500000002220, 0.5136718750000002220, 0.5156250000000002220 ),
 .UNSPECIFIED. ) 
 CURVE ( )  GEOMETRIC_REPRESENTATION_ITEM ( )  RATIONAL_B_SPLINE_CURVE ( ( 0.9999999999999977796, 0.9807852804032326510, 1.000000000000000000, 0.9807852804032304306, 1.000000000000000000, 0.9807852804032304306, 1.000000000000000000, 0.9807852804032304306, 1.000000000000000000, 0.9807852804032304306, 1.000000000000000000, 0.9807852804032304306, 1.000000000000000000, 0.9807852804032304306, 1.000000000000000000, 0.9807852804032282101, 1.000000000000002220 ) ) 
 REPRESENTATION_ITEM ( '' )  );
#10833=CARTESIAN_POINT ( 'NONE',  ( -10.20829729246298356, 337.6198905765656377, -7.653668647301794969 ) ) ;
#10835=CARTESIAN_POINT ( 'NONE',  ( -16.84014894278197971, 307.6198905683720000, 11.84573899990672530 ) ) ;
#10837=CARTESIAN_POINT ( 'NONE',  ( -45.43829269268871940, 455.0573905683720568, -3.332260488124726194 ) ) ;
#10841=VECTOR ( 'NONE', #4411, 1000.000000000000000 ) ;
#10842=CARTESIAN_POINT ( 'NONE',  ( -38.17536295476244845, 366.9323905683721136, 14.20200298773971781 ) ) ;
#10843=CARTESIAN_POINT ( 'NONE',  ( -13.20868407381887621, 508.2448905683720568, 6.410867750099229490 ) ) ;
#10844=EDGE_CURVE ( 'NONE', #10139, #11348, #4459, .T. ) ;
#10845=CARTESIAN_POINT ( 'NONE',  ( -17.35679799567831338, 503.8073905601785327, -16.95518130045146421 ) ) ;
#10846=CARTESIAN_POINT ( 'NONE',  ( -25.35362745456399125, 351.0573905683720568, -16.75240474999999307 ) ) ;
#10847=VERTEX_POINT ( 'NONE', #17200 ) ;
#10848=CARTESIAN_POINT ( 'NONE',  ( -25.35362745456400901, 511.0573905683720568, -16.75240474999999307 ) ) ;
#10851=CARTESIAN_POINT ( 'NONE',  ( -25.35362745456398770, 418.1823905683720568, 16.75240474999998952 ) ) ;
#10852=CARTESIAN_POINT ( 'NONE',  ( -21.03221929538691626, 288.8698905765656377, -18.47759065022572855 ) ) ;
#10853=CARTESIAN_POINT ( 'NONE',  ( -8.685887942688628627, 492.5573905601784190, -3.978247347592898553 ) ) ;
#10854=CARTESIAN_POINT ( 'NONE',  ( -11.93348319268873503, 469.1823905683719431, -3.332260488124732856 ) ) ;
#10855=ORIENTED_EDGE ( 'NONE', *, *, #19354, .F. ) ;
#10856=CARTESIAN_POINT ( 'NONE',  ( -22.27502019258949062, 466.9948905683720000, 15.47720386886985189 ) ) ;
#10857=CARTESIAN_POINT ( 'NONE',  ( -45.64106924314019409, 402.9323905765656946, 11.32908994701042715 ) ) ;
#10864=CARTESIAN_POINT ( 'NONE',  ( -42.82802356641964536, 238.4948905601784759, 14.14213562373094923 ) ) ;
#10866=CARTESIAN_POINT ( 'NONE',  ( -14.54375231895775578, 243.4948905601784759, -14.14213562373094746 ) ) ;
#10868=CARTESIAN_POINT ( 'NONE',  ( -25.35362745456399836, 432.5573905683719431, -16.75240474999999307 ) ) ;
#10870=CARTESIAN_POINT ( 'NONE',  ( -38.17536295476243424, 256.9323905683720568, 14.20200298773971781 ) ) ;
#10875=CARTESIAN_POINT ( 'NONE',  ( -38.17536295476246977, 493.8073905683720000, -14.20200298773971426 ) ) ;
#10877=EDGE_LOOP ( 'NONE', ( #9010, #2665, #12775, #8851 ) ) ;
#10878=CARTESIAN_POINT ( 'NONE',  ( -8.685887942688742314, 526.9948905765655809, -2.449293598294705724E-15 ) ) ;
#10879=CARTESIAN_POINT ( 'NONE',  ( -40.53162694259542320, 245.1198905683720284, 11.84573899990672885 ) ) ;
#10881=CARTESIAN_POINT ( 'NONE',  ( -45.43829269268873361, 523.5573905683720568, -3.332260488124726638 ) ) ;
#10886=CARTESIAN_POINT ( 'NONE',  ( -19.19641293061496867, 231.9323905683720000, -14.20200298773971603 ) ) ;
#10888=CARTESIAN_POINT ( 'NONE',  ( -44.16309181155859420, 514.7448905683720568, -6.410867750099231266 ) ) ;
#10889=CARTESIAN_POINT ( 'NONE',  ( -32.66413529028186957, 374.1823905765655809, 19.99999999999999289 ) ) ;
#10890=CARTESIAN_POINT ( 'NONE',  ( -44.16309181155855867, 233.2448905683720000, -6.410867750099231266 ) ) ;
#10891=CARTESIAN_POINT ( 'NONE',  ( -16.84014894278198682, 331.6198905683720000, -11.84573899990672707 ) ) ;
#10893=CARTESIAN_POINT ( 'NONE',  ( -11.73070664223723902, 306.0573905765655809, 11.32908994701042005 ) ) ;
#10894=CARTESIAN_POINT ( 'NONE',  ( -22.27502019258947996, 376.9948905683720568, 15.47720386886985189 ) ) ;
#10895=CARTESIAN_POINT ( 'NONE',  ( -8.685887942688895080, 326.6823905765656377, 3.978247347593586447 ) ) ;
#10896=CARTESIAN_POINT ( 'NONE',  ( -11.73070664223725146, 383.1823905601784759, -11.32908994701042715 ) ) ;
#10901=CARTESIAN_POINT ( 'NONE',  ( -11.93348319268873858, 510.3698905683720000, -2.051577885510841163E-15 ) ) ;
#10902=CARTESIAN_POINT ( 'NONE',  ( -36.33955658999050797, 293.8698905765656377, 18.47759065022572500 ) ) ;
#10903=VERTEX_POINT ( 'NONE', #2379 ) ;
#10904=CARTESIAN_POINT ( 'NONE',  ( -16.84014894278198327, 311.6198905683720000, -11.84573899990672707 ) ) ;
#10906=CARTESIAN_POINT ( 'NONE',  ( -28.68588794268871212, 331.3698905683720000, -16.75240474999999307 ) ) ;
#10907=CARTESIAN_POINT ( 'NONE',  ( -13.20868407381885845, 349.4948905683720000, -6.410867750099233042 ) ) ;
#10908=CARTESIAN_POINT ( 'NONE',  ( -21.03221929538691271, 268.8698905765656377, -18.47759065022572855 ) ) ;
#10909=CARTESIAN_POINT ( 'NONE',  ( -10.20829729246298889, 392.8698905601784759, -7.653668647301794969 ) ) ;
#10910=CARTESIAN_POINT ( 'NONE',  ( -38.17536295476243424, 245.4323905683720284, 14.20200298773971781 ) ) ;
#10911=CARTESIAN_POINT ( 'NONE',  ( -45.43829269268871940, 405.3698905683720000, 0.000000000000000000 ) ) ;
#10912=AXIS2_PLACEMENT_3D ( 'NONE', #254, #17862, #3380 ) ;
#10913=CARTESIAN_POINT ( 'NONE',  ( -10.20829729246298179, 332.8698905601785327, -7.653668647301794969 ) ) ;
#10915=CARTESIAN_POINT ( 'NONE',  ( -47.16347859291443001, 246.6198905601784759, -7.653668647301793193 ) ) ;
#10917=CARTESIAN_POINT ( 'NONE',  ( -45.43829269268871940, 443.8698905683720568, 0.000000000000000000 ) ) ;
#10919=CARTESIAN_POINT ( 'NONE',  ( -11.73070664223726034, 453.1823905601784759, -11.32908994701042715 ) ) ;
#10920=EDGE_CURVE ( 'NONE', #4317, #339, #11781, .T. ) ;
#10922=EDGE_LOOP ( 'NONE', ( #238, #4234, #20379, #3552 ) ) ;
#10923=ORIENTED_EDGE ( 'NONE', *, *, #1759, .T. ) ;
#10925=CARTESIAN_POINT ( 'NONE',  ( -28.68588794268871212, 324.7448905601784759, -19.99999999999999289 ) ) ;
#10928=CARTESIAN_POINT ( 'NONE',  ( -11.93348319268872260, 370.0573905683719431, 3.332260488124728859 ) ) ;
#10930=CARTESIAN_POINT ( 'NONE',  ( -45.64106924314020119, 501.0573905765656377, -11.32908994701042715 ) ) ;
#10931=CARTESIAN_POINT ( 'NONE',  ( -45.43829269268870519, 383.5573905683720000, -3.332260488124726194 ) ) ;
#10932=CARTESIAN_POINT ( 'NONE',  ( -45.43829269268869098, 245.0573905683720000, -3.332260488124726194 ) ) ;
#10933=CARTESIAN_POINT ( 'NONE',  ( -13.20868407381886378, 398.2448905683720568, 6.410867750099229490 ) ) ;
#10935=CARTESIAN_POINT ( 'NONE',  ( -17.35679799567828852, 335.4323905765656377, 16.95518130045146421 ) ) ;
#10937=CARTESIAN_POINT ( 'NONE',  ( -42.88789093042842637, 302.9323905683720568, -9.489475012073734561 ) ) ;
#10938=CARTESIAN_POINT ( 'NONE',  ( -45.43829269268871940, 465.0573905683720000, -3.332260488124726194 ) ) ;
#10944=CARTESIAN_POINT ( 'NONE',  ( -13.20868407381885845, 359.7448905683720568, 6.410867750099229490 ) ) ;
#10945=CARTESIAN_POINT ( 'NONE',  ( -45.43829269268871940, 504.1823905683721136, 3.332260488124734632 ) ) ;
#10946=CARTESIAN_POINT ( 'NONE',  ( -47.16347859291445843, 507.8698905601785327, 7.653668647301805628 ) ) ;
#10947=CARTESIAN_POINT ( 'NONE',  ( -16.84014894278198327, 327.6198905683720000, 11.84573899990672530 ) ) ;
#10948=VECTOR ( 'NONE', #1329, 1000.000000000000000 ) ;
#10949=ORIENTED_EDGE ( 'NONE', *, *, #6691, .T. ) ;
#10950=CARTESIAN_POINT ( 'NONE',  ( -32.01814843081346851, 506.0573905683719431, 16.75240474999999307 ) ) ;
#10952=( BOUNDED_CURVE ( )  B_SPLINE_CURVE ( 2, ( #19151, #20447, #14295, #12229, #12654, #10586, #5620, #994, #9181, #667, #13860, #4103, #13974, #7340, #18812, #1099, #3993 ),
 .UNSPECIFIED., .F., .T. ) 
 B_SPLINE_CURVE_WITH_KNOTS ( ( 3, 2, 2, 2, 2, 2, 2, 2, 3 ),
 ( 0.09375000000000008327, 0.09570312500000011102, 0.09765625000000013878, 0.09960937500000016653, 0.1015625000000001943, 0.1035156250000002082, 0.1054687500000002359, 0.1074218750000002637, 0.1093750000000002914 ),
 .UNSPECIFIED. ) 
 CURVE ( )  GEOMETRIC_REPRESENTATION_ITEM ( )  RATIONAL_B_SPLINE_CURVE ( ( 0.9999999999999992228, 0.9807852804032312077, 1.000000000000000000, 0.9807852804032304306, 1.000000000000000000, 0.9807852804032304306, 1.000000000000000000, 0.9807852804032304306, 1.000000000000000000, 0.9807852804032304306, 1.000000000000000000, 0.9807852804032304306, 1.000000000000000000, 0.9807852804032304306, 1.000000000000000000, 0.9807852804032275440, 1.000000000000002887 ) ) 
 REPRESENTATION_ITEM ( '' )  );
#10953=CARTESIAN_POINT ( 'NONE',  ( -28.68588794268870856, 314.4948905765656377, 19.99999999999999289 ) ) ;
#10954=CARTESIAN_POINT ( 'NONE',  ( -11.93348319268872970, 430.3698905683720568, -2.051577885510841163E-15 ) ) ;
#10955=CARTESIAN_POINT ( 'NONE',  ( -36.33955658999052218, 393.8698905765656377, 18.47759065022572500 ) ) ;
#10957=CARTESIAN_POINT ( 'NONE',  ( -22.27502019258948707, 456.9948905683720000, 15.47720386886985189 ) ) ;
#10959=CARTESIAN_POINT ( 'NONE',  ( -38.17536295476246266, 465.4323905683720568, 14.20200298773971781 ) ) ;
#10963=CARTESIAN_POINT ( 'NONE',  ( -47.16347859291445133, 402.6198905765655809, 7.653668647301805628 ) ) ;
#10965=CARTESIAN_POINT ( 'NONE',  ( -48.68588794268873698, 573.2448905601785327, 0.000000000000000000 ) ) ;
#10970=CARTESIAN_POINT ( 'NONE',  ( -44.28481028704773337, 223.9102039777117454, 9.367795489887496885 ) ) ;
#10971=CARTESIAN_POINT ( 'NONE',  ( -24.70764059509553334, 240.0573905601784759, 19.99999999999998934 ) ) ;
#10972=CARTESIAN_POINT ( 'NONE',  ( -21.03221929538691981, 450.3698905601784759, 18.47759065022572500 ) ) ;
#10973=CARTESIAN_POINT ( 'NONE',  ( -11.93348319268872970, 430.3698905683720568, -2.051577885510841163E-15 ) ) ;
#10974=CARTESIAN_POINT ( 'NONE',  ( -42.82802356641965957, 385.9948905601784759, -14.14213562373094746 ) ) ;
#10975=CARTESIAN_POINT ( 'NONE',  ( -11.93348319268870839, 250.0573905683720000, 3.332260488124728415 ) ) ;
#10978=CARTESIAN_POINT ( 'NONE',  ( -19.19641293061499354, 461.9323905683720568, -14.20200298773971603 ) ) ;
#10979=CARTESIAN_POINT ( 'NONE',  ( -48.68588794268869435, 231.9948905765656377, 0.000000000000000000 ) ) ;
#10980=ADVANCED_FACE ( 'NONE', ( #14288 ), #10796, .T. ) ;
#10981=ORIENTED_EDGE ( 'NONE', *, *, #8300, .T. ) ;
#10982=DIRECTION ( 'NONE',  ( -1.191790137725560488E-16, 1.000000000000000000, -0.000000000000000000 ) ) ;
#10983=CARTESIAN_POINT ( 'NONE',  ( -16.84014894278197616, 240.1198905683720284, -11.84573899990672707 ) ) ;
#10984=ORIENTED_EDGE ( 'NONE', *, *, #14317, .F. ) ;
#10985=CARTESIAN_POINT ( 'NONE',  ( -28.68588794268872988, 516.3698905683720568, 16.75240474999999307 ) ) ;
#10986=CARTESIAN_POINT ( 'NONE',  ( -31.26501780185373391, 205.1437886375728965, -5.000000000000001776 ) ) ;
#10987=CARTESIAN_POINT ( 'NONE',  ( -48.68588794268872277, 461.9948905765656377, 0.000000000000000000 ) ) ;
#10988=CARTESIAN_POINT ( 'NONE',  ( -45.64106924314017988, 348.1823905601784759, 11.32908994701042538 ) ) ;
#10990=CARTESIAN_POINT ( 'NONE',  ( -48.68588794268879383, 282.3073905765656946, 3.978247347592954952 ) ) ;
#10991=CARTESIAN_POINT ( 'NONE',  ( -24.85637767767141426, 223.9102039777116033, -18.72850036933187212 ) ) ;
#10995=CARTESIAN_POINT ( 'NONE',  ( -22.27502019258947286, 230.7448905683720000, -15.47720386886985544 ) ) ;
#10996=CARTESIAN_POINT ( 'NONE',  ( -19.19641293061497933, 328.8073905683720568, 14.20200298773971426 ) ) ;
#10997=CARTESIAN_POINT ( 'NONE',  ( -48.68588794268887199, 317.5573905601785327, 3.978247347592742678 ) ) ;
#10999=CARTESIAN_POINT ( 'NONE',  ( -28.68588794268870856, 302.8698905683720000, -16.75240474999999307 ) ) ;
#11000=CARTESIAN_POINT ( 'NONE',  ( -40.53162694259543741, 382.6198905683720568, -11.84573899990672707 ) ) ;
#11001=CARTESIAN_POINT ( 'NONE',  ( -22.27502019258949773, 528.4948905683719431, 15.47720386886985189 ) ) ;
#11002=CARTESIAN_POINT ( 'NONE',  ( -40.01497788969914637, 395.6823905601784190, -16.95518130045146421 ) ) ;
#11008=CARTESIAN_POINT ( 'NONE',  ( -38.17536295476247687, 513.8073905683720568, -14.20200298773971426 ) ) ;
#11010=B_SPLINE_CURVE_WITH_KNOTS ( 'NONE', 3,
 ( #17314, #7450, #8763, #8650, #18921, #5405, #15700, #18602, #13976, #7027, #562, #15383, #10272, #13649, #886, #5622, #15596, #4105, #20558, #2073, #20234, #12116 ),
 .UNSPECIFIED., .F., .F.,
 ( 4, 2, 2, 2, 2, 2, 2, 2, 2, 2, 4 ),
 ( 0.02361608169583585826, 0.02460001686704672841, 0.02509198445265212185, 0.02558395203825751876, 0.02656788720946830565, 0.02755182238067909600, 0.02853575755188988289, 0.02951969272310067324, 0.03001166030870608403, 0.03050362789431149482, 0.03148756306552229906 ),
 .UNSPECIFIED. ) ;
#11012=CARTESIAN_POINT ( 'NONE',  ( -44.16309181155855867, 295.9948905683720000, 6.410867750099241924 ) ) ;
#11013=CARTESIAN_POINT ( 'NONE',  ( -14.48388495494899608, 329.8073905683720000, -9.489475012073736337 ) ) ;
#11014=CARTESIAN_POINT ( 'NONE',  ( -48.68588794268870146, 271.9948905765656377, 0.000000000000000000 ) ) ;
#11015=CARTESIAN_POINT ( 'NONE',  ( -11.73070664223725323, 393.1823905601785896, -11.32908994701042538 ) ) ;
#11016=CARTESIAN_POINT ( 'NONE',  ( -45.43829269268869808, 243.5573905683720000, -3.332260488124726638 ) ) ;
#11017=CARTESIAN_POINT ( 'NONE',  ( -11.93348319268872615, 400.3698905683720000, -2.051577885510841163E-15 ) ) ;
#11020=CARTESIAN_POINT ( 'NONE',  ( -28.68588794268873698, 548.2448905601784190, 0.000000000000000000 ) ) ;
#11022=CARTESIAN_POINT ( 'NONE',  ( -17.35679799567831338, 508.5573905765655809, -16.95518130045146421 ) ) ;
#11023=CARTESIAN_POINT ( 'NONE',  ( -22.27502019258948707, 446.9948905683720000, 15.47720386886985189 ) ) ;
#11025=CARTESIAN_POINT ( 'NONE',  ( -21.03221929538693402, 454.1198905601784759, -18.47759065022572855 ) ) ;
#11026=ADVANCED_FACE ( 'NONE', ( #17412 ), #4532, .T. ) ;
#11031=CARTESIAN_POINT ( 'NONE',  ( -24.70764059509555821, 324.4323905601784190, -19.99999999999999289 ) ) ;
#11034=CARTESIAN_POINT ( 'NONE',  ( -14.48388495494899786, 359.4323905683720000, 9.489475012073731008 ) ) ;
#11035=CARTESIAN_POINT ( 'NONE',  ( -28.68588794268874054, 573.2448905601785327, 0.000000000000000000 ) ) ;
#11036=CARTESIAN_POINT ( 'NONE',  ( -24.70764059509557953, 509.1823905765655240, -19.99999999999999289 ) ) ;
#11037=CARTESIAN_POINT ( 'NONE',  ( -32.01814843081344719, 386.0573905683720000, 16.75240474999999307 ) ) ;
#11038=CARTESIAN_POINT ( 'NONE',  ( -44.16309181155855867, 224.7448905683720568, -6.410867750099231266 ) ) ;
#11039=CARTESIAN_POINT ( 'NONE',  ( -11.93348319268872615, 409.1823905683720568, -3.332260488124732856 ) ) ;
#11040=CARTESIAN_POINT ( 'NONE',  ( -28.68588794268871212, 329.4948905765656377, -19.99999999999999289 ) ) ;
#11042=CARTESIAN_POINT ( 'NONE',  ( -35.09675569278794427, 305.7448905683720568, 15.47720386886985366 ) ) ;
#11044=CARTESIAN_POINT ( 'NONE',  ( -19.19641293061498999, 448.8073905683720568, 14.20200298773971426 ) ) ;
#11046=CARTESIAN_POINT ( 'NONE',  ( -10.20829729246298712, 371.6198905601784759, 7.653668647301790529 ) ) ;
#11048=CARTESIAN_POINT ( 'NONE',  ( -32.01814843081344719, 373.1823905683720000, -16.75240474999999307 ) ) ;
#11049=CARTESIAN_POINT ( 'NONE',  ( -19.19641293061500065, 510.4323905683720000, -14.20200298773971603 ) ) ;
#11050=CARTESIAN_POINT ( 'NONE',  ( -8.685887942688740537, 501.9323905601784759, 3.978247347593161010 ) ) ;
#11051=CARTESIAN_POINT ( 'NONE',  ( -40.53162694259543031, 322.6198905683720568, -11.84573899990672707 ) ) ;
#11055=VERTEX_POINT ( 'NONE', #13964 ) ;
#11059=ADVANCED_FACE ( 'NONE', ( #5056 ), #19451, .T. ) ;
#11060=CARTESIAN_POINT ( 'NONE',  ( -32.01814843081344719, 417.5573905683720568, 16.75240474999999307 ) ) ;
#11061=CARTESIAN_POINT ( 'NONE',  ( -45.64106924314018698, 392.9323905765655809, 11.32908994701042538 ) ) ;
#11063=CARTESIAN_POINT ( 'NONE',  ( -25.35362745456399125, 436.6823905683720000, 16.75240474999998952 ) ) ;
#11065=CARTESIAN_POINT ( 'NONE',  ( -14.48388495494901029, 459.8073905683720000, -9.489475012073734561 ) ) ;
#11069=CARTESIAN_POINT ( 'NONE',  ( -42.82802356641966668, 393.2448905765655809, 14.14213562373094923 ) ) ;
#11070=CARTESIAN_POINT ( 'NONE',  ( -8.685887942688712116, 276.9948905765656377, -2.449293598294705724E-15 ) ) ;
#11078=CARTESIAN_POINT ( 'NONE',  ( -24.70764059509554755, 254.4323905601784759, -19.99999999999999289 ) ) ;
#11079=CARTESIAN_POINT ( 'NONE',  ( -43.68588794268869435, 213.9102039777116602, 0.000000000000000000 ) ) ;
#11080=CARTESIAN_POINT ( 'NONE',  ( -16.84014894278199392, 419.1198905683720000, 11.84573899990672530 ) ) ;
#11081=DIRECTION ( 'NONE',  ( -1.191790137725560488E-16, 1.000000000000000000, -0.000000000000000000 ) ) ;
#11083=( BOUNDED_CURVE ( )  B_SPLINE_CURVE ( 2, ( #6775, #2038, #18355, #16645, #2249, #11653, #11867, #15444, #208, #15346, #10020, #8607, #13396, #20305, #5475, #1829, #3855 ),
 .UNSPECIFIED., .F., .T. ) 
 B_SPLINE_CURVE_WITH_KNOTS ( ( 3, 2, 2, 2, 2, 2, 2, 2, 3 ),
 ( 0.000000000000000000, 0.001953125000000046838, 0.003906250000000093675, 0.005859375000000140513, 0.007812500000000187350, 0.009765625000000234188, 0.01171875000000028103, 0.01367187500000032786, 0.01562500000000037470 ),
 .UNSPECIFIED. ) 
 CURVE ( )  GEOMETRIC_REPRESENTATION_ITEM ( )  RATIONAL_B_SPLINE_CURVE ( ( 1.000000000000000000, 0.9807852804032304306, 1.000000000000000000, 0.9807852804032304306, 1.000000000000000000, 0.9807852804032304306, 1.000000000000000000, 0.9807852804032304306, 1.000000000000000000, 0.9807852804032304306, 1.000000000000000000, 0.9807852804032304306, 1.000000000000000000, 0.9807852804032304306, 1.000000000000000000, 0.9807852804032267668, 1.000000000000003775 ) ) 
 REPRESENTATION_ITEM ( '' )  );
#11084=CARTESIAN_POINT ( 'NONE',  ( -35.09675569278793006, 243.4948905683720284, -15.47720386886985544 ) ) ;
#11086=EDGE_LOOP ( 'NONE', ( #19079, #5363, #18402, #11762 ) ) ;
#11089=CARTESIAN_POINT ( 'NONE',  ( -28.68588794268872633, 467.8698905683720000, 16.75240474999999307 ) ) ;
#11090=CARTESIAN_POINT ( 'NONE',  ( -40.01497788969911795, 223.5573905765656093, 16.95518130045146776 ) ) ;
#11092=ORIENTED_EDGE ( 'NONE', *, *, #17674, .F. ) ;
#11094=CARTESIAN_POINT ( 'NONE',  ( -35.09675569278793716, 225.7448905683720568, 15.47720386886985366 ) ) ;
#11096=ORIENTED_EDGE ( 'NONE', *, *, #7575, .F. ) ;
#11097=CARTESIAN_POINT ( 'NONE',  ( -16.84014894278200813, 527.6198905683719431, 11.84573899990672530 ) ) ;
#11099=CARTESIAN_POINT ( 'NONE',  ( -21.03221929538691981, 455.1198905765655809, 18.47759065022572500 ) ) ;
#11102=DIRECTION ( 'NONE',  ( -1.191790137725560488E-16, 1.000000000000000000, -0.000000000000000000 ) ) ;
#11105=CARTESIAN_POINT ( 'NONE',  ( -35.09675569278793006, 231.9948905683720284, -15.47720386886985544 ) ) ;
#11106=CARTESIAN_POINT ( 'NONE',  ( -40.53162694259543031, 324.1198905683720568, -11.84573899990672707 ) ) ;
#11107=CARTESIAN_POINT ( 'NONE',  ( -21.03221929538693402, 444.1198905601784759, -18.47759065022572855 ) ) ;
#11108=CARTESIAN_POINT ( 'NONE',  ( -11.73070664223724791, 381.3073905601784759, 11.32908994701042005 ) ) ;
#11109=AXIS2_PLACEMENT_3D ( 'NONE', #12432, #20874, #17619 ) ;
#11110=CARTESIAN_POINT ( 'NONE',  ( -44.16309181155855867, 315.9948905683720568, 6.410867750099241924 ) ) ;
#11111=CARTESIAN_POINT ( 'NONE',  ( -38.17536295476244845, 385.4323905683720000, 14.20200298773971781 ) ) ;
#11112=ADVANCED_FACE ( 'NONE', ( #21076 ), #16327, .T. ) ;
#11113=CARTESIAN_POINT ( 'NONE',  ( -14.48388495494901917, 531.3073905683719431, -9.489475012073734561 ) ) ;
#11114=CARTESIAN_POINT ( 'NONE',  ( -8.685887942688720997, 362.5573905601784759, -3.978247347593165895 ) ) ;
#11115=CARTESIAN_POINT ( 'NONE',  ( -28.68588794268870146, 229.4948905765656377, -19.99999999999999289 ) ) ;
#11117=CARTESIAN_POINT ( 'NONE',  ( -16.84014894278200458, 491.6198905683720000, -11.84573899990672707 ) ) ;
#11118=DIRECTION ( 'NONE',  ( -1.000000000000000000, 0.000000000000000000, 0.000000000000000000 ) ) ;
#11119=CARTESIAN_POINT ( 'NONE',  ( -19.19641293061497578, 307.3073905683720000, 14.20200298773971426 ) ) ;
#11121=CARTESIAN_POINT ( 'NONE',  ( -11.93348319268871194, 290.3698905683720568, -2.051577885510841163E-15 ) ) ;
#11122=CARTESIAN_POINT ( 'NONE',  ( -45.43829269268870519, 323.8698905683720000, 0.000000000000000000 ) ) ;
#11124=CARTESIAN_POINT ( 'NONE',  ( -42.82802356641965247, 273.2448905765656377, 14.14213562373094923 ) ) ;
#11126=CARTESIAN_POINT ( 'NONE',  ( -28.68588794268870146, 231.3698905683720284, -16.75240474999999307 ) ) ;
#11127=CARTESIAN_POINT ( 'NONE',  ( -25.35362745456398414, 378.1823905683720568, 16.75240474999998952 ) ) ;
#11130=CARTESIAN_POINT ( 'NONE',  ( -48.68588794268869435, 257.2448905601784759, 0.000000000000000000 ) ) ;
#11133=AXIS2_PLACEMENT_3D ( 'NONE', #2445, #12386, #9026 ) ;
#11134=CARTESIAN_POINT ( 'NONE',  ( -47.16347859291446554, 511.3698905765655809, -7.653668647301793193 ) ) ;
#11135=CARTESIAN_POINT ( 'NONE',  ( -13.20868407381887089, 439.4948905683720568, -6.410867750099233042 ) ) ;
#11138=CARTESIAN_POINT ( 'NONE',  ( -42.82802356641966668, 448.4948905601784759, 14.14213562373094923 ) ) ;
#11139=ORIENTED_EDGE ( 'NONE', *, *, #20021, .T. ) ;
#11142=CARTESIAN_POINT ( 'NONE',  ( -42.82802356641965957, 335.9948905601784759, -14.14213562373094746 ) ) ;
#11143=CARTESIAN_POINT ( 'NONE',  ( -45.43280446313950449, 223.9102039777116602, 0.4287796227366179602 ) ) ;
#11145=CARTESIAN_POINT ( 'NONE',  ( -16.84014894278199037, 371.6198905683720000, -11.84573899990672707 ) ) ;
#11146=CARTESIAN_POINT ( 'NONE',  ( -48.68588794268873698, 573.2448905601785327, 0.000000000000000000 ) ) ;
#11147=CARTESIAN_POINT ( 'NONE',  ( -21.03221929538692692, 495.1198905765656377, 18.47759065022572500 ) ) ;
#11148=CARTESIAN_POINT ( 'NONE',  ( -42.88789093042844058, 392.9323905683720568, -9.489475012073736337 ) ) ;
#11149=CARTESIAN_POINT ( 'NONE',  ( -28.68588794268869790, 222.8698905683720284, -16.75240474999999307 ) ) ;
#11151=CARTESIAN_POINT ( 'NONE',  ( -35.09675569278795138, 391.9948905683720568, -15.47720386886985544 ) ) ;
#11153=CARTESIAN_POINT ( 'NONE',  ( -36.33955658999050087, 320.1198905765656377, -18.47759065022572855 ) ) ;
#11155=CARTESIAN_POINT ( 'NONE',  ( -25.35362745456398059, 281.0573905683720568, -16.75240474999999307 ) ) ;
#11156=CARTESIAN_POINT ( 'NONE',  ( -35.09675569278796559, 467.2448905683720568, 15.47720386886985366 ) ) ;
#11159=CARTESIAN_POINT ( 'NONE',  ( -48.68588794268871567, 417.2448905601784759, 0.000000000000000000 ) ) ;
#11162=CARTESIAN_POINT ( 'NONE',  ( -40.53162694259543741, 376.6198905683720568, 11.84573899990672885 ) ) ;
#11163=CARTESIAN_POINT ( 'NONE',  ( -42.88789093042845479, 512.9323905683719431, -9.489475012073736337 ) ) ;
#11165=CARTESIAN_POINT ( 'NONE',  ( -11.73070664223726745, 513.1823905601785327, -11.32908994701042715 ) ) ;
#11166=CARTESIAN_POINT ( 'NONE',  ( -44.16309181155855867, 324.4948905683720568, 6.410867750099241924 ) ) ;
#11168=CARTESIAN_POINT ( 'NONE',  ( -17.35679799567831694, 523.8073905601784190, -16.95518130045146421 ) ) ;
#11169=EDGE_LOOP ( 'NONE', ( #9964, #7462, #12268, #5419 ) ) ;
#11171=LINE ( 'NONE', #19395, #18080 ) ;
#11172=CARTESIAN_POINT ( 'NONE',  ( -28.68588794268871922, 417.8698905683720568, 16.75240474999999307 ) ) ;
#11173=CARTESIAN_POINT ( 'NONE',  ( -32.66413529028185536, 234.1823905765656662, 19.99999999999999289 ) ) ;
#11175=CARTESIAN_POINT ( 'NONE',  ( -35.09675569278795848, 435.7448905683720000, 15.47720386886985366 ) ) ;
#11177=CARTESIAN_POINT ( 'NONE',  ( -40.53162694259545162, 472.6198905683720000, -11.84573899990672707 ) ) ;
#11181=CARTESIAN_POINT ( 'NONE',  ( -36.33955658999051508, 373.8698905765656377, 18.47759065022572500 ) ) ;
#11183=CARTESIAN_POINT ( 'NONE',  ( -40.01497788969913927, 370.4323905765656946, -16.95518130045146421 ) ) ;
#11184=CARTESIAN_POINT ( 'NONE',  ( -36.33955658999051508, 430.1198905765656377, -18.47759065022572855 ) ) ;
#11185=CARTESIAN_POINT ( 'NONE',  ( -48.68588794268886488, 252.3073905765655240, 3.978247347592742678 ) ) ;
#11186=AXIS2_PLACEMENT_3D ( 'NONE', #14694, #14906, #14479 ) ;
#11188=CARTESIAN_POINT ( 'NONE',  ( -48.68588794268852382, 256.9323905601784759, -3.978247347593583783 ) ) ;
#11189=CARTESIAN_POINT ( 'NONE',  ( -48.68588794268870856, 347.2448905601784759, 0.000000000000000000 ) ) ;
#11191=CARTESIAN_POINT ( 'NONE',  ( -16.84014894278199392, 429.1198905683720000, 11.84573899990672530 ) ) ;
#11192=CARTESIAN_POINT ( 'NONE',  ( -48.68588794268870856, 387.2448905601784759, 0.000000000000000000 ) ) ;
#11193=CARTESIAN_POINT ( 'NONE',  ( -44.16309181155855867, 254.7448905683720284, -6.410867750099231266 ) ) ;
#11198=CARTESIAN_POINT ( 'NONE',  ( -32.01814843081345430, 467.5573905683721136, 16.75240474999999307 ) ) ;
#11199=CARTESIAN_POINT ( 'NONE',  ( -36.33955658999049376, 220.1198905765656093, -18.47759065022572855 ) ) ;
#11204=CARTESIAN_POINT ( 'NONE',  ( -35.09675569278793006, 221.9948905683720284, -15.47720386886985544 ) ) ;
#11207=CARTESIAN_POINT ( 'NONE',  ( -40.53162694259545873, 525.1198905683720568, 11.84573899990672885 ) ) ;
#11208=CYLINDRICAL_SURFACE ( 'NONE', #1415, 19.99999999999999645 ) ;
#11210=CARTESIAN_POINT ( 'NONE',  ( -8.685887942688731655, 446.6823905765656377, 3.978247347593161010 ) ) ;
#11215=CARTESIAN_POINT ( 'NONE',  ( -8.685887942688715668, 296.9948905765655809, -2.449293598294705724E-15 ) ) ;
#11216=CARTESIAN_POINT ( 'NONE',  ( -38.17536295476243424, 235.4323905683720284, 14.20200298773971781 ) ) ;
#11217=CARTESIAN_POINT ( 'NONE',  ( -19.19641293061497578, 308.8073905683721136, 14.20200298773971426 ) ) ;
#11220=CARTESIAN_POINT ( 'NONE',  ( -17.35679799567829207, 380.6823905601784759, 16.95518130045146421 ) ) ;
#11221=CARTESIAN_POINT ( 'NONE',  ( -11.93348319268871549, 300.0573905683720568, 3.332260488124728415 ) ) ;
#11222=CARTESIAN_POINT ( 'NONE',  ( -42.88789093042843348, 362.9323905683720568, -9.489475012073736337 ) ) ;
#11223=CARTESIAN_POINT ( 'NONE',  ( -45.43829269268873361, 525.3698905683720568, 0.000000000000000000 ) ) ;
#11224=CARTESIAN_POINT ( 'NONE',  ( -8.685887942688720997, 361.9323905601785327, 3.978247347593161010 ) ) ;
#11225=CARTESIAN_POINT ( 'NONE',  ( -21.03221929538692692, 404.1198905601784759, -18.47759065022572855 ) ) ;
#11227=CARTESIAN_POINT ( 'NONE',  ( -19.19641293061500065, 491.9323905683720000, -14.20200298773971603 ) ) ;
#11229=CARTESIAN_POINT ( 'NONE',  ( -19.19641293061497933, 290.4323905683720000, -14.20200298773971603 ) ) ;
#11230=ORIENTED_EDGE ( 'NONE', *, *, #5468, .F. ) ;
#11231=CARTESIAN_POINT ( 'NONE',  ( -19.19641293061496867, 278.8073905683720000, 14.20200298773971426 ) ) ;
#11232=CARTESIAN_POINT ( 'NONE',  ( -35.09675569278794427, 315.7448905683720000, 15.47720386886985366 ) ) ;
#11233=CARTESIAN_POINT ( 'NONE',  ( -24.70764059509553334, 254.8073905765656093, 19.99999999999998934 ) ) ;
#11235=CARTESIAN_POINT ( 'NONE',  ( -45.43829269268869808, 233.8698905683720284, 0.000000000000000000 ) ) ;
#11236=CARTESIAN_POINT ( 'NONE',  ( -16.84014894278199392, 381.6198905683720568, -11.84573899990672707 ) ) ;
#11239=CARTESIAN_POINT ( 'NONE',  ( -40.01497788969913216, 270.4323905765655809, -16.95518130045146421 ) ) ;
#11240=CARTESIAN_POINT ( 'NONE',  ( -40.53162694259544452, 415.1198905683720000, 11.84573899990672885 ) ) ;
#11243=CARTESIAN_POINT ( 'NONE',  ( -21.03221929538691626, 420.3698905601784759, 18.47759065022572500 ) ) ;
#11248=CARTESIAN_POINT ( 'NONE',  ( -48.68588794268870146, 307.5573905601785327, 3.978247347593168115 ) ) ;
#11251=CARTESIAN_POINT ( 'NONE',  ( -16.84014894278198682, 349.1198905683720568, 11.84573899990672530 ) ) ;
#11252=CARTESIAN_POINT ( 'NONE',  ( -8.685887942688740537, 497.3073905765656377, -3.978247347593165895 ) ) ;
#11253=CARTESIAN_POINT ( 'NONE',  ( -25.35362745456398414, 376.6823905683720000, 16.75240474999998952 ) ) ;
#11255=CARTESIAN_POINT ( 'NONE',  ( -42.88789093042844058, 392.9323905683720568, -9.489475012073734561 ) ) ;
#11256=CARTESIAN_POINT ( 'NONE',  ( -14.54375231895776288, 325.7448905765655809, 14.14213562373094568 ) ) ;
#11258=CARTESIAN_POINT ( 'NONE',  ( -14.48388495494898898, 287.9323905683720000, 9.489475012073731008 ) ) ;
#11260=CARTESIAN_POINT ( 'NONE',  ( -11.93348319268872970, 440.3698905683720000, -2.051577885510841163E-15 ) ) ;
#11261=CARTESIAN_POINT ( 'NONE',  ( -48.68588794268860909, 286.9323905601784190, -3.978247347593371508 ) ) ;
#11262=CARTESIAN_POINT ( 'NONE',  ( -17.35679799567828852, 370.6823905601784759, 16.95518130045146421 ) ) ;
#11265=CARTESIAN_POINT ( 'NONE',  ( -16.84014894278199037, 351.6198905683720000, -11.84573899990672707 ) ) ;
#11266=CARTESIAN_POINT ( 'NONE',  ( -32.01814843081346140, 501.6823905683720568, -16.75240474999999307 ) ) ;
#11267=CARTESIAN_POINT ( 'NONE',  ( -28.68588794268872988, 484.7448905601784759, -19.99999999999999289 ) ) ;
#11268=CARTESIAN_POINT ( 'NONE',  ( -25.35362745456398770, 331.0573905683720000, -16.75240474999999307 ) ) ;
#11270=EDGE_LOOP ( 'NONE', ( #21050, #12130, #7680, #15916 ) ) ;
#11273=ADVANCED_FACE ( 'NONE', ( #8724 ), #13716, .T. ) ;
#11274=AXIS2_PLACEMENT_3D ( 'NONE', #9489, #19648, #20964 ) ;
#11275=CARTESIAN_POINT ( 'NONE',  ( -19.19641293061498288, 398.8073905683720568, 14.20200298773971426 ) ) ;
#11278=( NAMED_UNIT ( * ) SI_UNIT ( $, .STERADIAN. ) SOLID_ANGLE_UNIT ( ) );
#11279=CARTESIAN_POINT ( 'NONE',  ( -14.48388495494900674, 447.9323905683720000, 9.489475012073732785 ) ) ;
#11280=CARTESIAN_POINT ( 'NONE',  ( -14.48388495494900852, 447.9323905683720568, 9.489475012073731008 ) ) ;
#11283=CARTESIAN_POINT ( 'NONE',  ( -47.16347859291445133, 391.3698905765656377, -7.653668647301793193 ) ) ;
#11285=CARTESIAN_POINT ( 'NONE',  ( -47.16347859291445133, 391.3698905765656377, -7.653668647301793193 ) ) ;
#11288=CARTESIAN_POINT ( 'NONE',  ( -35.09675569278795848, 493.4948905683720568, -15.47720386886985544 ) ) ;
#11292=CARTESIAN_POINT ( 'NONE',  ( -40.88226806564986759, 223.9102039777117170, 14.73426766465872539 ) ) ;
#11295=CARTESIAN_POINT ( 'NONE',  ( -42.88789093042844058, 414.4323905683721136, -9.489475012073736337 ) ) ;
#11297=CARTESIAN_POINT ( 'NONE',  ( -42.88789093042841927, 246.3073905683720284, 9.489475012073736337 ) ) ;
#11301=CARTESIAN_POINT ( 'NONE',  ( -16.84014894278199748, 459.1198905683720568, 11.84573899990672530 ) ) ;
#11302=CARTESIAN_POINT ( 'NONE',  ( -45.43829269268872650, 533.5573905683720568, -3.332260488124726194 ) ) ;
#11303=AXIS2_PLACEMENT_3D ( 'NONE', #21352, #11389, #3186 ) ;
#11305=CARTESIAN_POINT ( 'NONE',  ( -43.68588794268869435, 210.1437886375728965, 2.161863591991830530E-19 ) ) ;
#11306=CARTESIAN_POINT ( 'NONE',  ( -11.93348319268870483, 228.8698905683720284, -2.051577885510841163E-15 ) ) ;
#11308=CARTESIAN_POINT ( 'NONE',  ( -28.68588794268872988, 506.3698905683720000, 16.75240474999999307 ) ) ;
#11311=CARTESIAN_POINT ( 'NONE',  ( -10.20829729246299600, 447.6198905765656377, -7.653668647301794969 ) ) ;
#11313=CARTESIAN_POINT ( 'NONE',  ( -45.64106924314017277, 301.0573905765655809, -11.32908994701042538 ) ) ;
#11314=CARTESIAN_POINT ( 'NONE',  ( -14.48388495494899608, 337.9323905683720568, 9.489475012073731008 ) ) ;
#11316=CARTESIAN_POINT ( 'NONE',  ( -28.68588794268874054, 573.2448905601785327, 0.000000000000000000 ) ) ;
#11318=CARTESIAN_POINT ( 'NONE',  ( -35.86044580198795018, 223.9104597372275123, 18.66884633871304899 ) ) ;
#11319=CARTESIAN_POINT ( 'NONE',  ( -11.93348319268870483, 228.8698905683720284, -2.051577885510841163E-15 ) ) ;
#11320=CARTESIAN_POINT ( 'NONE',  ( -35.09675569278794427, 317.2448905683720000, 15.47720386886985366 ) ) ;
#11322=CARTESIAN_POINT ( 'NONE',  ( -48.68588794268870146, 276.9323905601784190, -3.978247347593158345 ) ) ;
#11323=CARTESIAN_POINT ( 'NONE',  ( -32.66413529028186957, 379.4323905601785327, 19.99999999999999289 ) ) ;
#11325=CARTESIAN_POINT ( 'NONE',  ( -22.27502019258946930, 308.4948905683720568, 15.47720386886985189 ) ) ;
#11326=CARTESIAN_POINT ( 'NONE',  ( -44.16309181155859420, 514.7448905683720568, -6.410867750099231266 ) ) ;
#11327=CARTESIAN_POINT ( 'NONE',  ( -32.66413529028187668, 365.0573905601784759, -19.99999999999999289 ) ) ;
#11330=CARTESIAN_POINT ( 'NONE',  ( -11.93348319268873681, 490.3698905683720568, -2.051577885510841163E-15 ) ) ;
#11332=CARTESIAN_POINT ( 'NONE',  ( -32.01814843081344009, 281.6823905683720568, -16.75240474999999307 ) ) ;
#11333=ORIENTED_EDGE ( 'NONE', *, *, #1654, .F. ) ;
#11334=EDGE_CURVE ( 'NONE', #13635, #4322, #13186, .T. ) ;
#11335=CARTESIAN_POINT ( 'NONE',  ( -38.17536295476244135, 286.9323905683720000, 14.20200298773971781 ) ) ;
#11336=CARTESIAN_POINT ( 'NONE',  ( -25.35362745456398770, 331.0573905683720000, -16.75240474999999307 ) ) ;
#11337=CARTESIAN_POINT ( 'NONE',  ( -11.93348319268870839, 260.3698905683720000, -2.051577885510841163E-15 ) ) ;
#11338=( BOUNDED_CURVE ( )  B_SPLINE_CURVE ( 2, ( #14340, #20920, #16382, #371, #160, #10080, #11495, #11920, #3394, #18092, #15082, #11712, #16592, #1890, #6619, #13240, #18411 ),
 .UNSPECIFIED., .F., .T. ) 
 B_SPLINE_CURVE_WITH_KNOTS ( ( 3, 2, 2, 2, 2, 2, 2, 2, 3 ),
 ( 0.2656250000000002220, 0.2675781250000002220, 0.2695312500000001665, 0.2714843750000001665, 0.2734375000000001110, 0.2753906250000001110, 0.2773437500000001110, 0.2792968750000000555, 0.2812500000000000555 ),
 .UNSPECIFIED. ) 
 CURVE ( )  GEOMETRIC_REPRESENTATION_ITEM ( )  RATIONAL_B_SPLINE_CURVE ( ( 0.9999999999999977796, 0.9807852804032326510, 1.000000000000000000, 0.9807852804032304306, 1.000000000000000000, 0.9807852804032304306, 1.000000000000000000, 0.9807852804032304306, 1.000000000000000000, 0.9807852804032304306, 1.000000000000000000, 0.9807852804032304306, 1.000000000000000000, 0.9807852804032304306, 1.000000000000000000, 0.9807852804032298755, 1.000000000000000444 ) ) 
 REPRESENTATION_ITEM ( '' )  );
#11339=CARTESIAN_POINT ( 'NONE',  ( -36.33955658999050087, 270.1198905765655809, -18.47759065022572855 ) ) ;
#11340=CARTESIAN_POINT ( 'NONE',  ( -8.685887942688548691, 392.5573905601785327, -3.978247347592740013 ) ) ;
#11341=CARTESIAN_POINT ( 'NONE',  ( -45.35320578180308360, 224.2032419181830107, 3.537678462365220877 ) ) ;
#11342=CARTESIAN_POINT ( 'NONE',  ( -28.68588794268871212, 367.8698905683720000, 16.75240474999999307 ) ) ;
#11343=CARTESIAN_POINT ( 'NONE',  ( -8.685887942688712116, 282.2448905601784759, -2.449293598294705724E-15 ) ) ;
#11346=CARTESIAN_POINT ( 'NONE',  ( -25.35362745456399836, 431.0573905683720000, -16.75240474999999307 ) ) ;
#11348=VERTEX_POINT ( 'NONE', #18250 ) ;
#11349=CARTESIAN_POINT ( 'NONE',  ( -40.01497788969914637, 435.6823905601784759, -16.95518130045146421 ) ) ;
#11354=CARTESIAN_POINT ( 'NONE',  ( -21.03221929538690205, 300.3698905601784759, 18.47759065022572500 ) ) ;
#11356=CARTESIAN_POINT ( 'NONE',  ( -22.27502019258947286, 338.4948905683720568, 15.47720386886985189 ) ) ;
#11357=CARTESIAN_POINT ( 'NONE',  ( -32.66413529028189089, 494.1823905765655240, 19.99999999999999289 ) ) ;
#11358=CARTESIAN_POINT ( 'NONE',  ( -22.27502019258947996, 386.9948905683720568, 15.47720386886985189 ) ) ;
#11360=CARTESIAN_POINT ( 'NONE',  ( -25.35362745456398414, 376.6823905683720000, 16.75240474999998952 ) ) ;
#11362=CARTESIAN_POINT ( 'NONE',  ( -17.35679799567829562, 328.5573905765656377, -16.95518130045146421 ) ) ;
#11364=CARTESIAN_POINT ( 'NONE',  ( -35.09675569278793716, 291.9948905683720000, -15.47720386886985544 ) ) ;
#11365=CARTESIAN_POINT ( 'NONE',  ( -16.84014894278199748, 439.1198905683720568, 11.84573899990672530 ) ) ;
#11371=CARTESIAN_POINT ( 'NONE',  ( -14.48388495494899608, 349.4323905683720000, 9.489475012073732785 ) ) ;
#11372=CARTESIAN_POINT ( 'NONE',  ( -28.68588794268872988, 481.3698905683720568, -16.75240474999999307 ) ) ;
#11373=CARTESIAN_POINT ( 'NONE',  ( -48.68588794268872277, 477.5573905601784759, 3.978247347593168115 ) ) ;
#11374=CARTESIAN_POINT ( 'NONE',  ( -28.68588794268870856, 326.3698905683720000, 16.75240474999999307 ) ) ;
#11377=CARTESIAN_POINT ( 'NONE',  ( -38.86787825240671168, 223.9102039777116318, -13.30301237467029019 ) ) ;
#11378=VERTEX_POINT ( 'NONE', #20415 ) ;
#11381=CARTESIAN_POINT ( 'NONE',  ( -35.09675569278795848, 407.2448905683720568, 15.47720386886985366 ) ) ;
#11382=CARTESIAN_POINT ( 'NONE',  ( -48.68588794268870856, 357.2448905601784759, 0.000000000000000000 ) ) ;
#11384=CARTESIAN_POINT ( 'NONE',  ( -28.68588794268872633, 441.3698905683720000, -16.75240474999999307 ) ) ;
#11385=CARTESIAN_POINT ( 'NONE',  ( -45.43829269268871940, 443.5573905683719431, -3.332260488124726638 ) ) ;
#11386=CARTESIAN_POINT ( 'NONE',  ( -11.73070664223725501, 413.1823905601784190, -11.32908994701042538 ) ) ;
#11387=CARTESIAN_POINT ( 'NONE',  ( -14.54375231895776999, 385.7448905765656377, 14.14213562373094568 ) ) ;
#11389=DIRECTION ( 'NONE',  ( -1.191790137725560488E-16, 1.000000000000000000, -0.000000000000000000 ) ) ;
#11392=CARTESIAN_POINT ( 'NONE',  ( -32.01814843081346140, 503.1823905683721136, -16.75240474999999307 ) ) ;
#11395=CARTESIAN_POINT ( 'NONE',  ( -8.685887942688740537, 522.2448905601784190, -2.449293598294705724E-15 ) ) ;
#11396=( BOUNDED_CURVE ( )  B_SPLINE_CURVE ( 2, ( #2848, #9001, #14431, #7697, #14107, #20692, #19383, #2740, #5865, #19279, #5972, #6181, #4568, #19177, #7798, #12474, #14326 ),
 .UNSPECIFIED., .F., .T. ) 
 B_SPLINE_CURVE_WITH_KNOTS ( ( 3, 2, 2, 2, 2, 2, 2, 2, 3 ),
 ( 0.2343750000000001943, 0.2363281250000001943, 0.2382812500000001943, 0.2402343750000001943, 0.2421875000000002220, 0.2441406250000002220, 0.2460937500000002220, 0.2480468750000002220, 0.2500000000000002220 ),
 .UNSPECIFIED. ) 
 CURVE ( )  GEOMETRIC_REPRESENTATION_ITEM ( )  RATIONAL_B_SPLINE_CURVE ( ( 0.9999999999999981126, 0.9807852804032323180, 1.000000000000000000, 0.9807852804032304306, 1.000000000000000000, 0.9807852804032304306, 1.000000000000000000, 0.9807852804032304306, 1.000000000000000000, 0.9807852804032304306, 1.000000000000000000, 0.9807852804032304306, 1.000000000000000000, 0.9807852804032304306, 1.000000000000000000, 0.9807852804032282101, 1.000000000000002220 ) ) 
 REPRESENTATION_ITEM ( '' )  );
#11397=ADVANCED_FACE ( 'NONE', ( #13616 ), #20100, .T. ) ;
#11398=CARTESIAN_POINT ( 'NONE',  ( -32.01814843081345430, 403.1823905683720000, -16.75240474999999307 ) ) ;
#11399=CARTESIAN_POINT ( 'NONE',  ( -24.70764059509557242, 469.1823905765656377, -19.99999999999999289 ) ) ;
#11400=CARTESIAN_POINT ( 'NONE',  ( -48.68588794268872988, 537.2448905601785327, 0.000000000000000000 ) ) ;
#11404=CARTESIAN_POINT ( 'NONE',  ( -16.84014894278200103, 469.1198905683720568, 11.84573899990672530 ) ) ;
#11405=CARTESIAN_POINT ( 'NONE',  ( -8.685887942688708563, 236.6823905765656093, 3.978247347593161010 ) ) ;
#11408=CARTESIAN_POINT ( 'NONE',  ( -35.09675569278797269, 527.2448905683719431, 15.47720386886985366 ) ) ;
#11409=VERTEX_POINT ( 'NONE', #18464 ) ;
#11410=CARTESIAN_POINT ( 'NONE',  ( -28.68588794268873343, 511.3698905683720000, -16.75240474999999307 ) ) ;
#11414=CARTESIAN_POINT ( 'NONE',  ( -24.70764059509557242, 449.1823905765655809, -19.99999999999999289 ) ) ;
#11418=CARTESIAN_POINT ( 'NONE',  ( -11.73070664223725856, 456.0573905765655809, 11.32908994701042005 ) ) ;
#11424=CARTESIAN_POINT ( 'NONE',  ( -11.93348319268871727, 310.6823905683720568, -3.332260488124732856 ) ) ;
#11427=CARTESIAN_POINT ( 'NONE',  ( -48.68588794268869435, 266.9323905601784759, -3.978247347593158345 ) ) ;
#11429=CARTESIAN_POINT ( 'NONE',  ( -32.01814843081344009, 283.1823905683720568, -16.75240474999999307 ) ) ;
#11430=AXIS2_PLACEMENT_3D ( 'NONE', #19399, #14341, #21345 ) ;
#11432=CARTESIAN_POINT ( 'NONE',  ( -44.16309181155858710, 515.9948905683720568, 6.410867750099241924 ) ) ;
#11433=CARTESIAN_POINT ( 'NONE',  ( -40.01497788969913216, 358.8073905601784190, 16.95518130045146776 ) ) ;
#11436=CARTESIAN_POINT ( 'NONE',  ( -45.43829269268871940, 495.0573905683719431, -3.332260488124726194 ) ) ;
#11438=CARTESIAN_POINT ( 'NONE',  ( -13.20868407381885135, 289.4948905683720000, -6.410867750099233042 ) ) ;
#11440=CARTESIAN_POINT ( 'NONE',  ( -45.43829269268870519, 275.6823905683720000, 3.332260488124734632 ) ) ;
#11441=CARTESIAN_POINT ( 'NONE',  ( -42.88789093042842637, 312.9323905683720000, -9.489475012073736337 ) ) ;
#11442=CARTESIAN_POINT ( 'NONE',  ( -40.53162694259542320, 256.6198905683720568, 11.84573899990672885 ) ) ;
#11443=CARTESIAN_POINT ( 'NONE',  ( -14.54375231895775578, 238.2448905765656093, -14.14213562373094746 ) ) ;
#11445=AXIS2_PLACEMENT_3D ( 'NONE', #9918, #4634, #8078 ) ;
#11447=CARTESIAN_POINT ( 'NONE',  ( -14.48388495494900141, 371.3073905683720568, -9.489475012073736337 ) ) ;
#11448=DIRECTION ( 'NONE',  ( -1.000000000000000000, 0.000000000000000000, 0.000000000000000000 ) ) ;
#11451=CARTESIAN_POINT ( 'NONE',  ( -42.82802356641965247, 270.7448905765656377, -14.14213562373094746 ) ) ;
#11452=ADVANCED_FACE ( 'NONE', ( #17384 ), #12192, .T. ) ;
#11453=CARTESIAN_POINT ( 'NONE',  ( -11.93348319268872793, 418.5573905683720568, 3.332260488124728415 ) ) ;
#11454=FACE_OUTER_BOUND ( 'NONE', #20010, .T. ) ;
#11456=CARTESIAN_POINT ( 'NONE',  ( -28.68588794268872277, 434.7448905601784759, -19.99999999999999289 ) ) ;
#11461=CARTESIAN_POINT ( 'NONE',  ( -40.01497788969913216, 353.5573905765656377, 16.95518130045146776 ) ) ;
#11462=CARTESIAN_POINT ( 'NONE',  ( -47.16347859291443712, 296.6198905601784759, -7.653668647301793193 ) ) ;
#11465=ADVANCED_FACE ( 'NONE', ( #14259 ), #19112, .T. ) ;
#11466=CARTESIAN_POINT ( 'NONE',  ( -45.43829269268871229, 335.6823905683720568, 3.332260488124734632 ) ) ;
#11467=CARTESIAN_POINT ( 'NONE',  ( -11.73070664223726034, 476.0573905765656377, 11.32908994701042005 ) ) ;
#11468=CARTESIAN_POINT ( 'NONE',  ( -44.16309181155857289, 363.2448905683720000, -6.410867750099231266 ) ) ;
#11469=CARTESIAN_POINT ( 'NONE',  ( -45.64106924314017277, 311.0573905765656377, -11.32908994701042538 ) ) ;
#11470=CARTESIAN_POINT ( 'NONE',  ( -14.48388495494900141, 379.8073905683721136, -9.489475012073734561 ) ) ;
#11472=CARTESIAN_POINT ( 'NONE',  ( -28.68588794268870856, 324.4948905765655809, 19.99999999999999289 ) ) ;
#11474=CARTESIAN_POINT ( 'NONE',  ( -11.93348319268871194, 279.1823905683720000, -3.332260488124732856 ) ) ;
#11477=CARTESIAN_POINT ( 'NONE',  ( -11.93348319268872970, 430.6823905683720568, -3.332260488124732856 ) ) ;
#11478=CARTESIAN_POINT ( 'NONE',  ( -17.35679799567828496, 283.8073905601784759, -16.95518130045146421 ) ) ;
#11479=CARTESIAN_POINT ( 'NONE',  ( -28.68588794268873343, 514.7448905601784190, -19.99999999999999289 ) ) ;
#11482=CARTESIAN_POINT ( 'NONE',  ( -42.82802356641966668, 448.4948905601784759, 14.14213562373094923 ) ) ;
#11484=CARTESIAN_POINT ( 'NONE',  ( -16.84014894278198327, 339.1198905683720568, 11.84573899990672530 ) ) ;
#11485=CARTESIAN_POINT ( 'NONE',  ( -45.43829269268871940, 483.5573905683720000, -3.332260488124726194 ) ) ;
#11486=ORIENTED_EDGE ( 'NONE', *, *, #13604, .T. ) ;
#11487=CARTESIAN_POINT ( 'NONE',  ( -14.54375231895778064, 480.9948905601784759, 14.14213562373094568 ) ) ;
#11488=CARTESIAN_POINT ( 'NONE',  ( -40.53162694259543031, 295.1198905683720000, 11.84573899990672885 ) ) ;
#11489=EDGE_LOOP ( 'NONE', ( #2831, #10045, #18929, #7198 ) ) ;
#11492=CARTESIAN_POINT ( 'NONE',  ( -28.68588794268874054, 573.2448905601785327, 0.000000000000000000 ) ) ;
#11494=CARTESIAN_POINT ( 'NONE',  ( -38.17536295476246266, 413.8073905683719431, -14.20200298773971426 ) ) ;
#11495=CARTESIAN_POINT ( 'NONE',  ( -21.03221929538691981, 445.1198905765655809, 18.47759065022572500 ) ) ;
#11497=CARTESIAN_POINT ( 'NONE',  ( -14.48388495494900496, 437.9323905683720000, 9.489475012073732785 ) ) ;
#11498=CARTESIAN_POINT ( 'NONE',  ( -11.93348319268872970, 439.1823905683720000, -3.332260488124732856 ) ) ;
#11500=CARTESIAN_POINT ( 'NONE',  ( -40.01497788969913927, 398.8073905601784759, 16.95518130045146776 ) ) ;
#11501=CARTESIAN_POINT ( 'NONE',  ( -45.64106924314018698, 382.9323905765656377, 11.32908994701042715 ) ) ;
#11503=CARTESIAN_POINT ( 'NONE',  ( -47.16347859291443001, 266.6198905601784759, -7.653668647301793193 ) ) ;
#11506=CARTESIAN_POINT ( 'NONE',  ( -40.53162694259545162, 494.1198905683720000, -11.84573899990672707 ) ) ;
#11509=CARTESIAN_POINT ( 'NONE',  ( -14.54375231895778242, 463.4948905601785327, -14.14213562373094746 ) ) ;
#11511=CARTESIAN_POINT ( 'NONE',  ( -48.68588794268871567, 417.2448905601784759, 0.000000000000000000 ) ) ;
#11513=CARTESIAN_POINT ( 'NONE',  ( -32.01814843081345430, 407.5573905683720568, 16.75240474999999307 ) ) ;
#11514=CARTESIAN_POINT ( 'NONE',  ( -40.01497788969911795, 263.5573905765656377, 16.95518130045146776 ) ) ;
#11515=ADVANCED_BREP_SHAPE_REPRESENTATION ( '', ( #12085, #12794 ), #4502 ) ;
#11516=CARTESIAN_POINT ( 'NONE',  ( -45.43829269268869808, 225.3698905683720284, 0.000000000000000000 ) ) ;
#11517=ORIENTED_EDGE ( 'NONE', *, *, #9958, .F. ) ;
#11518=FACE_OUTER_BOUND ( 'NONE', #11086, .T. ) ;
#11520=CARTESIAN_POINT ( 'NONE',  ( -40.53162694259544452, 444.1198905683720568, -11.84573899990672707 ) ) ;
#11521=CARTESIAN_POINT ( 'NONE',  ( -19.19641293061500420, 530.4323905683720568, -14.20200298773971603 ) ) ;
#11523=ORIENTED_EDGE ( 'NONE', *, *, #8682, .T. ) ;
#11524=CARTESIAN_POINT ( 'NONE',  ( -42.82802356641964536, 205.1437886375728965, 5.000000000000001776 ) ) ;
#11525=CARTESIAN_POINT ( 'NONE',  ( -22.27502019258946930, 220.7448905683720568, -15.47720386886985544 ) ) ;
#11527=CARTESIAN_POINT ( 'NONE',  ( -25.35362745456400901, 501.0573905683720568, -16.75240474999999307 ) ) ;
#11531=CARTESIAN_POINT ( 'NONE',  ( -14.54375231895778064, 438.2448905765656377, -14.14213562373094746 ) ) ;
#11533=CARTESIAN_POINT ( 'NONE',  ( -42.82802356641964536, 250.7448905765656377, -14.14213562373094746 ) ) ;
#11534=CARTESIAN_POINT ( 'NONE',  ( -28.68588794268872277, 454.4948905765656377, 19.99999999999999289 ) ) ;
#11536=CARTESIAN_POINT ( 'NONE',  ( -11.73070664223723725, 291.3073905601785327, 11.32908994701042005 ) ) ;
#11537=( BOUNDED_CURVE ( )  B_SPLINE_CURVE ( 2, ( #5461, #8494, #8814, #5354, #12175, #18762, #302, #15539, #5255, #3950, #10535, #7292, #8708, #20506, #5676, #12283, #18864 ),
 .UNSPECIFIED., .F., .T. ) 
 B_SPLINE_CURVE_WITH_KNOTS ( ( 3, 2, 2, 2, 2, 2, 2, 2, 3 ),
 ( 0.1562500000000001388, 0.1582031250000001388, 0.1601562500000001388, 0.1621093750000001388, 0.1640625000000001665, 0.1660156250000001665, 0.1679687500000001665, 0.1699218750000001665, 0.1718750000000001665 ),
 .UNSPECIFIED. ) 
 CURVE ( )  GEOMETRIC_REPRESENTATION_ITEM ( )  RATIONAL_B_SPLINE_CURVE ( ( 0.9999999999999986677, 0.9807852804032317628, 1.000000000000000000, 0.9807852804032304306, 1.000000000000000000, 0.9807852804032304306, 1.000000000000000000, 0.9807852804032304306, 1.000000000000000000, 0.9807852804032304306, 1.000000000000000000, 0.9807852804032304306, 1.000000000000000000, 0.9807852804032304306, 1.000000000000000000, 0.9807852804032287652, 1.000000000000001554 ) ) 
 REPRESENTATION_ITEM ( '' )  );
#11540=CARTESIAN_POINT ( 'NONE',  ( -38.17536295476244845, 323.8073905683719431, -14.20200298773971426 ) ) ;
#11542=CARTESIAN_POINT ( 'NONE',  ( -11.73070664223723547, 271.3073905601785327, 11.32908994701042005 ) ) ;
#11544=VECTOR ( 'NONE', #13561, 1000.000000000000000 ) ;
#11545=CARTESIAN_POINT ( 'NONE',  ( -32.01814843081344009, 297.5573905683720000, 16.75240474999999307 ) ) ;
#11546=EDGE_CURVE ( 'NONE', #16325, #17928, #7523, .T. ) ;
#11547=CARTESIAN_POINT ( 'NONE',  ( -16.84014894278200458, 499.1198905683720000, 11.84573899990672530 ) ) ;
#11548=CARTESIAN_POINT ( 'NONE',  ( -48.68588794268870856, 356.9323905601784759, -3.978247347593158345 ) ) ;
#11551=CARTESIAN_POINT ( 'NONE',  ( -35.09675569278795848, 463.4948905683720000, -15.47720386886985544 ) ) ;
#11553=CARTESIAN_POINT ( 'NONE',  ( -42.88789093042842637, 272.9323905683720568, -9.489475012073736337 ) ) ;
#11555=CARTESIAN_POINT ( 'NONE',  ( -42.82802356641964536, 228.4948905601784759, 14.14213562373094923 ) ) ;
#11556=EDGE_CURVE ( 'NONE', #10309, #9092, #16095, .T. ) ;
#11557=CARTESIAN_POINT ( 'NONE',  ( -19.19641293061497223, 281.9323905683720568, -14.20200298773971603 ) ) ;
#11558=CARTESIAN_POINT ( 'NONE',  ( -45.43829269268869808, 265.6823905683720568, 3.332260488124734632 ) ) ;
#11559=CARTESIAN_POINT ( 'NONE',  ( -24.70764059509553334, 244.8073905765656377, 19.99999999999998934 ) ) ;
#11561=FACE_OUTER_BOUND ( 'NONE', #13075, .T. ) ;
#11562=CARTESIAN_POINT ( 'NONE',  ( -45.43829269268869098, 264.1823905683720000, 3.332260488124734632 ) ) ;
#11563=CARTESIAN_POINT ( 'NONE',  ( -40.53162694259543741, 376.6198905683720568, 11.84573899990672885 ) ) ;
#11567=CARTESIAN_POINT ( 'NONE',  ( -13.20868407381886733, 428.2448905683720568, 6.410867750099229490 ) ) ;
#11570=CARTESIAN_POINT ( 'NONE',  ( -48.68588794268871567, 427.5573905601784759, 3.978247347593168115 ) ) ;
#11572=VERTEX_POINT ( 'NONE', #10878 ) ;
#11575=CARTESIAN_POINT ( 'NONE',  ( -42.82802356641965247, 298.4948905601784759, 14.14213562373094923 ) ) ;
#11577=CARTESIAN_POINT ( 'NONE',  ( -11.93348319268872260, 350.6823905683719431, -3.332260488124732856 ) ) ;
#11579=CARTESIAN_POINT ( 'NONE',  ( -8.685887942688738761, 486.6823905765656946, 3.978247347593161010 ) ) ;
#11580=CARTESIAN_POINT ( 'NONE',  ( -35.09675569278794427, 371.9948905683720568, -15.47720386886985544 ) ) ;
#11581=DIRECTION ( 'NONE',  ( -1.000000000000000000, 0.000000000000000000, 0.000000000000000000 ) ) ;
#11582=CARTESIAN_POINT ( 'NONE',  ( -44.16309181155857289, 394.4948905683720000, 6.410867750099241924 ) ) ;
#11583=CARTESIAN_POINT ( 'NONE',  ( -10.20829729246297823, 297.6198905765656377, -7.653668647301794969 ) ) ;
#11584=CARTESIAN_POINT ( 'NONE',  ( -8.685887942688728103, 422.2448905601784759, -2.449293598294705724E-15 ) ) ;
#11585=CARTESIAN_POINT ( 'NONE',  ( -32.01814843081344009, 291.6823905683720568, -16.75240474999999307 ) ) ;
#11586=FACE_OUTER_BOUND ( 'NONE', #10922, .T. ) ;
#11587=CARTESIAN_POINT ( 'NONE',  ( -42.88789093042844058, 436.3073905683720568, 9.489475012073736337 ) ) ;
#11588=CARTESIAN_POINT ( 'NONE',  ( -10.20829729246297646, 282.8698905601784759, -7.653668647301794969 ) ) ;
#11589=CARTESIAN_POINT ( 'NONE',  ( -40.01497788969914637, 498.8073905601784759, 16.95518130045146776 ) ) ;
#11594=CARTESIAN_POINT ( 'NONE',  ( -38.17536295476244845, 346.9323905683720568, 14.20200298773971781 ) ) ;
#11595=CARTESIAN_POINT ( 'NONE',  ( -42.88789093042844769, 474.8073905683720000, 9.489475012073736337 ) ) ;
#11596=EDGE_CURVE ( 'NONE', #11572, #6694, #5708, .T. ) ;
#11599=CARTESIAN_POINT ( 'NONE',  ( -24.70764059509556532, 480.0573905601784759, 19.99999999999998934 ) ) ;
#11600=CARTESIAN_POINT ( 'NONE',  ( -28.68588794268870856, 311.3698905683720568, -16.75240474999999307 ) ) ;
#11605=CARTESIAN_POINT ( 'NONE',  ( -45.43829269268871940, 395.0573905683719431, -3.332260488124726638 ) ) ;
#11607=CARTESIAN_POINT ( 'NONE',  ( -28.68588794268871922, 426.3698905683720568, 16.75240474999999307 ) ) ;
#11608=CARTESIAN_POINT ( 'NONE',  ( -32.01814843081345430, 451.6823905683720568, -16.75240474999999307 ) ) ;
#11609=CARTESIAN_POINT ( 'NONE',  ( -45.64106924314018698, 398.1823905601785327, 11.32908994701042538 ) ) ;
#11610=EDGE_CURVE ( 'NONE', #18327, #10139, #19633, .T. ) ;
#11611=CARTESIAN_POINT ( 'NONE',  ( -11.73070664223725146, 367.9323905765655809, -11.32908994701042715 ) ) ;
#11615=LINE ( 'NONE', #3710, #20751 ) ;
#11616=CARTESIAN_POINT ( 'NONE',  ( -14.48388495494901385, 489.4323905683720568, 9.489475012073732785 ) ) ;
#11618=CARTESIAN_POINT ( 'NONE',  ( -42.82802356641967378, 465.9948905601784759, -14.14213562373094746 ) ) ;
#11619=CARTESIAN_POINT ( 'NONE',  ( -48.68588794268872988, 517.2448905601785327, 0.000000000000000000 ) ) ;
#11621=CARTESIAN_POINT ( 'NONE',  ( -28.68588794268871567, 397.8698905683720000, 16.75240474999999307 ) ) ;
#11623=CARTESIAN_POINT ( 'NONE',  ( -11.93348319268870661, 230.6823905683720284, -3.332260488124732856 ) ) ;
#11624=CARTESIAN_POINT ( 'NONE',  ( -42.88789093042843348, 364.8073905683720568, 9.489475012073736337 ) ) ;
#11627=CARTESIAN_POINT ( 'NONE',  ( -16.84014894278201169, 520.1198905683720568, -11.84573899990672707 ) ) ;
#11629=CARTESIAN_POINT ( 'NONE',  ( -19.19641293061499354, 451.9323905683720568, -14.20200298773971603 ) ) ;
#11630=CARTESIAN_POINT ( 'NONE',  ( -25.35362745456401257, 531.0573905683720568, -16.75240474999999307 ) ) ;
#11632=CARTESIAN_POINT ( 'NONE',  ( -32.66413529028187668, 429.4323905601785896, 19.99999999999999289 ) ) ;
#11633=CARTESIAN_POINT ( 'NONE',  ( -11.93348319268873503, 478.5573905683721136, 3.332260488124728415 ) ) ;
#11635=CARTESIAN_POINT ( 'NONE',  ( -16.84014894278200458, 497.6198905683720000, 11.84573899990672530 ) ) ;
#11638=CARTESIAN_POINT ( 'NONE',  ( -36.33955658999052218, 450.1198905765655809, -18.47759065022572855 ) ) ;
#11640=CARTESIAN_POINT ( 'NONE',  ( -24.70764059509554755, 249.1823905765656093, -19.99999999999999289 ) ) ;
#11644=CARTESIAN_POINT ( 'NONE',  ( -28.68588794268874054, 573.2448905601785327, 0.000000000000000000 ) ) ;
#11645=CARTESIAN_POINT ( 'NONE',  ( -47.16347859291445843, 492.6198905765656377, 7.653668647301805628 ) ) ;
#11646=CARTESIAN_POINT ( 'NONE',  ( -40.53162694259543031, 294.1198905683720568, -11.84573899990672707 ) ) ;
#11647=CARTESIAN_POINT ( 'NONE',  ( -48.68588794268872988, 527.2448905601785327, 0.000000000000000000 ) ) ;
#11648=CARTESIAN_POINT ( 'NONE',  ( -10.20829729246297646, 271.6198905601784759, 7.653668647301790529 ) ) ;
#11649=CARTESIAN_POINT ( 'NONE',  ( -42.82802356641966668, 413.2448905765655809, 14.14213562373094923 ) ) ;
#11650=CARTESIAN_POINT ( 'NONE',  ( -44.16309181155856578, 294.7448905683720568, -6.410867750099231266 ) ) ;
#11651=EDGE_CURVE ( 'NONE', #20871, #11812, #5837, .T. ) ;
#11653=CARTESIAN_POINT ( 'NONE',  ( -40.01497788969916058, 535.6823905601784190, -16.95518130045146421 ) ) ;
#11654=CARTESIAN_POINT ( 'NONE',  ( -35.09675569278796559, 513.4948905683720568, -15.47720386886985544 ) ) ;
#11657=CARTESIAN_POINT ( 'NONE',  ( -28.68588794268872988, 472.8698905683720568, -16.75240474999999307 ) ) ;
#11660=CARTESIAN_POINT ( 'NONE',  ( -22.27502019258947641, 270.7448905683720568, -15.47720386886985544 ) ) ;
#11662=( BOUNDED_CURVE ( )  B_SPLINE_CURVE ( 2, ( #6882, #8826, #630, #1939, #8505, #10334, #5364, #314, #18460, #3649, #11968, #18565, #16957, #7196, #2138, #528, #13818 ),
 .UNSPECIFIED., .F., .T. ) 
 B_SPLINE_CURVE_WITH_KNOTS ( ( 3, 2, 2, 2, 2, 2, 2, 2, 3 ),
 ( 0.8281250000000002220, 0.8300781250000002220, 0.8320312500000002220, 0.8339843750000002220, 0.8359375000000002220, 0.8378906250000002220, 0.8398437500000002220, 0.8417968750000002220, 0.8437500000000002220 ),
 .UNSPECIFIED. ) 
 CURVE ( )  GEOMETRIC_REPRESENTATION_ITEM ( )  RATIONAL_B_SPLINE_CURVE ( ( 0.9999999999999977796, 0.9807852804032326510, 1.000000000000000000, 0.9807852804032304306, 1.000000000000000000, 0.9807852804032304306, 1.000000000000000000, 0.9807852804032304306, 1.000000000000000000, 0.9807852804032304306, 1.000000000000000000, 0.9807852804032304306, 1.000000000000000000, 0.9807852804032304306, 1.000000000000000000, 0.9807852804032282101, 1.000000000000002220 ) ) 
 REPRESENTATION_ITEM ( '' )  );
#11664=CARTESIAN_POINT ( 'NONE',  ( -13.20868407381884779, 269.7448905683720568, 6.410867750099229490 ) ) ;
#11665=CARTESIAN_POINT ( 'NONE',  ( -38.17536295476244135, 253.8073905683720284, -14.20200298773971426 ) ) ;
#11666=CARTESIAN_POINT ( 'NONE',  ( -28.68588794268869790, 244.4948905765655809, 19.99999999999999289 ) ) ;
#11668=CARTESIAN_POINT ( 'NONE',  ( -36.33955658999050087, 229.1198905601785043, 18.47759065022572500 ) ) ;
#11670=CARTESIAN_POINT ( 'NONE',  ( -16.84014894278197971, 270.1198905683720568, -11.84573899990672707 ) ) ;
#11671=CARTESIAN_POINT ( 'NONE',  ( -42.88789093042843348, 354.4323905683720568, -9.489475012073736337 ) ) ;
#11672=CARTESIAN_POINT ( 'NONE',  ( -48.68588794268870146, 277.2448905601784759, 0.000000000000000000 ) ) ;
#11675=CARTESIAN_POINT ( 'NONE',  ( -28.68588794268872277, 431.3698905683720000, -16.75240474999999307 ) ) ;
#11676=CARTESIAN_POINT ( 'NONE',  ( -24.70764059509555466, 339.1823905765656377, -19.99999999999999289 ) ) ;
#11677=ORIENTED_EDGE ( 'NONE', *, *, #5421, .T. ) ;
#11678=CARTESIAN_POINT ( 'NONE',  ( -8.685887942688728103, 421.9323905601785327, 3.978247347593161010 ) ) ;
#11683=CARTESIAN_POINT ( 'NONE',  ( -16.84014894278200813, 529.1198905683720568, 11.84573899990672530 ) ) ;
#11684=CARTESIAN_POINT ( 'NONE',  ( -24.70764059509554045, 310.0573905601784759, 19.99999999999998934 ) ) ;
#11686=CARTESIAN_POINT ( 'NONE',  ( -11.93348319268872260, 340.6823905683720000, -3.332260488124732856 ) ) ;
#11688=CARTESIAN_POINT ( 'NONE',  ( -8.685887942688736985, 476.6823905765656377, 3.978247347593161010 ) ) ;
#11689=CARTESIAN_POINT ( 'NONE',  ( -40.53162694259543741, 372.6198905683720000, -11.84573899990672707 ) ) ;
#11690=CARTESIAN_POINT ( 'NONE',  ( -44.16309181155857289, 363.2448905683720000, -6.410867750099231266 ) ) ;
#11692=CARTESIAN_POINT ( 'NONE',  ( -21.03221929538691626, 298.8698905765656377, -18.47759065022572855 ) ) ;
#11694=CARTESIAN_POINT ( 'NONE',  ( -35.09675569278793716, 265.7448905683720000, 15.47720386886985366 ) ) ;
#11696=CARTESIAN_POINT ( 'NONE',  ( -13.20868407381887089, 440.9948905683720568, -6.410867750099233042 ) ) ;
#11699=CARTESIAN_POINT ( 'NONE',  ( -45.64106924314020119, 516.3073905601785327, -11.32908994701042538 ) ) ;
#11700=CARTESIAN_POINT ( 'NONE',  ( -48.68588794268870146, 287.2448905601784759, 0.000000000000000000 ) ) ;
#11702=CARTESIAN_POINT ( 'NONE',  ( -32.01814843081344719, 333.1823905683720000, -16.75240474999999307 ) ) ;
#11703=CARTESIAN_POINT ( 'NONE',  ( -11.93348319268873681, 488.8698905683720568, -2.051577885510841163E-15 ) ) ;
#11705=CARTESIAN_POINT ( 'NONE',  ( -32.66413529028189089, 479.4323905601785327, 19.99999999999999289 ) ) ;
#11706=CARTESIAN_POINT ( 'NONE',  ( -19.19641293061497933, 300.4323905683721136, -14.20200298773971603 ) ) ;
#11708=ORIENTED_EDGE ( 'NONE', *, *, #15407, .T. ) ;
#11711=CARTESIAN_POINT ( 'NONE',  ( -14.48388495494900674, 399.4323905683720568, 9.489475012073731008 ) ) ;
#11712=CARTESIAN_POINT ( 'NONE',  ( -40.01497788969913927, 443.5573905765656377, 16.95518130045146776 ) ) ;
#11714=CARTESIAN_POINT ( 'NONE',  ( -11.93348319268872970, 428.8698905683720568, -2.051577885510841163E-15 ) ) ;
#11715=CARTESIAN_POINT ( 'NONE',  ( -19.19641293061497223, 251.9323905683720284, -14.20200298773971603 ) ) ;
#11716=CARTESIAN_POINT ( 'NONE',  ( -25.35362745456399125, 436.6823905683720568, 16.75240474999998952 ) ) ;
#11718=CARTESIAN_POINT ( 'NONE',  ( -47.16347859291445133, 397.8698905601784759, 7.653668647301805628 ) ) ;
#11719=CARTESIAN_POINT ( 'NONE',  ( -17.35679799567829917, 368.5573905765655809, -16.95518130045146421 ) ) ;
#11721=CARTESIAN_POINT ( 'NONE',  ( -8.685887942688548691, 387.3073905765655809, -3.978247347592740013 ) ) ;
#11722=CARTESIAN_POINT ( 'NONE',  ( -28.68588794268871212, 331.3698905683720000, -16.75240474999999307 ) ) ;
#11724=CARTESIAN_POINT ( 'NONE',  ( -44.16309181155857999, 505.9948905683720000, 6.410867750099241924 ) ) ;
#11725=DIRECTION ( 'NONE',  ( -1.191790137725560488E-16, 1.000000000000000000, -0.000000000000000000 ) ) ;
#11726=CARTESIAN_POINT ( 'NONE',  ( -47.16347859291445843, 466.6198905601784759, -7.653668647301793193 ) ) ;
#11729=CARTESIAN_POINT ( 'NONE',  ( -45.43829269268871229, 415.0573905683721136, -3.332260488124726194 ) ) ;
#11731=EDGE_CURVE ( 'NONE', #13900, #2082, #2992, .T. ) ;
#11732=CARTESIAN_POINT ( 'NONE',  ( -32.01814843081343298, 237.5573905683720568, 16.75240474999999307 ) ) ;
#11733=CARTESIAN_POINT ( 'NONE',  ( -40.53162694259543741, 365.1198905683720000, 11.84573899990672885 ) ) ;
#11734=EDGE_CURVE ( 'NONE', #13236, #10338, #13312, .T. ) ;
#11736=CARTESIAN_POINT ( 'NONE',  ( -11.93348319268874036, 519.1823905683719431, -3.332260488124732856 ) ) ;
#11738=CARTESIAN_POINT ( 'NONE',  ( -25.35362745456399125, 438.1823905683720000, 16.75240474999998952 ) ) ;
#11739=CARTESIAN_POINT ( 'NONE',  ( -38.17536295476247687, 522.3073905683721705, -14.20200298773971426 ) ) ;
#11740=ORIENTED_EDGE ( 'NONE', *, *, #6009, .T. ) ;
#11741=CYLINDRICAL_SURFACE ( 'NONE', #10022, 19.99999999999999645 ) ;
#11742=CARTESIAN_POINT ( 'NONE',  ( -44.16309181155858710, 483.2448905683720000, -6.410867750099231266 ) ) ;
#11744=CARTESIAN_POINT ( 'NONE',  ( -38.17536295476246977, 515.4323905683720568, 14.20200298773971781 ) ) ;
#11746=CARTESIAN_POINT ( 'NONE',  ( -36.33955658999052218, 413.8698905765655809, 18.47759065022572500 ) ) ;
#11747=CARTESIAN_POINT ( 'NONE',  ( -48.68588794268852382, 251.6823905765656093, -3.978247347593583783 ) ) ;
#11749=CARTESIAN_POINT ( 'NONE',  ( -42.82802356641964536, 205.1437886375728965, -5.000000000000001776 ) ) ;
#11752=CARTESIAN_POINT ( 'NONE',  ( -43.15146482487497792, 202.0901544311013538, -3.972812079771461224 ) ) ;
#11753=CARTESIAN_POINT ( 'NONE',  ( -16.84014894278197971, 289.1198905683720568, 11.84573899990672530 ) ) ;
#11755=CARTESIAN_POINT ( 'NONE',  ( -48.68588794268870146, 277.2448905601784759, 0.000000000000000000 ) ) ;
#11757=CARTESIAN_POINT ( 'NONE',  ( -11.93348319268871371, 280.6823905683720000, -3.332260488124732856 ) ) ;
#11760=CARTESIAN_POINT ( 'NONE',  ( -19.19641293061500065, 511.9323905683721705, -14.20200298773971603 ) ) ;
#11762=ORIENTED_EDGE ( 'NONE', *, *, #8416, .T. ) ;
#11763=CARTESIAN_POINT ( 'NONE',  ( -13.20868407381887266, 460.9948905683720000, -6.410867750099233042 ) ) ;
#11765=CARTESIAN_POINT ( 'NONE',  ( -25.35362745456396638, 256.6823905683720000, 16.75240474999998952 ) ) ;
#11767=DIRECTION ( 'NONE',  ( -1.191790137725560488E-16, 1.000000000000000000, -0.000000000000000000 ) ) ;
#11768=CARTESIAN_POINT ( 'NONE',  ( -19.19641293061497223, 271.9323905683720568, -14.20200298773971603 ) ) ;
#11769=CARTESIAN_POINT ( 'NONE',  ( -38.17536295476243424, 246.9323905683720284, 14.20200298773971781 ) ) ;
#11770=CARTESIAN_POINT ( 'NONE',  ( -36.33955658999049376, 250.1198905765656377, -18.47759065022572855 ) ) ;
#11771=CARTESIAN_POINT ( 'NONE',  ( -36.33955658999050797, 309.1198905601785327, 18.47759065022572500 ) ) ;
#11772=CARTESIAN_POINT ( 'NONE',  ( -42.82802356641964536, 228.4948905601784759, 14.14213562373094923 ) ) ;
#11773=CARTESIAN_POINT ( 'NONE',  ( -16.84014894278197971, 260.1198905683720568, -11.84573899990672707 ) ) ;
#11774=CARTESIAN_POINT ( 'NONE',  ( -19.19641293061498644, 361.9323905683721136, -14.20200298773971603 ) ) ;
#11775=CARTESIAN_POINT ( 'NONE',  ( -36.33955658999052218, 505.3698905601784190, -18.47759065022572855 ) ) ;
#11777=ADVANCED_FACE ( 'NONE', ( #3419 ), #11741, .T. ) ;
#11778=CARTESIAN_POINT ( 'NONE',  ( -25.35362745456399480, 401.0573905683720000, -16.75240474999999307 ) ) ;
#11779=CARTESIAN_POINT ( 'NONE',  ( -8.685887942688720997, 336.9948905765656377, -2.449293598294705724E-15 ) ) ;
#11781=( BOUNDED_CURVE ( )  B_SPLINE_CURVE ( 2, ( #19142, #7550, #20764, #19242, #18911, #1195, #4319, #4425, #986, #4213, #10902, #2486, #1092, #14175, #20549, #876, #15690 ),
 .UNSPECIFIED., .F., .T. ) 
 B_SPLINE_CURVE_WITH_KNOTS ( ( 3, 2, 2, 2, 2, 2, 2, 2, 3 ),
 ( 0.7343750000000003331, 0.7363281250000003331, 0.7382812500000002220, 0.7402343750000002220, 0.7421875000000002220, 0.7441406250000002220, 0.7460937500000002220, 0.7480468750000001110, 0.7500000000000001110 ),
 .UNSPECIFIED. ) 
 CURVE ( )  GEOMETRIC_REPRESENTATION_ITEM ( )  RATIONAL_B_SPLINE_CURVE ( ( 0.9999999999999966693, 0.9807852804032337612, 1.000000000000000000, 0.9807852804032304306, 1.000000000000000000, 0.9807852804032304306, 1.000000000000000000, 0.9807852804032304306, 1.000000000000000000, 0.9807852804032304306, 1.000000000000000000, 0.9807852804032304306, 1.000000000000000000, 0.9807852804032304306, 1.000000000000000000, 0.9807852804032293204, 1.000000000000001110 ) ) 
 REPRESENTATION_ITEM ( '' )  );
#11782=CARTESIAN_POINT ( 'NONE',  ( -8.685887942688726326, 412.2448905601784759, -2.449293598294705724E-15 ) ) ;
#11786=CARTESIAN_POINT ( 'NONE',  ( -16.84014894278201169, 521.6198905683719431, -11.84573899990672707 ) ) ;
#11787=CARTESIAN_POINT ( 'NONE',  ( -48.68588794268870146, 287.5573905601784759, 3.978247347593168115 ) ) ;
#11788=CARTESIAN_POINT ( 'NONE',  ( -43.37443857369948574, 209.1166545091122657, -3.053198389463521956 ) ) ;
#11789=CARTESIAN_POINT ( 'NONE',  ( -45.43829269268870519, 325.6823905683720568, 3.332260488124734632 ) ) ;
#11791=CARTESIAN_POINT ( 'NONE',  ( -13.20868407381886023, 359.4948905683720000, -6.410867750099233042 ) ) ;
#11792=CARTESIAN_POINT ( 'NONE',  ( -22.27502019258948707, 360.7448905683720568, -15.47720386886985544 ) ) ;
#11793=EDGE_CURVE ( 'NONE', #19427, #11572, #2950, .T. ) ;
#11794=CARTESIAN_POINT ( 'NONE',  ( -45.64106924314017988, 301.0573905765656377, -11.32908994701042715 ) ) ;
#11796=CARTESIAN_POINT ( 'NONE',  ( -11.93348319268871016, 268.8698905683720000, -2.051577885510841163E-15 ) ) ;
#11797=CARTESIAN_POINT ( 'NONE',  ( -48.68588794268871567, 437.2448905601785327, 0.000000000000000000 ) ) ;
#11798=CARTESIAN_POINT ( 'NONE',  ( -40.53162694259544452, 416.6198905683720000, 11.84573899990672885 ) ) ;
#11800=CARTESIAN_POINT ( 'NONE',  ( -10.20829729246300310, 512.8698905601785327, -7.653668647301794969 ) ) ;
#11801=CARTESIAN_POINT ( 'NONE',  ( -21.03221929538690915, 360.3698905601784759, 18.47759065022572500 ) ) ;
#11803=CARTESIAN_POINT ( 'NONE',  ( -28.68588794268871922, 409.7448905601784759, 19.99999999999999289 ) ) ;
#11804=CARTESIAN_POINT ( 'NONE',  ( -45.43829269268869808, 325.0573905683719431, -3.332260488124726194 ) ) ;
#11805=CARTESIAN_POINT ( 'NONE',  ( -13.20868407381887266, 478.2448905683720568, 6.410867750099229490 ) ) ;
#11809=CARTESIAN_POINT ( 'NONE',  ( -36.33955658999052929, 459.1198905601784759, 18.47759065022572500 ) ) ;
#11810=CARTESIAN_POINT ( 'NONE',  ( -13.20868407381885135, 308.2448905683720000, 6.410867750099229490 ) ) ;
#11812=VERTEX_POINT ( 'NONE', #2021 ) ;
#11813=CARTESIAN_POINT ( 'NONE',  ( -14.54375231895776466, 345.7448905765655809, 14.14213562373094568 ) ) ;
#11815=DIRECTION ( 'NONE',  ( -1.191790137725560488E-16, 1.000000000000000000, -0.000000000000000000 ) ) ;
#11816=CARTESIAN_POINT ( 'NONE',  ( -14.48388495494900141, 381.3073905683720568, -9.489475012073734561 ) ) ;
#11817=CARTESIAN_POINT ( 'NONE',  ( -28.68588794268872633, 479.7448905601784759, 19.99999999999999289 ) ) ;
#11819=CARTESIAN_POINT ( 'NONE',  ( -13.20868407381886733, 428.2448905683720568, 6.410867750099229490 ) ) ;
#11820=CARTESIAN_POINT ( 'NONE',  ( -40.53162694259542320, 264.1198905683720568, -11.84573899990672707 ) ) ;
#11821=CARTESIAN_POINT ( 'NONE',  ( -42.88789093042844058, 432.9323905683719431, -9.489475012073734561 ) ) ;
#11823=CARTESIAN_POINT ( 'NONE',  ( -21.03221929538691271, 400.3698905601785327, 18.47759065022572500 ) ) ;
#11825=CARTESIAN_POINT ( 'NONE',  ( -21.03221929538690915, 355.1198905765656377, 18.47759065022572500 ) ) ;
#11828=CARTESIAN_POINT ( 'NONE',  ( -22.27502019258948351, 330.7448905683720568, -15.47720386886985544 ) ) ;
#11830=CARTESIAN_POINT ( 'NONE',  ( -42.88789093042844769, 486.3073905683721136, 9.489475012073736337 ) ) ;
#11831=CARTESIAN_POINT ( 'NONE',  ( -48.68588794268871567, 431.9948905765656377, 0.000000000000000000 ) ) ;
#11834=CARTESIAN_POINT ( 'NONE',  ( -28.68588794268871922, 392.8698905683720000, -16.75240474999999307 ) ) ;
#11837=CARTESIAN_POINT ( 'NONE',  ( -28.68588794268869790, 237.8698905683720568, 16.75240474999999307 ) ) ;
#11838=CARTESIAN_POINT ( 'NONE',  ( -44.16309181155857289, 373.2448905683720000, -6.410867750099231266 ) ) ;
#11840=CARTESIAN_POINT ( 'NONE',  ( -44.16309181155858710, 514.4948905683720568, 6.410867750099241924 ) ) ;
#11842=CARTESIAN_POINT ( 'NONE',  ( -16.84014894278200103, 441.6198905683720568, -11.84573899990672707 ) ) ;
#11843=CARTESIAN_POINT ( 'NONE',  ( -16.84014894278200813, 527.6198905683719431, 11.84573899990672530 ) ) ;
#11844=ORIENTED_EDGE ( 'NONE', *, *, #10318, .T. ) ;
#11845=CARTESIAN_POINT ( 'NONE',  ( -47.16347859291445843, 496.6198905601784759, -7.653668647301793193 ) ) ;
#11846=CARTESIAN_POINT ( 'NONE',  ( -14.48388495494901562, 489.8073905683720568, -9.489475012073736337 ) ) ;
#11848=VERTEX_POINT ( 'NONE', #13268 ) ;
#11849=CARTESIAN_POINT ( 'NONE',  ( -16.84014894278200458, 490.1198905683720000, -11.84573899990672707 ) ) ;
#11851=CARTESIAN_POINT ( 'NONE',  ( -48.68588794268871567, 422.3073905765656946, 3.978247347593168115 ) ) ;
#11853=CARTESIAN_POINT ( 'NONE',  ( -10.20829729246297291, 247.6198905765656377, -7.653668647301794969 ) ) ;
#11855=FACE_OUTER_BOUND ( 'NONE', #11270, .T. ) ;
#11857=DIRECTION ( 'NONE',  ( -1.191790137725560488E-16, 1.000000000000000000, -0.000000000000000000 ) ) ;
#11859=CARTESIAN_POINT ( 'NONE',  ( -32.01814843081344009, 307.5573905683719431, 16.75240474999999307 ) ) ;
#11861=CARTESIAN_POINT ( 'NONE',  ( -44.16309181155857999, 455.9948905683720000, 6.410867750099241924 ) ) ;
#11862=DIRECTION ( 'NONE',  ( -1.000000000000000000, -0.000000000000000000, -0.000000000000000000 ) ) ;
#11863=CARTESIAN_POINT ( 'NONE',  ( -40.53162694259543031, 294.1198905683720568, -11.84573899990672707 ) ) ;
#11864=EDGE_CURVE ( 'NONE', #6799, #5796, #5156, .T. ) ;
#11866=ORIENTED_EDGE ( 'NONE', *, *, #1654, .T. ) ;
#11867=CARTESIAN_POINT ( 'NONE',  ( -36.33955658999052929, 535.3698905601784190, -18.47759065022572855 ) ) ;
#11868=CARTESIAN_POINT ( 'NONE',  ( -44.16309181155858710, 494.7448905683720000, -6.410867750099231266 ) ) ;
#11873=CARTESIAN_POINT ( 'NONE',  ( -28.68588794268872277, 457.8698905683720000, 16.75240474999999307 ) ) ;
#11875=CARTESIAN_POINT ( 'NONE',  ( -35.09675569278793716, 255.7448905683720284, 15.47720386886985366 ) ) ;
#11876=ORIENTED_EDGE ( 'NONE', *, *, #7494, .T. ) ;
#11878=CARTESIAN_POINT ( 'NONE',  ( -45.43829269268869808, 235.6823905683720284, 3.332260488124734632 ) ) ;
#11882=CARTESIAN_POINT ( 'NONE',  ( -14.48388495494898720, 267.9323905683720568, 9.489475012073732785 ) ) ;
#11884=CARTESIAN_POINT ( 'NONE',  ( -25.35362745456398059, 348.1823905683720000, 16.75240474999998952 ) ) ;
#11885=CARTESIAN_POINT ( 'NONE',  ( -25.35362745456399836, 411.0573905683720568, -16.75240474999999307 ) ) ;
#11888=CARTESIAN_POINT ( 'NONE',  ( -47.16347859291445133, 407.8698905601784759, 7.653668647301805628 ) ) ;
#11893=CARTESIAN_POINT ( 'NONE',  ( -11.93348319268874036, 520.3698905683720568, -2.051577885510841163E-15 ) ) ;
#11894=CARTESIAN_POINT ( 'NONE',  ( -48.68588794268870146, 286.9323905601785327, -3.978247347593158345 ) ) ;
#11896=CARTESIAN_POINT ( 'NONE',  ( -25.35362745456397704, 318.1823905683720568, 16.75240474999998952 ) ) ;
#11898=CARTESIAN_POINT ( 'NONE',  ( -45.43829269268870519, 363.5573905683720568, -3.332260488124726194 ) ) ;
#11899=CARTESIAN_POINT ( 'NONE',  ( -13.20868407381885845, 358.2448905683720000, 6.410867750099229490 ) ) ;
#11900=CARTESIAN_POINT ( 'NONE',  ( -48.68588794268870146, 301.6823905765655809, -3.978247347593158345 ) ) ;
#11902=CARTESIAN_POINT ( 'NONE',  ( -45.43829269268869808, 264.1823905683719431, 3.332260488124734632 ) ) ;
#11904=CARTESIAN_POINT ( 'NONE',  ( -42.88789093042844058, 414.4323905683721136, -9.489475012073736337 ) ) ;
#11906=CARTESIAN_POINT ( 'NONE',  ( -48.68588794268872277, 451.9948905765656377, 0.000000000000000000 ) ) ;
#11907=CARTESIAN_POINT ( 'NONE',  ( -45.64106924314017277, 302.9323905765656946, 11.32908994701042538 ) ) ;
#11908=CARTESIAN_POINT ( 'NONE',  ( -36.33955658999052218, 409.1198905601784759, 18.47759065022572500 ) ) ;
#11909=CARTESIAN_POINT ( 'NONE',  ( -22.27502019258947286, 328.4948905683720568, 15.47720386886985189 ) ) ;
#11910=CARTESIAN_POINT ( 'NONE',  ( -11.93348319268873503, 468.5573905683720000, 3.332260488124728415 ) ) ;
#11912=CARTESIAN_POINT ( 'NONE',  ( -28.68588794268872277, 459.7448905601784759, 19.99999999999999289 ) ) ;
#11913=CARTESIAN_POINT ( 'NONE',  ( -44.16309181155856578, 293.2448905683720000, -6.410867750099231266 ) ) ;
#11914=ADVANCED_FACE ( 'NONE', ( #18753 ), #2329, .T. ) ;
#11915=CARTESIAN_POINT ( 'NONE',  ( -10.20829729246298356, 341.6198905601784759, 7.653668647301790529 ) ) ;
#11919=CARTESIAN_POINT ( 'NONE',  ( -16.84014894278199392, 391.6198905683720568, -11.84573899990672707 ) ) ;
#11920=CARTESIAN_POINT ( 'NONE',  ( -24.70764059509555821, 444.8073905765655809, 19.99999999999998934 ) ) ;
#11922=CARTESIAN_POINT ( 'NONE',  ( -48.68588794268887199, 382.3073905765655240, 3.978247347592742678 ) ) ;
#11923=CARTESIAN_POINT ( 'NONE',  ( -19.19641293061498999, 420.4323905683720000, -14.20200298773971603 ) ) ;
#11924=CARTESIAN_POINT ( 'NONE',  ( -11.93348319268871016, 270.3698905683720000, -2.051577885510841163E-15 ) ) ;
#11925=CARTESIAN_POINT ( 'NONE',  ( -16.84014894278199748, 420.1198905683720000, -11.84573899990672707 ) ) ;
#11927=CARTESIAN_POINT ( 'NONE',  ( -8.685887942688719221, 326.9948905765656377, -2.449293598294705724E-15 ) ) ;
#11928=CARTESIAN_POINT ( 'NONE',  ( -36.33955658999050797, 370.1198905765656377, -18.47759065022572855 ) ) ;
#11930=CARTESIAN_POINT ( 'NONE',  ( -32.01814843081344009, 321.6823905683720568, -16.75240474999999307 ) ) ;
#11932=CARTESIAN_POINT ( 'NONE',  ( -38.17536295476246977, 473.8073905683720000, -14.20200298773971426 ) ) ;
#11933=CARTESIAN_POINT ( 'NONE',  ( -47.16347859291445133, 432.6198905765656377, 7.653668647301805628 ) ) ;
#11936=CARTESIAN_POINT ( 'NONE',  ( -42.88789093042844058, 394.4323905683720000, -9.489475012073736337 ) ) ;
#11938=CARTESIAN_POINT ( 'NONE',  ( -10.20829729246300666, 532.8698905601785327, -7.653668647301794969 ) ) ;
#11939=CARTESIAN_POINT ( 'NONE',  ( -19.19641293061498288, 357.3073905683720568, 14.20200298773971426 ) ) ;
#11940=EDGE_CURVE ( 'NONE', #6694, #9649, #16346, .T. ) ;
#11942=CARTESIAN_POINT ( 'NONE',  ( -19.19641293061499709, 517.3073905683720568, 14.20200298773971426 ) ) ;
#11943=VERTEX_POINT ( 'NONE', #15639 ) ;
#11944=CARTESIAN_POINT ( 'NONE',  ( -45.64106924314018698, 356.3073905601785896, -11.32908994701042715 ) ) ;
#11945=CARTESIAN_POINT ( 'NONE',  ( -11.93348319268874214, 528.5573905683720568, 3.332260488124728415 ) ) ;
#11948=CARTESIAN_POINT ( 'NONE',  ( -19.19641293061499354, 477.3073905683720568, 14.20200298773971426 ) ) ;
#11950=CARTESIAN_POINT ( 'NONE',  ( -44.16309181155857999, 484.4948905683720000, 6.410867750099241924 ) ) ;
#11952=CARTESIAN_POINT ( 'NONE',  ( -8.685887942688728103, 417.3073905765656377, -3.978247347593165895 ) ) ;
#11953=CARTESIAN_POINT ( 'NONE',  ( -8.685887942688868435, 476.6823905765656377, 3.978247347593479866 ) ) ;
#11960=CARTESIAN_POINT ( 'NONE',  ( -45.43829269268869808, 295.6823905683720000, 3.332260488124734632 ) ) ;
#11962=CARTESIAN_POINT ( 'NONE',  ( -32.66413529028189089, 529.4323905601785327, 19.99999999999999289 ) ) ;
#11963=CARTESIAN_POINT ( 'NONE',  ( -45.43829269268871229, 445.6823905683720000, 3.332260488124734632 ) ) ;
#11964=CARTESIAN_POINT ( 'NONE',  ( -32.66413529028187668, 414.1823905765656946, 19.99999999999999289 ) ) ;
#11965=CARTESIAN_POINT ( 'NONE',  ( -42.88789093042842637, 274.4323905683720568, -9.489475012073736337 ) ) ;
#11968=CARTESIAN_POINT ( 'NONE',  ( -36.33955658999050087, 269.1198905601784759, 18.47759065022572500 ) ) ;
#11969=CARTESIAN_POINT ( 'NONE',  ( -13.20868407381887621, 499.7448905683720000, 6.410867750099229490 ) ) ;
#11971=ORIENTED_EDGE ( 'NONE', *, *, #18440, .T. ) ;
#11972=CARTESIAN_POINT ( 'NONE',  ( -40.53162694259545162, 466.6198905683720000, 11.84573899990672885 ) ) ;
#11973=CARTESIAN_POINT ( 'NONE',  ( -28.68588794268872277, 409.4948905765656377, -19.99999999999999289 ) ) ;
#11974=CARTESIAN_POINT ( 'NONE',  ( -13.20868407381884957, 269.4948905683720000, -6.410867750099233042 ) ) ;
#11975=ORIENTED_EDGE ( 'NONE', *, *, #21380, .T. ) ;
#11977=CARTESIAN_POINT ( 'NONE',  ( -28.68588794268870146, 267.8698905683720000, 16.75240474999999307 ) ) ;
#11979=CARTESIAN_POINT ( 'NONE',  ( -28.68588794268874054, 573.2448905601785327, 0.000000000000000000 ) ) ;
#11981=CARTESIAN_POINT ( 'NONE',  ( -32.01814843081343298, 253.1823905683720568, -16.75240474999999307 ) ) ;
#11982=CARTESIAN_POINT ( 'NONE',  ( -45.64106924314018698, 421.0573905765655809, -11.32908994701042538 ) ) ;
#11983=CARTESIAN_POINT ( 'NONE',  ( -40.01497788969912506, 235.6823905601785043, -16.95518130045146421 ) ) ;
#11984=CARTESIAN_POINT ( 'NONE',  ( -25.35362745456398059, 271.0573905683720000, -16.75240474999999307 ) ) ;
#11985=CARTESIAN_POINT ( 'NONE',  ( -16.84014894278198682, 359.1198905683720568, 11.84573899990672530 ) ) ;
#11989=CARTESIAN_POINT ( 'NONE',  ( -22.27502019258949062, 400.7448905683720568, -15.47720386886985544 ) ) ;
#11991=EDGE_CURVE ( 'NONE', #12371, #13587, #7916, .T. ) ;
#11992=CARTESIAN_POINT ( 'NONE',  ( -8.685887942688726326, 402.2448905601784759, -2.449293598294705724E-15 ) ) ;
#11994=ORIENTED_EDGE ( 'NONE', *, *, #5505, .T. ) ;
#11995=CARTESIAN_POINT ( 'NONE',  ( -14.54375231895776821, 348.2448905765656377, -14.14213562373094746 ) ) ;
#11998=LINE ( 'NONE', #8319, #12866 ) ;
#11999=CARTESIAN_POINT ( 'NONE',  ( -42.82802356641965247, 288.4948905601785327, 14.14213562373094923 ) ) ;
#12000=CARTESIAN_POINT ( 'NONE',  ( -17.35679799567829207, 318.5573905765656377, -16.95518130045146421 ) ) ;
#12001=CARTESIAN_POINT ( 'NONE',  ( -11.93348319268871549, 320.6823905683720000, -3.332260488124732856 ) ) ;
#12002=AXIS2_PLACEMENT_3D ( 'NONE', #15433, #15039, #10539 ) ;
#12004=CARTESIAN_POINT ( 'NONE',  ( -32.01814843081344719, 336.0573905683721136, 16.75240474999999307 ) ) ;
#12005=CARTESIAN_POINT ( 'NONE',  ( -45.43829269268871229, 363.5573905683720568, -3.332260488124726638 ) ) ;
#12007=CARTESIAN_POINT ( 'NONE',  ( -28.68588794268870501, 304.4948905765656377, 19.99999999999999289 ) ) ;
#12009=CARTESIAN_POINT ( 'NONE',  ( -13.20868407381884957, 269.4948905683720000, -6.410867750099233042 ) ) ;
#12010=CARTESIAN_POINT ( 'NONE',  ( -11.73070664223725856, 466.0573905765656946, 11.32908994701042005 ) ) ;
#12011=CARTESIAN_POINT ( 'NONE',  ( -35.09675569278795138, 423.4948905683720568, -15.47720386886985544 ) ) ;
#12012=LINE ( 'NONE', #18709, #15135 ) ;
#12013=CARTESIAN_POINT ( 'NONE',  ( -24.70764059509556887, 449.1823905765655809, -19.99999999999999289 ) ) ;
#12015=CARTESIAN_POINT ( 'NONE',  ( -11.93348319268871904, 330.0573905683720568, 3.332260488124728415 ) ) ;
#12016=CARTESIAN_POINT ( 'NONE',  ( -42.88789093042844769, 472.9323905683720000, -9.489475012073736337 ) ) ;
#12018=CARTESIAN_POINT ( 'NONE',  ( -45.64106924314020119, 458.1823905601784190, 11.32908994701042715 ) ) ;
#12019=CARTESIAN_POINT ( 'NONE',  ( -45.43829269268869808, 283.5573905683720568, -3.332260488124726194 ) ) ;
#12022=DIRECTION ( 'NONE',  ( -1.000000000000000000, 0.000000000000000000, 0.000000000000000000 ) ) ;
#12023=CARTESIAN_POINT ( 'NONE',  ( -32.66413529028187668, 339.4323905601784759, 19.99999999999999289 ) ) ;
#12024=CARTESIAN_POINT ( 'NONE',  ( -44.16309181155856578, 293.2448905683720000, -6.410867750099231266 ) ) ;
#12025=CARTESIAN_POINT ( 'NONE',  ( -22.27502019258947996, 388.4948905683720000, 15.47720386886985189 ) ) ;
#12026=CARTESIAN_POINT ( 'NONE',  ( -21.03221929538689494, 230.3698905601784759, 18.47759065022572500 ) ) ;
#12027=CARTESIAN_POINT ( 'NONE',  ( -47.16347859291446554, 531.3698905765655809, -7.653668647301793193 ) ) ;
#12028=CARTESIAN_POINT ( 'NONE',  ( -25.35362745456398770, 416.6823905683720568, 16.75240474999998952 ) ) ;
#12029=CARTESIAN_POINT ( 'NONE',  ( -11.93348319268871016, 260.0573905683720000, 3.332260488124728415 ) ) ;
#12030=CARTESIAN_POINT ( 'NONE',  ( -13.20868407381886911, 429.4948905683720568, -6.410867750099233042 ) ) ;
#12032=CARTESIAN_POINT ( 'NONE',  ( -24.70764059509556176, 359.1823905765655809, -19.99999999999999289 ) ) ;
#12033=CARTESIAN_POINT ( 'NONE',  ( -8.685887942688534480, 272.5573905601784190, -3.978247347592740013 ) ) ;
#12034=CARTESIAN_POINT ( 'NONE',  ( -11.93348319268871549, 318.5573905683719431, 3.332260488124728859 ) ) ;
#12035=( BOUNDED_CURVE ( )  B_SPLINE_CURVE ( 2, ( #5604, #10895, #13838, #2478, #4205, #14168, #17504, #5707, #12211, #15575, #2695, #20645, #5815, #10569, #17405, #761, #19132 ),
 .UNSPECIFIED., .F., .T. ) 
 B_SPLINE_CURVE_WITH_KNOTS ( ( 3, 2, 2, 2, 2, 2, 2, 2, 3 ),
 ( 0.6406250000000002220, 0.6425781250000002220, 0.6445312500000002220, 0.6464843750000002220, 0.6484375000000002220, 0.6503906250000002220, 0.6523437500000002220, 0.6542968750000002220, 0.6562500000000002220 ),
 .UNSPECIFIED. ) 
 CURVE ( )  GEOMETRIC_REPRESENTATION_ITEM ( )  RATIONAL_B_SPLINE_CURVE ( ( 0.9999999999999977796, 0.9807852804032326510, 1.000000000000000000, 0.9807852804032304306, 1.000000000000000000, 0.9807852804032304306, 1.000000000000000000, 0.9807852804032304306, 1.000000000000000000, 0.9807852804032304306, 1.000000000000000000, 0.9807852804032304306, 1.000000000000000000, 0.9807852804032304306, 1.000000000000000000, 0.9807852804032282101, 1.000000000000002220 ) ) 
 REPRESENTATION_ITEM ( '' )  );
#12036=CARTESIAN_POINT ( 'NONE',  ( -32.01814843081346140, 473.1823905683720000, -16.75240474999999307 ) ) ;
#12039=CARTESIAN_POINT ( 'NONE',  ( -35.86044580198795018, 223.9104597372275123, 18.66884633871304899 ) ) ;
#12041=CARTESIAN_POINT ( 'NONE',  ( -14.48388495494900141, 381.3073905683720568, -9.489475012073736337 ) ) ;
#12044=CARTESIAN_POINT ( 'NONE',  ( -42.82802356641968089, 528.4948905601785327, 14.14213562373094923 ) ) ;
#12045=CARTESIAN_POINT ( 'NONE',  ( -11.93348319268872260, 338.5573905683720568, 3.332260488124728415 ) ) ;
#12048=CARTESIAN_POINT ( 'NONE',  ( -35.09675569278796559, 521.9948905683720568, -15.47720386886985544 ) ) ;
#12050=CARTESIAN_POINT ( 'NONE',  ( -40.01497788969913927, 355.6823905601784759, -16.95518130045146421 ) ) ;
#12051=CARTESIAN_POINT ( 'NONE',  ( -8.685887942688546914, 377.3073905765656377, -3.978247347592740013 ) ) ;
#12052=CARTESIAN_POINT ( 'NONE',  ( -10.20829729246297113, 227.6198905765656093, -7.653668647301794969 ) ) ;
#12055=CARTESIAN_POINT ( 'NONE',  ( -25.35362745456399480, 486.6823905683720568, 16.75240474999998952 ) ) ;
#12057=CARTESIAN_POINT ( 'NONE',  ( -32.01814843081345430, 481.6823905683720568, -16.75240474999999307 ) ) ;
#12059=CARTESIAN_POINT ( 'NONE',  ( -14.54375231895777354, 415.7448905765655809, 14.14213562373094568 ) ) ;
#12060=CARTESIAN_POINT ( 'NONE',  ( -8.685887942688715668, 296.9948905765655809, -2.449293598294705724E-15 ) ) ;
#12064=CARTESIAN_POINT ( 'NONE',  ( -8.685887942688733432, 462.2448905601784759, -2.449293598294705724E-15 ) ) ;
#12067=CARTESIAN_POINT ( 'NONE',  ( -16.84014894278198327, 301.6198905683720000, -11.84573899990672707 ) ) ;
#12068=CARTESIAN_POINT ( 'NONE',  ( -21.03221929538693047, 530.3698905601784190, 18.47759065022572500 ) ) ;
#12069=CARTESIAN_POINT ( 'NONE',  ( -13.20868407381886733, 439.7448905683720000, 6.410867750099229490 ) ) ;
#12070=CARTESIAN_POINT ( 'NONE',  ( -48.68588794268870856, 331.9948905765656377, 0.000000000000000000 ) ) ;
#12071=CARTESIAN_POINT ( 'NONE',  ( -16.84014894278197971, 271.6198905683720568, -11.84573899990672707 ) ) ;
#12074=CARTESIAN_POINT ( 'NONE',  ( -13.20868407381887266, 479.7448905683720568, 6.410867750099229490 ) ) ;
#12078=CARTESIAN_POINT ( 'NONE',  ( -22.27502019258948351, 428.4948905683720568, 15.47720386886985189 ) ) ;
#12080=CARTESIAN_POINT ( 'NONE',  ( -35.09675569278793006, 251.9948905683720568, -15.47720386886985544 ) ) ;
#12081=ORIENTED_EDGE ( 'NONE', *, *, #10365, .T. ) ;
#12083=CARTESIAN_POINT ( 'NONE',  ( -32.66413529028189089, 474.1823905765655809, 19.99999999999999289 ) ) ;
#12085=MANIFOLD_SOLID_BREP ( 'Cut-Extrude10[2]', #12445 ) ;
#12086=CARTESIAN_POINT ( 'NONE',  ( -44.16309181155855867, 244.7448905683720000, -6.410867750099231266 ) ) ;
#12087=ADVANCED_FACE ( 'NONE', ( #6195 ), #12807, .T. ) ;
#12088=CARTESIAN_POINT ( 'NONE',  ( -45.43829269268873361, 515.3698905683720568, 0.000000000000000000 ) ) ;
#12089=CARTESIAN_POINT ( 'NONE',  ( -11.73070664223723014, 231.3073905601784475, 11.32908994701042005 ) ) ;
#12090=CARTESIAN_POINT ( 'NONE',  ( -13.20868407381884602, 248.2448905683720000, 6.410867750099229490 ) ) ;
#12091=B_SPLINE_CURVE_WITH_KNOTS ( 'NONE', 1,
 ( #2338, #3844 ),
 .UNSPECIFIED., .F., .F.,
 ( 2, 2 ),
 ( 0.000000000000000000, 1.000000000000000000 ),
 .UNSPECIFIED. ) ;
#12092=CARTESIAN_POINT ( 'NONE',  ( -45.43829269268871229, 365.3698905683720568, 0.000000000000000000 ) ) ;
#12094=( BOUNDED_CURVE ( )  B_SPLINE_CURVE ( 2, ( #16575, #15167, #1761, #13432, #19694, #8331, #14953, #140, #16683, #5302, #1871, #8441, #3581, #5199, #247, #20025, #11797 ),
 .UNSPECIFIED., .F., .T. ) 
 B_SPLINE_CURVE_WITH_KNOTS ( ( 3, 2, 2, 2, 2, 2, 2, 2, 3 ),
 ( 0.2968750000000001110, 0.2988281250000001110, 0.3007812500000001110, 0.3027343750000001110, 0.3046875000000001110, 0.3066406250000001110, 0.3085937500000001110, 0.3105468750000001110, 0.3125000000000001110 ),
 .UNSPECIFIED. ) 
 CURVE ( )  GEOMETRIC_REPRESENTATION_ITEM ( )  RATIONAL_B_SPLINE_CURVE ( ( 0.9999999999999988898, 0.9807852804032315408, 1.000000000000000000, 0.9807852804032304306, 1.000000000000000000, 0.9807852804032304306, 1.000000000000000000, 0.9807852804032304306, 1.000000000000000000, 0.9807852804032304306, 1.000000000000000000, 0.9807852804032304306, 1.000000000000000000, 0.9807852804032304306, 1.000000000000000000, 0.9807852804032293204, 1.000000000000001110 ) ) 
 REPRESENTATION_ITEM ( '' )  );
#12095=CARTESIAN_POINT ( 'NONE',  ( -25.35362745456398414, 396.6823905683720000, 16.75240474999998952 ) ) ;
#12098=CARTESIAN_POINT ( 'NONE',  ( -14.54375231895777532, 403.4948905601784759, -14.14213562373094746 ) ) ;
#12099=ORIENTED_EDGE ( 'NONE', *, *, #8908, .F. ) ;
#12102=ORIENTED_EDGE ( 'NONE', *, *, #8908, .T. ) ;
#12103=CARTESIAN_POINT ( 'NONE',  ( -13.20868407381887799, 519.7448905683720568, 6.410867750099229490 ) ) ;
#12104=CARTESIAN_POINT ( 'NONE',  ( -28.68588794268870856, 294.7448905601784759, -19.99999999999999289 ) ) ;
#12105=CARTESIAN_POINT ( 'NONE',  ( -32.66413529028186247, 319.8073905765655809, -19.99999999999999289 ) ) ;
#12106=CARTESIAN_POINT ( 'NONE',  ( -11.93348319268871727, 330.3698905683720000, -2.051577885510841163E-15 ) ) ;
#12109=CARTESIAN_POINT ( 'NONE',  ( -11.93348319268871904, 348.8698905683720568, -2.051577885510841163E-15 ) ) ;
#12110=CARTESIAN_POINT ( 'NONE',  ( -45.43829269268871229, 373.8698905683720000, 0.000000000000000000 ) ) ;
#12112=CARTESIAN_POINT ( 'NONE',  ( -28.68588794268870856, 289.4948905765656377, -19.99999999999999289 ) ) ;
#12115=CARTESIAN_POINT ( 'NONE',  ( -16.84014894278197616, 267.6198905683720568, 11.84573899990672530 ) ) ;
#12116=CARTESIAN_POINT ( 'NONE',  ( -43.68588794268869435, 200.1437886375728965, -2.037320803886357560E-15 ) ) ;
#12119=CARTESIAN_POINT ( 'NONE',  ( -22.27502019258949417, 412.2448905683720568, -15.47720386886985544 ) ) ;
#12121=CARTESIAN_POINT ( 'NONE',  ( -14.54375231895776821, 353.4948905601785327, -14.14213562373094746 ) ) ;
#12123=CARTESIAN_POINT ( 'NONE',  ( -47.16347859291445133, 407.8698905601784759, 7.653668647301805628 ) ) ;
#12124=CARTESIAN_POINT ( 'NONE',  ( -35.09675569278794427, 333.4948905683720568, -15.47720386886985544 ) ) ;
#12125=CARTESIAN_POINT ( 'NONE',  ( -28.68588794268872988, 471.3698905683720568, -16.75240474999999307 ) ) ;
#12127=CARTESIAN_POINT ( 'NONE',  ( -17.35679799567830273, 460.6823905601784759, 16.95518130045146421 ) ) ;
#12128=CARTESIAN_POINT ( 'NONE',  ( -13.20868407381884957, 288.2448905683720000, 6.410867750099229490 ) ) ;
#12130=ORIENTED_EDGE ( 'NONE', *, *, #18674, .T. ) ;
#12131=CARTESIAN_POINT ( 'NONE',  ( -24.70764059509554755, 340.0573905601784190, 19.99999999999998934 ) ) ;
#12132=ORIENTED_EDGE ( 'NONE', *, *, #18687, .T. ) ;
#12134=CARTESIAN_POINT ( 'NONE',  ( -42.82802356641965957, 338.4948905601785327, 14.14213562373094923 ) ) ;
#12136=CARTESIAN_POINT ( 'NONE',  ( -40.53162694259543031, 292.6198905683720000, -11.84573899990672707 ) ) ;
#12138=CARTESIAN_POINT ( 'NONE',  ( -38.17536295476244845, 386.9323905683721136, 14.20200298773971781 ) ) ;
#12139=CARTESIAN_POINT ( 'NONE',  ( -17.35679799567829562, 373.8073905601784759, -16.95518130045146421 ) ) ;
#12140=CARTESIAN_POINT ( 'NONE',  ( -8.685887942688744090, 526.6823905765655809, 3.978247347593161010 ) ) ;
#12141=CARTESIAN_POINT ( 'NONE',  ( -19.19641293061498999, 410.4323905683720568, -14.20200298773971603 ) ) ;
#12142=CARTESIAN_POINT ( 'NONE',  ( -40.53162694259542320, 254.1198905683720284, -11.84573899990672707 ) ) ;
#12143=CARTESIAN_POINT ( 'NONE',  ( -45.43829269268871940, 423.5573905683720000, -3.332260488124726638 ) ) ;
#12145=CARTESIAN_POINT ( 'NONE',  ( -28.68588794268871212, 344.4948905765656377, 19.99999999999999289 ) ) ;
#12146=CARTESIAN_POINT ( 'NONE',  ( -8.685887942688708563, 236.9948905765656377, -2.449293598294705724E-15 ) ) ;
#12147=CARTESIAN_POINT ( 'NONE',  ( -13.20868407381885490, 328.2448905683720000, 6.410867750099229490 ) ) ;
#12148=CARTESIAN_POINT ( 'NONE',  ( -40.53162694259545162, 484.1198905683720000, -11.84573899990672707 ) ) ;
#12149=ADVANCED_FACE ( 'NONE', ( #3288 ), #16911, .T. ) ;
#12153=CARTESIAN_POINT ( 'NONE',  ( -8.685887942688795604, 226.6823905765656377, 3.978247347593374172 ) ) ;
#12154=CARTESIAN_POINT ( 'NONE',  ( -19.19641293061498644, 378.8073905683721136, 14.20200298773971426 ) ) ;
#12156=CARTESIAN_POINT ( 'NONE',  ( -17.35679799567831694, 523.8073905601785327, -16.95518130045146421 ) ) ;
#12157=CARTESIAN_POINT ( 'NONE',  ( -22.27502019258948707, 350.7448905683720568, -15.47720386886985544 ) ) ;
#12159=CARTESIAN_POINT ( 'NONE',  ( -22.27502019258949417, 506.9948905683721136, 15.47720386886985189 ) ) ;
#12162=CARTESIAN_POINT ( 'NONE',  ( -28.68588794268871212, 349.7448905601784759, 19.99999999999999289 ) ) ;
#12163=CARTESIAN_POINT ( 'NONE',  ( -36.33955658999050797, 380.1198905765656377, -18.47759065022572855 ) ) ;
#12166=CARTESIAN_POINT ( 'NONE',  ( -32.01814843081346140, 466.0573905683720000, 16.75240474999999307 ) ) ;
#12168=VERTEX_POINT ( 'NONE', #14870 ) ;
#12169=CARTESIAN_POINT ( 'NONE',  ( -25.35362745456400546, 481.0573905683720568, -16.75240474999999307 ) ) ;
#12170=( BOUNDED_CURVE ( )  B_SPLINE_CURVE ( 2, ( #8024, #14230, #1240, #20818, #12701, #4478, #14656, #7814, #15954, #6403, #10955, #5988, #12598, #11061, #14444, #6194, #19398 ),
 .UNSPECIFIED., .F., .T. ) 
 B_SPLINE_CURVE_WITH_KNOTS ( ( 3, 2, 2, 2, 2, 2, 2, 2, 3 ),
 ( 0.4218750000000001665, 0.4238281250000001665, 0.4257812500000001665, 0.4277343750000001665, 0.4296875000000002220, 0.4316406250000002220, 0.4335937500000002220, 0.4355468750000002220, 0.4375000000000002220 ),
 .UNSPECIFIED. ) 
 CURVE ( )  GEOMETRIC_REPRESENTATION_ITEM ( )  RATIONAL_B_SPLINE_CURVE ( ( 0.9999999999999983347, 0.9807852804032320959, 1.000000000000000000, 0.9807852804032304306, 1.000000000000000000, 0.9807852804032304306, 1.000000000000000000, 0.9807852804032304306, 1.000000000000000000, 0.9807852804032304306, 1.000000000000000000, 0.9807852804032304306, 1.000000000000000000, 0.9807852804032304306, 1.000000000000000000, 0.9807852804032282101, 1.000000000000002220 ) ) 
 REPRESENTATION_ITEM ( '' )  );
#12172=CARTESIAN_POINT ( 'NONE',  ( -24.70764059509556887, 419.1823905765655809, -19.99999999999999289 ) ) ;
#12173=CARTESIAN_POINT ( 'NONE',  ( -14.54375231895778064, 475.7448905765655809, 14.14213562373094568 ) ) ;
#12175=CARTESIAN_POINT ( 'NONE',  ( -42.82802356641967378, 485.9948905601784759, -14.14213562373094746 ) ) ;
#12181=CARTESIAN_POINT ( 'NONE',  ( -32.01814843081344009, 283.1823905683720568, -16.75240474999999307 ) ) ;
#12182=CARTESIAN_POINT ( 'NONE',  ( -47.16347859291443001, 247.8698905601785043, 7.653668647301805628 ) ) ;
#12184=CARTESIAN_POINT ( 'NONE',  ( -45.43829269268871940, 455.6823905683720000, 3.332260488124734632 ) ) ;
#12186=CARTESIAN_POINT ( 'NONE',  ( -38.17536295476244135, 263.8073905683720568, -14.20200298773971426 ) ) ;
#12188=CARTESIAN_POINT ( 'NONE',  ( -47.16347859291445843, 481.3698905765655809, -7.653668647301793193 ) ) ;
#12189=CARTESIAN_POINT ( 'NONE',  ( -19.19641293061500065, 491.9323905683720000, -14.20200298773971603 ) ) ;
#12192=CYLINDRICAL_SURFACE ( 'NONE', #724, 19.99999999999999645 ) ;
#12193=CARTESIAN_POINT ( 'NONE',  ( -28.68588794268869790, 236.3698905683720568, 16.75240474999999307 ) ) ;
#12196=CARTESIAN_POINT ( 'NONE',  ( -40.01497788969914637, 473.5573905765655809, 16.95518130045146776 ) ) ;
#12200=CARTESIAN_POINT ( 'NONE',  ( -32.01814843081343298, 247.5573905683720000, 16.75240474999999307 ) ) ;
#12201=CARTESIAN_POINT ( 'NONE',  ( -44.16309181155858710, 515.9948905683720568, 6.410867750099241924 ) ) ;
#12203=CARTESIAN_POINT ( 'NONE',  ( -25.35362745456396638, 246.6823905683720284, 16.75240474999998952 ) ) ;
#12204=CARTESIAN_POINT ( 'NONE',  ( -45.43829269268871229, 335.3698905683720000, 0.000000000000000000 ) ) ;
#12205=EDGE_CURVE ( 'NONE', #502, #8850, #1561, .T. ) ;
#12209=CARTESIAN_POINT ( 'NONE',  ( -38.17536295476246266, 402.3073905683720000, -14.20200298773971426 ) ) ;
#12211=CARTESIAN_POINT ( 'NONE',  ( -28.68588794268870856, 324.4948905765655809, 19.99999999999999289 ) ) ;
#12212=CARTESIAN_POINT ( 'NONE',  ( -28.68588794268871567, 399.7448905601784759, 19.99999999999999289 ) ) ;
#12215=ADVANCED_FACE ( 'NONE', ( #18412 ), #16806, .T. ) ;
#12216=CARTESIAN_POINT ( 'NONE',  ( -48.68588794268861619, 351.6823905765656946, -3.978247347593371508 ) ) ;
#12219=CARTESIAN_POINT ( 'NONE',  ( -25.35362745456400901, 512.5573905683719431, -16.75240474999999307 ) ) ;
#12220=CARTESIAN_POINT ( 'NONE',  ( -14.54375231895776466, 318.2448905765656377, -14.14213562373094746 ) ) ;
#12223=CARTESIAN_POINT ( 'NONE',  ( -42.88789093042842637, 304.4323905683720000, -9.489475012073734561 ) ) ;
#12225=CARTESIAN_POINT ( 'NONE',  ( -32.01814843081344719, 346.0573905683720568, 16.75240474999999307 ) ) ;
#12226=CARTESIAN_POINT ( 'NONE',  ( -38.17536295476245556, 352.3073905683719431, -14.20200298773971426 ) ) ;
#12228=CARTESIAN_POINT ( 'NONE',  ( -21.03221929538690205, 285.1198905765656377, 18.47759065022572500 ) ) ;
#12229=CARTESIAN_POINT ( 'NONE',  ( -45.64106924314019409, 501.0573905765656377, -11.32908994701042538 ) ) ;
#12230=CARTESIAN_POINT ( 'NONE',  ( -40.53162694259542320, 245.1198905683720284, 11.84573899990672885 ) ) ;
#12232=( BOUNDED_CURVE ( )  B_SPLINE_CURVE ( 2, ( #4507, #6122, #19219, #9579, #15989, #12730, #9477, #10772, #19000, #21160, #6334, #16088, #14371, #17805, #21054, #14473, #1170, #4186, #1267, #6224, #11097, #19321, #17486, #7844, #7742, #16195, #7944, #17700, #11207, #4297, #12839, #17388, #1374, #10881, #14576, #2995, #2571, #9150, #15879, #14151, #15772, #7526, #20738, #2786, #12628, #2676, #5911, #19115, #6019, #9262, #1068, #7637, #4402, #9373, #14262, #20849, #10985, #17594, #4816, #11744, #3099, #14789, #19636, #21264, #18336, #13158, #12946, #18120, #15112, #16306, #16517, #15006, #11410, #8056, #4930, #14687, #8382, #3422, #1479, #10113, #13047, #3315, #9894, #3208, #5034, #18230, #16734, #1921, #11308, #8489, #296, #9787, #9682, #13377, #6432, #19534, #18015, #16624, #16410, #1588, #8158, #21373, #6541, #19746, #17904, #11527, #1699, #5146, #8267, #14898, #84, #4711, #6650, #13272, #19857, #10001, #11635, #1815, #192, #6759, #19967, #2332, #10426, #13484, #18756, #8913, #20389, #510, #15215, #17047, #18445, #406, #15643, #5250, #6865, #7176, #3731, #15426, #6971, #5455, #11849, #10529, #20077, #8809, #10316, #2024, #3631, #10213, #8703, #18544, #16836, #12278, #611, #13693, #7073, #5563, #13798, #16940, #11950, #13594, #20181, #2122, #5349, #15325, #20285, #5670, #8592, #12057, #17151, #12169, #18645, #3837, #3944, #7287, #2228, #15534, #20500, #715, #13911, #18859, #4049, #10638, #17256, #2439, #9020, #2972, #9125, #12602, #19194, #12496, #14344, #6091, #21028, #12811, #20600, #6198, #11177, #19087, #12380, #1243, #15747, #19402, #9337, #9550, #17779, #18973, #4482, #14123, #17460, #17361, #5773, #934, #7500, #14448, #10856, #20710, #15855, #14021, #828, #10959, #4373, #17568, #7394, #2760, #4269, #15958, #17672, #4154, #7817, #10746, #20924, #7715, #1144, #1039, #4585, #12705, #19297, #11065, #2542, #5883, #2649, #9235, #2866, #7603, #9449, #14234, #20823, #5992, #16067, #12918, #16170, #17878, #21133, #14548, #5008, #13019, #3396, #6306, #52, #19507, #1346, #14977, #18199, #11608, #19718, #7919, #6622, #9976, #8241, #9761, #3071, #4902, #4685, #9655, #3497, #11280, #16277, #16490, #19611, #3290, #1453, #8026, #19938, #19833, #14659, #18095, #4788, #21240, #6406, #11385, #17984, #3182, #16385, #164, #9864, #1560, #8130, #14872, #1672, #14762, #21347, #6515, #13131, #11498, #13243, #16596, #1786, #6735, #8353, #13350, #5116, #11716, #18308, #10084, #15402, #10507, #3604, #18622, #2307, #13670, #13568, #5223, #2096, #11821, #5538, #585, #20046, #15507, #10188, #15299, #18415, #5646, #16809, #12253, #12030, #2201, #20363, #20476, #1894, #7153, #13885, #17128, #1999, #692, #8568, #13774, #271, #20156, #6945, #16706, #15189, #18836, #3810, #12143, #8890, #18731, #8461, #6838, #374, #5324, #15086, #20259, #5430, #3917, #11925, #18519, #3705, #8675, #10293, #7261, #13454, #16914, #486, #7050, #10401, #17020, #8786, #13997, #6174, #5965, #17544, #2415, #2842, #14425, #15723, #15616, #4454, #12357, #16044, #4129, #7692, #804, #7472, #908, #10614, #20578, #7792, #12578, #9314, #11039, #6068, #14102, #18944, #19063, #17232, #21006, #14209, #7581, #15932, #5746, #17335, #2519, #15831, #8995, #4350, #10718, #20683, #9102, #5858, #7369, #4021, #1222, #1015, #19172, #1120, #12466, #4246, #12785, #10830, #14321, #20797, #9425, #12679, #20900, #10933, #17440, #19273, #17650, #2734, #2624, #9206, #1645, #16357, #16569, #8327, #8105, #11582, #4664, #3263, #17755, #1755, #11255, #14949, #8217, #11151, #21317, #16250, #14523, #2946, #9525, #21218, #3157, #12992, #17854, #1535, #21, #6383, #6597, #18068, #13218, #19585, #9736, #14735, #9631, #19484, #12895, #3048, #18173, #16143, #1324, #14846, #6488, #19378, #9839, #19805, #1429, #13105, #3371, #19690, #8001, #9949, #4876, #21109, #11470, #7895, #4983, #16462, #4765, #14634, #136, #6709, #4563, #6280, #11360, #17957, #6812, #13428, #8644, #3577, #5510, #2279, #16995, #12110, #1970, #15163, #20019, #242, #18703, #13540, #13326, #18492, #456, #3889, #16885, #16784, #10478, #2069, #8541, #7125, #15272, #2173, #20230, #15480, #5195, #3681, #10266, #10166, #5400, #18596, #17100, #8859, #665, #5089, #3780, #19908, #12005, #11690, #20129, #18281, #7022, #3469, #10056, #16679, #8759, #11792, #351, #8437, #1867, #18388, #6914, #15060, #5297, #11899, #13644, #10370, #15378, #556, #13751, #20337, #13855, #17417, #4101, #9179, #2709, #5618, #14581, #10582, #5939, #14180, #15804, #7446, #12226, #18809, #17518, #10689, #16200, #3991, #12553, #17205, #20445, #10907, #16311, #1378, #7231, #12950, #19147, #20554, #13971, #17908, #991, #5720, #2384, #15591, #8967, #776, #7338, #7555, #17308, #20771, #12328, #5827, #18916, #10802, #15695, #2599, #20657, #14072, #19034, #4220, #2493, #4324, #9585, #7950, #21165, #3105, #9075, #6337, #11314, #19539, #882, #12437, #4716, #9688, #13889, #15512, #16711, #8790, #18422, #381, #277, #10090, #5541, #7157, #5122, #1900, #10194, #8573, #8468, #11722, #13779, #11828, #8679, #18314, #15303, #2005, #7055, #589, #3504, #12147, #15092, #3814, #6845, #13460, #20053, #5229, #3609, #15409, #15196, #20367, #16816, #10406, #6951, #13572, #18736, #20162, #3920, #5329, #10510, #17023, #11930, #18523, #3709, #10296, #490, #16920, #2101, #13673, #20263, #5433, #12034, #18626, #2204, #17132, #2312, #8894, #695, #7265, #2628, #12470, #20688, #15619, #18839, #913, #10722, #4026, #4457, #1020, #5863, #19066, #19175, #20800, #17338, #4132, #14001, #20581, #15833, #2523, #12683, #9429, #2738, #19276, #10619, #9318, #12581, #10835, #20479, #4353, #20903, #5751, #7584, #11042, #9212, #9105, #17653, #14213, #15726, #14324, #5968, #15935, #10937, #1225, #5650, #17548, #7475, #1124, #7695, #17235, #6071, #2418, #2845, #16047, #7796, #4249, #12256, #17442, #8999, #807, #7373, #12361, #18951, #14105, #21009, #18071, #1760, #8221, #14429, #19809, #13109, #6283, #21112, #3375, #8109, #12898, #3267, #11364, #11585, #9952, #3161, #6600, #19487, #19693, #18177, #4668, #16574, #9842, #6178, #16360, #11258, #9528, #12788, #19381, #16253, #17858, #4566, #4986, #1538, #21222, #14637, #4879, #14740, #3051, #8004, #4769, #17960, #9635, #14526, #7898, #1432, #13221, #11155, #17759, #16466, #6492, #9739, #2949, #11474, #14850, #6386, #21322, #16147, #1649, #12997, #1327, #19590, #24, #3784, #20233, #18285, #13754, #8440, #13543, #16682, #3892, #3474, #10483, #10271, #459, #18601, #18706, #139, #13648, #19912, #8762, #1870, #20340, #15064, #12009, #5093, #11796, #5198, #14952, #10060, #12115, #16888, #5404, #15382, #10375, #8330, #11694, #13431, #18392, #17103, #18495, #11902, #16998, #246, #2177, #3684, #561, #15276, #6713, #6816, #20133, #5301, #20024, #7026, #7128, #5515, #13329, #3580, #10169, #16787, #1975, #8545, #15166, #355, #6919, #2072, #8649, #12655, #13861, #5942, #15595, #18920, #18813, #7234, #17208, #2387, #15908, #12332, #8970, #5724, #20448, #2283, #4327, #780, #5831, #8863, #12440, #20557, #4223, #19152, #668, #9293, #5621, #995, #9182, #10806, #2496, #14296, #20660, #12557, #4104, #10910, #12230, #7558, #3994, #15483, #17522, #11016, #2712, #10587, #7669, #14184, #7341, #13975, #19250, #17421, #10692, #1100, #19039, #17313, #9078, #15699, #2602, #885, #15808, #7449, #14077, #20776, #20881, #6047, #4432, #9610, #17832, #12762, #3131, #20982, #3241, #1405, #11235, #19562, #3028, #16228, #16337, #17935, #7873, #1299, #11126, #17731, #12972, #14502, #9816, #6573, #21292, #16440, #6258, #19460, #2925, #4541, #1619, #1511, #18047, #9505, #4743, #8192, #21193, #21085, #14821, #6362, #12870, #11341, #4644 ),
 .UNSPECIFIED., .F., .T. ) 
 B_SPLINE_CURVE_WITH_KNOTS ( ( 3, 2, 2, 2, 2, 2, 2, 2, 2, 2, 2, 2, 2, 2, 2, 2, 2, 2, 2, 2, 2, 2, 2, 2, 2, 2, 2, 2, 2, 2, 2, 2, 2, 2, 2, 2, 2, 2, 2, 2, 2, 2, 2, 2, 2, 2, 2, 2, 2, 2, 2, 2, 2, 2, 2, 2, 2, 2, 2, 2, 2, 2, 2, 2, 2, 2, 2, 2, 2, 2, 2, 2, 2, 2, 2, 2, 2, 2, 2, 2, 2, 2, 2, 2, 2, 2, 2, 2, 2, 2, 2, 2, 2, 2, 2, 2, 2, 2, 2, 2, 2, 2, 2, 2, 2, 2, 2, 2, 2, 2, 2, 2, 2, 2, 2, 2, 2, 2, 2, 2, 2, 2, 2, 2, 2, 2, 2, 2, 2, 2, 2, 2, 2, 2, 2, 2, 2, 2, 2, 2, 2, 2, 2, 2, 2, 2, 2, 2, 2, 2, 2, 2, 2, 2, 2, 2, 2, 2, 2, 2, 2, 2, 2, 2, 2, 2, 2, 2, 2, 2, 2, 2, 2, 2, 2, 2, 2, 2, 2, 2, 2, 2, 2, 2, 2, 2, 2, 2, 2, 2, 2, 2, 2, 2, 2, 2, 2, 2, 2, 2, 2, 2, 2, 2, 2, 2, 2, 2, 2, 2, 2, 2, 2, 2, 2, 2, 2, 2, 2, 2, 2, 2, 2, 2, 2, 2, 2, 2, 2, 2, 2, 2, 2, 2, 2, 2, 2, 2, 2, 2, 2, 2, 2, 2, 2, 2, 2, 2, 2, 2, 2, 2, 2, 2, 2, 2, 2, 2, 2, 2, 2, 2, 2, 2, 2, 2, 2, 2, 2, 2, 2, 2, 2, 2, 2, 2, 2, 2, 2, 2, 2, 2, 2, 2, 2, 2, 2, 2, 2, 2, 2, 2, 2, 2, 2, 2, 2, 2, 2, 2, 2, 2, 2, 2, 2, 2, 2, 2, 2, 2, 2, 2, 2, 2, 2, 2, 2, 2, 2, 2, 2, 2, 2, 2, 2, 2, 2, 2, 2, 2, 2, 2, 2, 2, 2, 2, 2, 2, 2, 2, 2, 2, 2, 2, 2, 2, 2, 2, 2, 2, 2, 2, 2, 2, 2, 2, 2, 2, 2, 2, 2, 2, 2, 2, 2, 2, 2, 2, 2, 2, 2, 2, 2, 2, 2, 2, 2, 2, 2, 2, 2, 2, 2, 2, 2, 2, 2, 2, 2, 2, 2, 2, 2, 2, 2, 2, 2, 2, 2, 2, 2, 2, 2, 2, 2, 2, 2, 2, 2, 2, 2, 2, 2, 2, 2, 2, 2, 2, 2, 2, 2, 2, 2, 2, 2, 2, 2, 2, 2, 2, 2, 2, 2, 2, 2, 2, 2, 2, 2, 2, 2, 2, 2, 2, 2, 2, 2, 2, 2, 2, 2, 2, 2, 2, 2, 2, 2, 2, 2, 2, 2, 2, 2, 2, 2, 2, 2, 2, 2, 2, 2, 2, 2, 2, 2, 2, 2, 2, 2, 2, 2, 2, 2, 2, 2, 2, 2, 2, 2, 2, 2, 2, 2, 2, 2, 2, 3 ),
 ( 0.000000000000000000, 0.001994670335415893447, 0.003989340670831786895, 0.005984011006247681209, 0.007978681341663573789, 0.009973351677079468972, 0.01196802201249536242, 0.01396269234791125587, 0.01595736268332714758, 0.01795203301874304103, 0.01994670335415893794, 0.02194137368957482792, 0.02393604402499072484, 0.02593071436040661482, 0.02792538469582251173, 0.02992005503123840171, 0.03191472536665429516, 0.03390939570207018861, 0.03590406603748608205, 0.03789873637290198244, 0.03989340670831787589, 0.04188807704373376239, 0.04388274737914965584, 0.04587741771456555623, 0.04787208804998144968, 0.04986675838539734312, 0.05186142872081322963, 0.05385609905622912308, 0.05585076939164502347, 0.05784543972706091691, 0.05984011006247680342, 0.06183478039789269687, 0.06382945073330859032, 0.06582412106872448376, 0.06781879140414037721, 0.06981346173955627066, 0.07180813207497216411, 0.07380280241038805755, 0.07579747274580396488, 0.07779214308121985832, 0.07978681341663575177, 0.08178148375205164522, 0.08377615408746752479, 0.08577082442288341824, 0.08776549475829931168, 0.08976016509371520513, 0.09175483542913111246, 0.09374950576454700590, 0.09574417609996289935, 0.09773884643537879280, 0.09973351677079468625, 0.1017281871062105658, 0.1037228574416264593, 0.1057175277770423527, 0.1077121981124582462, 0.1097068684478741535, 0.1117015387832900469, 0.1136962091187059404, 0.1156908794541218338, 0.1176855497895377273, 0.1196802201249536068, 0.1216748904603695003, 0.1236695607957853937, 0.1256642311312012872, 0.1276589014666171806, 0.1296535718020330741, 0.1316482421374489675, 0.1336429124728648887, 0.1356375828082807544, 0.1376322531436966756, 0.1396269234791125413, 0.1416215938145284625, 0.1436162641499443282, 0.1456109344853602494, 0.1476056048207761151, 0.1496002751561920086, 0.1515949454916079298, 0.1535896158270237954, 0.1555842861624397166, 0.1575789564978555823, 0.1595736268332715035, 0.1615682971686873692, 0.1635629675041032904, 0.1655576378395191561, 0.1675523081749350496, 0.1695469785103509708, 0.1715416488457668365, 0.1735363191811827577, 0.1755309895165986234, 0.1775256598520145446, 0.1795203301874304103, 0.1815150005228463315, 0.1835096708582622249, 0.1855043411936780906, 0.1874990115290940118, 0.1894936818645098775, 0.1914883521999257987, 0.1934830225353416644, 0.1954776928707575856, 0.1974723632061734513, 0.1994670335415893725, 0.2014617038770052659, 0.2034563742124211316, 0.2054510445478370528, 0.2074457148832529185, 0.2094403852186688397, 0.2114350555540847054, 0.2134297258895006266, 0.2154243962249164923, 0.2174190665603324135, 0.2194137368957483070, 0.2214084072311641727, 0.2234030775665800939, 0.2253977479019959596, 0.2273924182374118808, 0.2293870885728277464, 0.2313817589082436676, 0.2333764292436595611, 0.2353710995790754545, 0.2373657699144913480, 0.2393604402499072137, 0.2413551105853231349, 0.2433497809207390006, 0.2453444512561549218, 0.2473391215915707875, 0.2493337919269867087, 0.2513284622624025744, 0.2533231325978185233, 0.2553178029332343613, 0.2573124732686502547, 0.2593071436040661482, 0.2613018139394820971, 0.2632964842748979351, 0.2652911546103138285, 0.2672858249457297775, 0.2692804952811456709, 0.2712751656165615088, 0.2732698359519774023, 0.2752645062873933512, 0.2772591766228091892, 0.2792538469582250826, 0.2812485172936409761, 0.2832431876290569250, 0.2852378579644727630, 0.2872325282998886564, 0.2892271986353046054, 0.2912218689707204988, 0.2932165393061363368, 0.2952112096415522302, 0.2972058799769681792, 0.2992005503123840171, 0.3011952206477999106, 0.3031898909832158595, 0.3051845613186317530, 0.3071792316540475909, 0.3091739019894634843, 0.3111685723248794333, 0.3131632426602952712, 0.3151579129957111647, 0.3171525833311271136, 0.3191472536665430071, 0.3211419240019588450, 0.3231365943373747385, 0.3251312646727906874, 0.3271259350082065809, 0.3291206053436224188, 0.3311152756790383123, 0.3331099460144542612, 0.3351046163498700992, 0.3370992866852859926, 0.3390939570207019416, 0.3410886273561178350, 0.3430832976915336729, 0.3450779680269495664, 0.3470726383623655154, 0.3490673086977813533, 0.3510619790331972467, 0.3530566493686131957, 0.3550513197040290891, 0.3570459900394449271, 0.3590406603748608205, 0.3610353307102767695, 0.3630300010456926629, 0.3650246713811085009, 0.3670193417165244498, 0.3690140120519403433, 0.3710086823873561812, 0.3730033527227720747, 0.3749980230581880236, 0.3769926933936039171, 0.3789873637290197550, 0.3809820340644356484, 0.3829767043998515974, 0.3849713747352674353, 0.3869660450706833288, 0.3889607154060992777, 0.3909553857415151712, 0.3929500560769310091, 0.3949447264123469026, 0.3969393967477628515, 0.3989340670831787450, 0.4009287374185945829, 0.4029234077540105319, 0.4049180780894264253, 0.4069127484248422633, 0.4089074187602581567, 0.4109020890956741057, 0.4128967594310899991, 0.4148914297665058371, 0.4168861001019217860, 0.4188807704373376795, 0.4208754407727535174, 0.4228701111081694108, 0.4248647814435853598, 0.4268594517790012532, 0.4288541221144170912, 0.4308487924498329846, 0.4328434627852489336, 0.4348381331206648270, 0.4368328034560806650, 0.4388274737914966139, 0.4408221441269125074, 0.4428168144623283453, 0.4448114847977442388, 0.4468061551331601877, 0.4488008254685760812, 0.4507954958039919191, 0.4527901661394078681, 0.4547848364748237615, 0.4567795068102395994, 0.4587741771456554929, 0.4607688474810714419, 0.4627635178164873353, 0.4647581881519031732, 0.4667528584873191222, 0.4687475288227350156, 0.4707421991581509091, 0.4727368694935667470, 0.4747315398289826960, 0.4767262101643985894, 0.4787208804998144274, 0.4807155508352303208, 0.4827102211706462698, 0.4847048915060621632, 0.4866995618414780012, 0.4886942321768939501, 0.4906889025123098436, 0.4926835728477256815, 0.4946782431831415749, 0.4966729135185575239, 0.4986675838539734174, 0.5006622541893892553, 0.5026569245248051487, 0.5046515948602210422, 0.5066462651956370467, 0.5086409355310528291, 0.5106356058664687225, 0.5126302762018846160, 0.5146249465373005094, 0.5166196168727164029, 0.5186142872081322963, 0.5206089575435483008, 0.5226036278789641942, 0.5245982982143800877, 0.5265929685497958701, 0.5285876388852117636, 0.5305823092206276570, 0.5325769795560435504, 0.5345716498914595549, 0.5365663202268754484, 0.5385609905622913418, 0.5405556608977071242, 0.5425503312331230177, 0.5445450015685389111, 0.5465396719039548046, 0.5485343422393708090, 0.5505290125747867025, 0.5525236829102025959, 0.5545183532456183784, 0.5565130235810342718, 0.5585076939164501653, 0.5605023642518660587, 0.5624970345872819522, 0.5644917049226979566, 0.5664863752581138501, 0.5684810455935296325, 0.5704757159289455259, 0.5724703862643614194, 0.5744650565997773128, 0.5764597269351932063, 0.5784543972706092108, 0.5804490676060251042, 0.5824437379414409977, 0.5844384082768567801, 0.5864330786122726735, 0.5884277489476885670, 0.5904224192831044604, 0.5924170896185204649, 0.5944117599539363583, 0.5964064302893522518, 0.5984011006247680342, 0.6003957709601839277, 0.6023904412955998211, 0.6043851116310157146, 0.6063797819664317190, 0.6083744523018476125, 0.6103691226372635059, 0.6123637929726792883, 0.6143584633080951818, 0.6163531336435110752, 0.6183478039789269687, 0.6203424743143429732, 0.6223371446497588666, 0.6243318149851747600, 0.6263264853205905425, 0.6283211556560064359, 0.6303158259914223294, 0.6323104963268382228, 0.6343051666622542273, 0.6362998369976701207, 0.6382945073330860142, 0.6402891776685017966, 0.6422838480039176901, 0.6442785183393335835, 0.6462731886747494769, 0.6482678590101653704, 0.6502625293455813749, 0.6522571996809972683, 0.6542518700164131618, 0.6562465403518289442, 0.6582412106872448376, 0.6602358810226607311, 0.6622305513580766245, 0.6642252216934926290, 0.6662198920289085224, 0.6682145623643244159, 0.6702092326997401983, 0.6722039030351560918, 0.6741985733705719852, 0.6761932437059878787, 0.6781879140414038831, 0.6801825843768197766, 0.6821772547122356700, 0.6841719250476514524, 0.6861665953830673459, 0.6881612657184832393, 0.6901559360538991328, 0.6921506063893151373, 0.6941452767247310307, 0.6961399470601469242, 0.6981346173955627066, 0.7001292877309786000, 0.7021239580663944935, 0.7041186284018103869, 0.7061132987372263914, 0.7081079690726422848, 0.7101026394080581783, 0.7120973097434739607, 0.7140919800788898542, 0.7160866504143057476, 0.7180813207497216411, 0.7200759910851376455, 0.7220706614205535390, 0.7240653317559694324, 0.7260600020913853259, 0.7280546724268011083, 0.7300493427622170017, 0.7320440130976328952, 0.7340386834330488997, 0.7360333537684647931, 0.7380280241038806865, 0.7400226944392965800, 0.7420173647747123624, 0.7440120351101282559, 0.7460067054455441493, 0.7480013757809600428, 0.7499960461163760472, 0.7519907164517919407, 0.7539853867872078341, 0.7559800571226236166, 0.7579747274580395100, 0.7599693977934554034, 0.7619640681288712969, 0.7639587384642873014, 0.7659534087997031948, 0.7679480791351190883, 0.7699427494705348707, 0.7719374198059507641, 0.7739320901413666576, 0.7759267604767825510, 0.7779214308121985555, 0.7799161011476144489, 0.7819107714830303424, 0.7839054418184462358, 0.7859001121538620183, 0.7878947824892779117, 0.7898894528246938052, 0.7918841231601098096, 0.7938787934955257031, 0.7958734638309415965, 0.7978681341663574900, 0.7998628045017732724, 0.8018574748371891658, 0.8038521451726050593, 0.8058468155080210638, 0.8078414858434369572, 0.8098361561788528507, 0.8118308265142687441, 0.8138254968496845265, 0.8158201671851004200, 0.8178148375205163134, 0.8198095078559323179, 0.8218041781913482113, 0.8237988485267641048, 0.8257935188621799982, 0.8277881891975957807, 0.8297828595330116741, 0.8317775298684275675, 0.8337722002038435720, 0.8357668705392594655, 0.8377615408746753589, 0.8397562112100912524, 0.8417508815455070348, 0.8437455518809229282, 0.8457402222163388217, 0.8477348925517547151, 0.8497295628871707196, 0.8517242332225866130, 0.8537189035580025065, 0.8557135738934183999, 0.8577082442288341824, 0.8597029145642500758, 0.8616975848996659693, 0.8636922552350819737, 0.8656869255704978672, 0.8676815959059137606, 0.8696762662413296541, 0.8716709365767454365, 0.8736656069121613299, 0.8756602772475772234, 0.8776549475829932279, 0.8796496179184091213, 0.8816442882538250148, 0.8836389585892409082, 0.8856336289246566906, 0.8876282992600725841, 0.8896229695954884775, 0.8916176399309044820, 0.8936123102663203754, 0.8956069806017362689, 0.8976016509371521623, 0.8995963212725679448, 0.9015909916079838382, 0.9035856619433997317, 0.9055803322788157361, 0.9075750026142316296, 0.9095696729496475230, 0.9115643432850634165, 0.9135590136204791989, 0.9155536839558950923, 0.9175483542913109858, 0.9195430246267269903, 0.9215376949621428837, 0.9235323652975587772, 0.9255270356329746706, 0.9275217059683905640, 0.9295163763038063465, 0.9315110466392222399, 0.9335057169746382444, 0.9355003873100541378, 0.9374950576454700313, 0.9394897279808859247, 0.9414843983163018182, 0.9434790686517176006, 0.9454737389871334940, 0.9474684093225493875, 0.9494630796579653920, 0.9514577499933812854, 0.9534524203287971789, 0.9554470906642130723, 0.9574417609996288547, 0.9594364313350447482, 0.9614311016704606416, 0.9634257720058766461, 0.9654204423412925395, 0.9674151126767084330, 0.9694097830121243264, 0.9714044533475401089, 0.9733991236829560023, 0.9753937940183718958, 0.9773884643537879002, 0.9793831346892037937, 0.9813778050246196871, 0.9833724753600355806, 0.9853671456954513630, 0.9873618160308672564, 0.9892257831175960137 ),
 .UNSPECIFIED. ) 
 CURVE ( )  GEOMETRIC_REPRESENTATION_ITEM ( )  RATIONAL_B_SPLINE_CURVE ( ( 1.000000000000000000, 0.9807852804032304306, 1.000000000000000000, 0.9807852804032304306, 1.000000000000000000, 0.9807852804032304306, 1.000000000000000000, 0.9807852804032304306, 1.000000000000000000, 0.9807852804032304306, 1.000000000000000000, 0.9807852804032304306, 1.000000000000000000, 0.9807852804032304306, 1.000000000000000000, 0.9807852804032304306, 1.000000000000000000, 0.9807852804032304306, 1.000000000000000000, 0.9807852804032304306, 1.000000000000000000, 0.9807852804032304306, 1.000000000000000000, 0.9807852804032304306, 1.000000000000000000, 0.9807852804032304306, 1.000000000000000000, 0.9807852804032304306, 1.000000000000000000, 0.9807852804032304306, 1.000000000000000000, 0.9807852804032304306, 1.000000000000000000, 0.9807852804032304306, 1.000000000000000000, 0.9807852804032304306, 1.000000000000000000, 0.9807852804032304306, 1.000000000000000000, 0.9807852804032304306, 1.000000000000000000, 0.9807852804032304306, 1.000000000000000000, 0.9807852804032304306, 1.000000000000000000, 0.9807852804032304306, 1.000000000000000000, 0.9807852804032304306, 1.000000000000000000, 0.9807852804032304306, 1.000000000000000000, 0.9807852804032304306, 1.000000000000000000, 0.9807852804032304306, 1.000000000000000000, 0.9807852804032304306, 1.000000000000000000, 0.9807852804032304306, 1.000000000000000000, 0.9807852804032304306, 1.000000000000000000, 0.9807852804032304306, 1.000000000000000000, 0.9807852804032304306, 1.000000000000000000, 0.9807852804032304306, 1.000000000000000000, 0.9807852804032304306, 1.000000000000000000, 0.9807852804032304306, 1.000000000000000000, 0.9807852804032304306, 1.000000000000000000, 0.9807852804032304306, 1.000000000000000000, 0.9807852804032304306, 1.000000000000000000, 0.9807852804032304306, 1.000000000000000000, 0.9807852804032304306, 1.000000000000000000, 0.9807852804032304306, 1.000000000000000000, 0.9807852804032304306, 1.000000000000000000, 0.9807852804032304306, 1.000000000000000000, 0.9807852804032304306, 1.000000000000000000, 0.9807852804032304306, 1.000000000000000000, 0.9807852804032304306, 1.000000000000000000, 0.9807852804032304306, 1.000000000000000000, 0.9807852804032304306, 1.000000000000000000, 0.9807852804032304306, 1.000000000000000000, 0.9807852804032304306, 1.000000000000000000, 0.9807852804032304306, 1.000000000000000000, 0.9807852804032304306, 1.000000000000000000, 0.9807852804032304306, 1.000000000000000000, 0.9807852804032304306, 1.000000000000000000, 0.9807852804032304306, 1.000000000000000000, 0.9807852804032304306, 1.000000000000000000, 0.9807852804032304306, 1.000000000000000000, 0.9807852804032304306, 1.000000000000000000, 0.9807852804032304306, 1.000000000000000000, 0.9807852804032304306, 1.000000000000000000, 0.9807852804032304306, 1.000000000000000000, 0.9807852804032304306, 1.000000000000000000, 0.9807852804032304306, 1.000000000000000000, 0.9807852804032304306, 1.000000000000000000, 0.9807852804032304306, 1.000000000000000000, 0.9807852804032304306, 1.000000000000000000, 0.9807852804032304306, 1.000000000000000000, 0.9807852804032304306, 1.000000000000000000, 0.9807852804032304306, 1.000000000000000000, 0.9807852804032304306, 1.000000000000000000, 0.9807852804032304306, 1.000000000000000000, 0.9807852804032304306, 1.000000000000000000, 0.9807852804032304306, 1.000000000000000000, 0.9807852804032304306, 1.000000000000000000, 0.9807852804032304306, 1.000000000000000000, 0.9807852804032304306, 1.000000000000000000, 0.9807852804032304306, 1.000000000000000000, 0.9807852804032304306, 1.000000000000000000, 0.9807852804032304306, 1.000000000000000000, 0.9807852804032304306, 1.000000000000000000, 0.9807852804032304306, 1.000000000000000000, 0.9807852804032304306, 1.000000000000000000, 0.9807852804032304306, 1.000000000000000000, 0.9807852804032304306, 1.000000000000000000, 0.9807852804032304306, 1.000000000000000000, 0.9807852804032304306, 1.000000000000000000, 0.9807852804032304306, 1.000000000000000000, 0.9807852804032304306, 1.000000000000000000, 0.9807852804032304306, 1.000000000000000000, 0.9807852804032304306, 1.000000000000000000, 0.9807852804032304306, 1.000000000000000000, 0.9807852804032304306, 1.000000000000000000, 0.9807852804032304306, 1.000000000000000000, 0.9807852804032304306, 1.000000000000000000, 0.9807852804032304306, 1.000000000000000000, 0.9807852804032304306, 1.000000000000000000, 0.9807852804032304306, 1.000000000000000000, 0.9807852804032304306, 1.000000000000000000, 0.9807852804032304306, 1.000000000000000000, 0.9807852804032304306, 1.000000000000000000, 0.9807852804032304306, 1.000000000000000000, 0.9807852804032304306, 1.000000000000000000, 0.9807852804032304306, 1.000000000000000000, 0.9807852804032304306, 1.000000000000000000, 0.9807852804032304306, 1.000000000000000000, 0.9807852804032304306, 1.000000000000000000, 0.9807852804032304306, 1.000000000000000000, 0.9807852804032304306, 1.000000000000000000, 0.9807852804032304306, 1.000000000000000000, 0.9807852804032304306, 1.000000000000000000, 0.9807852804032304306, 1.000000000000000000, 0.9807852804032304306, 1.000000000000000000, 0.9807852804032304306, 1.000000000000000000, 0.9807852804032304306, 1.000000000000000000, 0.9807852804032304306, 1.000000000000000000, 0.9807852804032304306, 1.000000000000000000, 0.9807852804032304306, 1.000000000000000000, 0.9807852804032304306, 1.000000000000000000, 0.9807852804032304306, 1.000000000000000000, 0.9807852804032304306, 1.000000000000000000, 0.9807852804032304306, 1.000000000000000000, 0.9807852804032304306, 1.000000000000000000, 0.9807852804032304306, 1.000000000000000000, 0.9807852804032304306, 1.000000000000000000, 0.9807852804032304306, 1.000000000000000000, 0.9807852804032304306, 1.000000000000000000, 0.9807852804032304306, 1.000000000000000000, 0.9807852804032304306, 1.000000000000000000, 0.9807852804032304306, 1.000000000000000000, 0.9807852804032304306, 1.000000000000000000, 0.9807852804032304306, 1.000000000000000000, 0.9807852804032304306, 1.000000000000000000, 0.9807852804032304306, 1.000000000000000000, 0.9807852804032304306, 1.000000000000000000, 0.9807852804032304306, 1.000000000000000000, 0.9807852804032304306, 1.000000000000000000, 0.9807852804032304306, 1.000000000000000000, 0.9807852804032304306, 1.000000000000000000, 0.9807852804032304306, 1.000000000000000000, 0.9807852804032304306, 1.000000000000000000, 0.9807852804032304306, 1.000000000000000000, 0.9807852804032304306, 1.000000000000000000, 0.9807852804032304306, 1.000000000000000000, 0.9807852804032304306, 1.000000000000000000, 0.9807852804032304306, 1.000000000000000000, 0.9807852804032304306, 1.000000000000000000, 0.9807852804032304306, 1.000000000000000000, 0.9807852804032304306, 1.000000000000000000, 0.9807852804032304306, 1.000000000000000000, 0.9807852804032304306, 1.000000000000000000, 0.9807852804032304306, 1.000000000000000000, 0.9807852804032304306, 1.000000000000000000, 0.9807852804032304306, 1.000000000000000000, 0.9807852804032304306, 1.000000000000000000, 0.9807852804032304306, 1.000000000000000000, 0.9807852804032304306, 1.000000000000000000, 0.9807852804032304306, 1.000000000000000000, 0.9807852804032304306, 1.000000000000000000, 0.9807852804032304306, 1.000000000000000000, 0.9807852804032304306, 1.000000000000000000, 0.9807852804032304306, 1.000000000000000000, 0.9807852804032304306, 1.000000000000000000, 0.9807852804032304306, 1.000000000000000000, 0.9807852804032304306, 1.000000000000000000, 0.9807852804032304306, 1.000000000000000000, 0.9807852804032304306, 1.000000000000000000, 0.9807852804032304306, 1.000000000000000000, 0.9807852804032304306, 1.000000000000000000, 0.9807852804032304306, 1.000000000000000000, 0.9807852804032304306, 1.000000000000000000, 0.9807852804032304306, 1.000000000000000000, 0.9807852804032304306, 1.000000000000000000, 0.9807852804032304306, 1.000000000000000000, 0.9807852804032304306, 1.000000000000000000, 0.9807852804032304306, 1.000000000000000000, 0.9807852804032304306, 1.000000000000000000, 0.9807852804032304306, 1.000000000000000000, 0.9807852804032304306, 1.000000000000000000, 0.9807852804032304306, 1.000000000000000000, 0.9807852804032304306, 1.000000000000000000, 0.9807852804032304306, 1.000000000000000000, 0.9807852804032304306, 1.000000000000000000, 0.9807852804032304306, 1.000000000000000000, 0.9807852804032304306, 1.000000000000000000, 0.9807852804032304306, 1.000000000000000000, 0.9807852804032304306, 1.000000000000000000, 0.9807852804032304306, 1.000000000000000000, 0.9807852804032304306, 1.000000000000000000, 0.9807852804032304306, 1.000000000000000000, 0.9807852804032304306, 1.000000000000000000, 0.9807852804032304306, 1.000000000000000000, 0.9807852804032304306, 1.000000000000000000, 0.9807852804032304306, 1.000000000000000000, 0.9807852804032304306, 1.000000000000000000, 0.9807852804032304306, 1.000000000000000000, 0.9807852804032304306, 1.000000000000000000, 0.9807852804032304306, 1.000000000000000000, 0.9807852804032304306, 1.000000000000000000, 0.9807852804032304306, 1.000000000000000000, 0.9807852804032304306, 1.000000000000000000, 0.9807852804032304306, 1.000000000000000000, 0.9807852804032304306, 1.000000000000000000, 0.9807852804032304306, 1.000000000000000000, 0.9807852804032304306, 1.000000000000000000, 0.9807852804032304306, 1.000000000000000000, 0.9807852804032304306, 1.000000000000000000, 0.9807852804032304306, 1.000000000000000000, 0.9807852804032304306, 1.000000000000000000, 0.9807852804032304306, 1.000000000000000000, 0.9807852804032304306, 1.000000000000000000, 0.9807852804032304306, 1.000000000000000000, 0.9807852804032304306, 1.000000000000000000, 0.9807852804032304306, 1.000000000000000000, 0.9807852804032304306, 1.000000000000000000, 0.9807852804032304306, 1.000000000000000000, 0.9807852804032304306, 1.000000000000000000, 0.9807852804032304306, 1.000000000000000000, 0.9807852804032304306, 1.000000000000000000, 0.9807852804032304306, 1.000000000000000000, 0.9807852804032304306, 1.000000000000000000, 0.9807852804032304306, 1.000000000000000000, 0.9807852804032304306, 1.000000000000000000, 0.9807852804032304306, 1.000000000000000000, 0.9807852804032304306, 1.000000000000000000, 0.9807852804032304306, 1.000000000000000000, 0.9807852804032304306, 1.000000000000000000, 0.9807852804032304306, 1.000000000000000000, 0.9807852804032304306, 1.000000000000000000, 0.9807852804032304306, 1.000000000000000000, 0.9807852804032304306, 1.000000000000000000, 0.9807852804032304306, 1.000000000000000000, 0.9807852804032304306, 1.000000000000000000, 0.9807852804032304306, 1.000000000000000000, 0.9807852804032304306, 1.000000000000000000, 0.9807852804032304306, 1.000000000000000000, 0.9807852804032304306, 1.000000000000000000, 0.9807852804032304306, 1.000000000000000000, 0.9807852804032304306, 1.000000000000000000, 0.9807852804032304306, 1.000000000000000000, 0.9807852804032304306, 1.000000000000000000, 0.9807852804032304306, 1.000000000000000000, 0.9807852804032304306, 1.000000000000000000, 0.9807852804032304306, 1.000000000000000000, 0.9807852804032304306, 1.000000000000000000, 0.9807852804032304306, 1.000000000000000000, 0.9807852804032304306, 1.000000000000000000, 0.9807852804032304306, 1.000000000000000000, 0.9807852804032304306, 1.000000000000000000, 0.9807852804032304306, 1.000000000000000000, 0.9807852804032304306, 1.000000000000000000, 0.9807852804032304306, 1.000000000000000000, 0.9807852804032304306, 1.000000000000000000, 0.9807852804032304306, 1.000000000000000000, 0.9807852804032304306, 1.000000000000000000, 0.9807852804032304306, 1.000000000000000000, 0.9807852804032304306, 1.000000000000000000, 0.9807852804032304306, 1.000000000000000000, 0.9807852804032304306, 1.000000000000000000, 0.9807852804032304306, 1.000000000000000000, 0.9807852804032304306, 1.000000000000000000, 0.9807852804032304306, 1.000000000000000000, 0.9807852804032304306, 1.000000000000000000, 0.9807852804032304306, 1.000000000000000000, 0.9807852804032304306, 1.000000000000000000, 0.9807852804032304306, 1.000000000000000000, 0.9807852804032304306, 1.000000000000000000, 0.9807852804032304306, 1.000000000000000000, 0.9807852804032304306, 1.000000000000000000, 0.9807852804032304306, 1.000000000000000000, 0.9807852804032304306, 1.000000000000000000, 0.9807852804032304306, 1.000000000000000000, 0.9807852804032304306, 1.000000000000000000, 0.9807852804032304306, 1.000000000000000000, 0.9807852804032304306, 1.000000000000000000, 0.9807852804032304306, 1.000000000000000000, 0.9807852804032304306, 1.000000000000000000, 0.9807852804032304306, 1.000000000000000000, 0.9807852804032304306, 1.000000000000000000, 0.9807852804032304306, 1.000000000000000000, 0.9807852804032304306, 1.000000000000000000, 0.9807852804032304306, 1.000000000000000000, 0.9807852804032304306, 1.000000000000000000, 0.9807852804032304306, 1.000000000000000000, 0.9807852804032304306, 1.000000000000000000, 0.9807852804032304306, 1.000000000000000000, 0.9807852804032304306, 1.000000000000000000, 0.9807852804032304306, 1.000000000000000000, 0.9807852804032304306, 1.000000000000000000, 0.9807852804032304306, 1.000000000000000000, 0.9807852804032304306, 1.000000000000000000, 0.9807852804032304306, 1.000000000000000000, 0.9807852804032304306, 1.000000000000000000, 0.9807852804032304306, 1.000000000000000000, 0.9807852804032304306, 1.000000000000000000, 0.9807852804032304306, 1.000000000000000000, 0.9807852804032304306, 1.000000000000000000, 0.9807852804032304306, 1.000000000000000000, 0.9807852804032304306, 1.000000000000000000, 0.9807852804032304306, 1.000000000000000000, 0.9807852804032304306, 1.000000000000000000, 0.9807852804032304306, 1.000000000000000000, 0.9807852804032304306, 1.000000000000000000, 0.9807852804032304306, 1.000000000000000000, 0.9807852804032304306, 1.000000000000000000, 0.9807852804032304306, 1.000000000000000000, 0.9807852804032304306, 1.000000000000000000, 0.9807852804032304306, 1.000000000000000000, 0.9807852804032304306, 1.000000000000000000, 0.9807852804032304306, 1.000000000000000000, 0.9807852804032304306, 1.000000000000000000, 0.9807852804032304306, 1.000000000000000000, 0.9807852804032304306, 1.000000000000000000, 0.9807852804032304306, 1.000000000000000000, 0.9807852804032304306, 1.000000000000000000, 0.9807852804032304306, 1.000000000000000000, 0.9807852804032304306, 1.000000000000000000, 0.9807852804032304306, 1.000000000000000000, 0.9807852804032304306, 1.000000000000000000, 0.9807852804032304306, 1.000000000000000000, 0.9807852804032304306, 1.000000000000000000, 0.9807852804032304306, 1.000000000000000000, 0.9807852804032304306, 1.000000000000000000, 0.9807852804032304306, 1.000000000000000000, 0.9807852804032304306, 1.000000000000000000, 0.9807852804032304306, 1.000000000000000000, 0.9807852804032304306, 1.000000000000000000, 0.9807852804032304306, 1.000000000000000000, 0.9807852804032304306, 1.000000000000000000, 0.9807852804032304306, 1.000000000000000000, 0.9807852804032304306, 1.000000000000000000, 0.9807852804032304306, 1.000000000000000000, 0.9807852804032304306, 1.000000000000000000, 0.9807852804032304306, 1.000000000000000000, 0.9807852804032304306, 1.000000000000000000, 0.9807852804032304306, 1.000000000000000000, 0.9807852804032304306, 1.000000000000000000, 0.9807852804032304306, 1.000000000000000000, 0.9807852804032304306, 1.000000000000000000, 0.9807852804032304306, 1.000000000000000000, 0.9807852804032304306, 1.000000000000000000, 0.9807852804032304306, 1.000000000000000000, 0.9807852804032304306, 1.000000000000000000, 0.9807852804032304306, 1.000000000000000000, 0.9807852804032304306, 1.000000000000000000, 0.9807852804032304306, 1.000000000000000000, 0.9807852804032304306, 1.000000000000000000, 0.9807852804032304306, 1.000000000000000000, 0.9807852804032304306, 1.000000000000000000, 0.9807852804032304306, 1.000000000000000000, 0.9807852804032304306, 1.000000000000000000, 0.9807852804032304306, 1.000000000000000000, 0.9807852804032304306, 1.000000000000000000, 0.9807852804032304306, 1.000000000000000000, 0.9807852804032304306, 1.000000000000000000, 0.9807852804032304306, 1.000000000000000000, 0.9807852804032304306, 1.000000000000000000, 0.9807852804032304306, 1.000000000000000000, 0.9807852804032304306, 1.000000000000000000, 0.9807852804032304306, 1.000000000000000000, 0.9807852804032304306, 1.000000000000000000, 0.9807852804032304306, 1.000000000000000000, 0.9807852804032304306, 1.000000000000000000, 0.9807852804032304306, 1.000000000000000000, 0.9807852804032304306, 1.000000000000000000, 0.9807852804032304306, 1.000000000000000000, 0.9807852804032304306, 1.000000000000000000, 0.9807852804032304306, 1.000000000000000000, 0.9807852804032304306, 1.000000000000000000, 0.9807852804032304306, 1.000000000000000000, 0.9807852804032304306, 1.000000000000000000, 0.9807852804032304306, 1.000000000000000000, 0.9807852804032304306, 1.000000000000000000, 0.9807852804032304306, 1.000000000000000000, 0.9807852804032304306, 1.000000000000000000, 0.9807852804032304306, 1.000000000000000000, 0.9807852804032304306, 1.000000000000000000, 0.9807852804032304306, 1.000000000000000000, 0.9807852804032304306, 1.000000000000000000, 0.9807852804032304306, 1.000000000000000000, 0.9807852804032304306, 1.000000000000000000, 0.9807852804032304306, 1.000000000000000000, 0.9807852804032304306, 1.000000000000000000, 0.9807852804032304306, 1.000000000000000000, 0.9807852804032304306, 1.000000000000000000, 0.9807852804032304306, 1.000000000000000000, 0.9807852804032304306, 1.000000000000000000, 0.9807852804032304306, 1.000000000000000000, 0.9807852804032304306, 1.000000000000000000, 0.9807852804032304306, 1.000000000000000000, 0.9807852804032304306, 1.000000000000000000, 0.9807852804032304306, 1.000000000000000000, 0.9807852804032304306, 1.000000000000000000, 0.9807852804032304306, 1.000000000000000000, 0.9807852804032304306, 1.000000000000000000, 0.9807852804032304306, 1.000000000000000000, 0.9807852804032304306, 1.000000000000000000, 0.9807852804032304306, 1.000000000000000000, 0.9807852804032304306, 1.000000000000000000, 0.9807852804032304306, 1.000000000000000000, 0.9807852804032304306, 1.000000000000000000, 0.9807852804032304306, 1.000000000000000000, 0.9807852804032304306, 1.000000000000000000, 0.9807852804032304306, 1.000000000000000000, 0.9807852804032304306, 1.000000000000000000, 0.9807852804032304306, 1.000000000000000000, 0.9807852804032304306, 1.000000000000000000, 0.9807852804032304306, 1.000000000000000000, 0.9807852804032304306, 1.000000000000000000, 0.9807852804032304306, 1.000000000000000000, 0.9807852804032304306, 1.000000000000000000, 0.9807852804032304306, 1.000000000000000000, 0.9807852804032304306, 1.000000000000000000, 0.9807852804032304306, 1.000000000000000000, 0.9807852804032304306, 1.000000000000000000, 0.9807852804032304306, 1.000000000000000000, 0.9807852804032304306, 1.000000000000000000, 0.9807852804032304306, 1.000000000000000000, 0.9807852804032304306, 1.000000000000000000, 0.9807852804032304306, 1.000000000000000000, 0.9807852804032304306, 1.000000000000000000, 0.9807852804032304306, 1.000000000000000000, 0.9807852804032304306, 1.000000000000000000, 0.9807852804032304306, 1.000000000000000000, 0.9807852804032304306, 1.000000000000000000, 0.9807852804032304306, 1.000000000000000000, 0.9807852804032304306, 1.000000000000000000, 0.9807852804032304306, 1.000000000000000000, 0.9807852804032304306, 1.000000000000000000, 0.9807852804032304306, 1.000000000000000000, 0.9807852804032304306, 1.000000000000000000, 0.9807852804032304306, 1.000000000000000000, 0.9807852804032304306, 1.000000000000000000, 0.9807852804032304306, 1.000000000000000000, 0.9807852804032304306, 1.000000000000000000, 0.9807852804032304306, 1.000000000000000000, 0.9807852804032304306, 1.000000000000000000, 0.9807852804032304306, 1.000000000000000000, 0.9807852804032304306, 1.000000000000000000, 0.9807852804032304306, 1.000000000000000000, 0.9807852804032304306, 1.000000000000000000, 0.9807852804032304306, 1.000000000000000000, 0.9807852804032304306, 1.000000000000000000, 0.9807852804032304306, 1.000000000000000000, 0.9807852804032304306, 1.000000000000000000, 0.9807852804032304306, 1.000000000000000000, 0.9807852804032304306, 1.000000000000000000, 0.9807852804032304306, 1.000000000000000000, 0.9807852804032304306, 1.000000000000000000, 0.9807852804032304306, 1.000000000000000000, 0.9807852804032304306, 1.000000000000000000, 0.9807852804032304306, 1.000000000000000000, 0.9807852804032304306, 1.000000000000000000, 0.9807852804032304306, 1.000000000000000000, 0.9807852804032304306, 1.000000000000000000, 0.9807852804032304306, 1.000000000000000000, 0.9807852804032304306, 1.000000000000000000, 0.9807852804032304306, 1.000000000000000000, 0.9807852804032304306, 1.000000000000000000, 0.9807852804032304306, 1.000000000000000000, 0.9807852804032304306, 1.000000000000000000, 0.9807852804032304306, 1.000000000000000000, 0.9807852804032304306, 1.000000000000000000, 0.9807852804032304306, 1.000000000000000000, 0.9807852804032304306, 1.000000000000000000, 0.9807852804032304306, 1.000000000000000000, 0.9807852804032304306, 1.000000000000000000, 0.9807852804032304306, 1.000000000000000000, 0.9807852804032304306, 1.000000000000000000, 0.9807852804032304306, 1.000000000000000000, 0.9807852804032304306, 1.000000000000000000, 0.9807852804032304306, 1.000000000000000000, 0.9807852804032304306, 1.000000000000000000, 0.9807852804032304306, 1.000000000000000000, 0.9807852804032304306, 1.000000000000000000, 0.9807852804032304306, 1.000000000000000000, 0.9807852804032304306, 1.000000000000000000, 0.9807852804032304306, 1.000000000000000000, 0.9807852804032304306, 1.000000000000000000, 0.9807852804032304306, 1.000000000000000000, 0.9807852804032304306, 1.000000000000000000, 0.9807852804032304306, 1.000000000000000000, 0.9807852804032304306, 1.000000000000000000, 0.9807852804032304306, 1.000000000000000000, 0.9807852804032304306, 1.000000000000000000, 0.9807852804032304306, 1.000000000000000000, 0.9807852804032304306, 1.000000000000000000, 0.9807852804032304306, 1.000000000000000000, 0.9807852804032304306, 1.000000000000000000, 0.9807852804032304306, 1.000000000000000000, 0.9807852804032304306, 1.000000000000000000, 0.9807852804032304306, 1.000000000000000000, 0.9807852804032304306, 1.000000000000000000, 0.9807852804032304306, 1.000000000000000000, 0.9807852804032304306, 1.000000000000000000, 0.9807852804032304306, 1.000000000000000000, 0.9820443487461643084, 0.9976468673449425673 ) ) 
 REPRESENTATION_ITEM ( '' )  );
#12233=CARTESIAN_POINT ( 'NONE',  ( -40.53162694259544452, 396.6198905683720568, 11.84573899990672885 ) ) ;
#12234=CARTESIAN_POINT ( 'NONE',  ( -8.685887942688735208, 482.2448905601784759, -2.449293598294705724E-15 ) ) ;
#12235=DIRECTION ( 'NONE',  ( 1.191790137725560488E-16, -1.000000000000000000, 0.000000000000000000 ) ) ;
#12237=CARTESIAN_POINT ( 'NONE',  ( -16.84014894278198327, 311.6198905683720000, -11.84573899990672707 ) ) ;
#12238=CARTESIAN_POINT ( 'NONE',  ( -35.09675569278796559, 465.7448905683720568, 15.47720386886985366 ) ) ;
#12240=CARTESIAN_POINT ( 'NONE',  ( -11.73070664223726212, 463.1823905601784759, -11.32908994701042715 ) ) ;
#12241=CARTESIAN_POINT ( 'NONE',  ( -19.19641293061497578, 287.3073905683720000, 14.20200298773971426 ) ) ;
#12244=CARTESIAN_POINT ( 'NONE',  ( -11.93348319268872970, 440.0573905683720000, 3.332260488124728859 ) ) ;
#12247=CARTESIAN_POINT ( 'NONE',  ( -35.09675569278794427, 305.7448905683720568, 15.47720386886985366 ) ) ;
#12248=CARTESIAN_POINT ( 'NONE',  ( -42.88789093042843348, 376.3073905683720000, 9.489475012073734561 ) ) ;
#12249=CARTESIAN_POINT ( 'NONE',  ( -14.54375231895777176, 373.4948905601784759, -14.14213562373094746 ) ) ;
#12250=CARTESIAN_POINT ( 'NONE',  ( -48.68588794268872988, 531.6823905765655809, -3.978247347593158345 ) ) ;
#12251=CARTESIAN_POINT ( 'NONE',  ( -38.17536295476245556, 395.4323905683720000, 14.20200298773971781 ) ) ;
#12252=CARTESIAN_POINT ( 'NONE',  ( -40.53162694259542320, 234.1198905683720000, -11.84573899990672707 ) ) ;
#12253=CARTESIAN_POINT ( 'NONE',  ( -14.48388495494900852, 429.8073905683720000, -9.489475012073734561 ) ) ;
#12254=CARTESIAN_POINT ( 'NONE',  ( -24.70764059509556176, 349.1823905765655809, -19.99999999999999289 ) ) ;
#12256=CARTESIAN_POINT ( 'NONE',  ( -11.93348319268871371, 298.5573905683720000, 3.332260488124728859 ) ) ;
#12257=CARTESIAN_POINT ( 'NONE',  ( -22.27502019258949773, 482.2448905683720568, -15.47720386886985544 ) ) ;
#12258=CARTESIAN_POINT ( 'NONE',  ( -8.685887942689062058, 516.6823905765653535, 3.978247347593932837 ) ) ;
#12260=CARTESIAN_POINT ( 'NONE',  ( -24.70764059509555111, 304.4323905601784759, -19.99999999999999289 ) ) ;
#12261=ADVANCED_FACE ( 'NONE', ( #5855 ), #12617, .T. ) ;
#12262=CARTESIAN_POINT ( 'NONE',  ( -40.53162694259544452, 396.6198905683720568, 11.84573899990672885 ) ) ;
#12264=CARTESIAN_POINT ( 'NONE',  ( -8.685887942688744090, 532.5573905601784190, -3.978247347593165895 ) ) ;
#12265=CARTESIAN_POINT ( 'NONE',  ( -38.17536295476244845, 345.4323905683719431, 14.20200298773971781 ) ) ;
#12267=CARTESIAN_POINT ( 'NONE',  ( -44.16309181155858710, 503.2448905683719431, -6.410867750099231266 ) ) ;
#12268=ORIENTED_EDGE ( 'NONE', *, *, #12310, .T. ) ;
#12269=CARTESIAN_POINT ( 'NONE',  ( -28.68588794268871567, 354.7448905601784759, -19.99999999999999289 ) ) ;
#12270=CARTESIAN_POINT ( 'NONE',  ( -48.68588794268870856, 381.9948905765655809, 0.000000000000000000 ) ) ;
#12275=CARTESIAN_POINT ( 'NONE',  ( -21.03221929538694468, 518.8698905765655809, -18.47759065022572855 ) ) ;
#12276=CARTESIAN_POINT ( 'NONE',  ( -16.84014894278199748, 457.6198905683720568, 11.84573899990672530 ) ) ;
#12278=CARTESIAN_POINT ( 'NONE',  ( -25.35362745456399480, 486.6823905683721136, 16.75240474999998952 ) ) ;
#12280=CARTESIAN_POINT ( 'NONE',  ( -24.70764059509556532, 399.1823905765656377, -19.99999999999999289 ) ) ;
#12281=CARTESIAN_POINT ( 'NONE',  ( -10.20829729246299955, 476.3698905765656377, 7.653668647301790529 ) ) ;
#12282=CYLINDRICAL_SURFACE ( 'NONE', #21313, 19.99999999999999645 ) ;
#12283=CARTESIAN_POINT ( 'NONE',  ( -8.685887942688605534, 482.5573905601784190, -3.978247347592846594 ) ) ;
#12287=CYLINDRICAL_SURFACE ( 'NONE', #5212, 15.00000000000000000 ) ;
#12288=CARTESIAN_POINT ( 'NONE',  ( -35.09675569278794427, 287.2448905683720000, 15.47720386886985366 ) ) ;
#12289=CARTESIAN_POINT ( 'NONE',  ( -47.16347859291445133, 402.6198905765655809, 7.653668647301805628 ) ) ;
#12290=CARTESIAN_POINT ( 'NONE',  ( -11.93348319268872970, 440.3698905683720000, -2.051577885510841163E-15 ) ) ;
#12292=CARTESIAN_POINT ( 'NONE',  ( -22.27502019258946575, 278.4948905683720000, 15.47720386886985189 ) ) ;
#12294=CYLINDRICAL_SURFACE ( 'NONE', #20860, 19.99999999999999645 ) ;
#12296=CARTESIAN_POINT ( 'NONE',  ( -19.19641293061499354, 488.8073905683720000, 14.20200298773971426 ) ) ;
#12297=VERTEX_POINT ( 'NONE', #12847 ) ;
#12298=CARTESIAN_POINT ( 'NONE',  ( -32.66413529028186957, 365.0573905601784190, -19.99999999999999289 ) ) ;
#12299=CARTESIAN_POINT ( 'NONE',  ( -35.09675569278793716, 245.7448905683720000, 15.47720386886985366 ) ) ;
#12302=CARTESIAN_POINT ( 'NONE',  ( -36.33955658999052929, 453.8698905765656377, 18.47759065022572500 ) ) ;
#12304=CARTESIAN_POINT ( 'NONE',  ( -48.68588794268872277, 457.2448905601784759, 0.000000000000000000 ) ) ;
#12305=CARTESIAN_POINT ( 'NONE',  ( -45.43829269268869808, 225.0573905683720284, -3.332260488124726638 ) ) ;
#12306=CARTESIAN_POINT ( 'NONE',  ( -40.53162694259545873, 526.6198905683720568, 11.84573899990672885 ) ) ;
#12308=CARTESIAN_POINT ( 'NONE',  ( -16.84014894278197616, 240.1198905683720284, -11.84573899990672707 ) ) ;
#12309=CARTESIAN_POINT ( 'NONE',  ( -11.93348319268871904, 330.6823905683721136, -3.332260488124732856 ) ) ;
#12310=EDGE_CURVE ( 'NONE', #13961, #15268, #7347, .T. ) ;
#12312=CARTESIAN_POINT ( 'NONE',  ( -10.20829729246298534, 361.6198905601784759, 7.653668647301790529 ) ) ;
#12313=VECTOR ( 'NONE', #18292, 1000.000000000000000 ) ;
#12314=CARTESIAN_POINT ( 'NONE',  ( -44.16309181155857999, 393.2448905683720568, -6.410867750099231266 ) ) ;
#12317=CARTESIAN_POINT ( 'NONE',  ( -24.70764059509556532, 384.4323905601784190, -19.99999999999999289 ) ) ;
#12321=ORIENTED_EDGE ( 'NONE', *, *, #8792, .T. ) ;
#12322=CARTESIAN_POINT ( 'NONE',  ( -16.84014894278200813, 511.6198905683720000, -11.84573899990672707 ) ) ;
#12325=CARTESIAN_POINT ( 'NONE',  ( -19.19641293061497578, 311.9323905683720000, -14.20200298773971603 ) ) ;
#12327=CARTESIAN_POINT ( 'NONE',  ( -11.93348319268871904, 338.8698905683720000, -2.051577885510841163E-15 ) ) ;
#12328=CARTESIAN_POINT ( 'NONE',  ( -45.43829269268871229, 343.5573905683720000, -3.332260488124726638 ) ) ;
#12330=CARTESIAN_POINT ( 'NONE',  ( -8.685887942688713892, 277.3073905765655809, -3.978247347593165895 ) ) ;
#12332=CARTESIAN_POINT ( 'NONE',  ( -42.88789093042841927, 252.9323905683720284, -9.489475012073734561 ) ) ;
#12333=CARTESIAN_POINT ( 'NONE',  ( -42.82802356641967378, 463.2448905765656377, 14.14213562373094923 ) ) ;
#12334=CARTESIAN_POINT ( 'NONE',  ( -44.16309181155857289, 405.9948905683720568, 6.410867750099241924 ) ) ;
#12335=EDGE_CURVE ( 'NONE', #2640, #13932, #9015, .T. ) ;
#12338=CARTESIAN_POINT ( 'NONE',  ( -40.01497788969913927, 355.6823905601784759, -16.95518130045146421 ) ) ;
#12340=CARTESIAN_POINT ( 'NONE',  ( -10.20829729246300310, 507.6198905765656377, -7.653668647301794969 ) ) ;
#12341=CARTESIAN_POINT ( 'NONE',  ( -32.01814843081346140, 471.6823905683720568, -16.75240474999999307 ) ) ;
#12342=ORIENTED_EDGE ( 'NONE', *, *, #6364, .F. ) ;
#12343=CARTESIAN_POINT ( 'NONE',  ( -47.16347859291445133, 446.6198905601784759, -7.653668647301793193 ) ) ;
#12349=CARTESIAN_POINT ( 'NONE',  ( -22.27502019258946930, 296.9948905683720000, 15.47720386886985189 ) ) ;
#12352=CARTESIAN_POINT ( 'NONE',  ( -11.93348319268872082, 360.3698905683720568, -2.051577885510841163E-15 ) ) ;
#12353=CARTESIAN_POINT ( 'NONE',  ( -42.82802356641965247, 295.9948905601784759, -14.14213562373094746 ) ) ;
#12354=CARTESIAN_POINT ( 'NONE',  ( -40.01497788969915348, 513.5573905765656946, 16.95518130045146776 ) ) ;
#12355=CARTESIAN_POINT ( 'NONE',  ( -35.09675569278795138, 411.9948905683720000, -15.47720386886985544 ) ) ;
#12356=CARTESIAN_POINT ( 'NONE',  ( -35.09675569278793006, 233.4948905683720284, -15.47720386886985544 ) ) ;
#12357=CARTESIAN_POINT ( 'NONE',  ( -42.88789093042844058, 412.9323905683720000, -9.489475012073734561 ) ) ;
#12358=( BOUNDED_CURVE ( )  B_SPLINE_CURVE ( 2, ( #11192, #1159, #15975, #4390, #10974, #6210, #7730, #9668, #6418, #21148, #16294, #20938, #12720, #17583, #19207, #1467, #17688 ),
 .UNSPECIFIED., .F., .T. ) 
 B_SPLINE_CURVE_WITH_KNOTS ( ( 3, 2, 2, 2, 2, 2, 2, 2, 3 ),
 ( 0.4687500000000002220, 0.4707031250000002220, 0.4726562500000002220, 0.4746093750000002220, 0.4765625000000002220, 0.4785156250000002220, 0.4804687500000002220, 0.4824218750000002220, 0.4843750000000002220 ),
 .UNSPECIFIED. ) 
 CURVE ( )  GEOMETRIC_REPRESENTATION_ITEM ( )  RATIONAL_B_SPLINE_CURVE ( ( 0.9999999999999977796, 0.9807852804032326510, 1.000000000000000000, 0.9807852804032304306, 1.000000000000000000, 0.9807852804032304306, 1.000000000000000000, 0.9807852804032304306, 1.000000000000000000, 0.9807852804032304306, 1.000000000000000000, 0.9807852804032304306, 1.000000000000000000, 0.9807852804032304306, 1.000000000000000000, 0.9807852804032282101, 1.000000000000002220 ) ) 
 REPRESENTATION_ITEM ( '' )  );
#12359=CARTESIAN_POINT ( 'NONE',  ( -8.685887942688719221, 346.6823905765656377, 3.978247347593161010 ) ) ;
#12361=CARTESIAN_POINT ( 'NONE',  ( -22.27502019258946930, 296.9948905683720000, 15.47720386886985189 ) ) ;
#12362=CARTESIAN_POINT ( 'NONE',  ( -11.93348319268873325, 460.6823905683720568, -3.332260488124732856 ) ) ;
#12363=EDGE_CURVE ( 'NONE', #313, #11378, #21385, .T. ) ;
#12364=DIRECTION ( 'NONE',  ( -1.000000000000000000, 0.000000000000000000, 0.000000000000000000 ) ) ;
#12366=DIRECTION ( 'NONE',  ( -1.191790137725560488E-16, 1.000000000000000000, -0.000000000000000000 ) ) ;
#12367=CARTESIAN_POINT ( 'NONE',  ( -45.43829269268870519, 375.0573905683720000, -3.332260488124726194 ) ) ;
#12369=CARTESIAN_POINT ( 'NONE',  ( -24.70764059509556887, 510.0573905601785327, 19.99999999999998934 ) ) ;
#12370=CARTESIAN_POINT ( 'NONE',  ( -14.48388495494899608, 337.9323905683720568, 9.489475012073732785 ) ) ;
#12371=VERTEX_POINT ( 'NONE', #16526 ) ;
#12372=CARTESIAN_POINT ( 'NONE',  ( -38.17536295476247687, 512.3073905683719431, -14.20200298773971426 ) ) ;
#12374=CARTESIAN_POINT ( 'NONE',  ( -44.08364905673433043, 223.9102039777116602, -6.632192423093624889 ) ) ;
#12376=CARTESIAN_POINT ( 'NONE',  ( -8.685887942688713892, 286.9948905765656377, -2.449293598294705724E-15 ) ) ;
#12377=CARTESIAN_POINT ( 'NONE',  ( -48.68588794268872988, 521.9948905765656946, 0.000000000000000000 ) ) ;
#12378=CARTESIAN_POINT ( 'NONE',  ( -22.27502019258949773, 470.7448905683720568, -15.47720386886985544 ) ) ;
#12379=ORIENTED_EDGE ( 'NONE', *, *, #12393, .T. ) ;
#12380=CARTESIAN_POINT ( 'NONE',  ( -35.09675569278795848, 471.9948905683720000, -15.47720386886985544 ) ) ;
#12381=CARTESIAN_POINT ( 'NONE',  ( -17.35679799567827786, 250.6823905601785043, 16.95518130045146421 ) ) ;
#12382=CARTESIAN_POINT ( 'NONE',  ( -42.82802356641966668, 403.2448905765655809, 14.14213562373094923 ) ) ;
#12384=CARTESIAN_POINT ( 'NONE',  ( -17.35679799567828141, 300.6823905601784759, 16.95518130045146421 ) ) ;
#12385=DIRECTION ( 'NONE',  ( -1.191790137725560488E-16, 1.000000000000000000, -0.000000000000000000 ) ) ;
#12386=DIRECTION ( 'NONE',  ( -1.191790137725560488E-16, 1.000000000000000000, -0.000000000000000000 ) ) ;
#12388=CARTESIAN_POINT ( 'NONE',  ( -40.01497788969911795, 238.8073905601784759, 16.95518130045146776 ) ) ;
#12391=CARTESIAN_POINT ( 'NONE',  ( -11.93348319268871016, 280.3698905683720000, -2.051577885510841163E-15 ) ) ;
#12393=EDGE_CURVE ( 'NONE', #9678, #20528, #1293, .T. ) ;
#12394=CARTESIAN_POINT ( 'NONE',  ( -36.33955658999049376, 255.3698905601785043, -18.47759065022572855 ) ) ;
#12396=CARTESIAN_POINT ( 'NONE',  ( -25.35362745456398770, 428.1823905683720000, 16.75240474999998952 ) ) ;
#12397=CARTESIAN_POINT ( 'NONE',  ( -17.35679799567829207, 328.5573905765656377, -16.95518130045146421 ) ) ;
#12398=CARTESIAN_POINT ( 'NONE',  ( -13.20868407381884957, 270.9948905683720000, -6.410867750099233042 ) ) ;
#12403=CARTESIAN_POINT ( 'NONE',  ( -35.09675569278796559, 487.2448905683720000, 15.47720386886985366 ) ) ;
#12406=CARTESIAN_POINT ( 'NONE',  ( -42.88789093042841927, 234.8073905683720284, 9.489475012073736337 ) ) ;
#12410=CARTESIAN_POINT ( 'NONE',  ( -36.33955658999052218, 470.1198905765656377, -18.47759065022572855 ) ) ;
#12413=CARTESIAN_POINT ( 'NONE',  ( -36.33955658999052218, 455.3698905601784759, -18.47759065022572855 ) ) ;
#12414=CARTESIAN_POINT ( 'NONE',  ( -38.17536295476243424, 226.9323905683720000, 14.20200298773971781 ) ) ;
#12415=CARTESIAN_POINT ( 'NONE',  ( -44.16309181155859420, 524.7448905683720568, -6.410867750099231266 ) ) ;
#12418=CARTESIAN_POINT ( 'NONE',  ( -22.27502019258947286, 240.7448905683720000, -15.47720386886985544 ) ) ;
#12419=CARTESIAN_POINT ( 'NONE',  ( -42.88789093042843348, 336.3073905683720568, 9.489475012073736337 ) ) ;
#12420=CARTESIAN_POINT ( 'NONE',  ( -42.82802356641967378, 468.4948905601785327, 14.14213562373094923 ) ) ;
#12421=CARTESIAN_POINT ( 'NONE',  ( -28.68588794268871212, 359.7448905601784759, 19.99999999999999289 ) ) ;
#12423=CARTESIAN_POINT ( 'NONE',  ( -35.09675569278795138, 385.7448905683720000, 15.47720386886985366 ) ) ;
#12425=CARTESIAN_POINT ( 'NONE',  ( -8.685887942688724550, 382.2448905601784759, -2.449293598294705724E-15 ) ) ;
#12426=VECTOR ( 'NONE', #8365, 1000.000000000000000 ) ;
#12428=CARTESIAN_POINT ( 'NONE',  ( -48.68588794268858067, 406.9323905601785327, -3.978247347593477201 ) ) ;
#12429=ORIENTED_EDGE ( 'NONE', *, *, #7481, .T. ) ;
#12431=CARTESIAN_POINT ( 'NONE',  ( -16.84014894278200813, 501.6198905683720000, -11.84573899990672707 ) ) ;
#12432=CARTESIAN_POINT ( 'NONE',  ( -28.68588794268874054, 573.2448905601785327, 0.000000000000000000 ) ) ;
#12434=CARTESIAN_POINT ( 'NONE',  ( -38.17536295476244135, 296.9323905683720000, 14.20200298773971781 ) ) ;
#12436=CARTESIAN_POINT ( 'NONE',  ( -13.20868407381885845, 339.4948905683720568, -6.410867750099233042 ) ) ;
#12437=CARTESIAN_POINT ( 'NONE',  ( -22.27502019258947286, 336.9948905683720000, 15.47720386886985189 ) ) ;
#12438=CARTESIAN_POINT ( 'NONE',  ( -48.68588794268870146, 281.9948905765656377, 0.000000000000000000 ) ) ;
#12439=CARTESIAN_POINT ( 'NONE',  ( -28.68588794268871922, 394.7448905601784759, -19.99999999999999289 ) ) ;
#12440=CARTESIAN_POINT ( 'NONE',  ( -16.84014894278197616, 250.1198905683720284, -11.84573899990672707 ) ) ;
#12441=DIRECTION ( 'NONE',  ( -1.191790137725560488E-16, 1.000000000000000000, -0.000000000000000000 ) ) ;
#12442=CARTESIAN_POINT ( 'NONE',  ( -16.84014894278199037, 389.1198905683720568, 11.84573899990672530 ) ) ;
#12443=CARTESIAN_POINT ( 'NONE',  ( -8.685887942688719221, 332.2448905601784759, -2.449293598294705724E-15 ) ) ;
#12445=CLOSED_SHELL ( 'NONE', ( #9805, #12549, #9483, #19623, #787, #10980, #1369, #20963, #18337, #9873, #2888, #2174, #701, #11465, #11452, #4014, #11112, #20791, #4988, #437, #316, #19924, #7975, #16891, #11273, #10078, #16197, #6526, #7541, #3486, #3547, #6617, #11026, #11397, #21189, #5793, #20199, #15343, #15715, #11059, #15405, #16633, #7757, #11914, #17026, #15059, #13333, #13418, #12087, #13190, #14189, #11777, #10668, #4380, #12976, #3293, #3760, #17294, #19076, #19982, #12149, #12215, #2349, #13536, #19105, #919, #7617, #19155, #17850, #8883, #2956, #3979, #7767, #12261, #2618, #1058, #19340, #384, #8936 ) ) ;
#12447=CARTESIAN_POINT ( 'NONE',  ( -35.09675569278795848, 445.7448905683720000, 15.47720386886985366 ) ) ;
#12449=CARTESIAN_POINT ( 'NONE',  ( -14.54375231895778064, 453.4948905601784759, -14.14213562373094746 ) ) ;
#12453=ORIENTED_EDGE ( 'NONE', *, *, #20470, .F. ) ;
#12455=CARTESIAN_POINT ( 'NONE',  ( -47.16347859291443712, 326.6198905601784759, -7.653668647301793193 ) ) ;
#12456=CARTESIAN_POINT ( 'NONE',  ( -44.16309181155856578, 303.2448905683720000, -6.410867750099231266 ) ) ;
#12458=CARTESIAN_POINT ( 'NONE',  ( -11.93348319268872260, 360.6823905683720568, -3.332260488124732856 ) ) ;
#12460=CARTESIAN_POINT ( 'NONE',  ( -8.685887942688713892, 292.2448905601784759, -2.449293598294705724E-15 ) ) ;
#12462=CARTESIAN_POINT ( 'NONE',  ( -45.64106924314020119, 522.9323905765656946, 11.32908994701042715 ) ) ;
#12463=CARTESIAN_POINT ( 'NONE',  ( -38.17536295476246266, 402.3073905683720000, -14.20200298773971426 ) ) ;
#12464=CARTESIAN_POINT ( 'NONE',  ( -13.20868407381884779, 240.9948905683720284, -6.410867750099233042 ) ) ;
#12466=CARTESIAN_POINT ( 'NONE',  ( -25.35362745456399480, 401.0573905683720568, -16.75240474999999307 ) ) ;
#12468=CARTESIAN_POINT ( 'NONE',  ( -21.03221929538691981, 338.8698905765656377, -18.47759065022572855 ) ) ;
#12470=CARTESIAN_POINT ( 'NONE',  ( -35.09675569278794427, 315.7448905683720000, 15.47720386886985366 ) ) ;
#12472=CARTESIAN_POINT ( 'NONE',  ( -45.43829269268872650, 455.3698905683720000, 0.000000000000000000 ) ) ;
#12474=CARTESIAN_POINT ( 'NONE',  ( -48.68588794268887909, 457.5573905601783622, 3.978247347592742678 ) ) ;
#12475=CYLINDRICAL_SURFACE ( 'NONE', #2125, 19.99999999999999645 ) ;
#12479=CARTESIAN_POINT ( 'NONE',  ( -42.88789093042843348, 374.4323905683720000, -9.489475012073736337 ) ) ;
#12481=CARTESIAN_POINT ( 'NONE',  ( -19.19641293061499709, 497.3073905683720568, 14.20200298773971426 ) ) ;
#12482=CARTESIAN_POINT ( 'NONE',  ( -14.54375231895778420, 500.9948905601784190, 14.14213562373094568 ) ) ;
#12483=CARTESIAN_POINT ( 'NONE',  ( -13.20868407381885845, 349.4948905683720000, -6.410867750099233042 ) ) ;
#12485=CARTESIAN_POINT ( 'NONE',  ( -11.93348319268873858, 499.1823905683720568, -3.332260488124732856 ) ) ;
#12486=ORIENTED_EDGE ( 'NONE', *, *, #13664, .T. ) ;
#12488=( BOUNDED_CURVE ( )  B_SPLINE_CURVE ( 2, ( #8665, #9855, #16483, #3490, #11813, #15289, #3596, #10179, #474, #1989, #14967, #6936, #1665, #7040, #5107, #15078, #263 ),
 .UNSPECIFIED., .F., .T. ) 
 B_SPLINE_CURVE_WITH_KNOTS ( ( 3, 2, 2, 2, 2, 2, 2, 2, 3 ),
 ( 0.5781250000000001110, 0.5800781250000001110, 0.5820312500000001110, 0.5839843750000001110, 0.5859375000000002220, 0.5878906250000002220, 0.5898437500000002220, 0.5917968750000002220, 0.5937500000000002220 ),
 .UNSPECIFIED. ) 
 CURVE ( )  GEOMETRIC_REPRESENTATION_ITEM ( )  RATIONAL_B_SPLINE_CURVE ( ( 0.9999999999999988898, 0.9807852804032315408, 1.000000000000000000, 0.9807852804032304306, 1.000000000000000000, 0.9807852804032304306, 1.000000000000000000, 0.9807852804032304306, 1.000000000000000000, 0.9807852804032304306, 1.000000000000000000, 0.9807852804032304306, 1.000000000000000000, 0.9807852804032304306, 1.000000000000000000, 0.9807852804032282101, 1.000000000000002220 ) ) 
 REPRESENTATION_ITEM ( '' )  );
#12489=CARTESIAN_POINT ( 'NONE',  ( -43.68588794268873698, 573.2448905601785327, 0.000000000000000000 ) ) ;
#12491=CARTESIAN_POINT ( 'NONE',  ( -38.17536295476246266, 433.8073905683721136, -14.20200298773971426 ) ) ;
#12494=CARTESIAN_POINT ( 'NONE',  ( -45.43829269268872650, 463.8698905683720000, 0.000000000000000000 ) ) ;
#12496=CARTESIAN_POINT ( 'NONE',  ( -42.88789093042844769, 474.8073905683720000, 9.489475012073734561 ) ) ;
#12497=DIRECTION ( 'NONE',  ( -1.191790137725560488E-16, 1.000000000000000000, -0.000000000000000000 ) ) ;
#12498=CARTESIAN_POINT ( 'NONE',  ( -36.33955658999051508, 400.1198905765656377, -18.47759065022572855 ) ) ;
#12500=DIRECTION ( 'NONE',  ( -1.000000000000000000, 0.000000000000000000, 0.000000000000000000 ) ) ;
#12506=CARTESIAN_POINT ( 'NONE',  ( -44.16309181155856578, 274.7448905683720568, -6.410867750099231266 ) ) ;
#12507=CARTESIAN_POINT ( 'NONE',  ( -14.54375231895775222, 250.9948905601784759, 14.14213562373094568 ) ) ;
#12509=CARTESIAN_POINT ( 'NONE',  ( -32.01814843081345430, 423.1823905683720568, -16.75240474999999307 ) ) ;
#12511=CARTESIAN_POINT ( 'NONE',  ( -38.17536295476244135, 253.8073905683720568, -14.20200298773971426 ) ) ;
#12512=ORIENTED_EDGE ( 'NONE', *, *, #9621, .F. ) ;
#12515=CARTESIAN_POINT ( 'NONE',  ( -35.09675569278796559, 477.2448905683720568, 15.47720386886985366 ) ) ;
#12518=CARTESIAN_POINT ( 'NONE',  ( -45.64106924314017988, 366.3073905601785896, -11.32908994701042538 ) ) ;
#12519=CARTESIAN_POINT ( 'NONE',  ( -45.43829269268869098, 234.1823905683720284, 3.332260488124734632 ) ) ;
#12523=CARTESIAN_POINT ( 'NONE',  ( -32.66413529028189089, 459.8073905765656377, -19.99999999999999289 ) ) ;
#12524=CARTESIAN_POINT ( 'NONE',  ( -11.73070664223724613, 351.3073905601785327, 11.32908994701042005 ) ) ;
#12525=CARTESIAN_POINT ( 'NONE',  ( -47.16347859291443712, 282.6198905765656377, 7.653668647301805628 ) ) ;
#12526=CARTESIAN_POINT ( 'NONE',  ( -11.73070664223726034, 453.1823905601785327, -11.32908994701042538 ) ) ;
#12528=CARTESIAN_POINT ( 'NONE',  ( -40.53162694259545873, 524.1198905683720568, -11.84573899990672707 ) ) ;
#12529=CARTESIAN_POINT ( 'NONE',  ( -24.70764059509555111, 374.8073905765655809, 19.99999999999998934 ) ) ;
#12530=CARTESIAN_POINT ( 'NONE',  ( -38.17536295476244135, 252.3073905683720284, -14.20200298773971426 ) ) ;
#12532=CARTESIAN_POINT ( 'NONE',  ( -22.27502019258948351, 342.2448905683720568, -15.47720386886985544 ) ) ;
#12535=CARTESIAN_POINT ( 'NONE',  ( -40.01497788969912506, 273.5573905765656377, 16.95518130045146776 ) ) ;
#12538=CARTESIAN_POINT ( 'NONE',  ( -13.20868407381886200, 379.4948905683720000, -6.410867750099233042 ) ) ;
#12541=CARTESIAN_POINT ( 'NONE',  ( -40.01497788969913927, 385.6823905601784190, -16.95518130045146421 ) ) ;
#12543=CARTESIAN_POINT ( 'NONE',  ( -11.73070664223725501, 403.1823905601785896, -11.32908994701042538 ) ) ;
#12545=ORIENTED_EDGE ( 'NONE', *, *, #17936, .F. ) ;
#12546=CARTESIAN_POINT ( 'NONE',  ( -45.43829269268873361, 515.3698905683720568, 0.000000000000000000 ) ) ;
#12549=ADVANCED_FACE ( 'NONE', ( #5786 ), #12287, .T. ) ;
#12550=CARTESIAN_POINT ( 'NONE',  ( -32.01814843081344009, 297.5573905683720000, 16.75240474999999307 ) ) ;
#12552=CARTESIAN_POINT ( 'NONE',  ( -13.20868407381885312, 318.2448905683720000, 6.410867750099229490 ) ) ;
#12553=CARTESIAN_POINT ( 'NONE',  ( -19.19641293061498288, 350.4323905683720000, -14.20200298773971603 ) ) ;
#12554=AXIS2_PLACEMENT_3D ( 'NONE', #8235, #10284, #9968 ) ;
#12555=CARTESIAN_POINT ( 'NONE',  ( -32.66413529028186957, 274.1823905765656377, 19.99999999999999289 ) ) ;
#12556=CARTESIAN_POINT ( 'NONE',  ( -17.35679799567829917, 393.8073905601785327, -16.95518130045146421 ) ) ;
#12557=CARTESIAN_POINT ( 'NONE',  ( -32.01814843081343298, 246.0573905683720000, 16.75240474999999307 ) ) ;
#12558=CARTESIAN_POINT ( 'NONE',  ( -36.33955658999049376, 225.3698905601784759, -18.47759065022572855 ) ) ;
#12559=AXIS2_PLACEMENT_3D ( 'NONE', #9689, #3427, #19863 ) ;
#12560=CARTESIAN_POINT ( 'NONE',  ( -42.88789093042844058, 394.4323905683720000, -9.489475012073736337 ) ) ;
#12564=CARTESIAN_POINT ( 'NONE',  ( -32.01814843081345430, 441.6823905683721136, -16.75240474999999307 ) ) ;
#12566=CARTESIAN_POINT ( 'NONE',  ( -10.20829729246299600, 452.8698905601785327, -7.653668647301794969 ) ) ;
#12571=CARTESIAN_POINT ( 'NONE',  ( -8.685887942688717445, 332.5573905601784190, -3.978247347593165895 ) ) ;
#12573=CARTESIAN_POINT ( 'NONE',  ( -16.84014894278198682, 359.1198905683720568, 11.84573899990672530 ) ) ;
#12575=CARTESIAN_POINT ( 'NONE',  ( -48.68588794268872277, 502.3073905765656946, 3.978247347593168115 ) ) ;
#12576=CARTESIAN_POINT ( 'NONE',  ( -40.53162694259543741, 385.1198905683720568, 11.84573899990672885 ) ) ;
#12577=CARTESIAN_POINT ( 'NONE',  ( -22.27502019258946220, 238.4948905683720284, 15.47720386886985189 ) ) ;
#12578=CARTESIAN_POINT ( 'NONE',  ( -14.48388495494900674, 409.8073905683720568, -9.489475012073734561 ) ) ;
#12579=CARTESIAN_POINT ( 'NONE',  ( -17.35679799567829917, 348.5573905765655809, -16.95518130045146421 ) ) ;
#12580=CARTESIAN_POINT ( 'NONE',  ( -32.66413529028186247, 325.0573905601785327, -19.99999999999999289 ) ) ;
#12581=CARTESIAN_POINT ( 'NONE',  ( -14.48388495494899075, 307.9323905683719431, 9.489475012073731008 ) ) ;
#12582=CARTESIAN_POINT ( 'NONE',  ( -42.88789093042844769, 454.4323905683720568, -9.489475012073736337 ) ) ;
#12588=CARTESIAN_POINT ( 'NONE',  ( -13.20868407381886023, 360.9948905683720568, -6.410867750099233042 ) ) ;
#12589=CARTESIAN_POINT ( 'NONE',  ( -22.27502019258949417, 496.9948905683720568, 15.47720386886985189 ) ) ;
#12590=CARTESIAN_POINT ( 'NONE',  ( -42.82802356641967378, 498.4948905601784759, 14.14213562373094923 ) ) ;
#12591=CARTESIAN_POINT ( 'NONE',  ( -19.19641293061498288, 320.4323905683720568, -14.20200298773971603 ) ) ;
#12593=CARTESIAN_POINT ( 'NONE',  ( -14.48388495494901740, 499.8073905683720568, -9.489475012073736337 ) ) ;
#12594=EDGE_LOOP ( 'NONE', ( #18485, #18644, #16726, #20352 ) ) ;
#12596=CARTESIAN_POINT ( 'NONE',  ( -36.33955658999050797, 313.8698905765656377, 18.47759065022572500 ) ) ;
#12597=CARTESIAN_POINT ( 'NONE',  ( -32.01814843081344719, 433.1823905683720568, -16.75240474999999307 ) ) ;
#12598=CARTESIAN_POINT ( 'NONE',  ( -42.82802356641966668, 393.2448905765655809, 14.14213562373094923 ) ) ;
#12600=CARTESIAN_POINT ( 'NONE',  ( -35.09675569278795848, 461.9948905683720000, -15.47720386886985544 ) ) ;
#12602=CARTESIAN_POINT ( 'NONE',  ( -38.17536295476246266, 475.4323905683720000, 14.20200298773971781 ) ) ;
#12603=CARTESIAN_POINT ( 'NONE',  ( -8.685887942688884422, 246.6823905765655809, 3.978247347593586447 ) ) ;
#12604=CARTESIAN_POINT ( 'NONE',  ( -40.01497788969914637, 400.4323905765656377, -16.95518130045146421 ) ) ;
#12607=CARTESIAN_POINT ( 'NONE',  ( -48.68588794268870856, 387.2448905601784759, 0.000000000000000000 ) ) ;
#12611=CARTESIAN_POINT ( 'NONE',  ( -45.55770059569361763, 223.9102039777116886, 1.340232597368489209 ) ) ;
#12613=CARTESIAN_POINT ( 'NONE',  ( -48.68588794268869435, 257.5573905601784759, 3.978247347593168115 ) ) ;
#12614=CARTESIAN_POINT ( 'NONE',  ( -24.70764059509555821, 450.0573905601785327, 19.99999999999998934 ) ) ;
#12615=CARTESIAN_POINT ( 'NONE',  ( -38.17536295476245556, 426.9323905683720000, 14.20200298773971781 ) ) ;
#12616=FACE_OUTER_BOUND ( 'NONE', #20564, .T. ) ;
#12617=( BOUNDED_SURFACE ( )  B_SPLINE_SURFACE ( 1, 2, ( 
 ( #10827, #12250, #12027, #4126, #20360, #5743, #20680, #14099, #18726, #7150, #4018, #13771, #7469, #2515, #582, #5642, #18941, #12140, #15399, #904, #10714, #7366, #5535, #17332, #3806, #7578, #18833, #15720, #15828, #12462, #10397, #19060, #3914, #2621, #10611, #1012, #2198, #17437, #10504, #7257, #17125, #17016, #2304, #8887, #9202, #689, #15504, #17229, #8783, #14205, #800, #15613, #20794, #13882, #20473, #2412, #8992, #13993, #20575, #12354, #1219, #4450, #20897, #21215, #1426, #6277, #19375, #4347, #16247, #2839, #14630, #9733, #2943, #11036, #6380, #9628, #14732, #12989, #5961, #14422, #12676, #19582, #16355, #9421, #15928, #17647, #1532, #9522, #3154, #8102, #16140, #21105, #12891, #6171, #4560, #12575, #19270, #19169, #7998, #10930, #7892, #16041, #1117, #4762, #19481, #1321, #6065, #4661, #17540, #2731, #12781, #11252, #9311, #17851, #7688, #3045, #7789, #17954, #11147, #14318, #21003, #11357, #17752, #14520, #16459, #4873, #14842, #18, #13826, #9947, #6594, #14947, #13102, #10558, #10346, #3467, #5485, #1642, #13215, #638, #19800, #4980, #8325, #9836, #16567, #11579, #18170, #15454, #17074, #536, #13323, #19687, #10454, #3368, #8834, #3968, #18279, #1753, #7204, #3864, #8940, #20419, #21314, #133, #6706, #5593, #17181, #19906, #8214, #5087, #2360, #16969, #18784, #6485, #2149, #15355, #7102, #11688, #8730, #11467, #13723, #18065, #2256, #3260, #20313, #12083, #18676, #12196, #13942, #17391, #5803, #20629, #10664, #7744, #17282, #15775, #14264, #15882, #12410, #19002, #9047, #15670, #17490, #4188, #14373, #4511, #19222, #20954, #10774, #2573, #856, #2467, #6124, #964, #15563, #7640, #7420, #9264, #2788, #17597, #14046, #9153, #7528, #14154, #10987, #6021, #4078, #20741, #1070, #5913, #18892, #12523, #20530, #4406, #19117, #9375, #19324, #4300, #2679, #15992, #1172, #2899, #12733, #748, #20851, #12631, #11099, #17702, #7313, #5695, #12302, #13275, #6436, #6653, #19860, #19638, #3211, #9789, #9685, #8058, #5036, #1376, #11638, #13161, #1269, #11414, #6336, #4615, #7848, #14475, #11311, #21162, #14578, #11210, #1702, #17807, #16309, #8161, #16412, #12948, #19537, #2998, #9582, #4819, #4714, #8270, #18232, #19749, #14901, #17906, #3103, #16198, #7948, #86, #1481, #9479, #1590, #14689, #14794, #18122, #11531, #21266, #13049, #18017, #21375, #4932, #6544, #19430, #3317, #9897, #16519, #12841, #16090, #21058, #6227, #18340, #10319, #10004, #20391, #3633, #8705, #7178, #16942, #16627, #15329, #3527, #15428, #16839, #13801, #15010, #7074, #16737, #20080, #19969, #8384, #10115, #1924, #17050, #13486, #8491, #18448, #1817, #5567, #13596, #6974, #513, #5148, #15116, #3839, #298, #6867, #11851, #13380, #5252, #10216, #2027, #18648, #20288, #3733, #8594, #15217, #12172, #409, #8811, #20183, #5351, #10428, #11952, #13695, #2124, #18548, #5458, #12059, #2232, #614, #3424, #194, #6762, #11746, #17462, #1147, #9022, #15645, #8915, #19196, #5673, #2651, #14347, #7718, #20926, #831, #7397, #3947, #13914, #6093, #5886, #9239, #4375, #20825, #18759, #15536, #2441, #14023, #2335, #10532, #5995, #4052, #936, #17153, #7503, #20602, #10640, #12382, #10857, #10963, #719, #15856, #4272, #14126, #7289, #14237, #12604, #12498, #1042, #20503, #12280, #18862, #5777, #17571, #18975, #2763, #9342, #15960, #20712, #4156, #10748, #17364, #2545, #17258, #9127, #15749, #7607, #19089, #57, #11069, #12708, #9763, #8133, #14450, #17783, #11283, #17675, #16281, #21137, #1456, #4689, #12921, #7820, #19614, #16069, #19722, #17881, #6408, #2975, #16388, #3294, #6309, #21350, #11387, #6517, #19510, #3074, #9657, #9553, #12815, #6201, #4587, #11501, #2869, #9454, #1563, #4791, #8031, #19300, #17988, #13133, #16172, #7922, #4905, #14662, #14764, #3184, #19405, #1349, #14551, #21243, #18098, #13022, #9867, #1245, #16492, #1674, #8245, #14874, #4485, #21030, #11181, #14980, #5327, #2202, #17021, #8788, #10087, #3501, #13246, #1789, #10404, #15193, #11928, #7053, #8677, #6625, #18202, #11719, #16708, #11611, #19835, #15301, #13353, #10191, #5011, #16813, #18311, #19942, #274, #20160, #13672, #9979, #18521, #13570, #2002, #15406, #2099, #488, #378, #3707, #3398, #16600, #6737, #1897, #20261, #8465, #5431, #12032, #18624, #8570, #13457, #15089, #5226, #6842, #3812, #8356, #167, #10294, #5119, #20050, #11825, #18419, #16917, #3606, #6948, #5648, #20579, #5539, #4130, #8997, #10720, #13999, #805, #17130, #7473, #3918, #7582, #5749, #15724, #12254, #19064, #12579, #15617, #9210, #20686, #15832, #7371, #12359, #18948, #18837, #693, #15510, #13887, #20798, #12145, #18734, #4247, #14103, #17336, #587, #5861, #1018, #4024, #2521, #9103, #17546, #10617, #5966, #911, #20365, #2416, #17233, #12468, #2310, #14211, #8892, #10833, #17441, #2626, #19173, #4351, #7263, #20477, #10935, #2736, #9316, #7155, #13777, #10508, #4564, #17757, #1223, #2843, #14738, #16145, #15933, #8002, #9427, #9633, #3159, #17958, #7794, #11040, #7897, #17651, #11362, #6384, #4455, #9526, #1430, #16045, #19274, #4767, #14635, #11256, #14427, #21220, #1122, #11472, #1325, #12995, #19691, #19587, #7693, #9737, #21007, #6489, #14524, #4877, #6069, #16358, #6176, #11153, #12786, #20901, #19379, #2947, #8107, #21110, #6281, #12896, #14322, #18069, #4666, #19485, #1536, #17856, #3049, #21320, #16251, #13107, #3265, #12681, #5091, #8328, #3373, #3683, #5298, #10167, #1868, #8219, #20131, #6711, #18493, #13645, #6814, #14950, #10269, #13541, #18599, #16886, #9840, #18283, #16572, #2070, #20231, #13327, #19807, #137, #5402, #13429, #7024, #12007, #20022, #3578, #16785, #10057, #8438, #16464, #1757, #1647, #11900, #14847, #11794, #19910, #4984, #22, #8646, #6598, #3472, #11692, #15274, #13219, #16680, #11583, #15062, #18175, #5196, #9950, #244, #18389, #1973, #8543, #15164, #353, #6916, #457, #7556, #7447, #16996, #5722, #666, #20338, #2175, #8760, #5619, #15481, #8861, #5513, #17419, #12112, #3992, #2494, #4102, #7232, #13858, #18704, #3890, #20555, #20446, #2600, #14182, #14075, #9180, #12228, #18811, #10481, #17101, #15806, #10585, #3782, #17310, #2281, #18918, #12438, #5829, #17206, #2385, #8968, #15593, #20658, #15697, #13752, #778, #10690, #7339, #7126, #19036, #9076, #12330, #13973, #883, #10372, #20772, #4221, #10804, #5940, #993, #15380, #12555, #558, #9714, #11124, #8083, #9291, #1403, #11014, #14398, #14294, #2710, #12653, #19248, #11339, #7770, #4430, #12760, #10908, #14713, #7871, #1297, #3026, #20880, #17624, #19560, #2816, #9400, #6148, #7666, #20980, #16018, #1200, #12970, #14607, #19458, #17729, #17520, #7978, #19349, #6360, #1509, #16118, #4539, #4741, #21191, #6464, #17933, #15906, #1098, #17830, #6045, #19150, #2923, #4325, #16226, #3128, #9503, #14500, #21083, #6256, #12868, #4642, #11233, #9608, #16335, #21290, #16658, #9814, #3556, #6681, #3447, #19774, #220, #1949, #9924, #5173, #1843, #11770, #1728, #13301, #19886, #4960, #14819, #738, #13191, #10145, #18045, #3239, #6788, #8412, #5062, #13080, #13406, #16761, #11559, #11666, #18256, #6893, #3343, #8518, #10031, #16543, #18365, #15036, #19995, #15144, #6570, #8301, #14926, #18146, #326, #13514, #19666, #16437, #4844, #11443, #1617, #108, #8190, #1164, #11405, #19315, #9676, #6535, #21367, #13152, #14467, #7839, #17589, #6115, #14781, #19527, #16300, #18008, #13041, #10979, #7736, #16083, #21049, #15982, #2781, #19631, #17695, #14570, #9367, #21156, #1262, #2887, #4607, #3094, #3203, #14366, #1473, #17899, #6327, #19740, #6425, #4811, #4706, #8049, #20945, #12726, #11090, #6217, #9780, #12833, #16405, #1582, #8153, #12941, #17800, #19423, #9573, #11199, #4501, #2990, #9471, #16190, #14681, #1368 ),
 ( #7939, #11302, #21259, #16512, #9994, #8377, #9888, #4924, #6966, #11630, #8484, #11521, #15107, #16619, #18224, #19962, #18439, #11945, #8262, #3626, #11843, #291, #7068, #400, #13589, #20071, #10208, #18114, #3310, #5029, #1808, #20177, #15000, #3726, #5343, #18539, #6860, #11739, #187, #3519, #5140, #10311, #1692, #14891, #16831, #13266, #13686, #78, #6645, #2019, #16935, #19852, #6754, #10106, #3417, #13478, #13372, #5243, #18329, #16728, #1916, #8587, #15210, #2118, #8697, #15320, #505, #11163, #4674, #1131, #1333, #12796, #7906, #7703, #4466, #11049, #4358, #14221, #7591, #5977, #12905, #4256, #10843, #17766, #6185, #17661, #14111, #19388, #14534, #19181, #19283, #2853, #9643, #17555, #19496, #10945, #21119, #2958, #1441, #6291, #20696, #14331, #20808, #11266, #17865, #2744, #2635, #9325, #3058, #9435, #16263, #5869, #16054, #7803, #14435, #20911, #12690, #12481, #12589, #19073, #9535, #17448, #1231, #15945, #9220, #15839, #1026, #6077, #21016, #4573, #16155, #257, #3170, #8229, #6722, #8339, #19702, #13117, #1546, #8118, #3384, #4887, #6824, #18401, #11703, #13440, #18082, #9850, #14750, #16370, #20032, #14858, #8012, #149, #21333, #1770, #16691, #10068, #6500, #9749, #34, #11485, #3482, #19923, #17967, #1660, #14962, #3276, #11372, #18295, #13339, #9963, #16477, #5102, #14645, #3589, #6608, #1880, #11805, #8448, #21229, #15073, #13230, #5208, #19820, #10175, #19599, #16796, #4996, #11595, #18186, #13005, #16582, #6394, #4775, #12016, #16899, #17005, #15175, #12341, #12125, #5523, #7241, #3692, #15285, #2396, #2081, #7033, #10385, #11910, #18609, #468, #8660, #17215, #18821, #2291, #15388, #363, #12238, #20240, #10595, #5731, #20348, #1984, #2186, #13655, #15602, #18928, #5412, #18504, #3793, #4111, #18713, #20563, #10700, #3901, #17112, #8872, #8770, #568, #8555, #7136, #6929, #5628, #13553, #10490, #13762, #10280, #20142, #5309, #15490, #676, #13869, #20457, #788, #4003, #8978, #7349, #13980, #7565, #1001, #10813, #17427, #12665, #14191, #9510, #6264, #20991, #16127, #5948, #19159, #2608, #4230, #1309, #17528, #17319, #9410, #9191, #11023, #4547, #19359, #15816, #12447, #9301, #19046, #12769, #7777, #5841, #10917, #2825, #20782, #20667, #6156, #16026, #19257, #12564, #1207, #2502, #12880, #2720, #14409, #21091, #11135, #9086, #17738, #4336, #7881, #15915, #19467, #7456, #2930, #1106, #7677, #14303, #892, #20886, #6054, #14508, #4439, #17634, #4650, #15705, #14085, #7, #14828, #16553, #12978, #3139, #11675, #11346, #16343, #19675, #21203, #6473, #9721, #4750, #5073, #6692, #11567, #3247, #9617, #118, #8091, #19894, #15045, #8202, #1519, #18266, #14934, #20005, #3455, #19569, #4969, #10041, #13309, #17942, #6368, #9823, #14721, #16666, #1738, #21301, #4857, #18156, #13088, #14618, #1852, #3355, #6581, #11453, #9933, #17838, #6797, #18053, #8311, #228, #8421, #3034, #13414, #16447, #11240, #1628, #16236, #1412, #7987, #13202, #19786, #334, #10152, #20113, #5282, #18796, #15257, #11885, #20216, #18374, #15574, #15365, #8742, #10464, #6900, #3665, #5603, #10249, #16872, #13630, #15152, #439, #2056, #8629, #20430, #650, #5494, #18580, #3563, #15466, #7007, #13837, #8953, #2160, #5384, #12209, #8844, #13955, #3978, #11778, #11989, #3768, #10568, #760, #10355, #13523, #16980, #7325, #544, #2370, #16769, #7112, #20321, #12095, #13737, #18688, #1956, #3875, #8526, #7214, #17084, #2266, #17192, #15682, #12314, #18904, #978, #10786, #4203, #868, #12747, #7431, #20754, #19234, #20867, #17404, #2586, #14059, #20643, #15893, #9165, #19337, #9492, #2800, #4524, #15789, #7540, #5814, #12423, #11111, #5926, #20541, #12643, #19018, #14167, #4418, #6137, #2477, #11000, #6031, #9277, #1282, #16005, #1188, #14279, #17611, #4088, #5706, #12538, #19131, #7758, #4311, #17714, #14384, #20968, #2694, #10894, #17503, #1083, #7653, #2912, #10676, #17296, #9387, #16105, #7860, #9060, #14488, #11838, #10204, #16212, #19847, #13366, #19443, #18324, #1803, #3514, #6749, #14995, #9595, #286, #17819, #395, #19957, #8479, #5024, #18434, #5339, #8371, #2015, #13473, #8582, #181, #5134, #11733, #11624, #14594, #7964, #6640, #13584, #4628, #11222, #3619, #6854, #10101, #21069, #20065, #15205, #18219, #16722, #1911, #10305, #3410, #20173, #15101, #9989, #6961, #5238, #16826, #11939, #72, #16613, #18534, #3722, #16931, #2113, #6242, #3011, #12855, #1389, #13261, #20378, #5551, #20273, #9115, #17035, #7384, #4258, #19075, #10846, #12157, #18745, #15315, #3826, #12483, #17244, #14010, #15736, #10735, #8692, #5445, #13788, #3933, #13682, #501, #17349, #15416, #12265, #7063, #18849, #10519, #922, #13899, #2427, #17141, #5760, #20698, #2322, #2532, #20590, #7487, #8902, #20489, #5660, #15520, #8799, #2216, #600, #14113, #12045, #18635, #12370, #817, #4037, #10414, #18958, #5871, #705, #10627, #9009, #17450, #7276, #7165, #15632, #4141, #17867, #19390, #6293, #9537, #2746, #12692, #6079, #7706, #11268, #21018, #12799, #20810, #6396, #1335, #13007, #14334, #20913, #14223, #3060, #10947, #7908, #19601, #4777, #11374, #19285, #4470, #9222, #19184, #2637, #11166, #14536, #9645, #4676, #15842, #5981, #11051, #17663, #7593, #1028, #16265, #9327, #6187, #12591, #4575, #2855, #15948, #9438, #16157, #1444, #4361, #21122, #12908, #17768, #17557, #19498, #8015, #2960, #14648, #1133, #16056, #1233, #7805, #21231, #14437, #16799, #20035, #13443, #153, #3387, #8232, #16585, #11600, #5211, #8121, #9752, #16694, #4891, #5312, #16375, #17970, #15076, #11810, #19705, #1663, #1773, #1549, #6725, #4999, #13342, #9966, #18189, #13120, #3485, #21336, #14861, #3280, #8343, #10073, #3592, #6504, #1883, #8451, #19927, #20145, #18404, #10178, #11706, #260, #14753, #3173, #18086, #37, #1987, #6612, #8558, #15179, #366, #5105, #14965, #13233, #18298, #6828, #6932, #11488, #9853, #13557, #16480, #19824, #3695, #11913, #5631, #18824, #7036, #3796, #5526, #16902, #3904, #571, #18717, #13765, #7139, #471, #15493, #8663, #2399, #12128, #2294, #10388, #12241, #792, #15391, #4006, #7244, #10598, #20351, #10493, #17115, #17009, #20243, #5415, #12019, #8981, #2084, #15288, #17218, #679, #8875, #18507, #15605, #7352, #2189, #13872, #20461, #10283, #13983, #13658, #20566, #5734, #18612, #8773, #13518, #16764, #9927, #19890, #13305, #14931, #18474, #6791, #19998, #6574, #13625, #8521, #20213, #112, #6685, #1, #10244, #18149, #15147, #5378, #11984, #18578, #5066, #11670, #16441, #4963, #9817, #18369, #329, #16869, #11882, #1620, #13195, #18260, #3451, #14822, #8193, #3661, #16547, #13409, #19777, #5176, #11562, #10036, #8306, #3347, #2051, #5278, #10148, #1847, #1732, #20108, #16662, #8625, #8415, #11773, #15040, #15249, #435, #224, #7002, #3559, #1952, #6896, #17398, #7535, #644, #13728, #8840, #14162, #755, #971, #20747, #13948, #18898, #4084, #3974, #2367, #5921, #17079, #12530, #7426, #16974, #5702, #7210, #20318, #2155, #8736, #5599, #15461, #13832, #5490, #2582, #12090, #10564, #2473, #10671, #20426, #12203, #18682, #3870, #20535, #18790, #9160, #3764, #14053, #15784, #17187, #8946, #10459, #2262, #10351, #15569, #15360, #17288, #7320, #9055, #12418, #5810, #12308, #15677, #863, #20637, #19012, #4195, #10781, #541, #7108, #19229, #1076, #7956, #4621, #14483, #12637, #11216, #4307, #14695, #19331, #3005, #1489, #17815, #10890, #9590, #4412, #9694, #11105, #8065, #9272, #1384, #10995, #14379, #14273, #2687, #17604, #2795, #11319, #7750, #9381, #12739, #17497, #21272, #7854, #1276, #16206, #20857, #15999, #19543, #1180, #20961, #6132, #12954, #19125, #4517, #17709, #17914, #6443, #2904, #7647, #9487, #15888, #16097, #16315, #6027, #21063 ) ),
 .UNSPECIFIED., .F., .F., .T. ) 
 B_SPLINE_SURFACE_WITH_KNOTS ( ( 2, 2 ),
 ( 3, 2, 2, 2, 2, 2, 2, 2, 2, 2, 2, 2, 2, 2, 2, 2, 2, 2, 2, 2, 2, 2, 2, 2, 2, 2, 2, 2, 2, 2, 2, 2, 2, 2, 2, 2, 2, 2, 2, 2, 2, 2, 2, 2, 2, 2, 2, 2, 2, 2, 2, 2, 2, 2, 2, 2, 2, 2, 2, 2, 2, 2, 2, 2, 2, 2, 2, 2, 2, 2, 2, 2, 2, 2, 2, 2, 2, 2, 2, 2, 2, 2, 2, 2, 2, 2, 2, 2, 2, 2, 2, 2, 2, 2, 2, 2, 2, 2, 2, 2, 2, 2, 2, 2, 2, 2, 2, 2, 2, 2, 2, 2, 2, 2, 2, 2, 2, 2, 2, 2, 2, 2, 2, 2, 2, 2, 2, 2, 2, 2, 2, 2, 2, 2, 2, 2, 2, 2, 2, 2, 2, 2, 2, 2, 2, 2, 2, 2, 2, 2, 2, 2, 2, 2, 2, 2, 2, 2, 2, 2, 2, 2, 2, 2, 2, 2, 2, 2, 2, 2, 2, 2, 2, 2, 2, 2, 2, 2, 2, 2, 2, 2, 2, 2, 2, 2, 2, 2, 2, 2, 2, 2, 2, 2, 2, 2, 2, 2, 2, 2, 2, 2, 2, 2, 2, 2, 2, 2, 2, 2, 2, 2, 2, 2, 2, 2, 2, 2, 2, 2, 2, 2, 2, 2, 2, 2, 2, 2, 2, 2, 2, 2, 2, 2, 2, 2, 2, 2, 2, 2, 2, 2, 2, 2, 2, 2, 2, 2, 2, 2, 2, 2, 2, 2, 2, 2, 2, 2, 2, 2, 2, 2, 2, 2, 2, 2, 2, 2, 2, 2, 2, 2, 2, 2, 2, 2, 2, 2, 2, 2, 2, 2, 2, 2, 2, 2, 2, 2, 2, 2, 2, 2, 2, 2, 2, 2, 2, 2, 2, 2, 2, 2, 2, 2, 2, 2, 2, 2, 2, 2, 2, 2, 2, 2, 2, 2, 2, 2, 2, 2, 2, 2, 2, 2, 2, 2, 2, 2, 2, 2, 2, 2, 2, 2, 2, 2, 2, 2, 2, 2, 2, 2, 2, 2, 2, 2, 2, 2, 2, 2, 2, 2, 2, 2, 2, 2, 2, 2, 2, 2, 2, 2, 2, 2, 2, 2, 2, 2, 2, 2, 2, 2, 2, 2, 2, 2, 2, 2, 2, 2, 2, 2, 2, 2, 2, 2, 2, 2, 2, 2, 2, 2, 2, 2, 2, 2, 2, 2, 2, 2, 2, 2, 2, 2, 2, 2, 2, 2, 2, 2, 2, 2, 2, 2, 2, 2, 2, 2, 2, 2, 2, 2, 2, 2, 2, 2, 2, 2, 2, 2, 2, 2, 2, 2, 2, 2, 2, 2, 2, 2, 2, 2, 2, 2, 2, 2, 2, 2, 2, 2, 2, 2, 2, 2, 2, 2, 2, 2, 2, 2, 2, 2, 2, 2, 2, 2, 2, 2, 2, 2, 2, 2, 2, 2, 2, 2, 2, 2, 2, 2, 2, 2, 2, 2, 2, 2, 2, 2, 2, 2, 2, 2, 2, 2, 2, 2, 2, 2, 2, 2, 2, 2, 3 ),
 ( 0.000000000000000000, 1.000000000000000000 ),
 ( 0.000000000000000000, 0.001953125000000000000, 0.003906250000000000000, 0.005859375000000000000, 0.007812500000000000000, 0.009765625000000000000, 0.01171875000000000000, 0.01367187500000000000, 0.01562500000000000000, 0.01757812500000000000, 0.01953125000000000000, 0.02148437500000000000, 0.02343750000000000000, 0.02539062500000000000, 0.02734375000000000000, 0.02929687500000000000, 0.03125000000000000000, 0.03320312500000000000, 0.03515625000000000000, 0.03710937500000000000, 0.03906250000000000000, 0.04101562500000000000, 0.04296875000000000000, 0.04492187500000000000, 0.04687500000000000000, 0.04882812500000000000, 0.05078125000000000000, 0.05273437500000000000, 0.05468750000000000000, 0.05664062500000000000, 0.05859375000000000000, 0.06054687500000000000, 0.06250000000000000000, 0.06445312500000000000, 0.06640625000000000000, 0.06835937500000000000, 0.07031250000000000000, 0.07226562500000000000, 0.07421875000000000000, 0.07617187500000000000, 0.07812500000000000000, 0.08007812500000000000, 0.08203125000000000000, 0.08398437500000000000, 0.08593750000000000000, 0.08789062500000000000, 0.08984375000000000000, 0.09179687500000000000, 0.09375000000000000000, 0.09570312500000000000, 0.09765625000000000000, 0.09960937500000000000, 0.1015625000000000000, 0.1035156250000000000, 0.1054687500000000000, 0.1074218750000000000, 0.1093750000000000000, 0.1113281250000000000, 0.1132812500000000000, 0.1152343750000000000, 0.1171875000000000000, 0.1191406250000000000, 0.1210937500000000000, 0.1230468750000000000, 0.1250000000000000000, 0.1269531250000000000, 0.1289062500000000000, 0.1308593750000000000, 0.1328125000000000000, 0.1347656250000000000, 0.1367187500000000000, 0.1386718750000000000, 0.1406250000000000000, 0.1425781250000000000, 0.1445312500000000000, 0.1464843750000000000, 0.1484375000000000000, 0.1503906250000000000, 0.1523437500000000000, 0.1542968750000000000, 0.1562500000000000000, 0.1582031250000000000, 0.1601562500000000000, 0.1621093750000000000, 0.1640625000000000000, 0.1660156250000000000, 0.1679687500000000000, 0.1699218750000000000, 0.1718750000000000000, 0.1738281250000000000, 0.1757812500000000000, 0.1777343750000000000, 0.1796875000000000000, 0.1816406250000000000, 0.1835937500000000000, 0.1855468750000000000, 0.1875000000000000000, 0.1894531250000000000, 0.1914062500000000000, 0.1933593750000000000, 0.1953125000000000000, 0.1972656250000000000, 0.1992187500000000000, 0.2011718750000000000, 0.2031250000000000000, 0.2050781250000000000, 0.2070312500000000000, 0.2089843750000000000, 0.2109375000000000000, 0.2128906250000000000, 0.2148437500000000000, 0.2167968750000000000, 0.2187500000000000000, 0.2207031250000000000, 0.2226562500000000000, 0.2246093750000000000, 0.2265625000000000000, 0.2285156250000000000, 0.2304687500000000000, 0.2324218750000000000, 0.2343750000000000000, 0.2363281250000000000, 0.2382812500000000000, 0.2402343750000000000, 0.2421875000000000000, 0.2441406250000000000, 0.2460937500000000000, 0.2480468750000000000, 0.2500000000000000000, 0.2519531250000000000, 0.2539062500000000000, 0.2558593750000000000, 0.2578125000000000000, 0.2597656250000000000, 0.2617187500000000000, 0.2636718750000000000, 0.2656250000000000000, 0.2675781250000000000, 0.2695312500000000000, 0.2714843750000000000, 0.2734375000000000000, 0.2753906250000000000, 0.2773437500000000000, 0.2792968750000000000, 0.2812500000000000000, 0.2832031250000000000, 0.2851562500000000000, 0.2871093750000000000, 0.2890625000000000000, 0.2910156250000000000, 0.2929687500000000000, 0.2949218750000000000, 0.2968750000000000000, 0.2988281250000000000, 0.3007812500000000000, 0.3027343750000000000, 0.3046875000000000000, 0.3066406250000000000, 0.3085937500000000000, 0.3105468750000000000, 0.3125000000000000000, 0.3144531250000000000, 0.3164062500000000000, 0.3183593750000000000, 0.3203125000000000000, 0.3222656250000000000, 0.3242187500000000000, 0.3261718750000000000, 0.3281250000000000000, 0.3300781250000000000, 0.3320312500000000000, 0.3339843750000000000, 0.3359375000000000000, 0.3378906250000000000, 0.3398437500000000000, 0.3417968750000000000, 0.3437500000000000000, 0.3457031250000000000, 0.3476562500000000000, 0.3496093750000000000, 0.3515625000000000000, 0.3535156250000000000, 0.3554687500000000000, 0.3574218750000000000, 0.3593750000000000000, 0.3613281250000000000, 0.3632812500000000000, 0.3652343750000000000, 0.3671875000000000000, 0.3691406250000000000, 0.3710937500000000000, 0.3730468750000000000, 0.3750000000000000000, 0.3769531250000000000, 0.3789062500000000000, 0.3808593750000000000, 0.3828125000000000000, 0.3847656250000000000, 0.3867187500000000000, 0.3886718750000000000, 0.3906250000000000000, 0.3925781250000000000, 0.3945312500000000000, 0.3964843750000000000, 0.3984375000000000000, 0.4003906250000000000, 0.4023437500000000000, 0.4042968750000000000, 0.4062500000000000000, 0.4082031250000000000, 0.4101562500000000000, 0.4121093750000000000, 0.4140625000000000000, 0.4160156250000000000, 0.4179687500000000000, 0.4199218750000000000, 0.4218750000000000000, 0.4238281250000000000, 0.4257812500000000000, 0.4277343750000000000, 0.4296875000000000000, 0.4316406250000000000, 0.4335937500000000000, 0.4355468750000000000, 0.4375000000000000000, 0.4394531250000000000, 0.4414062500000000000, 0.4433593750000000000, 0.4453125000000000000, 0.4472656250000000000, 0.4492187500000000000, 0.4511718750000000000, 0.4531250000000000000, 0.4550781250000000000, 0.4570312500000000000, 0.4589843750000000000, 0.4609375000000000000, 0.4628906250000000000, 0.4648437500000000000, 0.4667968750000000000, 0.4687500000000000000, 0.4707031250000000000, 0.4726562500000000000, 0.4746093750000000000, 0.4765625000000000000, 0.4785156250000000000, 0.4804687500000000000, 0.4824218750000000000, 0.4843750000000000000, 0.4863281250000000000, 0.4882812500000000000, 0.4902343750000000000, 0.4921875000000000000, 0.4941406250000000000, 0.4960937500000000000, 0.4980468750000000000, 0.5000000000000000000, 0.5019531250000000000, 0.5039062500000000000, 0.5058593750000000000, 0.5078125000000000000, 0.5097656250000000000, 0.5117187500000000000, 0.5136718750000000000, 0.5156250000000000000, 0.5175781250000000000, 0.5195312500000000000, 0.5214843750000000000, 0.5234375000000000000, 0.5253906250000000000, 0.5273437500000000000, 0.5292968750000000000, 0.5312500000000000000, 0.5332031250000000000, 0.5351562500000000000, 0.5371093750000000000, 0.5390625000000000000, 0.5410156250000000000, 0.5429687500000000000, 0.5449218750000000000, 0.5468750000000000000, 0.5488281250000000000, 0.5507812500000000000, 0.5527343750000000000, 0.5546875000000000000, 0.5566406250000000000, 0.5585937500000000000, 0.5605468750000000000, 0.5625000000000000000, 0.5644531250000000000, 0.5664062500000000000, 0.5683593750000000000, 0.5703125000000000000, 0.5722656250000000000, 0.5742187500000000000, 0.5761718750000000000, 0.5781250000000000000, 0.5800781250000000000, 0.5820312500000000000, 0.5839843750000000000, 0.5859375000000000000, 0.5878906250000000000, 0.5898437500000000000, 0.5917968750000000000, 0.5937500000000000000, 0.5957031250000000000, 0.5976562500000000000, 0.5996093750000000000, 0.6015625000000000000, 0.6035156250000000000, 0.6054687500000000000, 0.6074218750000000000, 0.6093750000000000000, 0.6113281250000000000, 0.6132812500000000000, 0.6152343750000000000, 0.6171875000000000000, 0.6191406250000000000, 0.6210937500000000000, 0.6230468750000000000, 0.6250000000000000000, 0.6269531250000000000, 0.6289062500000000000, 0.6308593750000000000, 0.6328125000000000000, 0.6347656250000000000, 0.6367187500000000000, 0.6386718750000000000, 0.6406250000000000000, 0.6425781250000000000, 0.6445312500000000000, 0.6464843750000000000, 0.6484375000000000000, 0.6503906250000000000, 0.6523437500000000000, 0.6542968750000000000, 0.6562500000000000000, 0.6582031250000000000, 0.6601562500000000000, 0.6621093750000000000, 0.6640625000000000000, 0.6660156250000000000, 0.6679687500000000000, 0.6699218750000000000, 0.6718750000000000000, 0.6738281250000000000, 0.6757812500000000000, 0.6777343750000000000, 0.6796875000000000000, 0.6816406250000000000, 0.6835937500000000000, 0.6855468750000000000, 0.6875000000000000000, 0.6894531250000000000, 0.6914062500000000000, 0.6933593750000000000, 0.6953125000000000000, 0.6972656250000000000, 0.6992187500000000000, 0.7011718750000000000, 0.7031250000000000000, 0.7050781250000000000, 0.7070312500000000000, 0.7089843750000000000, 0.7109375000000000000, 0.7128906250000000000, 0.7148437500000000000, 0.7167968750000000000, 0.7187500000000000000, 0.7207031250000000000, 0.7226562500000000000, 0.7246093750000000000, 0.7265625000000000000, 0.7285156250000000000, 0.7304687500000000000, 0.7324218750000000000, 0.7343750000000000000, 0.7363281250000000000, 0.7382812500000000000, 0.7402343750000000000, 0.7421875000000000000, 0.7441406250000000000, 0.7460937500000000000, 0.7480468750000000000, 0.7500000000000000000, 0.7519531250000000000, 0.7539062500000000000, 0.7558593750000000000, 0.7578125000000000000, 0.7597656250000000000, 0.7617187500000000000, 0.7636718750000000000, 0.7656250000000000000, 0.7675781250000000000, 0.7695312500000000000, 0.7714843750000000000, 0.7734375000000000000, 0.7753906250000000000, 0.7773437500000000000, 0.7792968750000000000, 0.7812500000000000000, 0.7832031250000000000, 0.7851562500000000000, 0.7871093750000000000, 0.7890625000000000000, 0.7910156250000000000, 0.7929687500000000000, 0.7949218750000000000, 0.7968750000000000000, 0.7988281250000000000, 0.8007812500000000000, 0.8027343750000000000, 0.8046875000000000000, 0.8066406250000000000, 0.8085937500000000000, 0.8105468750000000000, 0.8125000000000000000, 0.8144531250000000000, 0.8164062500000000000, 0.8183593750000000000, 0.8203125000000000000, 0.8222656250000000000, 0.8242187500000000000, 0.8261718750000000000, 0.8281250000000000000, 0.8300781250000000000, 0.8320312500000000000, 0.8339843750000000000, 0.8359375000000000000, 0.8378906250000000000, 0.8398437500000000000, 0.8417968750000000000, 0.8437500000000000000, 0.8457031250000000000, 0.8476562500000000000, 0.8496093750000000000, 0.8515625000000000000, 0.8535156250000000000, 0.8554687500000000000, 0.8574218750000000000, 0.8593750000000000000, 0.8613281250000000000, 0.8632812500000000000, 0.8652343750000000000, 0.8671875000000000000, 0.8691406250000000000, 0.8710937500000000000, 0.8730468750000000000, 0.8750000000000000000, 0.8769531250000000000, 0.8789062500000000000, 0.8808593750000000000, 0.8828125000000000000, 0.8847656250000000000, 0.8867187500000000000, 0.8886718750000000000, 0.8906250000000000000, 0.8925781250000000000, 0.8945312500000000000, 0.8964843750000000000, 0.8984375000000000000, 0.9003906250000000000, 0.9023437500000000000, 0.9042968750000000000, 0.9062500000000000000, 0.9082031250000000000, 0.9101562500000000000, 0.9121093750000000000, 0.9140625000000000000, 0.9160156250000000000, 0.9179687500000000000, 0.9199218750000000000, 0.9218750000000000000, 0.9238281250000000000, 0.9257812500000000000, 0.9277343750000000000, 0.9296875000000000000, 0.9316406250000000000, 0.9335937500000000000, 0.9355468750000000000, 0.9375000000000000000, 0.9394531250000000000, 0.9414062500000000000, 0.9433593750000000000, 0.9453125000000000000, 0.9472656250000000000, 0.9492187500000000000, 0.9511718750000000000, 0.9531250000000000000, 0.9550781250000000000, 0.9570312500000000000, 0.9589843750000000000, 0.9609375000000000000, 0.9628906250000000000, 0.9648437500000000000, 0.9667968750000000000, 0.9687500000000000000, 0.9707031250000000000, 0.9726562500000000000, 0.9746093750000000000, 0.9765625000000000000, 0.9785156250000000000, 0.9791718287086115247 ),
 .UNSPECIFIED. ) 
 GEOMETRIC_REPRESENTATION_ITEM ( )  RATIONAL_B_SPLINE_SURFACE ( (
 ( 1.000000000000000000, 0.9807852804032304306, 1.000000000000000000, 0.9807852804032304306, 1.000000000000000000, 0.9807852804032304306, 1.000000000000000000, 0.9807852804032304306, 1.000000000000000000, 0.9807852804032304306, 1.000000000000000000, 0.9807852804032304306, 1.000000000000000000, 0.9807852804032304306, 1.000000000000000000, 0.9807852804032304306, 1.000000000000000000, 0.9807852804032304306, 1.000000000000000000, 0.9807852804032304306, 1.000000000000000000, 0.9807852804032304306, 1.000000000000000000, 0.9807852804032304306, 1.000000000000000000, 0.9807852804032304306, 1.000000000000000000, 0.9807852804032304306, 1.000000000000000000, 0.9807852804032304306, 1.000000000000000000, 0.9807852804032304306, 1.000000000000000000, 0.9807852804032304306, 1.000000000000000000, 0.9807852804032304306, 1.000000000000000000, 0.9807852804032304306, 1.000000000000000000, 0.9807852804032304306, 1.000000000000000000, 0.9807852804032304306, 1.000000000000000000, 0.9807852804032304306, 1.000000000000000000, 0.9807852804032304306, 1.000000000000000000, 0.9807852804032304306, 1.000000000000000000, 0.9807852804032304306, 1.000000000000000000, 0.9807852804032304306, 1.000000000000000000, 0.9807852804032304306, 1.000000000000000000, 0.9807852804032304306, 1.000000000000000000, 0.9807852804032304306, 1.000000000000000000, 0.9807852804032304306, 1.000000000000000000, 0.9807852804032304306, 1.000000000000000000, 0.9807852804032304306, 1.000000000000000000, 0.9807852804032304306, 1.000000000000000000, 0.9807852804032304306, 1.000000000000000000, 0.9807852804032304306, 1.000000000000000000, 0.9807852804032304306, 1.000000000000000000, 0.9807852804032304306, 1.000000000000000000, 0.9807852804032304306, 1.000000000000000000, 0.9807852804032304306, 1.000000000000000000, 0.9807852804032304306, 1.000000000000000000, 0.9807852804032304306, 1.000000000000000000, 0.9807852804032304306, 1.000000000000000000, 0.9807852804032304306, 1.000000000000000000, 0.9807852804032304306, 1.000000000000000000, 0.9807852804032304306, 1.000000000000000000, 0.9807852804032304306, 1.000000000000000000, 0.9807852804032304306, 1.000000000000000000, 0.9807852804032304306, 1.000000000000000000, 0.9807852804032304306, 1.000000000000000000, 0.9807852804032304306, 1.000000000000000000, 0.9807852804032304306, 1.000000000000000000, 0.9807852804032304306, 1.000000000000000000, 0.9807852804032304306, 1.000000000000000000, 0.9807852804032304306, 1.000000000000000000, 0.9807852804032304306, 1.000000000000000000, 0.9807852804032304306, 1.000000000000000000, 0.9807852804032304306, 1.000000000000000000, 0.9807852804032304306, 1.000000000000000000, 0.9807852804032304306, 1.000000000000000000, 0.9807852804032304306, 1.000000000000000000, 0.9807852804032304306, 1.000000000000000000, 0.9807852804032304306, 1.000000000000000000, 0.9807852804032304306, 1.000000000000000000, 0.9807852804032304306, 1.000000000000000000, 0.9807852804032304306, 1.000000000000000000, 0.9807852804032304306, 1.000000000000000000, 0.9807852804032304306, 1.000000000000000000, 0.9807852804032304306, 1.000000000000000000, 0.9807852804032304306, 1.000000000000000000, 0.9807852804032304306, 1.000000000000000000, 0.9807852804032304306, 1.000000000000000000, 0.9807852804032304306, 1.000000000000000000, 0.9807852804032304306, 1.000000000000000000, 0.9807852804032304306, 1.000000000000000000, 0.9807852804032304306, 1.000000000000000000, 0.9807852804032304306, 1.000000000000000000, 0.9807852804032304306, 1.000000000000000000, 0.9807852804032304306, 1.000000000000000000, 0.9807852804032304306, 1.000000000000000000, 0.9807852804032304306, 1.000000000000000000, 0.9807852804032304306, 1.000000000000000000, 0.9807852804032304306, 1.000000000000000000, 0.9807852804032304306, 1.000000000000000000, 0.9807852804032304306, 1.000000000000000000, 0.9807852804032304306, 1.000000000000000000, 0.9807852804032304306, 1.000000000000000000, 0.9807852804032304306, 1.000000000000000000, 0.9807852804032304306, 1.000000000000000000, 0.9807852804032304306, 1.000000000000000000, 0.9807852804032304306, 1.000000000000000000, 0.9807852804032304306, 1.000000000000000000, 0.9807852804032304306, 1.000000000000000000, 0.9807852804032304306, 1.000000000000000000, 0.9807852804032304306, 1.000000000000000000, 0.9807852804032304306, 1.000000000000000000, 0.9807852804032304306, 1.000000000000000000, 0.9807852804032304306, 1.000000000000000000, 0.9807852804032304306, 1.000000000000000000, 0.9807852804032304306, 1.000000000000000000, 0.9807852804032304306, 1.000000000000000000, 0.9807852804032304306, 1.000000000000000000, 0.9807852804032304306, 1.000000000000000000, 0.9807852804032304306, 1.000000000000000000, 0.9807852804032304306, 1.000000000000000000, 0.9807852804032304306, 1.000000000000000000, 0.9807852804032304306, 1.000000000000000000, 0.9807852804032304306, 1.000000000000000000, 0.9807852804032304306, 1.000000000000000000, 0.9807852804032304306, 1.000000000000000000, 0.9807852804032304306, 1.000000000000000000, 0.9807852804032304306, 1.000000000000000000, 0.9807852804032304306, 1.000000000000000000, 0.9807852804032304306, 1.000000000000000000, 0.9807852804032304306, 1.000000000000000000, 0.9807852804032304306, 1.000000000000000000, 0.9807852804032304306, 1.000000000000000000, 0.9807852804032304306, 1.000000000000000000, 0.9807852804032304306, 1.000000000000000000, 0.9807852804032304306, 1.000000000000000000, 0.9807852804032304306, 1.000000000000000000, 0.9807852804032304306, 1.000000000000000000, 0.9807852804032304306, 1.000000000000000000, 0.9807852804032304306, 1.000000000000000000, 0.9807852804032304306, 1.000000000000000000, 0.9807852804032304306, 1.000000000000000000, 0.9807852804032304306, 1.000000000000000000, 0.9807852804032304306, 1.000000000000000000, 0.9807852804032304306, 1.000000000000000000, 0.9807852804032304306, 1.000000000000000000, 0.9807852804032304306, 1.000000000000000000, 0.9807852804032304306, 1.000000000000000000, 0.9807852804032304306, 1.000000000000000000, 0.9807852804032304306, 1.000000000000000000, 0.9807852804032304306, 1.000000000000000000, 0.9807852804032304306, 1.000000000000000000, 0.9807852804032304306, 1.000000000000000000, 0.9807852804032304306, 1.000000000000000000, 0.9807852804032304306, 1.000000000000000000, 0.9807852804032304306, 1.000000000000000000, 0.9807852804032304306, 1.000000000000000000, 0.9807852804032304306, 1.000000000000000000, 0.9807852804032304306, 1.000000000000000000, 0.9807852804032304306, 1.000000000000000000, 0.9807852804032304306, 1.000000000000000000, 0.9807852804032304306, 1.000000000000000000, 0.9807852804032304306, 1.000000000000000000, 0.9807852804032304306, 1.000000000000000000, 0.9807852804032304306, 1.000000000000000000, 0.9807852804032304306, 1.000000000000000000, 0.9807852804032304306, 1.000000000000000000, 0.9807852804032304306, 1.000000000000000000, 0.9807852804032304306, 1.000000000000000000, 0.9807852804032304306, 1.000000000000000000, 0.9807852804032304306, 1.000000000000000000, 0.9807852804032304306, 1.000000000000000000, 0.9807852804032304306, 1.000000000000000000, 0.9807852804032304306, 1.000000000000000000, 0.9807852804032304306, 1.000000000000000000, 0.9807852804032304306, 1.000000000000000000, 0.9807852804032304306, 1.000000000000000000, 0.9807852804032304306, 1.000000000000000000, 0.9807852804032304306, 1.000000000000000000, 0.9807852804032304306, 1.000000000000000000, 0.9807852804032304306, 1.000000000000000000, 0.9807852804032304306, 1.000000000000000000, 0.9807852804032304306, 1.000000000000000000, 0.9807852804032304306, 1.000000000000000000, 0.9807852804032304306, 1.000000000000000000, 0.9807852804032304306, 1.000000000000000000, 0.9807852804032304306, 1.000000000000000000, 0.9807852804032304306, 1.000000000000000000, 0.9807852804032304306, 1.000000000000000000, 0.9807852804032304306, 1.000000000000000000, 0.9807852804032304306, 1.000000000000000000, 0.9807852804032304306, 1.000000000000000000, 0.9807852804032304306, 1.000000000000000000, 0.9807852804032304306, 1.000000000000000000, 0.9807852804032304306, 1.000000000000000000, 0.9807852804032304306, 1.000000000000000000, 0.9807852804032304306, 1.000000000000000000, 0.9807852804032304306, 1.000000000000000000, 0.9807852804032304306, 1.000000000000000000, 0.9807852804032304306, 1.000000000000000000, 0.9807852804032304306, 1.000000000000000000, 0.9807852804032304306, 1.000000000000000000, 0.9807852804032304306, 1.000000000000000000, 0.9807852804032304306, 1.000000000000000000, 0.9807852804032304306, 1.000000000000000000, 0.9807852804032304306, 1.000000000000000000, 0.9807852804032304306, 1.000000000000000000, 0.9807852804032304306, 1.000000000000000000, 0.9807852804032304306, 1.000000000000000000, 0.9807852804032304306, 1.000000000000000000, 0.9807852804032304306, 1.000000000000000000, 0.9807852804032304306, 1.000000000000000000, 0.9807852804032304306, 1.000000000000000000, 0.9807852804032304306, 1.000000000000000000, 0.9807852804032304306, 1.000000000000000000, 0.9807852804032304306, 1.000000000000000000, 0.9807852804032304306, 1.000000000000000000, 0.9807852804032304306, 1.000000000000000000, 0.9807852804032304306, 1.000000000000000000, 0.9807852804032304306, 1.000000000000000000, 0.9807852804032304306, 1.000000000000000000, 0.9807852804032304306, 1.000000000000000000, 0.9807852804032304306, 1.000000000000000000, 0.9807852804032304306, 1.000000000000000000, 0.9807852804032304306, 1.000000000000000000, 0.9807852804032304306, 1.000000000000000000, 0.9807852804032304306, 1.000000000000000000, 0.9807852804032304306, 1.000000000000000000, 0.9807852804032304306, 1.000000000000000000, 0.9807852804032304306, 1.000000000000000000, 0.9807852804032304306, 1.000000000000000000, 0.9807852804032304306, 1.000000000000000000, 0.9807852804032304306, 1.000000000000000000, 0.9807852804032304306, 1.000000000000000000, 0.9807852804032304306, 1.000000000000000000, 0.9807852804032304306, 1.000000000000000000, 0.9807852804032304306, 1.000000000000000000, 0.9807852804032304306, 1.000000000000000000, 0.9807852804032304306, 1.000000000000000000, 0.9807852804032304306, 1.000000000000000000, 0.9807852804032304306, 1.000000000000000000, 0.9807852804032304306, 1.000000000000000000, 0.9807852804032304306, 1.000000000000000000, 0.9807852804032304306, 1.000000000000000000, 0.9807852804032304306, 1.000000000000000000, 0.9807852804032304306, 1.000000000000000000, 0.9807852804032304306, 1.000000000000000000, 0.9807852804032304306, 1.000000000000000000, 0.9807852804032304306, 1.000000000000000000, 0.9807852804032304306, 1.000000000000000000, 0.9807852804032304306, 1.000000000000000000, 0.9807852804032304306, 1.000000000000000000, 0.9807852804032304306, 1.000000000000000000, 0.9807852804032304306, 1.000000000000000000, 0.9807852804032304306, 1.000000000000000000, 0.9807852804032304306, 1.000000000000000000, 0.9807852804032304306, 1.000000000000000000, 0.9807852804032304306, 1.000000000000000000, 0.9807852804032304306, 1.000000000000000000, 0.9807852804032304306, 1.000000000000000000, 0.9807852804032304306, 1.000000000000000000, 0.9807852804032304306, 1.000000000000000000, 0.9807852804032304306, 1.000000000000000000, 0.9807852804032304306, 1.000000000000000000, 0.9807852804032304306, 1.000000000000000000, 0.9807852804032304306, 1.000000000000000000, 0.9807852804032304306, 1.000000000000000000, 0.9807852804032304306, 1.000000000000000000, 0.9807852804032304306, 1.000000000000000000, 0.9807852804032304306, 1.000000000000000000, 0.9807852804032304306, 1.000000000000000000, 0.9807852804032304306, 1.000000000000000000, 0.9807852804032304306, 1.000000000000000000, 0.9807852804032304306, 1.000000000000000000, 0.9807852804032304306, 1.000000000000000000, 0.9807852804032304306, 1.000000000000000000, 0.9807852804032304306, 1.000000000000000000, 0.9807852804032304306, 1.000000000000000000, 0.9807852804032304306, 1.000000000000000000, 0.9807852804032304306, 1.000000000000000000, 0.9807852804032304306, 1.000000000000000000, 0.9807852804032304306, 1.000000000000000000, 0.9807852804032304306, 1.000000000000000000, 0.9807852804032304306, 1.000000000000000000, 0.9807852804032304306, 1.000000000000000000, 0.9807852804032304306, 1.000000000000000000, 0.9807852804032304306, 1.000000000000000000, 0.9807852804032304306, 1.000000000000000000, 0.9807852804032304306, 1.000000000000000000, 0.9807852804032304306, 1.000000000000000000, 0.9807852804032304306, 1.000000000000000000, 0.9807852804032304306, 1.000000000000000000, 0.9807852804032304306, 1.000000000000000000, 0.9807852804032304306, 1.000000000000000000, 0.9807852804032304306, 1.000000000000000000, 0.9807852804032304306, 1.000000000000000000, 0.9807852804032304306, 1.000000000000000000, 0.9807852804032304306, 1.000000000000000000, 0.9807852804032304306, 1.000000000000000000, 0.9807852804032304306, 1.000000000000000000, 0.9807852804032304306, 1.000000000000000000, 0.9807852804032304306, 1.000000000000000000, 0.9807852804032304306, 1.000000000000000000, 0.9807852804032304306, 1.000000000000000000, 0.9807852804032304306, 1.000000000000000000, 0.9807852804032304306, 1.000000000000000000, 0.9807852804032304306, 1.000000000000000000, 0.9807852804032304306, 1.000000000000000000, 0.9807852804032304306, 1.000000000000000000, 0.9807852804032304306, 1.000000000000000000, 0.9807852804032304306, 1.000000000000000000, 0.9807852804032304306, 1.000000000000000000, 0.9807852804032304306, 1.000000000000000000, 0.9807852804032304306, 1.000000000000000000, 0.9807852804032304306, 1.000000000000000000, 0.9807852804032304306, 1.000000000000000000, 0.9807852804032304306, 1.000000000000000000, 0.9807852804032304306, 1.000000000000000000, 0.9807852804032304306, 1.000000000000000000, 0.9807852804032304306, 1.000000000000000000, 0.9807852804032304306, 1.000000000000000000, 0.9807852804032304306, 1.000000000000000000, 0.9807852804032304306, 1.000000000000000000, 0.9807852804032304306, 1.000000000000000000, 0.9807852804032304306, 1.000000000000000000, 0.9807852804032304306, 1.000000000000000000, 0.9807852804032304306, 1.000000000000000000, 0.9807852804032304306, 1.000000000000000000, 0.9807852804032304306, 1.000000000000000000, 0.9807852804032304306, 1.000000000000000000, 0.9807852804032304306, 1.000000000000000000, 0.9807852804032304306, 1.000000000000000000, 0.9807852804032304306, 1.000000000000000000, 0.9807852804032304306, 1.000000000000000000, 0.9807852804032304306, 1.000000000000000000, 0.9807852804032304306, 1.000000000000000000, 0.9807852804032304306, 1.000000000000000000, 0.9807852804032304306, 1.000000000000000000, 0.9807852804032304306, 1.000000000000000000, 0.9807852804032304306, 1.000000000000000000, 0.9807852804032304306, 1.000000000000000000, 0.9807852804032304306, 1.000000000000000000, 0.9807852804032304306, 1.000000000000000000, 0.9807852804032304306, 1.000000000000000000, 0.9807852804032304306, 1.000000000000000000, 0.9807852804032304306, 1.000000000000000000, 0.9807852804032304306, 1.000000000000000000, 0.9807852804032304306, 1.000000000000000000, 0.9807852804032304306, 1.000000000000000000, 0.9807852804032304306, 1.000000000000000000, 0.9807852804032304306, 1.000000000000000000, 0.9807852804032304306, 1.000000000000000000, 0.9807852804032304306, 1.000000000000000000, 0.9807852804032304306, 1.000000000000000000, 0.9807852804032304306, 1.000000000000000000, 0.9807852804032304306, 1.000000000000000000, 0.9807852804032304306, 1.000000000000000000, 0.9807852804032304306, 1.000000000000000000, 0.9807852804032304306, 1.000000000000000000, 0.9807852804032304306, 1.000000000000000000, 0.9807852804032304306, 1.000000000000000000, 0.9807852804032304306, 1.000000000000000000, 0.9807852804032304306, 1.000000000000000000, 0.9807852804032304306, 1.000000000000000000, 0.9807852804032304306, 1.000000000000000000, 0.9807852804032304306, 1.000000000000000000, 0.9807852804032304306, 1.000000000000000000, 0.9807852804032304306, 1.000000000000000000, 0.9807852804032304306, 1.000000000000000000, 0.9807852804032304306, 1.000000000000000000, 0.9807852804032304306, 1.000000000000000000, 0.9807852804032304306, 1.000000000000000000, 0.9807852804032304306, 1.000000000000000000, 0.9807852804032304306, 1.000000000000000000, 0.9807852804032304306, 1.000000000000000000, 0.9807852804032304306, 1.000000000000000000, 0.9807852804032304306, 1.000000000000000000, 0.9807852804032304306, 1.000000000000000000, 0.9807852804032304306, 1.000000000000000000, 0.9807852804032304306, 1.000000000000000000, 0.9807852804032304306, 1.000000000000000000, 0.9807852804032304306, 1.000000000000000000, 0.9807852804032304306, 1.000000000000000000, 0.9807852804032304306, 1.000000000000000000, 0.9807852804032304306, 1.000000000000000000, 0.9807852804032304306, 1.000000000000000000, 0.9807852804032304306, 1.000000000000000000, 0.9807852804032304306, 1.000000000000000000, 0.9807852804032304306, 1.000000000000000000, 0.9807852804032304306, 1.000000000000000000, 0.9807852804032304306, 1.000000000000000000, 0.9807852804032304306, 1.000000000000000000, 0.9807852804032304306, 1.000000000000000000, 0.9807852804032304306, 1.000000000000000000, 0.9807852804032304306, 1.000000000000000000, 0.9807852804032304306, 1.000000000000000000, 0.9807852804032304306, 1.000000000000000000, 0.9807852804032304306, 1.000000000000000000, 0.9807852804032304306, 1.000000000000000000, 0.9807852804032304306, 1.000000000000000000, 0.9807852804032304306, 1.000000000000000000, 0.9807852804032304306, 1.000000000000000000, 0.9807852804032304306, 1.000000000000000000, 0.9807852804032304306, 1.000000000000000000, 0.9807852804032304306, 1.000000000000000000, 0.9807852804032304306, 1.000000000000000000, 0.9807852804032304306, 1.000000000000000000, 0.9807852804032304306, 1.000000000000000000, 0.9807852804032304306, 1.000000000000000000, 0.9807852804032304306, 1.000000000000000000, 0.9807852804032304306, 1.000000000000000000, 0.9807852804032304306, 1.000000000000000000, 0.9807852804032304306, 1.000000000000000000, 0.9807852804032304306, 1.000000000000000000, 0.9807852804032304306, 1.000000000000000000, 0.9807852804032304306, 1.000000000000000000, 0.9807852804032304306, 1.000000000000000000, 0.9807852804032304306, 1.000000000000000000, 0.9807852804032304306, 1.000000000000000000, 0.9807852804032304306, 1.000000000000000000, 0.9807852804032304306, 1.000000000000000000, 0.9807852804032304306, 1.000000000000000000, 0.9807852804032304306, 1.000000000000000000, 0.9807852804032304306, 1.000000000000000000, 0.9807852804032304306, 1.000000000000000000, 0.9807852804032304306, 1.000000000000000000, 0.9807852804032304306, 1.000000000000000000, 0.9807852804032304306, 1.000000000000000000, 0.9807852804032304306, 1.000000000000000000, 0.9807852804032304306, 1.000000000000000000, 0.9807852804032304306, 1.000000000000000000, 0.9807852804032304306, 1.000000000000000000, 0.9807852804032304306, 1.000000000000000000, 0.9807852804032304306, 1.000000000000000000, 0.9807852804032304306, 1.000000000000000000, 0.9807852804032304306, 1.000000000000000000, 0.9807852804032304306, 1.000000000000000000, 0.9807852804032304306, 1.000000000000000000, 0.9807852804032304306, 1.000000000000000000, 0.9807852804032304306, 1.000000000000000000, 0.9807852804032304306, 1.000000000000000000, 0.9807852804032304306, 1.000000000000000000, 0.9807852804032304306, 1.000000000000000000, 0.9807852804032304306, 1.000000000000000000, 0.9807852804032304306, 1.000000000000000000, 0.9807852804032304306, 1.000000000000000000, 0.9807852804032304306, 1.000000000000000000, 0.9807852804032304306, 1.000000000000000000, 0.9807852804032304306, 1.000000000000000000, 0.9807852804032304306, 1.000000000000000000, 0.9807852804032304306, 1.000000000000000000, 0.9807852804032304306, 1.000000000000000000, 0.9807852804032304306, 1.000000000000000000, 0.9807852804032304306, 1.000000000000000000, 0.9807852804032304306, 1.000000000000000000, 0.9807852804032304306, 1.000000000000000000, 0.9807852804032304306, 1.000000000000000000, 0.9807852804032304306, 1.000000000000000000, 0.9807852804032304306, 1.000000000000000000, 0.9807852804032304306, 1.000000000000000000, 0.9807852804032304306, 1.000000000000000000, 0.9807852804032304306, 1.000000000000000000, 0.9807852804032304306, 1.000000000000000000, 0.9807852804032304306, 1.000000000000000000, 0.9807852804032304306, 1.000000000000000000, 0.9807852804032304306, 1.000000000000000000, 0.9807852804032304306, 1.000000000000000000, 0.9807852804032304306, 1.000000000000000000, 0.9807852804032304306, 1.000000000000000000, 0.9807852804032304306, 1.000000000000000000, 0.9807852804032304306, 1.000000000000000000, 0.9807852804032304306, 1.000000000000000000, 0.9807852804032304306, 1.000000000000000000, 0.9807852804032304306, 1.000000000000000000, 0.9807852804032304306, 1.000000000000000000, 0.9807852804032304306, 1.000000000000000000, 0.9807852804032304306, 1.000000000000000000, 0.9807852804032304306, 1.000000000000000000, 0.9807852804032304306, 1.000000000000000000, 0.9807852804032304306, 1.000000000000000000, 0.9807852804032304306, 1.000000000000000000, 0.9807852804032304306, 1.000000000000000000, 0.9807852804032304306, 1.000000000000000000, 0.9807852804032304306, 1.000000000000000000, 0.9807852804032304306, 1.000000000000000000, 0.9807852804032304306, 1.000000000000000000, 0.9807852804032304306, 1.000000000000000000, 0.9807852804032304306, 1.000000000000000000, 0.9807852804032304306, 1.000000000000000000, 0.9807852804032304306, 1.000000000000000000, 0.9807852804032304306, 1.000000000000000000, 0.9807852804032304306, 1.000000000000000000, 0.9807852804032304306, 1.000000000000000000, 0.9807852804032304306, 1.000000000000000000, 0.9807852804032304306, 1.000000000000000000, 0.9807852804032304306, 1.000000000000000000, 0.9807852804032304306, 1.000000000000000000, 0.9807852804032304306, 1.000000000000000000, 0.9807852804032304306, 1.000000000000000000, 0.9807852804032304306, 1.000000000000000000, 0.9807852804032304306, 1.000000000000000000, 0.9807852804032304306, 1.000000000000000000, 0.9807852804032304306, 1.000000000000000000, 0.9807852804032304306, 1.000000000000000000, 0.9807852804032304306, 1.000000000000000000, 0.9807852804032304306, 1.000000000000000000, 0.9807852804032304306, 1.000000000000000000, 0.9807852804032304306, 1.000000000000000000, 0.9807852804032304306, 1.000000000000000000, 0.9807852804032304306, 1.000000000000000000, 0.9807852804032304306, 1.000000000000000000, 0.9807852804032304306, 1.000000000000000000, 0.9807852804032304306, 1.000000000000000000, 0.9807852804032304306, 1.000000000000000000, 0.9807852804032304306, 1.000000000000000000, 0.9807852804032304306, 1.000000000000000000, 0.9807852804032304306, 1.000000000000000000, 0.9807852804032304306, 1.000000000000000000, 0.9935443096272227326, 0.9914265371698519624),
 ( 1.000000000000000000, 0.9807852804032304306, 1.000000000000000000, 0.9807852804032304306, 1.000000000000000000, 0.9807852804032304306, 1.000000000000000000, 0.9807852804032304306, 1.000000000000000000, 0.9807852804032304306, 1.000000000000000000, 0.9807852804032304306, 1.000000000000000000, 0.9807852804032304306, 1.000000000000000000, 0.9807852804032304306, 1.000000000000000000, 0.9807852804032304306, 1.000000000000000000, 0.9807852804032304306, 1.000000000000000000, 0.9807852804032304306, 1.000000000000000000, 0.9807852804032304306, 1.000000000000000000, 0.9807852804032304306, 1.000000000000000000, 0.9807852804032304306, 1.000000000000000000, 0.9807852804032304306, 1.000000000000000000, 0.9807852804032304306, 1.000000000000000000, 0.9807852804032304306, 1.000000000000000000, 0.9807852804032304306, 1.000000000000000000, 0.9807852804032304306, 1.000000000000000000, 0.9807852804032304306, 1.000000000000000000, 0.9807852804032304306, 1.000000000000000000, 0.9807852804032304306, 1.000000000000000000, 0.9807852804032304306, 1.000000000000000000, 0.9807852804032304306, 1.000000000000000000, 0.9807852804032304306, 1.000000000000000000, 0.9807852804032304306, 1.000000000000000000, 0.9807852804032304306, 1.000000000000000000, 0.9807852804032304306, 1.000000000000000000, 0.9807852804032304306, 1.000000000000000000, 0.9807852804032304306, 1.000000000000000000, 0.9807852804032304306, 1.000000000000000000, 0.9807852804032304306, 1.000000000000000000, 0.9807852804032304306, 1.000000000000000000, 0.9807852804032304306, 1.000000000000000000, 0.9807852804032304306, 1.000000000000000000, 0.9807852804032304306, 1.000000000000000000, 0.9807852804032304306, 1.000000000000000000, 0.9807852804032304306, 1.000000000000000000, 0.9807852804032304306, 1.000000000000000000, 0.9807852804032304306, 1.000000000000000000, 0.9807852804032304306, 1.000000000000000000, 0.9807852804032304306, 1.000000000000000000, 0.9807852804032304306, 1.000000000000000000, 0.9807852804032304306, 1.000000000000000000, 0.9807852804032304306, 1.000000000000000000, 0.9807852804032304306, 1.000000000000000000, 0.9807852804032304306, 1.000000000000000000, 0.9807852804032304306, 1.000000000000000000, 0.9807852804032304306, 1.000000000000000000, 0.9807852804032304306, 1.000000000000000000, 0.9807852804032304306, 1.000000000000000000, 0.9807852804032304306, 1.000000000000000000, 0.9807852804032304306, 1.000000000000000000, 0.9807852804032304306, 1.000000000000000000, 0.9807852804032304306, 1.000000000000000000, 0.9807852804032304306, 1.000000000000000000, 0.9807852804032304306, 1.000000000000000000, 0.9807852804032304306, 1.000000000000000000, 0.9807852804032304306, 1.000000000000000000, 0.9807852804032304306, 1.000000000000000000, 0.9807852804032304306, 1.000000000000000000, 0.9807852804032304306, 1.000000000000000000, 0.9807852804032304306, 1.000000000000000000, 0.9807852804032304306, 1.000000000000000000, 0.9807852804032304306, 1.000000000000000000, 0.9807852804032304306, 1.000000000000000000, 0.9807852804032304306, 1.000000000000000000, 0.9807852804032304306, 1.000000000000000000, 0.9807852804032304306, 1.000000000000000000, 0.9807852804032304306, 1.000000000000000000, 0.9807852804032304306, 1.000000000000000000, 0.9807852804032304306, 1.000000000000000000, 0.9807852804032304306, 1.000000000000000000, 0.9807852804032304306, 1.000000000000000000, 0.9807852804032304306, 1.000000000000000000, 0.9807852804032304306, 1.000000000000000000, 0.9807852804032304306, 1.000000000000000000, 0.9807852804032304306, 1.000000000000000000, 0.9807852804032304306, 1.000000000000000000, 0.9807852804032304306, 1.000000000000000000, 0.9807852804032304306, 1.000000000000000000, 0.9807852804032304306, 1.000000000000000000, 0.9807852804032304306, 1.000000000000000000, 0.9807852804032304306, 1.000000000000000000, 0.9807852804032304306, 1.000000000000000000, 0.9807852804032304306, 1.000000000000000000, 0.9807852804032304306, 1.000000000000000000, 0.9807852804032304306, 1.000000000000000000, 0.9807852804032304306, 1.000000000000000000, 0.9807852804032304306, 1.000000000000000000, 0.9807852804032304306, 1.000000000000000000, 0.9807852804032304306, 1.000000000000000000, 0.9807852804032304306, 1.000000000000000000, 0.9807852804032304306, 1.000000000000000000, 0.9807852804032304306, 1.000000000000000000, 0.9807852804032304306, 1.000000000000000000, 0.9807852804032304306, 1.000000000000000000, 0.9807852804032304306, 1.000000000000000000, 0.9807852804032304306, 1.000000000000000000, 0.9807852804032304306, 1.000000000000000000, 0.9807852804032304306, 1.000000000000000000, 0.9807852804032304306, 1.000000000000000000, 0.9807852804032304306, 1.000000000000000000, 0.9807852804032304306, 1.000000000000000000, 0.9807852804032304306, 1.000000000000000000, 0.9807852804032304306, 1.000000000000000000, 0.9807852804032304306, 1.000000000000000000, 0.9807852804032304306, 1.000000000000000000, 0.9807852804032304306, 1.000000000000000000, 0.9807852804032304306, 1.000000000000000000, 0.9807852804032304306, 1.000000000000000000, 0.9807852804032304306, 1.000000000000000000, 0.9807852804032304306, 1.000000000000000000, 0.9807852804032304306, 1.000000000000000000, 0.9807852804032304306, 1.000000000000000000, 0.9807852804032304306, 1.000000000000000000, 0.9807852804032304306, 1.000000000000000000, 0.9807852804032304306, 1.000000000000000000, 0.9807852804032304306, 1.000000000000000000, 0.9807852804032304306, 1.000000000000000000, 0.9807852804032304306, 1.000000000000000000, 0.9807852804032304306, 1.000000000000000000, 0.9807852804032304306, 1.000000000000000000, 0.9807852804032304306, 1.000000000000000000, 0.9807852804032304306, 1.000000000000000000, 0.9807852804032304306, 1.000000000000000000, 0.9807852804032304306, 1.000000000000000000, 0.9807852804032304306, 1.000000000000000000, 0.9807852804032304306, 1.000000000000000000, 0.9807852804032304306, 1.000000000000000000, 0.9807852804032304306, 1.000000000000000000, 0.9807852804032304306, 1.000000000000000000, 0.9807852804032304306, 1.000000000000000000, 0.9807852804032304306, 1.000000000000000000, 0.9807852804032304306, 1.000000000000000000, 0.9807852804032304306, 1.000000000000000000, 0.9807852804032304306, 1.000000000000000000, 0.9807852804032304306, 1.000000000000000000, 0.9807852804032304306, 1.000000000000000000, 0.9807852804032304306, 1.000000000000000000, 0.9807852804032304306, 1.000000000000000000, 0.9807852804032304306, 1.000000000000000000, 0.9807852804032304306, 1.000000000000000000, 0.9807852804032304306, 1.000000000000000000, 0.9807852804032304306, 1.000000000000000000, 0.9807852804032304306, 1.000000000000000000, 0.9807852804032304306, 1.000000000000000000, 0.9807852804032304306, 1.000000000000000000, 0.9807852804032304306, 1.000000000000000000, 0.9807852804032304306, 1.000000000000000000, 0.9807852804032304306, 1.000000000000000000, 0.9807852804032304306, 1.000000000000000000, 0.9807852804032304306, 1.000000000000000000, 0.9807852804032304306, 1.000000000000000000, 0.9807852804032304306, 1.000000000000000000, 0.9807852804032304306, 1.000000000000000000, 0.9807852804032304306, 1.000000000000000000, 0.9807852804032304306, 1.000000000000000000, 0.9807852804032304306, 1.000000000000000000, 0.9807852804032304306, 1.000000000000000000, 0.9807852804032304306, 1.000000000000000000, 0.9807852804032304306, 1.000000000000000000, 0.9807852804032304306, 1.000000000000000000, 0.9807852804032304306, 1.000000000000000000, 0.9807852804032304306, 1.000000000000000000, 0.9807852804032304306, 1.000000000000000000, 0.9807852804032304306, 1.000000000000000000, 0.9807852804032304306, 1.000000000000000000, 0.9807852804032304306, 1.000000000000000000, 0.9807852804032304306, 1.000000000000000000, 0.9807852804032304306, 1.000000000000000000, 0.9807852804032304306, 1.000000000000000000, 0.9807852804032304306, 1.000000000000000000, 0.9807852804032304306, 1.000000000000000000, 0.9807852804032304306, 1.000000000000000000, 0.9807852804032304306, 1.000000000000000000, 0.9807852804032304306, 1.000000000000000000, 0.9807852804032304306, 1.000000000000000000, 0.9807852804032304306, 1.000000000000000000, 0.9807852804032304306, 1.000000000000000000, 0.9807852804032304306, 1.000000000000000000, 0.9807852804032304306, 1.000000000000000000, 0.9807852804032304306, 1.000000000000000000, 0.9807852804032304306, 1.000000000000000000, 0.9807852804032304306, 1.000000000000000000, 0.9807852804032304306, 1.000000000000000000, 0.9807852804032304306, 1.000000000000000000, 0.9807852804032304306, 1.000000000000000000, 0.9807852804032304306, 1.000000000000000000, 0.9807852804032304306, 1.000000000000000000, 0.9807852804032304306, 1.000000000000000000, 0.9807852804032304306, 1.000000000000000000, 0.9807852804032304306, 1.000000000000000000, 0.9807852804032304306, 1.000000000000000000, 0.9807852804032304306, 1.000000000000000000, 0.9807852804032304306, 1.000000000000000000, 0.9807852804032304306, 1.000000000000000000, 0.9807852804032304306, 1.000000000000000000, 0.9807852804032304306, 1.000000000000000000, 0.9807852804032304306, 1.000000000000000000, 0.9807852804032304306, 1.000000000000000000, 0.9807852804032304306, 1.000000000000000000, 0.9807852804032304306, 1.000000000000000000, 0.9807852804032304306, 1.000000000000000000, 0.9807852804032304306, 1.000000000000000000, 0.9807852804032304306, 1.000000000000000000, 0.9807852804032304306, 1.000000000000000000, 0.9807852804032304306, 1.000000000000000000, 0.9807852804032304306, 1.000000000000000000, 0.9807852804032304306, 1.000000000000000000, 0.9807852804032304306, 1.000000000000000000, 0.9807852804032304306, 1.000000000000000000, 0.9807852804032304306, 1.000000000000000000, 0.9807852804032304306, 1.000000000000000000, 0.9807852804032304306, 1.000000000000000000, 0.9807852804032304306, 1.000000000000000000, 0.9807852804032304306, 1.000000000000000000, 0.9807852804032304306, 1.000000000000000000, 0.9807852804032304306, 1.000000000000000000, 0.9807852804032304306, 1.000000000000000000, 0.9807852804032304306, 1.000000000000000000, 0.9807852804032304306, 1.000000000000000000, 0.9807852804032304306, 1.000000000000000000, 0.9807852804032304306, 1.000000000000000000, 0.9807852804032304306, 1.000000000000000000, 0.9807852804032304306, 1.000000000000000000, 0.9807852804032304306, 1.000000000000000000, 0.9807852804032304306, 1.000000000000000000, 0.9807852804032304306, 1.000000000000000000, 0.9807852804032304306, 1.000000000000000000, 0.9807852804032304306, 1.000000000000000000, 0.9807852804032304306, 1.000000000000000000, 0.9807852804032304306, 1.000000000000000000, 0.9807852804032304306, 1.000000000000000000, 0.9807852804032304306, 1.000000000000000000, 0.9807852804032304306, 1.000000000000000000, 0.9807852804032304306, 1.000000000000000000, 0.9807852804032304306, 1.000000000000000000, 0.9807852804032304306, 1.000000000000000000, 0.9807852804032304306, 1.000000000000000000, 0.9807852804032304306, 1.000000000000000000, 0.9807852804032304306, 1.000000000000000000, 0.9807852804032304306, 1.000000000000000000, 0.9807852804032304306, 1.000000000000000000, 0.9807852804032304306, 1.000000000000000000, 0.9807852804032304306, 1.000000000000000000, 0.9807852804032304306, 1.000000000000000000, 0.9807852804032304306, 1.000000000000000000, 0.9807852804032304306, 1.000000000000000000, 0.9807852804032304306, 1.000000000000000000, 0.9807852804032304306, 1.000000000000000000, 0.9807852804032304306, 1.000000000000000000, 0.9807852804032304306, 1.000000000000000000, 0.9807852804032304306, 1.000000000000000000, 0.9807852804032304306, 1.000000000000000000, 0.9807852804032304306, 1.000000000000000000, 0.9807852804032304306, 1.000000000000000000, 0.9807852804032304306, 1.000000000000000000, 0.9807852804032304306, 1.000000000000000000, 0.9807852804032304306, 1.000000000000000000, 0.9807852804032304306, 1.000000000000000000, 0.9807852804032304306, 1.000000000000000000, 0.9807852804032304306, 1.000000000000000000, 0.9807852804032304306, 1.000000000000000000, 0.9807852804032304306, 1.000000000000000000, 0.9807852804032304306, 1.000000000000000000, 0.9807852804032304306, 1.000000000000000000, 0.9807852804032304306, 1.000000000000000000, 0.9807852804032304306, 1.000000000000000000, 0.9807852804032304306, 1.000000000000000000, 0.9807852804032304306, 1.000000000000000000, 0.9807852804032304306, 1.000000000000000000, 0.9807852804032304306, 1.000000000000000000, 0.9807852804032304306, 1.000000000000000000, 0.9807852804032304306, 1.000000000000000000, 0.9807852804032304306, 1.000000000000000000, 0.9807852804032304306, 1.000000000000000000, 0.9807852804032304306, 1.000000000000000000, 0.9807852804032304306, 1.000000000000000000, 0.9807852804032304306, 1.000000000000000000, 0.9807852804032304306, 1.000000000000000000, 0.9807852804032304306, 1.000000000000000000, 0.9807852804032304306, 1.000000000000000000, 0.9807852804032304306, 1.000000000000000000, 0.9807852804032304306, 1.000000000000000000, 0.9807852804032304306, 1.000000000000000000, 0.9807852804032304306, 1.000000000000000000, 0.9807852804032304306, 1.000000000000000000, 0.9807852804032304306, 1.000000000000000000, 0.9807852804032304306, 1.000000000000000000, 0.9807852804032304306, 1.000000000000000000, 0.9807852804032304306, 1.000000000000000000, 0.9807852804032304306, 1.000000000000000000, 0.9807852804032304306, 1.000000000000000000, 0.9807852804032304306, 1.000000000000000000, 0.9807852804032304306, 1.000000000000000000, 0.9807852804032304306, 1.000000000000000000, 0.9807852804032304306, 1.000000000000000000, 0.9807852804032304306, 1.000000000000000000, 0.9807852804032304306, 1.000000000000000000, 0.9807852804032304306, 1.000000000000000000, 0.9807852804032304306, 1.000000000000000000, 0.9807852804032304306, 1.000000000000000000, 0.9807852804032304306, 1.000000000000000000, 0.9807852804032304306, 1.000000000000000000, 0.9807852804032304306, 1.000000000000000000, 0.9807852804032304306, 1.000000000000000000, 0.9807852804032304306, 1.000000000000000000, 0.9807852804032304306, 1.000000000000000000, 0.9807852804032304306, 1.000000000000000000, 0.9807852804032304306, 1.000000000000000000, 0.9807852804032304306, 1.000000000000000000, 0.9807852804032304306, 1.000000000000000000, 0.9807852804032304306, 1.000000000000000000, 0.9807852804032304306, 1.000000000000000000, 0.9807852804032304306, 1.000000000000000000, 0.9807852804032304306, 1.000000000000000000, 0.9807852804032304306, 1.000000000000000000, 0.9807852804032304306, 1.000000000000000000, 0.9807852804032304306, 1.000000000000000000, 0.9807852804032304306, 1.000000000000000000, 0.9807852804032304306, 1.000000000000000000, 0.9807852804032304306, 1.000000000000000000, 0.9807852804032304306, 1.000000000000000000, 0.9807852804032304306, 1.000000000000000000, 0.9807852804032304306, 1.000000000000000000, 0.9807852804032304306, 1.000000000000000000, 0.9807852804032304306, 1.000000000000000000, 0.9807852804032304306, 1.000000000000000000, 0.9807852804032304306, 1.000000000000000000, 0.9807852804032304306, 1.000000000000000000, 0.9807852804032304306, 1.000000000000000000, 0.9807852804032304306, 1.000000000000000000, 0.9807852804032304306, 1.000000000000000000, 0.9807852804032304306, 1.000000000000000000, 0.9807852804032304306, 1.000000000000000000, 0.9807852804032304306, 1.000000000000000000, 0.9807852804032304306, 1.000000000000000000, 0.9807852804032304306, 1.000000000000000000, 0.9807852804032304306, 1.000000000000000000, 0.9807852804032304306, 1.000000000000000000, 0.9807852804032304306, 1.000000000000000000, 0.9807852804032304306, 1.000000000000000000, 0.9807852804032304306, 1.000000000000000000, 0.9807852804032304306, 1.000000000000000000, 0.9807852804032304306, 1.000000000000000000, 0.9807852804032304306, 1.000000000000000000, 0.9807852804032304306, 1.000000000000000000, 0.9807852804032304306, 1.000000000000000000, 0.9807852804032304306, 1.000000000000000000, 0.9807852804032304306, 1.000000000000000000, 0.9807852804032304306, 1.000000000000000000, 0.9807852804032304306, 1.000000000000000000, 0.9807852804032304306, 1.000000000000000000, 0.9807852804032304306, 1.000000000000000000, 0.9807852804032304306, 1.000000000000000000, 0.9807852804032304306, 1.000000000000000000, 0.9807852804032304306, 1.000000000000000000, 0.9807852804032304306, 1.000000000000000000, 0.9807852804032304306, 1.000000000000000000, 0.9807852804032304306, 1.000000000000000000, 0.9807852804032304306, 1.000000000000000000, 0.9807852804032304306, 1.000000000000000000, 0.9807852804032304306, 1.000000000000000000, 0.9807852804032304306, 1.000000000000000000, 0.9807852804032304306, 1.000000000000000000, 0.9807852804032304306, 1.000000000000000000, 0.9807852804032304306, 1.000000000000000000, 0.9807852804032304306, 1.000000000000000000, 0.9807852804032304306, 1.000000000000000000, 0.9807852804032304306, 1.000000000000000000, 0.9807852804032304306, 1.000000000000000000, 0.9807852804032304306, 1.000000000000000000, 0.9807852804032304306, 1.000000000000000000, 0.9807852804032304306, 1.000000000000000000, 0.9807852804032304306, 1.000000000000000000, 0.9807852804032304306, 1.000000000000000000, 0.9807852804032304306, 1.000000000000000000, 0.9807852804032304306, 1.000000000000000000, 0.9807852804032304306, 1.000000000000000000, 0.9807852804032304306, 1.000000000000000000, 0.9807852804032304306, 1.000000000000000000, 0.9807852804032304306, 1.000000000000000000, 0.9807852804032304306, 1.000000000000000000, 0.9807852804032304306, 1.000000000000000000, 0.9807852804032304306, 1.000000000000000000, 0.9807852804032304306, 1.000000000000000000, 0.9807852804032304306, 1.000000000000000000, 0.9807852804032304306, 1.000000000000000000, 0.9807852804032304306, 1.000000000000000000, 0.9807852804032304306, 1.000000000000000000, 0.9807852804032304306, 1.000000000000000000, 0.9807852804032304306, 1.000000000000000000, 0.9807852804032304306, 1.000000000000000000, 0.9807852804032304306, 1.000000000000000000, 0.9807852804032304306, 1.000000000000000000, 0.9807852804032304306, 1.000000000000000000, 0.9807852804032304306, 1.000000000000000000, 0.9807852804032304306, 1.000000000000000000, 0.9807852804032304306, 1.000000000000000000, 0.9807852804032304306, 1.000000000000000000, 0.9807852804032304306, 1.000000000000000000, 0.9807852804032304306, 1.000000000000000000, 0.9807852804032304306, 1.000000000000000000, 0.9807852804032304306, 1.000000000000000000, 0.9807852804032304306, 1.000000000000000000, 0.9807852804032304306, 1.000000000000000000, 0.9807852804032304306, 1.000000000000000000, 0.9807852804032304306, 1.000000000000000000, 0.9807852804032304306, 1.000000000000000000, 0.9807852804032304306, 1.000000000000000000, 0.9807852804032304306, 1.000000000000000000, 0.9807852804032304306, 1.000000000000000000, 0.9807852804032304306, 1.000000000000000000, 0.9807852804032304306, 1.000000000000000000, 0.9807852804032304306, 1.000000000000000000, 0.9807852804032304306, 1.000000000000000000, 0.9807852804032304306, 1.000000000000000000, 0.9807852804032304306, 1.000000000000000000, 0.9807852804032304306, 1.000000000000000000, 0.9807852804032304306, 1.000000000000000000, 0.9807852804032304306, 1.000000000000000000, 0.9807852804032304306, 1.000000000000000000, 0.9807852804032304306, 1.000000000000000000, 0.9807852804032304306, 1.000000000000000000, 0.9807852804032304306, 1.000000000000000000, 0.9807852804032304306, 1.000000000000000000, 0.9807852804032304306, 1.000000000000000000, 0.9807852804032304306, 1.000000000000000000, 0.9807852804032304306, 1.000000000000000000, 0.9807852804032304306, 1.000000000000000000, 0.9807852804032304306, 1.000000000000000000, 0.9807852804032304306, 1.000000000000000000, 0.9807852804032304306, 1.000000000000000000, 0.9807852804032304306, 1.000000000000000000, 0.9807852804032304306, 1.000000000000000000, 0.9807852804032304306, 1.000000000000000000, 0.9807852804032304306, 1.000000000000000000, 0.9807852804032304306, 1.000000000000000000, 0.9807852804032304306, 1.000000000000000000, 0.9807852804032304306, 1.000000000000000000, 0.9807852804032304306, 1.000000000000000000, 0.9807852804032304306, 1.000000000000000000, 0.9807852804032304306, 1.000000000000000000, 0.9807852804032304306, 1.000000000000000000, 0.9807852804032304306, 1.000000000000000000, 0.9807852804032304306, 1.000000000000000000, 0.9807852804032304306, 1.000000000000000000, 0.9807852804032304306, 1.000000000000000000, 0.9807852804032304306, 1.000000000000000000, 0.9807852804032304306, 1.000000000000000000, 0.9807852804032304306, 1.000000000000000000, 0.9807852804032304306, 1.000000000000000000, 0.9807852804032304306, 1.000000000000000000, 0.9807852804032304306, 1.000000000000000000, 0.9807852804032304306, 1.000000000000000000, 0.9807852804032304306, 1.000000000000000000, 0.9807852804032304306, 1.000000000000000000, 0.9807852804032304306, 1.000000000000000000, 0.9807852804032304306, 1.000000000000000000, 0.9807852804032304306, 1.000000000000000000, 0.9807852804032304306, 1.000000000000000000, 0.9807852804032304306, 1.000000000000000000, 0.9807852804032304306, 1.000000000000000000, 0.9807852804032304306, 1.000000000000000000, 0.9807852804032304306, 1.000000000000000000, 0.9807852804032304306, 1.000000000000000000, 0.9807852804032304306, 1.000000000000000000, 0.9807852804032304306, 1.000000000000000000, 0.9807852804032304306, 1.000000000000000000, 0.9807852804032304306, 1.000000000000000000, 0.9807852804032304306, 1.000000000000000000, 0.9807852804032304306, 1.000000000000000000, 0.9807852804032304306, 1.000000000000000000, 0.9807852804032304306, 1.000000000000000000, 0.9807852804032304306, 1.000000000000000000, 0.9807852804032304306, 1.000000000000000000, 0.9807852804032304306, 1.000000000000000000, 0.9807852804032304306, 1.000000000000000000, 0.9807852804032304306, 1.000000000000000000, 0.9807852804032304306, 1.000000000000000000, 0.9807852804032304306, 1.000000000000000000, 0.9807852804032304306, 1.000000000000000000, 0.9807852804032304306, 1.000000000000000000, 0.9807852804032304306, 1.000000000000000000, 0.9807852804032304306, 1.000000000000000000, 0.9807852804032304306, 1.000000000000000000, 0.9807852804032304306, 1.000000000000000000, 0.9807852804032304306, 1.000000000000000000, 0.9807852804032304306, 1.000000000000000000, 0.9807852804032304306, 1.000000000000000000, 0.9807852804032304306, 1.000000000000000000, 0.9807852804032304306, 1.000000000000000000, 0.9807852804032304306, 1.000000000000000000, 0.9807852804032304306, 1.000000000000000000, 0.9807852804032304306, 1.000000000000000000, 0.9807852804032304306, 1.000000000000000000, 0.9807852804032304306, 1.000000000000000000, 0.9807852804032304306, 1.000000000000000000, 0.9807852804032304306, 1.000000000000000000, 0.9807852804032304306, 1.000000000000000000, 0.9935443096272227326, 0.9914265371698519624) ) ) 
 REPRESENTATION_ITEM ( '' )  SURFACE ( )  );
#12618=CARTESIAN_POINT ( 'NONE',  ( -45.43829269268869098, 255.0573905683720000, -3.332260488124726194 ) ) ;
#12622=ORIENTED_EDGE ( 'NONE', *, *, #9889, .F. ) ;
#12623=CARTESIAN_POINT ( 'NONE',  ( -11.93348319268873325, 460.3698905683720000, -2.051577885510841163E-15 ) ) ;
#12626=CARTESIAN_POINT ( 'NONE',  ( -13.20868407381884779, 239.4948905683720284, -6.410867750099233042 ) ) ;
#12628=CARTESIAN_POINT ( 'NONE',  ( -16.84014894278201169, 520.1198905683720568, -11.84573899990672707 ) ) ;
#12631=CARTESIAN_POINT ( 'NONE',  ( -17.35679799567830273, 455.4323905765655809, 16.95518130045146421 ) ) ;
#12633=CARTESIAN_POINT ( 'NONE',  ( -8.685887942688802710, 286.6823905765655809, 3.978247347593374172 ) ) ;
#12634=CARTESIAN_POINT ( 'NONE',  ( -31.15659063867058265, 223.9102039777115749, -18.01685762724678597 ) ) ;
#12635=CARTESIAN_POINT ( 'NONE',  ( -11.93348319268870661, 230.6823905683720284, -3.332260488124732856 ) ) ;
#12637=CARTESIAN_POINT ( 'NONE',  ( -35.09675569278793716, 235.7448905683720000, 15.47720386886985366 ) ) ;
#12638=CARTESIAN_POINT ( 'NONE',  ( -14.48388495494899608, 331.3073905683720000, -9.489475012073736337 ) ) ;
#12641=CARTESIAN_POINT ( 'NONE',  ( -48.68588794268873698, 573.2448905601785327, 0.000000000000000000 ) ) ;
#12642=CARTESIAN_POINT ( 'NONE',  ( -44.16309181155855867, 305.9948905683720568, 6.410867750099241924 ) ) ;
#12643=CARTESIAN_POINT ( 'NONE',  ( -44.16309181155856578, 384.4948905683720000, 6.410867750099241924 ) ) ;
#12644=CARTESIAN_POINT ( 'NONE',  ( -16.84014894278201169, 531.6198905683720568, -11.84573899990672707 ) ) ;
#12645=CARTESIAN_POINT ( 'NONE',  ( -45.64106924314019409, 396.3073905601785327, -11.32908994701042715 ) ) ;
#12649=CARTESIAN_POINT ( 'NONE',  ( -13.20868407381887621, 509.7448905683720000, 6.410867750099229490 ) ) ;
#12651=CARTESIAN_POINT ( 'NONE',  ( -19.19641293061497578, 301.9323905683720000, -14.20200298773971603 ) ) ;
#12652=CARTESIAN_POINT ( 'NONE',  ( -11.93348319268871904, 329.1823905683720568, -3.332260488124732856 ) ) ;
#12653=CARTESIAN_POINT ( 'NONE',  ( -42.82802356641965247, 270.7448905765656377, -14.14213562373094746 ) ) ;
#12654=CARTESIAN_POINT ( 'NONE',  ( -42.82802356641967378, 500.7448905765656946, -14.14213562373094746 ) ) ;
#12655=CARTESIAN_POINT ( 'NONE',  ( -32.01814843081343298, 256.0573905683720000, 16.75240474999999307 ) ) ;
#12657=CARTESIAN_POINT ( 'NONE',  ( -13.20868407381886378, 399.7448905683720568, 6.410867750099229490 ) ) ;
#12665=CARTESIAN_POINT ( 'NONE',  ( -32.01814843081346140, 451.6823905683720568, -16.75240474999999307 ) ) ;
#12667=CARTESIAN_POINT ( 'NONE',  ( -48.68588794268871567, 436.9323905601784759, -3.978247347593158345 ) ) ;
#12671=DIRECTION ( 'NONE',  ( -1.191790137725560488E-16, 1.000000000000000000, -0.000000000000000000 ) ) ;
#12672=CARTESIAN_POINT ( 'NONE',  ( -8.685887942688717445, 331.9323905601784190, 3.978247347593161010 ) ) ;
#12673=CARTESIAN_POINT ( 'NONE',  ( -38.17536295476245556, 373.8073905683720568, -14.20200298773971426 ) ) ;
#12675=CARTESIAN_POINT ( 'NONE',  ( -13.68588794268873521, 548.2448905601784190, 1.836970198721029983E-15 ) ) ;
#12676=CARTESIAN_POINT ( 'NONE',  ( -8.685887942688738761, 506.9948905765655240, -2.449293598294705724E-15 ) ) ;
#12677=CARTESIAN_POINT ( 'NONE',  ( -19.19641293061498644, 387.3073905683720000, 14.20200298773971426 ) ) ;
#12678=CARTESIAN_POINT ( 'NONE',  ( -42.88789093042841927, 234.4323905683720284, -9.489475012073736337 ) ) ;
#12679=CARTESIAN_POINT ( 'NONE',  ( -11.93348319268872615, 398.8698905683720000, -2.051577885510841163E-15 ) ) ;
#12680=AXIS2_PLACEMENT_3D ( 'NONE', #4912, #65, #18105 ) ;
#12681=CARTESIAN_POINT ( 'NONE',  ( -36.33955658999050797, 313.8698905765656377, 18.47759065022572500 ) ) ;
#12683=CARTESIAN_POINT ( 'NONE',  ( -14.48388495494899431, 309.8073905683721136, -9.489475012073734561 ) ) ;
#12684=CARTESIAN_POINT ( 'NONE',  ( -11.93348319268873325, 460.3698905683720000, -2.051577885510841163E-15 ) ) ;
#12685=CARTESIAN_POINT ( 'NONE',  ( -21.03221929538692692, 515.1198905765656946, 18.47759065022572500 ) ) ;
#12686=CARTESIAN_POINT ( 'NONE',  ( -48.68588794268898567, 367.5573905601784759, 3.978247347592529071 ) ) ;
#12689=CARTESIAN_POINT ( 'NONE',  ( -22.27502019258947641, 358.4948905683720000, 15.47720386886985189 ) ) ;
#12690=CARTESIAN_POINT ( 'NONE',  ( -16.84014894278200458, 497.6198905683720000, 11.84573899990672530 ) ) ;
#12691=CARTESIAN_POINT ( 'NONE',  ( -24.70764059509556887, 500.0573905601786464, 19.99999999999998934 ) ) ;
#12692=CARTESIAN_POINT ( 'NONE',  ( -35.09675569278794427, 331.9948905683720000, -15.47720386886985544 ) ) ;
#12695=CARTESIAN_POINT ( 'NONE',  ( -11.73070664223723369, 261.3073905601784759, 11.32908994701042005 ) ) ;
#12700=CARTESIAN_POINT ( 'NONE',  ( -14.48388495494900852, 431.3073905683720000, -9.489475012073734561 ) ) ;
#12701=CARTESIAN_POINT ( 'NONE',  ( -14.54375231895777176, 395.7448905765656377, 14.14213562373094568 ) ) ;
#12703=CARTESIAN_POINT ( 'NONE',  ( -19.19641293061498999, 437.3073905683720000, 14.20200298773971426 ) ) ;
#12705=CARTESIAN_POINT ( 'NONE',  ( -19.19641293061499354, 460.4323905683721136, -14.20200298773971603 ) ) ;
#12707=CARTESIAN_POINT ( 'NONE',  ( -48.68588794268871567, 417.2448905601784759, 0.000000000000000000 ) ) ;
#12708=CARTESIAN_POINT ( 'NONE',  ( -45.64106924314019409, 392.9323905765656377, 11.32908994701042715 ) ) ;
#12709=CARTESIAN_POINT ( 'NONE',  ( -32.66413529028186247, 279.8073905765656377, -19.99999999999999289 ) ) ;
#12715=EDGE_CURVE ( 'NONE', #1587, #6189, #16775, .T. ) ;
#12716=CARTESIAN_POINT ( 'NONE',  ( -36.66917619319848853, 223.9102039777117170, 18.22452296251983483 ) ) ;
#12717=CARTESIAN_POINT ( 'NONE',  ( -36.33955658999050087, 239.1198905601784475, 18.47759065022572500 ) ) ;
#12718=CARTESIAN_POINT ( 'NONE',  ( -14.54375231895777709, 450.9948905601784759, 14.14213562373094568 ) ) ;
#12719=CARTESIAN_POINT ( 'NONE',  ( -44.16309181155857999, 424.7448905683720000, -6.410867750099231266 ) ) ;
#12720=CARTESIAN_POINT ( 'NONE',  ( -14.54375231895777176, 383.4948905601784759, -14.14213562373094746 ) ) ;
#12721=CARTESIAN_POINT ( 'NONE',  ( -25.35362745456396638, 248.1823905683720284, 16.75240474999998952 ) ) ;
#12725=CARTESIAN_POINT ( 'NONE',  ( -44.16309181155857999, 455.9948905683720000, 6.410867750099241924 ) ) ;
#12726=CARTESIAN_POINT ( 'NONE',  ( -36.33955658999050087, 223.8698905765656377, 18.47759065022572500 ) ) ;
#12730=CARTESIAN_POINT ( 'NONE',  ( -38.17536295476247687, 532.3073905683719431, -14.20200298773971426 ) ) ;
#12732=EDGE_CURVE ( 'NONE', #17801, #9678, #2982, .T. ) ;
#12733=CARTESIAN_POINT ( 'NONE',  ( -10.20829729246299777, 456.3698905765656377, 7.653668647301790529 ) ) ;
#12735=CARTESIAN_POINT ( 'NONE',  ( -28.68588794268874054, 573.2448905601785327, 0.000000000000000000 ) ) ;
#12737=CARTESIAN_POINT ( 'NONE',  ( -44.16309181155855157, 225.9948905683720284, 6.410867750099241924 ) ) ;
#12738=CARTESIAN_POINT ( 'NONE',  ( -29.56664704377478969, 223.9102039777116886, 20.04572207461867706 ) ) ;
#12739=CARTESIAN_POINT ( 'NONE',  ( -14.48388495494898187, 227.9323905683720000, 9.489475012073732785 ) ) ;
#12740=( BOUNDED_CURVE ( )  B_SPLINE_CURVE ( 2, ( #2161, #3356, #10042, #6798, #1853, #20114, #15366, #8422, #14935, #11676, #16981, #13310, #8527, #10250, #13631, #8744, #11779 ),
 .UNSPECIFIED., .F., .T. ) 
 B_SPLINE_CURVE_WITH_KNOTS ( ( 3, 2, 2, 2, 2, 2, 2, 2, 3 ),
 ( 0.5937500000000002220, 0.5957031250000002220, 0.5976562500000002220, 0.5996093750000002220, 0.6015625000000002220, 0.6035156250000002220, 0.6054687500000002220, 0.6074218750000002220, 0.6093750000000002220 ),
 .UNSPECIFIED. ) 
 CURVE ( )  GEOMETRIC_REPRESENTATION_ITEM ( )  RATIONAL_B_SPLINE_CURVE ( ( 0.9999999999999977796, 0.9807852804032326510, 1.000000000000000000, 0.9807852804032304306, 1.000000000000000000, 0.9807852804032304306, 1.000000000000000000, 0.9807852804032304306, 1.000000000000000000, 0.9807852804032304306, 1.000000000000000000, 0.9807852804032304306, 1.000000000000000000, 0.9807852804032304306, 1.000000000000000000, 0.9807852804032282101, 1.000000000000002220 ) ) 
 REPRESENTATION_ITEM ( '' )  );
#12741=CARTESIAN_POINT ( 'NONE',  ( -42.88789093042842637, 324.4323905683719431, -9.489475012073736337 ) ) ;
#12743=CARTESIAN_POINT ( 'NONE',  ( -47.16347859291444422, 377.8698905601784190, 7.653668647301805628 ) ) ;
#12744=CARTESIAN_POINT ( 'NONE',  ( -32.01814843081344009, 307.5573905683719431, 16.75240474999999307 ) ) ;
#12745=VECTOR ( 'NONE', #16598, 1000.000000000000000 ) ;
#12747=CARTESIAN_POINT ( 'NONE',  ( -28.68588794268871922, 391.3698905683720000, -16.75240474999999307 ) ) ;
#12748=CARTESIAN_POINT ( 'NONE',  ( -13.20868407381887977, 529.7448905683720568, 6.410867750099229490 ) ) ;
#12749=CARTESIAN_POINT ( 'NONE',  ( -40.01497788969913927, 375.6823905601784759, -16.95518130045146421 ) ) ;
#12751=CARTESIAN_POINT ( 'NONE',  ( -32.66413529028185536, 229.8073905765656377, -19.99999999999999289 ) ) ;
#12754=CARTESIAN_POINT ( 'NONE',  ( -11.93348319268873681, 490.0573905683720568, 3.332260488124728415 ) ) ;
#12758=CARTESIAN_POINT ( 'NONE',  ( -32.01814843081344009, 283.1823905683720000, -16.75240474999999307 ) ) ;
#12759=CARTESIAN_POINT ( 'NONE',  ( -25.35362745456397704, 326.6823905683720568, 16.75240474999998952 ) ) ;
#12760=CARTESIAN_POINT ( 'NONE',  ( -24.70764059509555111, 269.1823905765655809, -19.99999999999999289 ) ) ;
#12762=CARTESIAN_POINT ( 'NONE',  ( -38.17536295476243424, 235.4323905683720284, 14.20200298773971781 ) ) ;
#12763=CARTESIAN_POINT ( 'NONE',  ( -43.68588794268869435, 223.9102039777116602, 0.000000000000000000 ) ) ;
#12764=CARTESIAN_POINT ( 'NONE',  ( -42.88789093042843348, 384.4323905683720000, -9.489475012073736337 ) ) ;
#12769=CARTESIAN_POINT ( 'NONE',  ( -42.88789093042844058, 444.8073905683720568, 9.489475012073736337 ) ) ;
#12772=CARTESIAN_POINT ( 'NONE',  ( -24.70764059509557242, 444.4323905601784759, -19.99999999999999289 ) ) ;
#12775=ORIENTED_EDGE ( 'NONE', *, *, #11596, .T. ) ;
#12776=CARTESIAN_POINT ( 'NONE',  ( -8.685887942688722774, 356.9948905765655809, -2.449293598294705724E-15 ) ) ;
#12777=CARTESIAN_POINT ( 'NONE',  ( -36.33955658999050797, 335.3698905601784759, -18.47759065022572855 ) ) ;
#12778=CARTESIAN_POINT ( 'NONE',  ( -44.75779996082702894, 223.9102039777117170, -4.771598740727748478 ) ) ;
#12779=CARTESIAN_POINT ( 'NONE',  ( -32.01814843081344719, 373.1823905683720568, -16.75240474999999307 ) ) ;
#12781=CARTESIAN_POINT ( 'NONE',  ( -10.20829729246300310, 497.6198905765656377, -7.653668647301794969 ) ) ;
#12782=CARTESIAN_POINT ( 'NONE',  ( -11.93348319268872437, 388.8698905683720000, -2.051577885510841163E-15 ) ) ;
#12785=CARTESIAN_POINT ( 'NONE',  ( -19.19641293061498644, 400.4323905683720568, -14.20200298773971603 ) ) ;
#12786=CARTESIAN_POINT ( 'NONE',  ( -32.66413529028186957, 319.8073905765655809, -19.99999999999999289 ) ) ;
#12787=CARTESIAN_POINT ( 'NONE',  ( -21.03221929538693047, 424.1198905601784759, -18.47759065022572855 ) ) ;
#12788=CARTESIAN_POINT ( 'NONE',  ( -19.19641293061497223, 287.3073905683720000, 14.20200298773971426 ) ) ;
#12789=CARTESIAN_POINT ( 'NONE',  ( -13.20868407381887266, 460.9948905683720000, -6.410867750099233042 ) ) ;
#12793=EDGE_CURVE ( 'NONE', #1107, #11848, #54, .T. ) ;
#12794=AXIS2_PLACEMENT_3D ( 'NONE', #808, #2419, #696 ) ;
#12795=CARTESIAN_POINT ( 'NONE',  ( -25.35362745456399125, 372.5573905683720568, -16.75240474999999307 ) ) ;
#12796=CARTESIAN_POINT ( 'NONE',  ( -32.01814843081346851, 511.6823905683720000, -16.75240474999999307 ) ) ;
#12797=EDGE_CURVE ( 'NONE', #2613, #5272, #4333, .T. ) ;
#12798=CARTESIAN_POINT ( 'NONE',  ( -21.03221929538694113, 504.1198905601784759, -18.47759065022572855 ) ) ;
#12799=CARTESIAN_POINT ( 'NONE',  ( -19.19641293061498288, 330.4323905683720000, -14.20200298773971603 ) ) ;
#12800=EDGE_CURVE ( 'NONE', #5272, #15878, #21358, .T. ) ;
#12805=CARTESIAN_POINT ( 'NONE',  ( -11.93348319268872970, 430.6823905683721136, -3.332260488124732856 ) ) ;
#12806=CARTESIAN_POINT ( 'NONE',  ( -10.20829729246297291, 236.3698905765656093, 7.653668647301790529 ) ) ;
#12807=CYLINDRICAL_SURFACE ( 'NONE', #11430, 19.99999999999999645 ) ;
#12808=CARTESIAN_POINT ( 'NONE',  ( -32.01814843081345430, 436.0573905683720568, 16.75240474999999307 ) ) ;
#12811=CARTESIAN_POINT ( 'NONE',  ( -45.43829269268872650, 473.5573905683720568, -3.332260488124726638 ) ) ;
#12813=CARTESIAN_POINT ( 'NONE',  ( -42.82802356641966668, 415.9948905601785327, -14.14213562373094746 ) ) ;
#12815=CARTESIAN_POINT ( 'NONE',  ( -36.33955658999051508, 383.8698905765656377, 18.47759065022572500 ) ) ;
#12817=CARTESIAN_POINT ( 'NONE',  ( -36.33955658999050797, 370.1198905765656377, -18.47759065022572855 ) ) ;
#12819=CARTESIAN_POINT ( 'NONE',  ( -42.82802356641964536, 253.2448905765656377, 14.14213562373094923 ) ) ;
#12822=AXIS2_PLACEMENT_3D ( 'NONE', #9405, #14406, #6153 ) ;
#12824=CARTESIAN_POINT ( 'NONE',  ( -14.54375231895776821, 343.4948905601785327, -14.14213562373094746 ) ) ;
#12825=CARTESIAN_POINT ( 'NONE',  ( -45.43829269268871229, 425.0573905683720568, -3.332260488124726194 ) ) ;
#12827=CARTESIAN_POINT ( 'NONE',  ( -11.93348319268870839, 240.6823905683720284, -3.332260488124732856 ) ) ;
#12830=CARTESIAN_POINT ( 'NONE',  ( -42.82802356641966668, 423.2448905765656377, 14.14213562373094923 ) ) ;
#12832=CARTESIAN_POINT ( 'NONE',  ( -22.27502019258949773, 462.2448905683720568, -15.47720386886985544 ) ) ;
#12833=CARTESIAN_POINT ( 'NONE',  ( -47.16347859291443001, 222.6198905765656093, 7.653668647301805628 ) ) ;
#12836=CARTESIAN_POINT ( 'NONE',  ( -42.83993802355417557, 205.8067832142904479, 4.966639429937474759 ) ) ;
#12837=CARTESIAN_POINT ( 'NONE',  ( -22.27502019258950483, 532.2448905683720568, -15.47720386886985544 ) ) ;
#12839=CARTESIAN_POINT ( 'NONE',  ( -44.16309181155858710, 524.4948905683719431, 6.410867750099241924 ) ) ;
#12841=CARTESIAN_POINT ( 'NONE',  ( -24.70764059509556176, 434.8073905765656377, 19.99999999999998934 ) ) ;
#12842=CARTESIAN_POINT ( 'NONE',  ( -28.68588794268871212, 349.7448905601784759, 19.99999999999999289 ) ) ;
#12843=CARTESIAN_POINT ( 'NONE',  ( -48.68588794268872277, 451.9948905765656377, 0.000000000000000000 ) ) ;
#12844=CARTESIAN_POINT ( 'NONE',  ( -36.33955658999049376, 240.1198905765656377, -18.47759065022572855 ) ) ;
#12845=DIRECTION ( 'NONE',  ( 1.191790137725560488E-16, -1.000000000000000000, 0.000000000000000000 ) ) ;
#12847=CARTESIAN_POINT ( 'NONE',  ( -8.685887942688726326, 396.9948905765656377, -2.449293598294705724E-15 ) ) ;
#12848=CARTESIAN_POINT ( 'NONE',  ( -45.43829269268869808, 325.0573905683719431, -3.332260488124726194 ) ) ;
#12849=CARTESIAN_POINT ( 'NONE',  ( -48.68588794268871567, 447.2448905601785327, 0.000000000000000000 ) ) ;
#12853=CARTESIAN_POINT ( 'NONE',  ( -11.93348319268871549, 300.6823905683720568, -3.332260488124732856 ) ) ;
#12854=EDGE_CURVE ( 'NONE', #15132, #4208, #2260, .T. ) ;
#12855=CARTESIAN_POINT ( 'NONE',  ( -44.16309181155856578, 354.4948905683720000, 6.410867750099241924 ) ) ;
#12856=CARTESIAN_POINT ( 'NONE',  ( -44.16309181155859420, 524.7448905683720568, -6.410867750099231266 ) ) ;
#12857=CARTESIAN_POINT ( 'NONE',  ( -17.35679799567829917, 363.8073905601784759, -16.95518130045146421 ) ) ;
#12860=CARTESIAN_POINT ( 'NONE',  ( -40.53162694259545162, 494.1198905683720000, -11.84573899990672707 ) ) ;
#12862=CARTESIAN_POINT ( 'NONE',  ( -42.88789093042842637, 284.8073905683720568, 9.489475012073736337 ) ) ;
#12864=CARTESIAN_POINT ( 'NONE',  ( -13.20868407381885135, 280.9948905683720000, -6.410867750099233042 ) ) ;
#12865=CARTESIAN_POINT ( 'NONE',  ( -35.09675569278794427, 325.7448905683720000, 15.47720386886985366 ) ) ;
#12866=VECTOR ( 'NONE', #3775, 1000.000000000000000 ) ;
#12868=CARTESIAN_POINT ( 'NONE',  ( -17.35679799567827786, 255.4323905765656662, 16.95518130045146421 ) ) ;
#12870=CARTESIAN_POINT ( 'NONE',  ( -44.16309181155855157, 224.4948905683720284, 6.410867750099241924 ) ) ;
#12871=DIRECTION ( 'NONE',  ( -1.000000000000000000, 0.000000000000000000, 0.000000000000000000 ) ) ;
#12872=CARTESIAN_POINT ( 'NONE',  ( -44.16309181155856578, 385.9948905683720568, 6.410867750099241924 ) ) ;
#12880=CARTESIAN_POINT ( 'NONE',  ( -22.27502019258949773, 440.7448905683720000, -15.47720386886985544 ) ) ;
#12883=CARTESIAN_POINT ( 'NONE',  ( -40.01497788969914637, 425.6823905601784759, -16.95518130045146421 ) ) ;
#12886=ORIENTED_EDGE ( 'NONE', *, *, #5509, .F. ) ;
#12887=CARTESIAN_POINT ( 'NONE',  ( -10.20829729246298534, 356.3698905765655809, 7.653668647301790529 ) ) ;
#12888=CARTESIAN_POINT ( 'NONE',  ( -36.33955658999050797, 319.1198905601784759, 18.47759065022572500 ) ) ;
#12890=CARTESIAN_POINT ( 'NONE',  ( -19.19641293061497933, 341.9323905683721136, -14.20200298773971603 ) ) ;
#12891=CARTESIAN_POINT ( 'NONE',  ( -42.82802356641968089, 503.2448905765656377, 14.14213562373094923 ) ) ;
#12892=CARTESIAN_POINT ( 'NONE',  ( -11.93348319268872437, 389.1823905683721136, -3.332260488124732856 ) ) ;
#12894=VECTOR ( 'NONE', #21299, 1000.000000000000000 ) ;
#12895=CARTESIAN_POINT ( 'NONE',  ( -38.17536295476244845, 385.4323905683720568, 14.20200298773971781 ) ) ;
#12896=CARTESIAN_POINT ( 'NONE',  ( -10.20829729246298001, 317.6198905765655809, -7.653668647301794969 ) ) ;
#12898=CARTESIAN_POINT ( 'NONE',  ( -40.53162694259543031, 292.6198905683720000, -11.84573899990672707 ) ) ;
#12899=CARTESIAN_POINT ( 'NONE',  ( -35.09675569278795848, 447.2448905683720000, 15.47720386886985366 ) ) ;
#12903=CARTESIAN_POINT ( 'NONE',  ( -28.68588794268874054, 573.2448905601785327, 0.000000000000000000 ) ) ;
#12904=CARTESIAN_POINT ( 'NONE',  ( -13.20868407381885845, 350.9948905683720000, -6.410867750099233042 ) ) ;
#12905=CARTESIAN_POINT ( 'NONE',  ( -11.93348319268873858, 508.8698905683719431, -2.051577885510841163E-15 ) ) ;
#12907=CARTESIAN_POINT ( 'NONE',  ( -11.73070664223726567, 493.1823905601785327, -11.32908994701042715 ) ) ;
#12908=CARTESIAN_POINT ( 'NONE',  ( -16.84014894278198327, 317.6198905683720568, 11.84573899990672530 ) ) ;
#12909=ORIENTED_EDGE ( 'NONE', *, *, #2617, .F. ) ;
#12910=CARTESIAN_POINT ( 'NONE',  ( -40.01497788969911795, 258.8073905601784190, 16.95518130045146776 ) ) ;
#12911=ORIENTED_EDGE ( 'NONE', *, *, #13058, .T. ) ;
#12913=CARTESIAN_POINT ( 'NONE',  ( -44.16309181155857289, 405.9948905683720568, 6.410867750099241924 ) ) ;
#12914=CARTESIAN_POINT ( 'NONE',  ( -11.73070664223723192, 236.0573905765656093, 11.32908994701042005 ) ) ;
#12916=CARTESIAN_POINT ( 'NONE',  ( -16.84014894278199748, 447.6198905683720568, 11.84573899990672530 ) ) ;
#12917=ORIENTED_EDGE ( 'NONE', *, *, #14924, .T. ) ;
#12918=CARTESIAN_POINT ( 'NONE',  ( -32.01814843081345430, 456.0573905683720000, 16.75240474999999307 ) ) ;
#12921=CARTESIAN_POINT ( 'NONE',  ( -28.68588794268871922, 389.4948905765656377, -19.99999999999999289 ) ) ;
#12928=CARTESIAN_POINT ( 'NONE',  ( -11.93348319268873858, 500.0573905683720568, 3.332260488124728415 ) ) ;
#12930=CARTESIAN_POINT ( 'NONE',  ( -48.68588794268869435, 257.2448905601784759, 0.000000000000000000 ) ) ;
#12931=CARTESIAN_POINT ( 'NONE',  ( -8.685887942688818697, 421.9323905601785327, 3.978247347593374172 ) ) ;
#12932=( BOUNDED_CURVE ( )  B_SPLINE_CURVE ( 2, ( #3850, #18875, #15866, #5789, #6005, #7620, #8821, #7514, #10544, #13926, #13813, #2243, #18769, #3957, #17473, #7300, #17166 ),
 .UNSPECIFIED., .F., .T. ) 
 B_SPLINE_CURVE_WITH_KNOTS ( ( 3, 2, 2, 2, 2, 2, 2, 2, 3 ),
 ( 0.5156250000000002220, 0.5175781250000002220, 0.5195312500000002220, 0.5214843750000002220, 0.5234375000000002220, 0.5253906250000003331, 0.5273437500000003331, 0.5292968750000003331, 0.5312500000000003331 ),
 .UNSPECIFIED. ) 
 CURVE ( )  GEOMETRIC_REPRESENTATION_ITEM ( )  RATIONAL_B_SPLINE_CURVE ( ( 0.9999999999999977796, 0.9807852804032326510, 1.000000000000000000, 0.9807852804032304306, 1.000000000000000000, 0.9807852804032304306, 1.000000000000000000, 0.9807852804032304306, 1.000000000000000000, 0.9807852804032304306, 1.000000000000000000, 0.9807852804032304306, 1.000000000000000000, 0.9807852804032304306, 1.000000000000000000, 0.9807852804032270999, 1.000000000000003331 ) ) 
 REPRESENTATION_ITEM ( '' )  );
#12933=CARTESIAN_POINT ( 'NONE',  ( -19.19641293061498999, 408.8073905683720000, 14.20200298773971426 ) ) ;
#12934=CARTESIAN_POINT ( 'NONE',  ( -11.93348319268870661, 250.3698905683720000, -2.051577885510841163E-15 ) ) ;
#12939=ORIENTED_EDGE ( 'NONE', *, *, #12800, .F. ) ;
#12940=CARTESIAN_POINT ( 'NONE',  ( -45.43829269268872650, 455.3698905683720000, 0.000000000000000000 ) ) ;
#12941=CARTESIAN_POINT ( 'NONE',  ( -47.16347859291443001, 221.3698905765656377, -7.653668647301793193 ) ) ;
#12943=CARTESIAN_POINT ( 'NONE',  ( -42.99872675744465766, 207.3681867157733052, 4.490020761129740912 ) ) ;
#12944=CARTESIAN_POINT ( 'NONE',  ( -38.17536295476243424, 225.4323905683720000, 14.20200298773971781 ) ) ;
#12946=CARTESIAN_POINT ( 'NONE',  ( -44.16309181155859420, 513.2448905683719431, -6.410867750099231266 ) ) ;
#12948=CARTESIAN_POINT ( 'NONE',  ( -24.70764059509556176, 444.8073905765655809, 19.99999999999998934 ) ) ;
#12949=CARTESIAN_POINT ( 'NONE',  ( -48.68588794268853803, 301.6823905765655809, -3.978247347593583783 ) ) ;
#12950=CARTESIAN_POINT ( 'NONE',  ( -13.20868407381885667, 348.2448905683720000, 6.410867750099229490 ) ) ;
#12951=CARTESIAN_POINT ( 'NONE',  ( -17.35679799567828141, 238.5573905765656093, -16.95518130045146421 ) ) ;
#12952=CARTESIAN_POINT ( 'NONE',  ( -42.82802356641965247, 288.4948905601785327, 14.14213562373094923 ) ) ;
#12954=CARTESIAN_POINT ( 'NONE',  ( -45.43829269268869098, 224.1823905683720284, 3.332260488124734632 ) ) ;
#12955=CARTESIAN_POINT ( 'NONE',  ( -38.17536295476244135, 316.9323905683719431, 14.20200298773971781 ) ) ;
#12958=CARTESIAN_POINT ( 'NONE',  ( -19.19641293061497578, 298.8073905683719431, 14.20200298773971426 ) ) ;
#12959=CARTESIAN_POINT ( 'NONE',  ( -35.09675569278797269, 517.2448905683719431, 15.47720386886985366 ) ) ;
#12960=CARTESIAN_POINT ( 'NONE',  ( -40.01497788969913927, 365.6823905601784759, -16.95518130045146421 ) ) ;
#12961=CARTESIAN_POINT ( 'NONE',  ( -47.16347859291443001, 231.3698905765656093, -7.653668647301793193 ) ) ;
#12963=CARTESIAN_POINT ( 'NONE',  ( -25.35362745456400901, 492.5573905683721136, -16.75240474999999307 ) ) ;
#12965=CARTESIAN_POINT ( 'NONE',  ( -42.88789093042842637, 282.9323905683721136, -9.489475012073736337 ) ) ;
#12967=CARTESIAN_POINT ( 'NONE',  ( -42.88789093042842637, 286.3073905683720000, 9.489475012073734561 ) ) ;
#12968=CARTESIAN_POINT ( 'NONE',  ( -16.84014894278198327, 317.6198905683720568, 11.84573899990672530 ) ) ;
#12969=CARTESIAN_POINT ( 'NONE',  ( -42.88789093042841927, 266.3073905683720568, 9.489475012073734561 ) ) ;
#12970=CARTESIAN_POINT ( 'NONE',  ( -32.66413529028186247, 264.1823905765656377, 19.99999999999999289 ) ) ;
#12971=CARTESIAN_POINT ( 'NONE',  ( -11.73070664223726389, 473.1823905601784759, -11.32908994701042538 ) ) ;
#12972=CARTESIAN_POINT ( 'NONE',  ( -22.27502019258947286, 230.7448905683720000, -15.47720386886985544 ) ) ;
#12973=CARTESIAN_POINT ( 'NONE',  ( -32.01814843081344719, 387.5573905683719431, 16.75240474999999307 ) ) ;
#12975=CARTESIAN_POINT ( 'NONE',  ( -8.685887942688886199, 261.9323905601784759, 3.978247347593586447 ) ) ;
#12976=ADVANCED_FACE ( 'NONE', ( #13894 ), #20371, .T. ) ;
#12977=CARTESIAN_POINT ( 'NONE',  ( -11.73070664223723902, 267.9323905765656377, -11.32908994701042538 ) ) ;
#12978=CARTESIAN_POINT ( 'NONE',  ( -35.09675569278795138, 431.9948905683720568, -15.47720386886985544 ) ) ;
#12979=FACE_OUTER_BOUND ( 'NONE', #2811, .T. ) ;
#12980=ORIENTED_EDGE ( 'NONE', *, *, #8218, .T. ) ;
#12981=CARTESIAN_POINT ( 'NONE',  ( -48.68588794268871567, 416.9323905601784759, -3.978247347593158345 ) ) ;
#12986=CARTESIAN_POINT ( 'NONE',  ( -14.54375231895775933, 300.9948905601784759, 14.14213562373094568 ) ) ;
#12988=CARTESIAN_POINT ( 'NONE',  ( -28.68588794268871567, 352.8698905683720568, -16.75240474999999307 ) ) ;
#12989=CARTESIAN_POINT ( 'NONE',  ( -11.73070664223726745, 507.9323905765655809, -11.32908994701042715 ) ) ;
#12990=CARTESIAN_POINT ( 'NONE',  ( -14.48388495494900141, 387.9323905683720000, 9.489475012073732785 ) ) ;
#12991=CARTESIAN_POINT ( 'NONE',  ( -35.09675569278793006, 223.4948905683720284, -15.47720386886985544 ) ) ;
#12992=CARTESIAN_POINT ( 'NONE',  ( -13.20868407381886378, 389.4948905683720000, -6.410867750099233042 ) ) ;
#12995=CARTESIAN_POINT ( 'NONE',  ( -36.33955658999050797, 323.8698905765656377, 18.47759065022572500 ) ) ;
#12997=CARTESIAN_POINT ( 'NONE',  ( -19.19641293061496867, 277.3073905683720000, 14.20200298773971426 ) ) ;
#12999=CARTESIAN_POINT ( 'NONE',  ( -40.53162694259544452, 446.6198905683720568, 11.84573899990672885 ) ) ;
#13002=CARTESIAN_POINT ( 'NONE',  ( -21.03221929538692692, 500.3698905601785327, 18.47759065022572500 ) ) ;
#13003=LINE ( 'NONE', #8445, #12313 ) ;
#13004=CARTESIAN_POINT ( 'NONE',  ( -16.84014894278198682, 349.1198905683720568, 11.84573899990672530 ) ) ;
#13005=CARTESIAN_POINT ( 'NONE',  ( -45.43829269268871940, 474.1823905683720000, 3.332260488124734632 ) ) ;
#13006=CARTESIAN_POINT ( 'NONE',  ( -47.16347859291445843, 486.6198905601784759, -7.653668647301793193 ) ) ;
#13007=CARTESIAN_POINT ( 'NONE',  ( -11.93348319268871904, 329.1823905683720568, -3.332260488124732856 ) ) ;
#13008=EDGE_CURVE ( 'NONE', #19239, #16434, #8745, .T. ) ;
#13009=AXIS2_PLACEMENT_3D ( 'NONE', #21253, #21042, #3086 ) ;
#13010=ORIENTED_EDGE ( 'NONE', *, *, #1603, .T. ) ;
#13015=CARTESIAN_POINT ( 'NONE',  ( -14.48388495494900674, 409.4323905683720568, 9.489475012073731008 ) ) ;
#13018=CARTESIAN_POINT ( 'NONE',  ( -45.43829269268871229, 444.1823905683719431, 3.332260488124734632 ) ) ;
#13019=CARTESIAN_POINT ( 'NONE',  ( -45.43829269268872650, 454.1823905683720568, 3.332260488124734632 ) ) ;
#13020=DIRECTION ( 'NONE',  ( -1.191790137725560488E-16, 1.000000000000000000, -0.000000000000000000 ) ) ;
#13022=CARTESIAN_POINT ( 'NONE',  ( -8.685887942688722774, 376.6823905765656946, 3.978247347593161010 ) ) ;
#13024=CARTESIAN_POINT ( 'NONE',  ( -32.66413529028187668, 389.8073905765656377, -19.99999999999999289 ) ) ;
#13025=CARTESIAN_POINT ( 'NONE',  ( -17.35679799567830273, 428.5573905765656377, -16.95518130045146421 ) ) ;
#13026=CARTESIAN_POINT ( 'NONE',  ( -28.68588794268874054, 573.2448905601785327, 0.000000000000000000 ) ) ;
#13027=CARTESIAN_POINT ( 'NONE',  ( -11.93348319268873681, 490.6823905683720568, -3.332260488124732856 ) ) ;
#13034=CARTESIAN_POINT ( 'NONE',  ( -40.53162694259544452, 404.1198905683720000, -11.84573899990672707 ) ) ;
#13035=CARTESIAN_POINT ( 'NONE',  ( -8.685887942688729879, 436.9948905765656377, -2.449293598294705724E-15 ) ) ;
#13036=CARTESIAN_POINT ( 'NONE',  ( -35.09675569278793716, 237.2448905683720000, 15.47720386886985366 ) ) ;
#13038=CARTESIAN_POINT ( 'NONE',  ( -17.35679799567829562, 425.4323905765656377, 16.95518130045146421 ) ) ;
#13040=CARTESIAN_POINT ( 'NONE',  ( -25.35362745456400191, 462.5573905683720568, -16.75240474999999307 ) ) ;
#13041=CARTESIAN_POINT ( 'NONE',  ( -48.68588794268869435, 232.3073905765656377, 3.978247347593168115 ) ) ;
#13045=CARTESIAN_POINT ( 'NONE',  ( -25.35362745456397349, 221.0573905683720284, -16.75240474999999307 ) ) ;
#13047=CARTESIAN_POINT ( 'NONE',  ( -11.93348319268873858, 508.8698905683719431, -2.051577885510841163E-15 ) ) ;
#13049=CARTESIAN_POINT ( 'NONE',  ( -10.20829729246299600, 437.6198905765656377, -7.653668647301794969 ) ) ;
#13052=CARTESIAN_POINT ( 'NONE',  ( -8.685887942688708563, 246.9948905765656093, -2.449293598294705724E-15 ) ) ;
#13053=CARTESIAN_POINT ( 'NONE',  ( -10.20829729246299777, 456.3698905765656377, 7.653668647301790529 ) ) ;
#13057=( BOUNDED_CURVE ( )  B_SPLINE_CURVE ( 2, ( #13459, #3076, #11285, #17883, #16494, #8033, #5121, #13024, #9659, #14664, #1791, #21245, #169, #6410, #6739, #11721, #5228 ),
 .UNSPECIFIED., .F., .T. ) 
 B_SPLINE_CURVE_WITH_KNOTS ( ( 3, 2, 2, 2, 2, 2, 2, 2, 3 ),
 ( 0.4375000000000002220, 0.4394531250000002220, 0.4414062500000002220, 0.4433593750000002220, 0.4453125000000002220, 0.4472656250000002220, 0.4492187500000002220, 0.4511718750000002220, 0.4531250000000002220 ),
 .UNSPECIFIED. ) 
 CURVE ( )  GEOMETRIC_REPRESENTATION_ITEM ( )  RATIONAL_B_SPLINE_CURVE ( ( 0.9999999999999977796, 0.9807852804032326510, 1.000000000000000000, 0.9807852804032304306, 1.000000000000000000, 0.9807852804032304306, 1.000000000000000000, 0.9807852804032304306, 1.000000000000000000, 0.9807852804032304306, 1.000000000000000000, 0.9807852804032304306, 1.000000000000000000, 0.9807852804032304306, 1.000000000000000000, 0.9807852804032282101, 1.000000000000002220 ) ) 
 REPRESENTATION_ITEM ( '' )  );
#13058=EDGE_CURVE ( 'NONE', #8642, #6189, #9566, .T. ) ;
#13060=CARTESIAN_POINT ( 'NONE',  ( -8.915191811234558728, 223.9102039777117739, -3.487082981424983519 ) ) ;
#13061=CARTESIAN_POINT ( 'NONE',  ( -35.09675569278793716, 313.4948905683720000, -15.47720386886985544 ) ) ;
#13063=CARTESIAN_POINT ( 'NONE',  ( -10.20829729246297468, 261.6198905601784759, 7.653668647301790529 ) ) ;
#13064=CARTESIAN_POINT ( 'NONE',  ( -14.54375231895776821, 380.9948905601784759, 14.14213562373094568 ) ) ;
#13065=CARTESIAN_POINT ( 'NONE',  ( -32.01814843081344009, 293.1823905683720568, -16.75240474999999307 ) ) ;
#13067=CARTESIAN_POINT ( 'NONE',  ( -42.88789093042845479, 516.3073905683720568, 9.489475012073734561 ) ) ;
#13068=CARTESIAN_POINT ( 'NONE',  ( -32.66413529028187668, 359.4323905601784759, 19.99999999999999289 ) ) ;
#13070=CARTESIAN_POINT ( 'NONE',  ( -11.73070664223724613, 313.1823905601784190, -11.32908994701042538 ) ) ;
#13072=CARTESIAN_POINT ( 'NONE',  ( -38.17536295476246266, 496.9323905683720568, 14.20200298773971781 ) ) ;
#13074=CARTESIAN_POINT ( 'NONE',  ( -28.68588794268870501, 281.3698905683720000, -16.75240474999999307 ) ) ;
#13075=EDGE_LOOP ( 'NONE', ( #15978, #10628, #11866, #1631 ) ) ;
#13076=CARTESIAN_POINT ( 'NONE',  ( -40.53162694259543031, 276.6198905683720568, 11.84573899990672885 ) ) ;
#13077=CARTESIAN_POINT ( 'NONE',  ( -45.43829269268869808, 313.5573905683720000, -3.332260488124726194 ) ) ;
#13078=CARTESIAN_POINT ( 'NONE',  ( -13.20868407381884779, 259.7448905683720000, 6.410867750099229490 ) ) ;
#13080=CARTESIAN_POINT ( 'NONE',  ( -14.54375231895775222, 245.7448905765656093, 14.14213562373094568 ) ) ;
#13083=CARTESIAN_POINT ( 'NONE',  ( -19.19641293061498644, 378.8073905683721136, 14.20200298773971426 ) ) ;
#13084=CARTESIAN_POINT ( 'NONE',  ( -10.20829729246297646, 281.6198905601784759, 7.653668647301790529 ) ) ;
#13085=CARTESIAN_POINT ( 'NONE',  ( -42.82802356641967378, 460.7448905765655809, -14.14213562373094746 ) ) ;
#13086=CARTESIAN_POINT ( 'NONE',  ( -14.54375231895775933, 268.2448905765656377, -14.14213562373094746 ) ) ;
#13088=CARTESIAN_POINT ( 'NONE',  ( -16.84014894278199748, 420.1198905683720000, -11.84573899990672707 ) ) ;
#13092=CARTESIAN_POINT ( 'NONE',  ( -17.35679799567830628, 423.8073905601784759, -16.95518130045146421 ) ) ;
#13093=ORIENTED_EDGE ( 'NONE', *, *, #15327, .F. ) ;
#13096=EDGE_LOOP ( 'NONE', ( #850, #6533, #14086, #17409 ) ) ;
#13098=CARTESIAN_POINT ( 'NONE',  ( -48.68588794268870146, 297.5573905601785327, 3.978247347593168115 ) ) ;
#13100=CARTESIAN_POINT ( 'NONE',  ( -44.16309181155856578, 345.9948905683720000, 6.410867750099241924 ) ) ;
#13102=CARTESIAN_POINT ( 'NONE',  ( -42.82802356641967378, 490.7448905765656377, -14.14213562373094746 ) ) ;
#13103=CARTESIAN_POINT ( 'NONE',  ( -45.43829269268870519, 364.1823905683720568, 3.332260488124734632 ) ) ;
#13105=CARTESIAN_POINT ( 'NONE',  ( -35.09675569278794427, 381.9948905683720568, -15.47720386886985544 ) ) ;
#13107=CARTESIAN_POINT ( 'NONE',  ( -28.68588794268870856, 314.4948905765656377, 19.99999999999999289 ) ) ;
#13109=CARTESIAN_POINT ( 'NONE',  ( -45.43829269268870519, 294.1823905683720568, 3.332260488124734632 ) ) ;
#13111=CARTESIAN_POINT ( 'NONE',  ( -13.20868407381886911, 430.9948905683720568, -6.410867750099233042 ) ) ;
#13114=CARTESIAN_POINT ( 'NONE',  ( -48.68588794268869435, 227.2448905601785043, 0.000000000000000000 ) ) ;
#13116=CARTESIAN_POINT ( 'NONE',  ( -35.09675569278795138, 357.2448905683720000, 15.47720386886985366 ) ) ;
#13117=CARTESIAN_POINT ( 'NONE',  ( -25.35362745456400901, 491.0573905683720000, -16.75240474999999307 ) ) ;
#13119=CARTESIAN_POINT ( 'NONE',  ( -36.33955658999052218, 485.3698905601784759, -18.47759065022572855 ) ) ;
#13120=CARTESIAN_POINT ( 'NONE',  ( -40.53162694259543031, 305.1198905683720000, 11.84573899990672885 ) ) ;
#13121=AXIS2_PLACEMENT_3D ( 'NONE', #3027, #56, #20981 ) ;
#13124=CARTESIAN_POINT ( 'NONE',  ( -36.33955658999052929, 525.3698905601784190, -18.47759065022572855 ) ) ;
#13127=CARTESIAN_POINT ( 'NONE',  ( -25.35362745456398414, 398.1823905683720568, 16.75240474999998952 ) ) ;
#13129=( NAMED_UNIT ( * ) PLANE_ANGLE_UNIT ( ) SI_UNIT ( $, .RADIAN. ) );
#13130=CARTESIAN_POINT ( 'NONE',  ( -19.19641293061499354, 450.4323905683720000, -14.20200298773971603 ) ) ;
#13131=CARTESIAN_POINT ( 'NONE',  ( -13.20868407381887089, 439.4948905683720568, -6.410867750099233042 ) ) ;
#13133=CARTESIAN_POINT ( 'NONE',  ( -40.01497788969913927, 380.4323905765655240, -16.95518130045146421 ) ) ;
#13137=CARTESIAN_POINT ( 'NONE',  ( -8.685887942688736985, 486.9948905765656377, -2.449293598294705724E-15 ) ) ;
#13138=CARTESIAN_POINT ( 'NONE',  ( -13.20868407381887621, 490.9948905683720568, -6.410867750099233042 ) ) ;
#13143=CARTESIAN_POINT ( 'NONE',  ( -19.19641293061498999, 401.9323905683720000, -14.20200298773971603 ) ) ;
#13144=CARTESIAN_POINT ( 'NONE',  ( -10.20829729246299955, 467.6198905765656377, -7.653668647301794969 ) ) ;
#13146=CARTESIAN_POINT ( 'NONE',  ( -13.20868407381884424, 229.7448905683720568, 6.410867750099229490 ) ) ;
#13148=ORIENTED_EDGE ( 'NONE', *, *, #12393, .F. ) ;
#13151=CARTESIAN_POINT ( 'NONE',  ( -44.16309181155857999, 434.7448905683720000, -6.410867750099231266 ) ) ;
#13152=CARTESIAN_POINT ( 'NONE',  ( -21.03221929538689849, 235.1198905765656377, 18.47759065022572500 ) ) ;
#13156=CARTESIAN_POINT ( 'NONE',  ( -38.17536295476247687, 533.8073905683720568, -14.20200298773971426 ) ) ;
#13158=CARTESIAN_POINT ( 'NONE',  ( -45.43829269268873361, 513.5573905683720568, -3.332260488124726638 ) ) ;
#13161=CARTESIAN_POINT ( 'NONE',  ( -32.66413529028189089, 449.8073905765656946, -19.99999999999999289 ) ) ;
#13164=CARTESIAN_POINT ( 'NONE',  ( -10.20829729246298179, 331.6198905601784759, 7.653668647301790529 ) ) ;
#13167=CARTESIAN_POINT ( 'NONE',  ( -21.03221929538690915, 238.8698905765656093, -18.47759065022572855 ) ) ;
#13170=CARTESIAN_POINT ( 'NONE',  ( -18.66797547166049753, 223.9102039777116602, -17.31025331282116397 ) ) ;
#13171=CARTESIAN_POINT ( 'NONE',  ( -44.16309181155856578, 324.7448905683720000, -6.410867750099231266 ) ) ;
#13172=CARTESIAN_POINT ( 'NONE',  ( -47.16347859291443001, 236.6198905601784475, -7.653668647301793193 ) ) ;
#13173=PRODUCT_DEFINITION_FORMATION_WITH_SPECIFIED_SOURCE ( 'ANY', '', #15993, .NOT_KNOWN. ) ;
#13174=CARTESIAN_POINT ( 'NONE',  ( -10.20829729246297468, 262.8698905601785327, -7.653668647301794969 ) ) ;
#13176=CARTESIAN_POINT ( 'NONE',  ( -28.68588794268870501, 282.8698905683720568, -16.75240474999999307 ) ) ;
#13178=CARTESIAN_POINT ( 'NONE',  ( -28.68588794268873343, 512.8698905683719431, -16.75240474999999307 ) ) ;
#13179=CARTESIAN_POINT ( 'NONE',  ( -40.01497788969913216, 368.8073905601785327, 16.95518130045146776 ) ) ;
#13181=ORIENTED_EDGE ( 'NONE', *, *, #16163, .T. ) ;
#13182=CARTESIAN_POINT ( 'NONE',  ( -13.20868407381887444, 489.7448905683720568, 6.410867750099229490 ) ) ;
#13184=CARTESIAN_POINT ( 'NONE',  ( -38.17536295476244135, 275.4323905683720568, 14.20200298773971781 ) ) ;
#13186=( BOUNDED_CURVE ( )  B_SPLINE_CURVE ( 2, ( #20309, #8406, #8829, #13401, #7199, #19988, #15030, #15351, #11973, #16652, #5168, #13507, #1943, #16756, #18359, #3859, #8511 ),
 .UNSPECIFIED., .F., .T. ) 
 B_SPLINE_CURVE_WITH_KNOTS ( ( 3, 2, 2, 2, 2, 2, 2, 2, 3 ),
 ( 0.3750000000000001665, 0.3769531250000001665, 0.3789062500000001665, 0.3808593750000001665, 0.3828125000000001665, 0.3847656250000001665, 0.3867187500000001665, 0.3886718750000001665, 0.3906250000000001665 ),
 .UNSPECIFIED. ) 
 CURVE ( )  GEOMETRIC_REPRESENTATION_ITEM ( )  RATIONAL_B_SPLINE_CURVE ( ( 0.9999999999999983347, 0.9807852804032320959, 1.000000000000000000, 0.9807852804032304306, 1.000000000000000000, 0.9807852804032304306, 1.000000000000000000, 0.9807852804032304306, 1.000000000000000000, 0.9807852804032304306, 1.000000000000000000, 0.9807852804032304306, 1.000000000000000000, 0.9807852804032304306, 1.000000000000000000, 0.9807852804032287652, 1.000000000000001554 ) ) 
 REPRESENTATION_ITEM ( '' )  );
#13188=CARTESIAN_POINT ( 'NONE',  ( -40.53162694259543031, 274.1198905683720568, -11.84573899990672707 ) ) ;
#13189=CARTESIAN_POINT ( 'NONE',  ( -44.16309181155855867, 254.7448905683720284, -6.410867750099231266 ) ) ;
#13190=ADVANCED_FACE ( 'NONE', ( #17342 ), #21014, .T. ) ;
#13191=CARTESIAN_POINT ( 'NONE',  ( -11.73070664223723547, 247.9323905765656377, -11.32908994701042715 ) ) ;
#13192=CARTESIAN_POINT ( 'NONE',  ( -36.33955658999052218, 475.3698905601784759, -18.47759065022572855 ) ) ;
#13195=CARTESIAN_POINT ( 'NONE',  ( -19.19641293061497223, 267.3073905683720568, 14.20200298773971426 ) ) ;
#13197=CARTESIAN_POINT ( 'NONE',  ( -40.53162694259543741, 384.1198905683720568, -11.84573899990672707 ) ) ;
#13202=CARTESIAN_POINT ( 'NONE',  ( -45.43829269268871229, 413.5573905683720000, -3.332260488124726194 ) ) ;
#13205=CARTESIAN_POINT ( 'NONE',  ( -42.82802356641966668, 425.9948905601784759, -14.14213562373094746 ) ) ;
#13209=ORIENTED_EDGE ( 'NONE', *, *, #20244, .T. ) ;
#13210=ORIENTED_EDGE ( 'NONE', *, *, #9030, .T. ) ;
#13212=CARTESIAN_POINT ( 'NONE',  ( -47.16347859291443712, 306.6198905601784759, -7.653668647301793193 ) ) ;
#13214=CARTESIAN_POINT ( 'NONE',  ( -25.35362745456398059, 348.1823905683720000, 16.75240474999998952 ) ) ;
#13215=CARTESIAN_POINT ( 'NONE',  ( -21.03221929538694113, 488.8698905765655809, -18.47759065022572855 ) ) ;
#13216=CARTESIAN_POINT ( 'NONE',  ( -42.88789093042843348, 364.8073905683720568, 9.489475012073736337 ) ) ;
#13218=CARTESIAN_POINT ( 'NONE',  ( -19.19641293061498288, 387.3073905683720000, 14.20200298773971426 ) ) ;
#13219=CARTESIAN_POINT ( 'NONE',  ( -14.54375231895776288, 298.2448905765656377, -14.14213562373094746 ) ) ;
#13221=CARTESIAN_POINT ( 'NONE',  ( -28.68588794268870501, 281.3698905683720000, -16.75240474999999307 ) ) ;
#13222=DIRECTION ( 'NONE',  ( -1.191790137725560488E-16, 1.000000000000000000, -0.000000000000000000 ) ) ;
#13224=CARTESIAN_POINT ( 'NONE',  ( -19.19641293061498999, 428.8073905683720000, 14.20200298773971426 ) ) ;
#13226=DIRECTION ( 'NONE',  ( -1.000000000000000000, 0.000000000000000000, 0.000000000000000000 ) ) ;
#13227=CARTESIAN_POINT ( 'NONE',  ( -28.68588794268872277, 449.7448905601784759, 19.99999999999999289 ) ) ;
#13229=CARTESIAN_POINT ( 'NONE',  ( -25.35362745456398059, 358.1823905683720000, 16.75240474999998952 ) ) ;
#13230=CARTESIAN_POINT ( 'NONE',  ( -22.27502019258949062, 476.9948905683720000, 15.47720386886985189 ) ) ;
#13232=CARTESIAN_POINT ( 'NONE',  ( -40.01497788969915348, 485.6823905601785327, -16.95518130045146421 ) ) ;
#13233=CARTESIAN_POINT ( 'NONE',  ( -28.68588794268870501, 296.3698905683720568, 16.75240474999999307 ) ) ;
#13236=VERTEX_POINT ( 'NONE', #6075 ) ;
#13239=CARTESIAN_POINT ( 'NONE',  ( -44.16309181155857289, 395.9948905683720568, 6.410867750099241924 ) ) ;
#13240=CARTESIAN_POINT ( 'NONE',  ( -48.68588794268877251, 442.3073905765656377, 3.978247347593061978 ) ) ;
#13242=CARTESIAN_POINT ( 'NONE',  ( -35.09675569278795138, 431.9948905683720568, -15.47720386886985544 ) ) ;
#13243=CARTESIAN_POINT ( 'NONE',  ( -11.93348319268872970, 438.8698905683720568, -2.051577885510841163E-15 ) ) ;
#13245=CARTESIAN_POINT ( 'NONE',  ( -36.33955658999052218, 399.1198905601784759, 18.47759065022572500 ) ) ;
#13246=CARTESIAN_POINT ( 'NONE',  ( -47.16347859291444422, 371.3698905765655809, -7.653668647301793193 ) ) ;
#13247=DIRECTION ( 'NONE',  ( -1.000000000000000000, 0.000000000000000000, 0.000000000000000000 ) ) ;
#13248=CARTESIAN_POINT ( 'NONE',  ( -21.03221929538691271, 264.1198905601784759, -18.47759065022572855 ) ) ;
#13251=CARTESIAN_POINT ( 'NONE',  ( -38.17536295476246977, 493.8073905683720000, -14.20200298773971426 ) ) ;
#13257=CARTESIAN_POINT ( 'NONE',  ( -11.93348319268872615, 400.0573905683720568, 3.332260488124728415 ) ) ;
#13259=EDGE_CURVE ( 'NONE', #8266, #9067, #14328, .T. ) ;
#13260=CARTESIAN_POINT ( 'NONE',  ( -44.16309181155855867, 234.7448905683720000, -6.410867750099231266 ) ) ;
#13261=CARTESIAN_POINT ( 'NONE',  ( -45.43829269268871229, 353.8698905683720568, 0.000000000000000000 ) ) ;
#13263=CARTESIAN_POINT ( 'NONE',  ( -32.01814843081346851, 526.0573905683720568, 16.75240474999999307 ) ) ;
#13264=ORIENTED_EDGE ( 'NONE', *, *, #17251, .T. ) ;
#13265=CARTESIAN_POINT ( 'NONE',  ( -22.27502019258949773, 442.2448905683720000, -15.47720386886985544 ) ) ;
#13266=CARTESIAN_POINT ( 'NONE',  ( -14.48388495494901740, 519.8073905683720568, -9.489475012073736337 ) ) ;
#13267=VERTEX_POINT ( 'NONE', #9110 ) ;
#13268=CARTESIAN_POINT ( 'NONE',  ( -8.685887942688720997, 342.2448905601784759, -2.449293598294705724E-15 ) ) ;
#13269=CARTESIAN_POINT ( 'NONE',  ( -11.93348319268873681, 489.1823905683720568, -3.332260488124732856 ) ) ;
#13272=CARTESIAN_POINT ( 'NONE',  ( -11.93348319268873858, 498.5573905683720568, 3.332260488124728859 ) ) ;
#13273=CARTESIAN_POINT ( 'NONE',  ( -28.68588794268872633, 489.7448905601784759, 19.99999999999999289 ) ) ;
#13275=CARTESIAN_POINT ( 'NONE',  ( -40.01497788969914637, 453.5573905765656377, 16.95518130045146776 ) ) ;
#13283=CARTESIAN_POINT ( 'NONE',  ( -45.64106924314019409, 492.9323905765655809, 11.32908994701042538 ) ) ;
#13284=CARTESIAN_POINT ( 'NONE',  ( -35.09675569278794427, 307.2448905683720000, 15.47720386886985366 ) ) ;
#13285=CARTESIAN_POINT ( 'NONE',  ( -24.70764059509556887, 530.0573905601785327, 19.99999999999998934 ) ) ;
#13286=CARTESIAN_POINT ( 'NONE',  ( -24.70764059509553690, 270.0573905601784759, 19.99999999999998934 ) ) ;
#13287=CARTESIAN_POINT ( 'NONE',  ( -10.20829729246299244, 416.3698905765656377, 7.653668647301790529 ) ) ;
#13289=CARTESIAN_POINT ( 'NONE',  ( -19.19641293061497933, 291.9323905683720568, -14.20200298773971603 ) ) ;
#13290=CARTESIAN_POINT ( 'NONE',  ( -32.01814843081346140, 507.5573905683720000, 16.75240474999999307 ) ) ;
#13293=CARTESIAN_POINT ( 'NONE',  ( -32.01814843081346140, 467.5573905683721136, 16.75240474999999307 ) ) ;
#13295=CARTESIAN_POINT ( 'NONE',  ( -32.01814843081343298, 271.6823905683720000, -16.75240474999999307 ) ) ;
#13298=CARTESIAN_POINT ( 'NONE',  ( -32.01814843081343298, 273.1823905683720000, -16.75240474999999307 ) ) ;
#13299=CARTESIAN_POINT ( 'NONE',  ( -28.68588794268869790, 257.8698905683720000, 16.75240474999999307 ) ) ;
#13301=CARTESIAN_POINT ( 'NONE',  ( -28.68588794268870146, 249.4948905765656093, -19.99999999999999289 ) ) ;
#13303=CARTESIAN_POINT ( 'NONE',  ( -48.68588794268869435, 237.5573905601785043, 3.978247347593168115 ) ) ;
#13305=CARTESIAN_POINT ( 'NONE',  ( -32.01814843081344009, 276.0573905683720000, 16.75240474999999307 ) ) ;
#13306=CARTESIAN_POINT ( 'NONE',  ( -38.17536295476244845, 366.9323905683721136, 14.20200298773971781 ) ) ;
#13307=CARTESIAN_POINT ( 'NONE',  ( -40.01497788969912506, 278.8073905601785327, 16.95518130045146776 ) ) ;
#13308=CARTESIAN_POINT ( 'NONE',  ( -14.54375231895778242, 458.2448905765656377, -14.14213562373094746 ) ) ;
#13309=CARTESIAN_POINT ( 'NONE',  ( -44.16309181155857999, 423.2448905683720568, -6.410867750099231266 ) ) ;
#13310=CARTESIAN_POINT ( 'NONE',  ( -17.35679799567829207, 338.5573905765655809, -16.95518130045146421 ) ) ;
#13312=( BOUNDED_CURVE ( )  B_SPLINE_CURVE ( 2, ( #6330, #16621, #19964, #6862, #6647, #13481, #9997, #1811, #19854, #11632, #81, #403, #18227, #507, #20074, #8589, #5143 ),
 .UNSPECIFIED., .F., .T. ) 
 B_SPLINE_CURVE_WITH_KNOTS ( ( 3, 2, 2, 2, 2, 2, 2, 2, 3 ),
 ( 0.3281250000000001110, 0.3300781250000001110, 0.3320312500000001110, 0.3339843750000001110, 0.3359375000000001110, 0.3378906250000001110, 0.3398437500000001110, 0.3417968750000001110, 0.3437500000000001110 ),
 .UNSPECIFIED. ) 
 CURVE ( )  GEOMETRIC_REPRESENTATION_ITEM ( )  RATIONAL_B_SPLINE_CURVE ( ( 0.9999999999999988898, 0.9807852804032315408, 1.000000000000000000, 0.9807852804032304306, 1.000000000000000000, 0.9807852804032304306, 1.000000000000000000, 0.9807852804032304306, 1.000000000000000000, 0.9807852804032304306, 1.000000000000000000, 0.9807852804032304306, 1.000000000000000000, 0.9807852804032304306, 1.000000000000000000, 0.9807852804032293204, 1.000000000000001110 ) ) 
 REPRESENTATION_ITEM ( '' )  );
#13313=CARTESIAN_POINT ( 'NONE',  ( -36.33955658999052218, 419.1198905601784759, 18.47759065022572500 ) ) ;
#13318=CARTESIAN_POINT ( 'NONE',  ( -45.43829269268872650, 525.0573905683720568, -3.332260488124726194 ) ) ;
#13319=CARTESIAN_POINT ( 'NONE',  ( -32.66413529028186957, 315.0573905601784190, -19.99999999999999289 ) ) ;
#13321=CARTESIAN_POINT ( 'NONE',  ( -14.48388495494899786, 341.3073905683721136, -9.489475012073734561 ) ) ;
#13322=ORIENTED_EDGE ( 'NONE', *, *, #6364, .T. ) ;
#13323=CARTESIAN_POINT ( 'NONE',  ( -21.03221929538692336, 485.1198905765656377, 18.47759065022572500 ) ) ;
#13324=CARTESIAN_POINT ( 'NONE',  ( -22.27502019258947641, 366.9948905683720568, 15.47720386886985189 ) ) ;
#13326=CARTESIAN_POINT ( 'NONE',  ( -32.01814843081344719, 371.6823905683720000, -16.75240474999999307 ) ) ;
#13327=CARTESIAN_POINT ( 'NONE',  ( -10.20829729246297823, 306.3698905765655809, 7.653668647301790529 ) ) ;
#13329=CARTESIAN_POINT ( 'NONE',  ( -13.20868407381884779, 259.4948905683720568, -6.410867750099233042 ) ) ;
#13330=DIRECTION ( 'NONE',  ( -1.000000000000000000, 0.000000000000000000, 0.000000000000000000 ) ) ;
#13332=CARTESIAN_POINT ( 'NONE',  ( -44.16309181155857999, 444.7448905683720000, -6.410867750099231266 ) ) ;
#13333=ADVANCED_FACE ( 'NONE', ( #7904 ), #21116, .T. ) ;
#13338=CARTESIAN_POINT ( 'NONE',  ( -38.17536295476245556, 343.8073905683720000, -14.20200298773971426 ) ) ;
#13339=CARTESIAN_POINT ( 'NONE',  ( -22.27502019258949773, 480.7448905683720568, -15.47720386886985544 ) ) ;
#13340=ORIENTED_EDGE ( 'NONE', *, *, #5421, .F. ) ;
#13341=CARTESIAN_POINT ( 'NONE',  ( -8.685887942688736985, 492.2448905601785327, -2.449293598294705724E-15 ) ) ;
#13342=CARTESIAN_POINT ( 'NONE',  ( -32.01814843081344009, 306.0573905683720000, 16.75240474999999307 ) ) ;
#13346=CARTESIAN_POINT ( 'NONE',  ( -16.84014894278199748, 411.6198905683720568, -11.84573899990672707 ) ) ;
#13347=CARTESIAN_POINT ( 'NONE',  ( -40.01497788969913927, 375.6823905601784190, -16.95518130045146421 ) ) ;
#13348=CARTESIAN_POINT ( 'NONE',  ( -16.84014894278199748, 430.1198905683720000, -11.84573899990672707 ) ) ;
#13349=CARTESIAN_POINT ( 'NONE',  ( -38.17536295476244135, 263.8073905683720568, -14.20200298773971426 ) ) ;
#13350=CARTESIAN_POINT ( 'NONE',  ( -19.19641293061498999, 437.3073905683720568, 14.20200298773971426 ) ) ;
#13353=CARTESIAN_POINT ( 'NONE',  ( -8.685887942688724550, 366.9948905765655809, -2.449293598294705724E-15 ) ) ;
#13357=DIRECTION ( 'NONE',  ( -1.191790137725560488E-16, 1.000000000000000000, -0.000000000000000000 ) ) ;
#13358=CARTESIAN_POINT ( 'NONE',  ( -40.53162694259545873, 506.6198905683721136, 11.84573899990672885 ) ) ;
#13360=CARTESIAN_POINT ( 'NONE',  ( -21.03221929538693402, 464.1198905601784759, -18.47759065022572855 ) ) ;
#13362=VECTOR ( 'NONE', #16151, 1000.000000000000000 ) ;
#13363=CARTESIAN_POINT ( 'NONE',  ( -38.17536295476246266, 413.8073905683719431, -14.20200298773971426 ) ) ;
#13365=CARTESIAN_POINT ( 'NONE',  ( -13.20868407381884602, 230.9948905683720284, -6.410867750099233042 ) ) ;
#13366=CARTESIAN_POINT ( 'NONE',  ( -35.09675569278794427, 371.9948905683720568, -15.47720386886985544 ) ) ;
#13369=CARTESIAN_POINT ( 'NONE',  ( -22.27502019258949417, 516.9948905683720568, 15.47720386886985189 ) ) ;
#13371=CARTESIAN_POINT ( 'NONE',  ( -38.17536295476246266, 443.8073905683720568, -14.20200298773971426 ) ) ;
#13372=CARTESIAN_POINT ( 'NONE',  ( -28.68588794268872988, 516.3698905683720568, 16.75240474999999307 ) ) ;
#13374=CARTESIAN_POINT ( 'NONE',  ( -21.03221929538694468, 528.8698905765656946, -18.47759065022572855 ) ) ;
#13375=CARTESIAN_POINT ( 'NONE',  ( -28.68588794268873343, 491.3698905683720568, -16.75240474999999307 ) ) ;
#13377=CARTESIAN_POINT ( 'NONE',  ( -42.88789093042845479, 504.8073905683721136, 9.489475012073734561 ) ) ;
#13380=CARTESIAN_POINT ( 'NONE',  ( -48.68588794268871567, 421.9948905765656377, 0.000000000000000000 ) ) ;
#13381=CARTESIAN_POINT ( 'NONE',  ( -24.70764059509555821, 359.1823905765655809, -19.99999999999999289 ) ) ;
#13384=FACE_OUTER_BOUND ( 'NONE', #18187, .T. ) ;
#13389=CARTESIAN_POINT ( 'NONE',  ( -42.82802356641967378, 493.2448905765656377, 14.14213562373094923 ) ) ;
#13390=CARTESIAN_POINT ( 'NONE',  ( -13.20868407381884957, 289.7448905683720568, 6.410867750099229490 ) ) ;
#13391=CARTESIAN_POINT ( 'NONE',  ( -24.70764059509554755, 234.4323905601785043, -19.99999999999999289 ) ) ;
#13392=CARTESIAN_POINT ( 'NONE',  ( -11.73070664223723902, 273.1823905601784759, -11.32908994701042715 ) ) ;
#13394=CARTESIAN_POINT ( 'NONE',  ( -38.17536295476244845, 283.8073905683720568, -14.20200298773971426 ) ) ;
#13396=CARTESIAN_POINT ( 'NONE',  ( -14.54375231895779130, 533.4948905601785327, -14.14213562373094746 ) ) ;
#13397=CARTESIAN_POINT ( 'NONE',  ( -22.27502019258949417, 508.4948905683720568, 15.47720386886985189 ) ) ;
#13398=EDGE_CURVE ( 'NONE', #16131, #11348, #13003, .T. ) ;
#13399=ORIENTED_EDGE ( 'NONE', *, *, #16446, .T. ) ;
#13400=CARTESIAN_POINT ( 'NONE',  ( -44.16309181155857999, 465.9948905683720000, 6.410867750099241924 ) ) ;
#13401=CARTESIAN_POINT ( 'NONE',  ( -45.64106924314018698, 411.0573905765655809, -11.32908994701042538 ) ) ;
#13402=CARTESIAN_POINT ( 'NONE',  ( -42.88789093042841927, 262.9323905683720568, -9.489475012073736337 ) ) ;
#13405=CARTESIAN_POINT ( 'NONE',  ( -38.17536295476244135, 243.8073905683720284, -14.20200298773971426 ) ) ;
#13406=CARTESIAN_POINT ( 'NONE',  ( -17.35679799567827786, 245.4323905765656377, 16.95518130045146421 ) ) ;
#13407=CARTESIAN_POINT ( 'NONE',  ( -24.70764059509554045, 310.0573905601784759, 19.99999999999998934 ) ) ;
#13408=CARTESIAN_POINT ( 'NONE',  ( -48.68588794268869435, 236.9323905601785043, -3.978247347593158345 ) ) ;
#13409=CARTESIAN_POINT ( 'NONE',  ( -40.53162694259542320, 265.1198905683720568, 11.84573899990672885 ) ) ;
#13410=CARTESIAN_POINT ( 'NONE',  ( -13.20868407381885667, 349.7448905683720568, 6.410867750099229490 ) ) ;
#13412=CARTESIAN_POINT ( 'NONE',  ( -28.68588794268870146, 279.7448905601784759, 19.99999999999999289 ) ) ;
#13414=CARTESIAN_POINT ( 'NONE',  ( -35.09675569278795848, 415.7448905683720000, 15.47720386886985366 ) ) ;
#13417=CARTESIAN_POINT ( 'NONE',  ( -24.70764059509555466, 400.0573905601784759, 19.99999999999998934 ) ) ;
#13418=ADVANCED_FACE ( 'NONE', ( #9745 ), #8335, .T. ) ;
#13421=VERTEX_POINT ( 'NONE', #9960 ) ;
#13422=CARTESIAN_POINT ( 'NONE',  ( -13.20868407381888154, 530.9948905683720568, -6.410867750099233042 ) ) ;
#13423=CARTESIAN_POINT ( 'NONE',  ( -14.54375231895776110, 293.4948905601785327, -14.14213562373094746 ) ) ;
#13425=CARTESIAN_POINT ( 'NONE',  ( -13.20868407381885490, 320.9948905683720568, -6.410867750099233042 ) ) ;
#13426=ORIENTED_EDGE ( 'NONE', *, *, #6635, .F. ) ;
#13427=CARTESIAN_POINT ( 'NONE',  ( -45.43829269268870519, 373.5573905683720568, -3.332260488124726194 ) ) ;
#13428=CARTESIAN_POINT ( 'NONE',  ( -35.09675569278795138, 375.7448905683720000, 15.47720386886985366 ) ) ;
#13429=CARTESIAN_POINT ( 'NONE',  ( -21.03221929538690205, 305.1198905765656377, 18.47759065022572500 ) ) ;
#13430=DIRECTION ( 'NONE',  ( -1.000000000000000000, -0.000000000000000000, -0.000000000000000000 ) ) ;
#13431=CARTESIAN_POINT ( 'NONE',  ( -38.17536295476243424, 265.4323905683721136, 14.20200298773971781 ) ) ;
#13432=CARTESIAN_POINT ( 'NONE',  ( -11.73070664223725501, 441.3073905601785327, 11.32908994701042005 ) ) ;
#13433=CARTESIAN_POINT ( 'NONE',  ( -32.01814843081345430, 423.1823905683720568, -16.75240474999999307 ) ) ;
#13436=CARTESIAN_POINT ( 'NONE',  ( -17.35679799567830628, 500.6823905601784759, 16.95518130045146421 ) ) ;
#13437=CARTESIAN_POINT ( 'NONE',  ( -24.70764059509554755, 360.0573905601785327, 19.99999999999998934 ) ) ;
#13438=CARTESIAN_POINT ( 'NONE',  ( -48.68588794268871567, 407.2448905601784759, 0.000000000000000000 ) ) ;
#13439=CARTESIAN_POINT ( 'NONE',  ( -16.84014894278198327, 319.1198905683720568, 11.84573899990672530 ) ) ;
#13440=CARTESIAN_POINT ( 'NONE',  ( -11.93348319268873681, 488.5573905683720568, 3.332260488124728415 ) ) ;
#13441=EDGE_LOOP ( 'NONE', ( #15154, #2220, #10768, #4552 ) ) ;
#13442=CARTESIAN_POINT ( 'NONE',  ( -28.68588794268872988, 464.7448905601784759, -19.99999999999999289 ) ) ;
#13443=CARTESIAN_POINT ( 'NONE',  ( -42.88789093042842637, 312.9323905683720000, -9.489475012073736337 ) ) ;
#13444=ORIENTED_EDGE ( 'NONE', *, *, #7360, .F. ) ;
#13448=AXIS2_PLACEMENT_3D ( 'NONE', #1350, #16173, #9658 ) ;
#13449=CARTESIAN_POINT ( 'NONE',  ( -11.93348319268872437, 390.3698905683720568, -2.051577885510841163E-15 ) ) ;
#13450=CARTESIAN_POINT ( 'NONE',  ( -14.54375231895778064, 480.9948905601784759, 14.14213562373094568 ) ) ;
#13452=CARTESIAN_POINT ( 'NONE',  ( -11.93348319268872970, 428.5573905683720568, 3.332260488124728415 ) ) ;
#13453=CARTESIAN_POINT ( 'NONE',  ( -14.48388495494898542, 251.3073905683720284, -9.489475012073736337 ) ) ;
#13454=CARTESIAN_POINT ( 'NONE',  ( -13.20868407381886556, 418.2448905683720568, 6.410867750099229490 ) ) ;
#13456=DIRECTION ( 'NONE',  ( -1.191790137725560488E-16, 1.000000000000000000, -0.000000000000000000 ) ) ;
#13457=CARTESIAN_POINT ( 'NONE',  ( -14.54375231895776999, 358.2448905765656377, -14.14213562373094746 ) ) ;
#13459=CARTESIAN_POINT ( 'NONE',  ( -48.68588794268871567, 391.9948905765656377, 0.000000000000000000 ) ) ;
#13460=CARTESIAN_POINT ( 'NONE',  ( -22.27502019258947286, 326.9948905683720000, 15.47720386886985189 ) ) ;
#13462=CARTESIAN_POINT ( 'NONE',  ( -19.19641293061499709, 481.9323905683720000, -14.20200298773971603 ) ) ;
#13464=CARTESIAN_POINT ( 'NONE',  ( -36.33955658999052218, 433.8698905765655809, 18.47759065022572500 ) ) ;
#13465=CARTESIAN_POINT ( 'NONE',  ( -8.685887942688742314, 573.2448905601785327, 2.449293598294706119E-15 ) ) ;
#13466=CARTESIAN_POINT ( 'NONE',  ( -32.66413529028187668, 419.4323905601784190, 19.99999999999999289 ) ) ;
#13467=EDGE_CURVE ( 'NONE', #2613, #15821, #4993, .T. ) ;
#13470=CARTESIAN_POINT ( 'NONE',  ( -44.16309181155856578, 385.9948905683720568, 6.410867750099241924 ) ) ;
#13472=CARTESIAN_POINT ( 'NONE',  ( -32.01814843081343298, 223.1823905683720000, -16.75240474999999307 ) ) ;
#13473=CARTESIAN_POINT ( 'NONE',  ( -28.68588794268871212, 366.3698905683720568, 16.75240474999999307 ) ) ;
#13475=CARTESIAN_POINT ( 'NONE',  ( -45.43829269268873361, 533.8698905683720568, 0.000000000000000000 ) ) ;
#13477=CARTESIAN_POINT ( 'NONE',  ( -16.84014894278199748, 449.1198905683720568, 11.84573899990672530 ) ) ;
#13478=CARTESIAN_POINT ( 'NONE',  ( -25.35362745456399836, 516.6823905683720568, 16.75240474999998952 ) ) ;
#13481=CARTESIAN_POINT ( 'NONE',  ( -17.35679799567829562, 430.6823905601785327, 16.95518130045146421 ) ) ;
#13482=CARTESIAN_POINT ( 'NONE',  ( -38.17536295476246977, 482.3073905683720568, -14.20200298773971426 ) ) ;
#13484=CARTESIAN_POINT ( 'NONE',  ( -38.17536295476246266, 495.4323905683719431, 14.20200298773971781 ) ) ;
#13485=CARTESIAN_POINT ( 'NONE',  ( -48.68588794268882936, 487.5573905601784190, 3.978247347592901217 ) ) ;
#13486=CARTESIAN_POINT ( 'NONE',  ( -10.20829729246299422, 426.3698905765656377, 7.653668647301790529 ) ) ;
#13488=CARTESIAN_POINT ( 'NONE',  ( -17.35679799567828141, 248.5573905765656093, -16.95518130045146421 ) ) ;
#13489=CARTESIAN_POINT ( 'NONE',  ( -48.68588794268871567, 407.2448905601784759, 0.000000000000000000 ) ) ;
#13492=FACE_OUTER_BOUND ( 'NONE', #8634, .T. ) ;
#13493=CARTESIAN_POINT ( 'NONE',  ( -43.63268616469407846, 200.3053519615658615, -1.302651870180923099 ) ) ;
#13496=CARTESIAN_POINT ( 'NONE',  ( -38.17536295476244135, 296.9323905683720000, 14.20200298773971781 ) ) ;
#13497=CARTESIAN_POINT ( 'NONE',  ( -28.68588794268873343, 529.7448905601785327, 19.99999999999999289 ) ) ;
#13498=CARTESIAN_POINT ( 'NONE',  ( -48.68588794268869435, 267.2448905601784759, 0.000000000000000000 ) ) ;
#13500=CARTESIAN_POINT ( 'NONE',  ( -11.93348319268871371, 290.0573905683720000, 3.332260488124728415 ) ) ;
#13503=CARTESIAN_POINT ( 'NONE',  ( -45.43829269268872650, 495.6823905683720568, 3.332260488124734632 ) ) ;
#13506=CARTESIAN_POINT ( 'NONE',  ( -45.43829269268871940, 465.6823905683720000, 3.332260488124734632 ) ) ;
#13507=CARTESIAN_POINT ( 'NONE',  ( -17.35679799567830273, 408.5573905765656377, -16.95518130045146421 ) ) ;
#13508=CARTESIAN_POINT ( 'NONE',  ( -22.27502019258946575, 266.9948905683720000, 15.47720386886985189 ) ) ;
#13511=CARTESIAN_POINT ( 'NONE',  ( -48.68588794268870856, 331.9948905765656377, 0.000000000000000000 ) ) ;
#13512=CARTESIAN_POINT ( 'NONE',  ( -45.43829269268869808, 245.0573905683720000, -3.332260488124726638 ) ) ;
#13513=AXIS2_PLACEMENT_3D ( 'NONE', #5591, #20739, #7527 ) ;
#13514=CARTESIAN_POINT ( 'NONE',  ( -28.68588794268870146, 239.4948905765656377, -19.99999999999999289 ) ) ;
#13516=CARTESIAN_POINT ( 'NONE',  ( -48.68588794268870856, 367.2448905601784759, 0.000000000000000000 ) ) ;
#13517=CARTESIAN_POINT ( 'NONE',  ( -19.81321358049341086, 224.0162454934389586, -17.97266195050653437 ) ) ;
#13518=CARTESIAN_POINT ( 'NONE',  ( -19.19641293061497223, 277.3073905683720000, 14.20200298773971426 ) ) ;
#13519=CARTESIAN_POINT ( 'NONE',  ( -22.27502019258947641, 348.4948905683720000, 15.47720386886985189 ) ) ;
#13521=LINE ( 'NONE', #3561, #9244 ) ;
#13522=VECTOR ( 'NONE', #1681, 1000.000000000000000 ) ;
#13523=CARTESIAN_POINT ( 'NONE',  ( -11.93348319268872615, 399.1823905683720568, -3.332260488124732856 ) ) ;
#13524=CARTESIAN_POINT ( 'NONE',  ( -45.64106924314020119, 508.1823905601784190, 11.32908994701042538 ) ) ;
#13526=CIRCLE ( 'NONE', #5222, 15.00000000000000000 ) ;
#13527=CARTESIAN_POINT ( 'NONE',  ( -32.66413529028188378, 405.0573905601784759, -19.99999999999999289 ) ) ;
#13528=EDGE_LOOP ( 'NONE', ( #9365, #13264 ) ) ;
#13531=VERTEX_POINT ( 'NONE', #9641 ) ;
#13532=CARTESIAN_POINT ( 'NONE',  ( -44.16309181155859420, 524.7448905683720568, -6.410867750099231266 ) ) ;
#13533=CARTESIAN_POINT ( 'NONE',  ( -8.685887942688713892, 282.5573905601784759, -3.978247347593165895 ) ) ;
#13534=CARTESIAN_POINT ( 'NONE',  ( -43.68320130047528238, 210.1357463702879613, -0.3279153920022768731 ) ) ;
#13536=ADVANCED_FACE ( 'NONE', ( #1766 ), #4672, .T. ) ;
#13537=CARTESIAN_POINT ( 'NONE',  ( -32.01814843081344009, 327.5573905683720568, 16.75240474999999307 ) ) ;
#13539=CARTESIAN_POINT ( 'NONE',  ( -42.88789093042843348, 372.9323905683720568, -9.489475012073736337 ) ) ;
#13540=CARTESIAN_POINT ( 'NONE',  ( -35.09675569278794427, 371.9948905683720568, -15.47720386886985544 ) ) ;
#13541=CARTESIAN_POINT ( 'NONE',  ( -21.03221929538691626, 308.8698905765655809, -18.47759065022572855 ) ) ;
#13542=CARTESIAN_POINT ( 'NONE',  ( -8.685887942688740537, 516.9948905765655809, -2.449293598294705724E-15 ) ) ;
#13543=CARTESIAN_POINT ( 'NONE',  ( -44.16309181155855867, 274.4948905683720000, 6.410867750099241924 ) ) ;
#13545=CARTESIAN_POINT ( 'NONE',  ( -35.09675569278795848, 427.2448905683720568, 15.47720386886985366 ) ) ;
#13549=CARTESIAN_POINT ( 'NONE',  ( -45.64106924314019409, 451.0573905765656377, -11.32908994701042538 ) ) ;
#13550=CARTESIAN_POINT ( 'NONE',  ( -17.35679799567827786, 275.4323905765655809, 16.95518130045146421 ) ) ;
#13552=CARTESIAN_POINT ( 'NONE',  ( -28.68588794268870856, 337.8698905683720000, 16.75240474999999307 ) ) ;
#13553=CARTESIAN_POINT ( 'NONE',  ( -16.84014894278199748, 457.6198905683720568, 11.84573899990672530 ) ) ;
#13556=CARTESIAN_POINT ( 'NONE',  ( -48.68588794268872277, 467.5573905601785327, 3.978247347593168115 ) ) ;
#13557=CARTESIAN_POINT ( 'NONE',  ( -44.16309181155855867, 294.4948905683720000, 6.410867750099241924 ) ) ;
#13560=VERTEX_POINT ( 'NONE', #13114 ) ;
#13561=DIRECTION ( 'NONE',  ( -1.191790137725560488E-16, 1.000000000000000000, -0.000000000000000000 ) ) ;
#13563=CARTESIAN_POINT ( 'NONE',  ( -11.93348319268872260, 380.0573905683720568, 3.332260488124728859 ) ) ;
#13566=CARTESIAN_POINT ( 'NONE',  ( -32.01814843081345430, 426.0573905683720568, 16.75240474999999307 ) ) ;
#13567=CARTESIAN_POINT ( 'NONE',  ( -44.16309181155855867, 264.7448905683720000, -6.410867750099231266 ) ) ;
#13568=CARTESIAN_POINT ( 'NONE',  ( -45.43829269268871940, 433.8698905683720568, 0.000000000000000000 ) ) ;
#13569=CARTESIAN_POINT ( 'NONE',  ( -48.68588794268871567, 397.2448905601784759, 0.000000000000000000 ) ) ;
#13570=CARTESIAN_POINT ( 'NONE',  ( -40.01497788969913216, 363.5573905765656377, 16.95518130045146776 ) ) ;
#13572=CARTESIAN_POINT ( 'NONE',  ( -45.43829269268870519, 323.8698905683720000, 0.000000000000000000 ) ) ;
#13573=LINE ( 'NONE', #14878, #6219 ) ;
#13575=( BOUNDED_CURVE ( )  B_SPLINE_CURVE ( 2, ( #20390, #12603, #19195, #13912, #15644, #4050, #829, #612, #2229, #2333, #20501, #17152, #7177, #935, #14124, #14235, #2543 ),
 .UNSPECIFIED., .F., .T. ) 
 B_SPLINE_CURVE_WITH_KNOTS ( ( 3, 2, 2, 2, 2, 2, 2, 2, 3 ),
 ( 0.8906250000000002220, 0.8925781250000002220, 0.8945312500000002220, 0.8964843750000002220, 0.8984375000000002220, 0.9003906250000001110, 0.9023437500000001110, 0.9042968750000001110, 0.9062500000000001110 ),
 .UNSPECIFIED. ) 
 CURVE ( )  GEOMETRIC_REPRESENTATION_ITEM ( )  RATIONAL_B_SPLINE_CURVE ( ( 0.9999999999999977796, 0.9807852804032326510, 1.000000000000000000, 0.9807852804032304306, 1.000000000000000000, 0.9807852804032304306, 1.000000000000000000, 0.9807852804032304306, 1.000000000000000000, 0.9807852804032304306, 1.000000000000000000, 0.9807852804032304306, 1.000000000000000000, 0.9807852804032304306, 1.000000000000000000, 0.9807852804032293204, 1.000000000000001110 ) ) 
 REPRESENTATION_ITEM ( '' )  );
#13576=CARTESIAN_POINT ( 'NONE',  ( -16.84014894278200103, 469.1198905683720568, 11.84573899990672530 ) ) ;
#13579=CARTESIAN_POINT ( 'NONE',  ( -17.35679799567828852, 303.8073905601784759, -16.95518130045146421 ) ) ;
#13580=CARTESIAN_POINT ( 'NONE',  ( -32.01814843081344719, 383.1823905683720568, -16.75240474999999307 ) ) ;
#13581=CARTESIAN_POINT ( 'NONE',  ( -48.68588794268858777, 471.6823905765655240, -3.978247347593477201 ) ) ;
#13583=CARTESIAN_POINT ( 'NONE',  ( -47.16347859291446554, 527.8698905601784190, 7.653668647301805628 ) ) ;
#13584=CARTESIAN_POINT ( 'NONE',  ( -45.43829269268870519, 363.5573905683720568, -3.332260488124726194 ) ) ;
#13586=CARTESIAN_POINT ( 'NONE',  ( -19.19641293061500420, 530.4323905683720568, -14.20200298773971603 ) ) ;
#13587=VERTEX_POINT ( 'NONE', #16472 ) ;
#13588=CARTESIAN_POINT ( 'NONE',  ( -36.33955658999050797, 355.3698905601784759, -18.47759065022572855 ) ) ;
#13589=CARTESIAN_POINT ( 'NONE',  ( -28.68588794268873343, 526.3698905683720568, 16.75240474999999307 ) ) ;
#13590=ORIENTED_EDGE ( 'NONE', *, *, #248, .T. ) ;
#13591=CARTESIAN_POINT ( 'NONE',  ( -40.01497788969916058, 530.4323905765655809, -16.95518130045146421 ) ) ;
#13592=CARTESIAN_POINT ( 'NONE',  ( -13.20868407381887266, 478.2448905683720568, 6.410867750099229490 ) ) ;
#13594=CARTESIAN_POINT ( 'NONE',  ( -45.43829269268872650, 484.1823905683720568, 3.332260488124734632 ) ) ;
#13595=CARTESIAN_POINT ( 'NONE',  ( -40.01497788969914637, 488.8073905601784759, 16.95518130045146776 ) ) ;
#13596=CARTESIAN_POINT ( 'NONE',  ( -24.70764059509555821, 424.8073905765656377, 19.99999999999998934 ) ) ;
#13597=CARTESIAN_POINT ( 'NONE',  ( -24.70764059509556176, 474.8073905765655809, 19.99999999999998934 ) ) ;
#13598=CARTESIAN_POINT ( 'NONE',  ( -48.68588794268879383, 297.5573905601784759, 3.978247347592954952 ) ) ;
#13599=CARTESIAN_POINT ( 'NONE',  ( -17.35679799567830628, 438.5573905765655809, -16.95518130045146421 ) ) ;
#13603=CARTESIAN_POINT ( 'NONE',  ( -16.84014894278197971, 299.1198905683720000, 11.84573899990672530 ) ) ;
#13604=EDGE_CURVE ( 'NONE', #19032, #2991, #3641, .T. ) ;
#13606=CARTESIAN_POINT ( 'NONE',  ( -11.93348319268872970, 440.6823905683721136, -3.332260488124732856 ) ) ;
#13608=CARTESIAN_POINT ( 'NONE',  ( -42.88789093042841927, 264.4323905683720568, -9.489475012073736337 ) ) ;
#13609=CIRCLE ( 'NONE', #10817, 5.000000000000001776 ) ;
#13612=CARTESIAN_POINT ( 'NONE',  ( -11.93348319268873858, 500.3698905683720000, -2.051577885510841163E-15 ) ) ;
#13615=CARTESIAN_POINT ( 'NONE',  ( -16.84014894278200458, 471.6198905683720000, -11.84573899990672707 ) ) ;
#13616=FACE_OUTER_BOUND ( 'NONE', #10158, .T. ) ;
#13617=CARTESIAN_POINT ( 'NONE',  ( -38.17536295476243424, 255.4323905683720284, 14.20200298773971781 ) ) ;
#13619=CARTESIAN_POINT ( 'NONE',  ( -10.20829729246298356, 336.3698905765656377, 7.653668647301790529 ) ) ;
#13621=CARTESIAN_POINT ( 'NONE',  ( -25.35362745456397704, 242.5573905683720000, -16.75240474999999307 ) ) ;
#13623=CARTESIAN_POINT ( 'NONE',  ( -40.01497788969912506, 225.6823905601784759, -16.95518130045146421 ) ) ;
#13625=CARTESIAN_POINT ( 'NONE',  ( -45.43829269268869808, 274.1823905683720000, 3.332260488124734632 ) ) ;
#13627=CARTESIAN_POINT ( 'NONE',  ( -44.16309181155857289, 354.7448905683720568, -6.410867750099231266 ) ) ;
#13629=( BOUNDED_CURVE ( )  B_SPLINE_CURVE ( 2, ( #3843, #2127, #20604, #13803, #5779, #12384, #5569, #9024, #515, #7291, #6976, #18977, #7076, #4158, #20505, #13598, #18761 ),
 .UNSPECIFIED., .F., .T. ) 
 B_SPLINE_CURVE_WITH_KNOTS ( ( 3, 2, 2, 2, 2, 2, 2, 2, 3 ),
 ( 0.7343750000000003331, 0.7363281250000003331, 0.7382812500000002220, 0.7402343750000002220, 0.7421875000000002220, 0.7441406250000002220, 0.7460937500000002220, 0.7480468750000001110, 0.7500000000000001110 ),
 .UNSPECIFIED. ) 
 CURVE ( )  GEOMETRIC_REPRESENTATION_ITEM ( )  RATIONAL_B_SPLINE_CURVE ( ( 0.9999999999999966693, 0.9807852804032337612, 1.000000000000000000, 0.9807852804032304306, 1.000000000000000000, 0.9807852804032304306, 1.000000000000000000, 0.9807852804032304306, 1.000000000000000000, 0.9807852804032304306, 1.000000000000000000, 0.9807852804032304306, 1.000000000000000000, 0.9807852804032304306, 1.000000000000000000, 0.9807852804032293204, 1.000000000000001110 ) ) 
 REPRESENTATION_ITEM ( '' )  );
#13630=CARTESIAN_POINT ( 'NONE',  ( -19.19641293061498999, 407.3073905683720000, 14.20200298773971426 ) ) ;
#13631=CARTESIAN_POINT ( 'NONE',  ( -10.20829729246298356, 337.6198905765656377, -7.653668647301794969 ) ) ;
#13632=CARTESIAN_POINT ( 'NONE',  ( -47.16347859291445133, 406.6198905601784759, -7.653668647301793193 ) ) ;
#13635=VERTEX_POINT ( 'NONE', #8655 ) ;
#13637=CARTESIAN_POINT ( 'NONE',  ( -19.19641293061499709, 518.8073905683720568, 14.20200298773971426 ) ) ;
#13638=CARTESIAN_POINT ( 'NONE',  ( -11.73070664223723725, 291.3073905601784759, 11.32908994701042005 ) ) ;
#13640=ORIENTED_EDGE ( 'NONE', *, *, #6166, .F. ) ;
#13641=CARTESIAN_POINT ( 'NONE',  ( -45.43829269268870519, 315.3698905683720568, 0.000000000000000000 ) ) ;
#13642=EDGE_LOOP ( 'NONE', ( #19391, #5589, #1633, #12512 ) ) ;
#13643=CARTESIAN_POINT ( 'NONE',  ( -45.43829269268871229, 343.8698905683720000, 0.000000000000000000 ) ) ;
#13644=CARTESIAN_POINT ( 'NONE',  ( -14.48388495494899786, 357.9323905683720000, 9.489475012073731008 ) ) ;
#13645=CARTESIAN_POINT ( 'NONE',  ( -36.33955658999050087, 310.1198905765656377, -18.47759065022572855 ) ) ;
#13647=EDGE_CURVE ( 'NONE', #1235, #12168, #6662, .T. ) ;
#13648=CARTESIAN_POINT ( 'NONE',  ( -28.68588794268870501, 271.3698905683720000, -16.75240474999999307 ) ) ;
#13649=CARTESIAN_POINT ( 'NONE',  ( -43.47668584505345990, 200.8081422174835780, 2.511554223531089036 ) ) ;
#13650=CARTESIAN_POINT ( 'NONE',  ( -45.43829269268871229, 415.6823905683721136, 3.332260488124734632 ) ) ;
#13652=CARTESIAN_POINT ( 'NONE',  ( -32.66413529028189089, 504.1823905765656377, 19.99999999999999289 ) ) ;
#13654=CARTESIAN_POINT ( 'NONE',  ( -38.17536295476244845, 336.9323905683720568, 14.20200298773971781 ) ) ;
#13655=CARTESIAN_POINT ( 'NONE',  ( -45.43829269268871940, 463.5573905683720568, -3.332260488124726194 ) ) ;
#13656=ORIENTED_EDGE ( 'NONE', *, *, #13998, .F. ) ;
#13657=CARTESIAN_POINT ( 'NONE',  ( -32.66413529028189089, 469.4323905601784759, 19.99999999999999289 ) ) ;
#13658=CARTESIAN_POINT ( 'NONE',  ( -11.93348319268871016, 278.8698905683720000, -2.051577885510841163E-15 ) ) ;
#13662=CARTESIAN_POINT ( 'NONE',  ( -24.70764059509554755, 340.0573905601784759, 19.99999999999998934 ) ) ;
#13663=CARTESIAN_POINT ( 'NONE',  ( -35.09675569278793716, 301.9948905683720568, -15.47720386886985544 ) ) ;
#13664=EDGE_CURVE ( 'NONE', #9092, #349, #8869, .T. ) ;
#13665=CARTESIAN_POINT ( 'NONE',  ( -19.19641293061498644, 381.9323905683720000, -14.20200298773971603 ) ) ;
#13666=CARTESIAN_POINT ( 'NONE',  ( -17.35679799567827430, 230.6823905601784759, 16.95518130045146421 ) ) ;
#13668=CARTESIAN_POINT ( 'NONE',  ( -11.93348319268872793, 418.8698905683720568, -2.051577885510841163E-15 ) ) ;
#13669=CARTESIAN_POINT ( 'NONE',  ( -11.93348319268871194, 270.6823905683719431, -3.332260488124732856 ) ) ;
#13670=CARTESIAN_POINT ( 'NONE',  ( -45.43829269268871940, 434.1823905683721136, 3.332260488124734632 ) ) ;
#13672=CARTESIAN_POINT ( 'NONE',  ( -28.68588794268871212, 364.4948905765656377, 19.99999999999999289 ) ) ;
#13673=CARTESIAN_POINT ( 'NONE',  ( -13.20868407381885490, 319.4948905683720000, -6.410867750099233042 ) ) ;
#13674=CARTESIAN_POINT ( 'NONE',  ( -11.93348319268873503, 470.0573905683720568, 3.332260488124728415 ) ) ;
#13677=CARTESIAN_POINT ( 'NONE',  ( -48.68588794268853803, 306.9323905601784759, -3.978247347593583783 ) ) ;
#13679=CARTESIAN_POINT ( 'NONE',  ( -28.68588794268871922, 382.8698905683720000, -16.75240474999999307 ) ) ;
#13680=LINE ( 'NONE', #16929, #7482 ) ;
#13681=CARTESIAN_POINT ( 'NONE',  ( -28.68588794268873698, 534.7448905601785327, -19.99999999999999289 ) ) ;
#13682=CARTESIAN_POINT ( 'NONE',  ( -25.35362745456398059, 346.6823905683720568, 16.75240474999998952 ) ) ;
#13684=CARTESIAN_POINT ( 'NONE',  ( -13.20868407381887977, 528.2448905683720568, 6.410867750099229490 ) ) ;
#13686=CARTESIAN_POINT ( 'NONE',  ( -13.20868407381887977, 519.4948905683720568, -6.410867750099233042 ) ) ;
#13688=EDGE_CURVE ( 'NONE', #11055, #232, #5839, .T. ) ;
#13690=CARTESIAN_POINT ( 'NONE',  ( -11.73070664223727100, 527.9323905765655809, -11.32908994701042538 ) ) ;
#13691=CARTESIAN_POINT ( 'NONE',  ( -40.53162694259545162, 482.6198905683720000, -11.84573899990672707 ) ) ;
#13693=CARTESIAN_POINT ( 'NONE',  ( -32.01814843081345430, 486.0573905683721136, 16.75240474999999307 ) ) ;
#13694=CARTESIAN_POINT ( 'NONE',  ( -32.66413529028188378, 489.4323905601784759, 19.99999999999999289 ) ) ;
#13695=CARTESIAN_POINT ( 'NONE',  ( -8.685887942688728103, 416.9948905765656377, -2.449293598294705724E-15 ) ) ;
#13701=CARTESIAN_POINT ( 'NONE',  ( -48.68588794268873698, 548.2448905601784190, 0.000000000000000000 ) ) ;
#13704=CARTESIAN_POINT ( 'NONE',  ( -14.48388495494899253, 301.3073905683720568, -9.489475012073736337 ) ) ;
#13707=CARTESIAN_POINT ( 'NONE',  ( -25.35362745456400191, 442.5573905683720568, -16.75240474999999307 ) ) ;
#13708=CARTESIAN_POINT ( 'NONE',  ( -32.66413529028187668, 399.8073905765656377, -19.99999999999999289 ) ) ;
#13709=CARTESIAN_POINT ( 'NONE',  ( -40.53162694259543031, 274.1198905683720568, -11.84573899990672707 ) ) ;
#13710=VERTEX_POINT ( 'NONE', #18029 ) ;
#13712=CARTESIAN_POINT ( 'NONE',  ( -11.93348319268873681, 490.6823905683720568, -3.332260488124732856 ) ) ;
#13715=CARTESIAN_POINT ( 'NONE',  ( -32.01814843081346140, 473.1823905683720000, -16.75240474999999307 ) ) ;
#13716=CYLINDRICAL_SURFACE ( 'NONE', #10371, 19.99999999999999645 ) ;
#13717=CARTESIAN_POINT ( 'NONE',  ( -32.01814843081343298, 251.6823905683720568, -16.75240474999999307 ) ) ;
#13720=CARTESIAN_POINT ( 'NONE',  ( -28.68588794268874054, 573.2448905601785327, 0.000000000000000000 ) ) ;
#13723=CARTESIAN_POINT ( 'NONE',  ( -14.54375231895778064, 475.7448905765655809, 14.14213562373094568 ) ) ;
#13724=CARTESIAN_POINT ( 'NONE',  ( -28.68588794268871567, 389.7448905601785327, 19.99999999999999289 ) ) ;
#13725=CARTESIAN_POINT ( 'NONE',  ( -16.84014894278197261, 249.1198905683720284, 11.84573899990672530 ) ) ;
#13726=CARTESIAN_POINT ( 'NONE',  ( -28.68588794268872277, 419.4948905765656377, -19.99999999999999289 ) ) ;
#13727=CARTESIAN_POINT ( 'NONE',  ( -32.66413529028186247, 235.0573905601785043, -19.99999999999999289 ) ) ;
#13728=CARTESIAN_POINT ( 'NONE',  ( -28.68588794268869790, 256.3698905683720000, 16.75240474999999307 ) ) ;
#13729=CARTESIAN_POINT ( 'NONE',  ( -25.35362745456398059, 358.1823905683720000, 16.75240474999998952 ) ) ;
#13731=CIRCLE ( 'NONE', #7502, 15.00000000000000000 ) ;
#13736=VECTOR ( 'NONE', #10274, 1000.000000000000000 ) ;
#13737=CARTESIAN_POINT ( 'NONE',  ( -28.68588794268871567, 396.3698905683720000, 16.75240474999999307 ) ) ;
#13738=CARTESIAN_POINT ( 'NONE',  ( -32.66413529028189089, 509.4323905601784190, 19.99999999999999289 ) ) ;
#13739=CARTESIAN_POINT ( 'NONE',  ( -40.01497788969913927, 408.8073905601784759, 16.95518130045146776 ) ) ;
#13741=DIRECTION ( 'NONE',  ( -1.000000000000000000, 0.000000000000000000, 0.000000000000000000 ) ) ;
#13743=ORIENTED_EDGE ( 'NONE', *, *, #13688, .T. ) ;
#13744=CARTESIAN_POINT ( 'NONE',  ( -38.17536295476246977, 526.9323905683719431, 14.20200298773971781 ) ) ;
#13745=CARTESIAN_POINT ( 'NONE',  ( -42.82802356641965247, 285.9948905601784759, -14.14213562373094746 ) ) ;
#13748=CARTESIAN_POINT ( 'NONE',  ( -19.19641293061497578, 318.8073905683720568, 14.20200298773971426 ) ) ;
#13750=CARTESIAN_POINT ( 'NONE',  ( -25.35362745456399125, 351.0573905683720568, -16.75240474999999307 ) ) ;
#13751=CARTESIAN_POINT ( 'NONE',  ( -25.35362745456398059, 356.6823905683720568, 16.75240474999998952 ) ) ;
#13752=CARTESIAN_POINT ( 'NONE',  ( -28.68588794268870501, 279.4948905765656377, -19.99999999999999289 ) ) ;
#13754=CARTESIAN_POINT ( 'NONE',  ( -40.53162694259543031, 275.1198905683720568, 11.84573899990672885 ) ) ;
#13756=( BOUNDED_CURVE ( )  B_SPLINE_CURVE ( 2, ( #14351, #4591, #2767, #9557, #14454, #21247, #19618, #7824, #16176, #3188, #1249, #7926, #12819, #19410, #17885, #11185, #17787 ),
 .UNSPECIFIED., .F., .T. ) 
 B_SPLINE_CURVE_WITH_KNOTS ( ( 3, 2, 2, 2, 2, 2, 2, 2, 3 ),
 ( 0.8593750000000002220, 0.8613281250000002220, 0.8632812500000002220, 0.8652343750000002220, 0.8671875000000002220, 0.8691406250000002220, 0.8710937500000002220, 0.8730468750000002220, 0.8750000000000002220 ),
 .UNSPECIFIED. ) 
 CURVE ( )  GEOMETRIC_REPRESENTATION_ITEM ( )  RATIONAL_B_SPLINE_CURVE ( ( 0.9999999999999977796, 0.9807852804032326510, 1.000000000000000000, 0.9807852804032304306, 1.000000000000000000, 0.9807852804032304306, 1.000000000000000000, 0.9807852804032304306, 1.000000000000000000, 0.9807852804032304306, 1.000000000000000000, 0.9807852804032304306, 1.000000000000000000, 0.9807852804032304306, 1.000000000000000000, 0.9807852804032282101, 1.000000000000002220 ) ) 
 REPRESENTATION_ITEM ( '' )  );
#13757=CARTESIAN_POINT ( 'NONE',  ( -19.19641293061498999, 408.8073905683720000, 14.20200298773971426 ) ) ;
#13758=LINE ( 'NONE', #18290, #14096 ) ;
#13759=CARTESIAN_POINT ( 'NONE',  ( -48.68588794268872277, 501.9948905765656377, 0.000000000000000000 ) ) ;
#13760=CARTESIAN_POINT ( 'NONE',  ( -8.685887942688726326, 412.2448905601784759, -2.449293598294705724E-15 ) ) ;
#13761=CARTESIAN_POINT ( 'NONE',  ( -14.48388495494899431, 329.4323905683720568, 9.489475012073732785 ) ) ;
#13762=CARTESIAN_POINT ( 'NONE',  ( -22.27502019258948707, 456.9948905683720000, 15.47720386886985189 ) ) ;
#13764=CARTESIAN_POINT ( 'NONE',  ( -8.685887942688736985, 472.5573905601784759, -3.978247347593165895 ) ) ;
#13765=CARTESIAN_POINT ( 'NONE',  ( -16.84014894278198327, 290.1198905683720568, -11.84573899990672707 ) ) ;
#13768=CARTESIAN_POINT ( 'NONE',  ( -48.68588794268870856, 337.5573905601784759, 3.978247347593168115 ) ) ;
#13769=CARTESIAN_POINT ( 'NONE',  ( -42.88789093042842637, 292.9323905683720568, -9.489475012073736337 ) ) ;
#13770=CARTESIAN_POINT ( 'NONE',  ( -45.43829269268871229, 375.0573905683720000, -3.332260488124726638 ) ) ;
#13771=CARTESIAN_POINT ( 'NONE',  ( -17.35679799567831694, 528.5573905765656946, -16.95518130045146421 ) ) ;
#13772=CARTESIAN_POINT ( 'NONE',  ( -44.16309181155857999, 413.2448905683720568, -6.410867750099231266 ) ) ;
#13773=CARTESIAN_POINT ( 'NONE',  ( -13.20868407381884779, 259.7448905683720000, 6.410867750099229490 ) ) ;
#13774=CARTESIAN_POINT ( 'NONE',  ( -32.01814843081344719, 426.0573905683720568, 16.75240474999999307 ) ) ;
#13776=AXIS2_PLACEMENT_3D ( 'NONE', #11979, #9049, #11581 ) ;
#13777=CARTESIAN_POINT ( 'NONE',  ( -32.66413529028187668, 334.1823905765656377, 19.99999999999999289 ) ) ;
#13778=CARTESIAN_POINT ( 'NONE',  ( -21.03221929538691271, 274.1198905601784759, -18.47759065022572855 ) ) ;
#13779=CARTESIAN_POINT ( 'NONE',  ( -25.35362745456398770, 331.0573905683720000, -16.75240474999999307 ) ) ;
#13780=CARTESIAN_POINT ( 'NONE',  ( -38.17536295476246266, 476.9323905683720568, 14.20200298773971781 ) ) ;
#13784=EDGE_CURVE ( 'NONE', #18441, #339, #20862, .T. ) ;
#13785=CARTESIAN_POINT ( 'NONE',  ( -13.20868407381886023, 379.7448905683720000, 6.410867750099229490 ) ) ;
#13787=CARTESIAN_POINT ( 'NONE',  ( -10.20829729246300488, 521.6198905601785327, 7.653668647301790529 ) ) ;
#13788=CARTESIAN_POINT ( 'NONE',  ( -19.19641293061498288, 347.3073905683720568, 14.20200298773971426 ) ) ;
#13791=CARTESIAN_POINT ( 'NONE',  ( -25.35362745456400901, 501.0573905683720568, -16.75240474999999307 ) ) ;
#13794=CARTESIAN_POINT ( 'NONE',  ( -28.68588794268870856, 314.7448905601785327, -19.99999999999999289 ) ) ;
#13795=DIRECTION ( 'NONE',  ( 1.191790137725560488E-16, -1.000000000000000000, 0.000000000000000000 ) ) ;
#13796=CARTESIAN_POINT ( 'NONE',  ( -32.01814843081346140, 461.6823905683720568, -16.75240474999999307 ) ) ;
#13798=CARTESIAN_POINT ( 'NONE',  ( -40.53162694259545162, 485.1198905683720000, 11.84573899990672885 ) ) ;
#13801=CARTESIAN_POINT ( 'NONE',  ( -28.68588794268872277, 429.4948905765655809, -19.99999999999999289 ) ) ;
#13803=CARTESIAN_POINT ( 'NONE',  ( -11.73070664223723902, 301.3073905601784759, 11.32908994701042005 ) ) ;
#13804=CARTESIAN_POINT ( 'NONE',  ( -28.68588794268869435, 193.9102039777116602, 0.000000000000000000 ) ) ;
#13805=CARTESIAN_POINT ( 'NONE',  ( -43.68588794268869435, 210.1437886375728965, 2.161863591991830530E-19 ) ) ;
#13806=VECTOR ( 'NONE', #20774, 1000.000000000000000 ) ;
#13809=DIRECTION ( 'NONE',  ( -1.191790137725560488E-16, 1.000000000000000000, -0.000000000000000000 ) ) ;
#13810=CARTESIAN_POINT ( 'NONE',  ( -16.84014894278197971, 271.6198905683720568, -11.84573899990672707 ) ) ;
#13812=CARTESIAN_POINT ( 'NONE',  ( -24.70764059509554755, 254.4323905601784759, -19.99999999999999289 ) ) ;
#13813=CARTESIAN_POINT ( 'NONE',  ( -36.33955658999051508, 363.8698905765656377, 18.47759065022572500 ) ) ;
#13814=CARTESIAN_POINT ( 'NONE',  ( -28.68588794268872277, 447.8698905683720000, 16.75240474999999307 ) ) ;
#13816=CARTESIAN_POINT ( 'NONE',  ( -42.88789093042842637, 276.3073905683720568, 9.489475012073736337 ) ) ;
#13818=CARTESIAN_POINT ( 'NONE',  ( -48.68588794268869435, 267.2448905601784759, 0.000000000000000000 ) ) ;
#13819=CARTESIAN_POINT ( 'NONE',  ( -22.27502019258949062, 478.4948905683720000, 15.47720386886985189 ) ) ;
#13821=EDGE_LOOP ( 'NONE', ( #5289, #11230, #10653, #10981 ) ) ;
#13823=CARTESIAN_POINT ( 'NONE',  ( -40.53162694259542320, 262.6198905683720568, -11.84573899990672707 ) ) ;
#13826=CARTESIAN_POINT ( 'NONE',  ( -48.68588794268872277, 491.9948905765656377, 0.000000000000000000 ) ) ;
#13827=CARTESIAN_POINT ( 'NONE',  ( -14.54375231895776466, 308.2448905765656377, -14.14213562373094746 ) ) ;
#13828=CARTESIAN_POINT ( 'NONE',  ( -8.685887942688555796, 452.5573905601784190, -3.978247347592740013 ) ) ;
#13829=CARTESIAN_POINT ( 'NONE',  ( -45.43829269268869808, 235.3698905683720284, 0.000000000000000000 ) ) ;
#13830=CARTESIAN_POINT ( 'NONE',  ( -11.93348319268874036, 520.0573905683719431, 3.332260488124728415 ) ) ;
#13832=CARTESIAN_POINT ( 'NONE',  ( -11.93348319268870839, 249.1823905683720568, -3.332260488124732856 ) ) ;
#13833=CARTESIAN_POINT ( 'NONE',  ( -45.43829269268871229, 345.3698905683720568, 0.000000000000000000 ) ) ;
#13837=CARTESIAN_POINT ( 'NONE',  ( -45.43829269268871229, 403.5573905683720000, -3.332260488124726194 ) ) ;
#13838=CARTESIAN_POINT ( 'NONE',  ( -10.20829729246298179, 326.3698905765656377, 7.653668647301790529 ) ) ;
#13839=CARTESIAN_POINT ( 'NONE',  ( -45.64106924314019409, 408.1823905601784759, 11.32908994701042715 ) ) ;
#13841=CARTESIAN_POINT ( 'NONE',  ( -21.03221929538692336, 348.8698905765656377, -18.47759065022572855 ) ) ;
#13842=ORIENTED_EDGE ( 'NONE', *, *, #15446, .T. ) ;
#13844=CARTESIAN_POINT ( 'NONE',  ( -22.27502019258949417, 498.4948905683720568, 15.47720386886985189 ) ) ;
#13845=CARTESIAN_POINT ( 'NONE',  ( -17.35679799567828496, 290.6823905601785327, 16.95518130045146421 ) ) ;
#13846=CARTESIAN_POINT ( 'NONE',  ( -21.03221929538691981, 318.8698905765656377, -18.47759065022572855 ) ) ;
#13848=ORIENTED_EDGE ( 'NONE', *, *, #1969, .T. ) ;
#13850=CARTESIAN_POINT ( 'NONE',  ( -44.16309181155856578, 324.7448905683720000, -6.410867750099231266 ) ) ;
#13853=CARTESIAN_POINT ( 'NONE',  ( -35.09675569278794427, 351.9948905683720000, -15.47720386886985544 ) ) ;
#13854=EDGE_CURVE ( 'NONE', #19602, #13635, #15970, .T. ) ;
#13855=CARTESIAN_POINT ( 'NONE',  ( -32.01814843081344719, 356.0573905683719431, 16.75240474999999307 ) ) ;
#13858=CARTESIAN_POINT ( 'NONE',  ( -11.73070664223724080, 287.9323905765655809, -11.32908994701042715 ) ) ;
#13860=CARTESIAN_POINT ( 'NONE',  ( -21.03221929538694113, 498.8698905765656377, -18.47759065022572855 ) ) ;
#13861=CARTESIAN_POINT ( 'NONE',  ( -35.09675569278793716, 255.7448905683720284, 15.47720386886985366 ) ) ;
#13862=CARTESIAN_POINT ( 'NONE',  ( -47.16347859291443001, 226.6198905601785043, -7.653668647301793193 ) ) ;
#13863=CARTESIAN_POINT ( 'NONE',  ( -28.68588794268872277, 422.8698905683720568, -16.75240474999999307 ) ) ;
#13865=CARTESIAN_POINT ( 'NONE',  ( -42.82802356641967378, 450.7448905765656377, -14.14213562373094746 ) ) ;
#13868=CARTESIAN_POINT ( 'NONE',  ( -13.20868407381885490, 320.9948905683720568, -6.410867750099233042 ) ) ;
#13869=CARTESIAN_POINT ( 'NONE',  ( -40.53162694259545162, 455.1198905683720568, 11.84573899990672885 ) ) ;
#13871=CARTESIAN_POINT ( 'NONE',  ( -42.82802356641967378, 475.9948905601784759, -14.14213562373094746 ) ) ;
#13872=CARTESIAN_POINT ( 'NONE',  ( -16.84014894278197971, 280.1198905683720000, -11.84573899990672707 ) ) ;
#13876=CARTESIAN_POINT ( 'NONE',  ( -45.43829269268871940, 445.3698905683720000, 0.000000000000000000 ) ) ;
#13877=ORIENTED_EDGE ( 'NONE', *, *, #16765, .T. ) ;
#13879=CARTESIAN_POINT ( 'NONE',  ( -14.48388495494899431, 309.8073905683720568, -9.489475012073736337 ) ) ;
#13880=CARTESIAN_POINT ( 'NONE',  ( -14.48388495494900674, 391.3073905683720568, -9.489475012073734561 ) ) ;
#13882=CARTESIAN_POINT ( 'NONE',  ( -17.35679799567830983, 515.4323905765655809, 16.95518130045146421 ) ) ;
#13883=CARTESIAN_POINT ( 'NONE',  ( -35.09675569278795138, 401.9948905683720568, -15.47720386886985544 ) ) ;
#13884=CARTESIAN_POINT ( 'NONE',  ( -45.43829269268869098, 235.0573905683720568, -3.332260488124726194 ) ) ;
#13885=CARTESIAN_POINT ( 'NONE',  ( -16.84014894278199392, 427.6198905683720000, 11.84573899990672530 ) ) ;
#13886=( BOUNDED_CURVE ( )  B_SPLINE_CURVE ( 2, ( #1534, #8104, #4875, #11469, #18067, #8216, #14844, #16043, #20, #2047, #5696, #3865, #13827, #3757, #17182, #10665, #8620 ),
 .UNSPECIFIED., .F., .T. ) 
 B_SPLINE_CURVE_WITH_KNOTS ( ( 3, 2, 2, 2, 2, 2, 2, 2, 3 ),
 ( 0.6875000000000002220, 0.6894531250000002220, 0.6914062500000002220, 0.6933593750000002220, 0.6953125000000002220, 0.6972656250000002220, 0.6992187500000002220, 0.7011718750000002220, 0.7031250000000002220 ),
 .UNSPECIFIED. ) 
 CURVE ( )  GEOMETRIC_REPRESENTATION_ITEM ( )  RATIONAL_B_SPLINE_CURVE ( ( 0.9999999999999977796, 0.9807852804032326510, 1.000000000000000000, 0.9807852804032304306, 1.000000000000000000, 0.9807852804032304306, 1.000000000000000000, 0.9807852804032304306, 1.000000000000000000, 0.9807852804032304306, 1.000000000000000000, 0.9807852804032304306, 1.000000000000000000, 0.9807852804032304306, 1.000000000000000000, 0.9807852804032282101, 1.000000000000002220 ) ) 
 REPRESENTATION_ITEM ( '' )  );
#13887=CARTESIAN_POINT ( 'NONE',  ( -21.03221929538690915, 345.1198905765656377, 18.47759065022572500 ) ) ;
#13889=CARTESIAN_POINT ( 'NONE',  ( -32.01814843081344719, 336.0573905683720568, 16.75240474999999307 ) ) ;
#13890=CARTESIAN_POINT ( 'NONE',  ( -22.27502019258949062, 478.4948905683720000, 15.47720386886985189 ) ) ;
#13891=CARTESIAN_POINT ( 'NONE',  ( -8.685887942688740537, 516.9948905765655809, -2.449293598294705724E-15 ) ) ;
#13894=FACE_OUTER_BOUND ( 'NONE', #9811, .T. ) ;
#13895=VECTOR ( 'NONE', #6101, 1000.000000000000000 ) ;
#13896=CARTESIAN_POINT ( 'NONE',  ( -11.93348319268872437, 390.3698905683720568, -2.051577885510841163E-15 ) ) ;
#13898=CARTESIAN_POINT ( 'NONE',  ( -48.68588794268872988, 527.5573905601784190, 3.978247347593168115 ) ) ;
#13899=CARTESIAN_POINT ( 'NONE',  ( -45.43829269268871229, 343.8698905683720000, 0.000000000000000000 ) ) ;
#13900=VERTEX_POINT ( 'NONE', #8175 ) ;
#13901=CARTESIAN_POINT ( 'NONE',  ( -28.68588794268872988, 506.3698905683720000, 16.75240474999999307 ) ) ;
#13902=VERTEX_POINT ( 'NONE', #14806 ) ;
#13903=CARTESIAN_POINT ( 'NONE',  ( -47.16347859291444422, 356.6198905601784759, -7.653668647301793193 ) ) ;
#13904=CARTESIAN_POINT ( 'NONE',  ( -45.44977940338448974, 223.9102039777116602, -0.2342134211204321415 ) ) ;
#13905=DIRECTION ( 'NONE',  ( -1.191790137725560488E-16, 1.000000000000000000, -0.000000000000000000 ) ) ;
#13906=CARTESIAN_POINT ( 'NONE',  ( -11.73070664223724080, 287.9323905765655809, -11.32908994701042538 ) ) ;
#13907=CARTESIAN_POINT ( 'NONE',  ( -36.33955658999052929, 520.1198905765655809, -18.47759065022572855 ) ) ;
#13908=CARTESIAN_POINT ( 'NONE',  ( -32.01814843081346140, 471.6823905683720568, -16.75240474999999307 ) ) ;
#13910=ORIENTED_EDGE ( 'NONE', *, *, #6887, .F. ) ;
#13911=CARTESIAN_POINT ( 'NONE',  ( -13.20868407381887266, 478.2448905683720568, 6.410867750099229490 ) ) ;
#13912=CARTESIAN_POINT ( 'NONE',  ( -11.73070664223723192, 246.0573905765656093, 11.32908994701042005 ) ) ;
#13914=CARTESIAN_POINT ( 'NONE',  ( -24.70764059509556887, 409.1823905765655809, -19.99999999999999289 ) ) ;
#13918=CARTESIAN_POINT ( 'NONE',  ( -42.82802356641967378, 483.2448905765656377, 14.14213562373094923 ) ) ;
#13920=CARTESIAN_POINT ( 'NONE',  ( -32.66413529028185536, 239.4323905601785043, 19.99999999999999289 ) ) ;
#13924=CARTESIAN_POINT ( 'NONE',  ( -19.19641293061497578, 281.9323905683720568, -14.20200298773971603 ) ) ;
#13925=CARTESIAN_POINT ( 'NONE',  ( -45.64106924314017277, 246.3073905601784759, -11.32908994701042715 ) ) ;
#13926=CARTESIAN_POINT ( 'NONE',  ( -32.66413529028186957, 364.1823905765656377, 19.99999999999999289 ) ) ;
#13927=CARTESIAN_POINT ( 'NONE',  ( -44.16309181155858710, 454.7448905683720568, -6.410867750099231266 ) ) ;
#13928=CARTESIAN_POINT ( 'NONE',  ( -40.01497788969914637, 400.4323905765655809, -16.95518130045146421 ) ) ;
#13929=CARTESIAN_POINT ( 'NONE',  ( -45.43829269268869808, 275.0573905683720568, -3.332260488124726194 ) ) ;
#13932=VERTEX_POINT ( 'NONE', #3327 ) ;
#13933=CARTESIAN_POINT ( 'NONE',  ( -38.17536295476246977, 483.8073905683720000, -14.20200298773971426 ) ) ;
#13937=CARTESIAN_POINT ( 'NONE',  ( -19.19641293061497223, 240.4323905683720284, -14.20200298773971603 ) ) ;
#13941=EDGE_CURVE ( 'NONE', #16379, #11812, #16748, .T. ) ;
#13942=CARTESIAN_POINT ( 'NONE',  ( -42.82802356641967378, 473.2448905765655809, 14.14213562373094923 ) ) ;
#13943=CARTESIAN_POINT ( 'NONE',  ( -8.685887942688905738, 391.9323905601784759, 3.978247347593586447 ) ) ;
#13946=CARTESIAN_POINT ( 'NONE',  ( -42.88789093042845479, 516.3073905683720568, 9.489475012073736337 ) ) ;
#13947=CARTESIAN_POINT ( 'NONE',  ( -36.33955658999051508, 373.8698905765656377, 18.47759065022572500 ) ) ;
#13948=CARTESIAN_POINT ( 'NONE',  ( -44.16309181155855157, 254.4948905683720568, 6.410867750099241924 ) ) ;
#13949=CARTESIAN_POINT ( 'NONE',  ( -22.27502019258948351, 332.2448905683720568, -15.47720386886985544 ) ) ;
#13952=CARTESIAN_POINT ( 'NONE',  ( -48.68588794268887199, 302.3073905765655240, 3.978247347592742678 ) ) ;
#13954=EDGE_CURVE ( 'NONE', #10309, #21365, #18457, .T. ) ;
#13955=CARTESIAN_POINT ( 'NONE',  ( -32.01814843081345430, 401.6823905683720000, -16.75240474999999307 ) ) ;
#13958=CARTESIAN_POINT ( 'NONE',  ( -17.35679799567830273, 383.8073905601784190, -16.95518130045146421 ) ) ;
#13960=CARTESIAN_POINT ( 'NONE',  ( -32.66413529028186957, 349.8073905765655809, -19.99999999999999289 ) ) ;
#13961=VERTEX_POINT ( 'NONE', #10228 ) ;
#13962=ORIENTED_EDGE ( 'NONE', *, *, #13954, .F. ) ;
#13963=CARTESIAN_POINT ( 'NONE',  ( -42.88789093042845479, 516.3073905683720568, 9.489475012073736337 ) ) ;
#13964=CARTESIAN_POINT ( 'NONE',  ( -8.685887942688724550, 382.2448905601784759, -2.449293598294705724E-15 ) ) ;
#13968=CARTESIAN_POINT ( 'NONE',  ( -25.35362745456398414, 302.5573905683720568, -16.75240474999999307 ) ) ;
#13970=CARTESIAN_POINT ( 'NONE',  ( -16.84014894278198682, 340.1198905683720568, -11.84573899990672707 ) ) ;
#13971=CARTESIAN_POINT ( 'NONE',  ( -19.19641293061497933, 347.3073905683720568, 14.20200298773971426 ) ) ;
#13972=AXIS2_PLACEMENT_3D ( 'NONE', #9278, #15895, #10677 ) ;
#13973=CARTESIAN_POINT ( 'NONE',  ( -8.685887942688712116, 276.9948905765656377, -2.449293598294705724E-15 ) ) ;
#13974=CARTESIAN_POINT ( 'NONE',  ( -14.54375231895778775, 498.2448905765656377, -14.14213562373094746 ) ) ;
#13975=CARTESIAN_POINT ( 'NONE',  ( -32.01814843081343298, 241.6823905683720568, -16.75240474999999307 ) ) ;
#13976=CARTESIAN_POINT ( 'NONE',  ( -43.04679578547633412, 202.6324317550694332, 4.335932898175371086 ) ) ;
#13977=CARTESIAN_POINT ( 'NONE',  ( -11.93348319268872615, 400.6823905683720568, -3.332260488124732856 ) ) ;
#13979=CARTESIAN_POINT ( 'NONE',  ( -32.66413529028188378, 449.8073905765656377, -19.99999999999999289 ) ) ;
#13980=CARTESIAN_POINT ( 'NONE',  ( -44.16309181155858710, 453.2448905683720000, -6.410867750099231266 ) ) ;
#13982=CARTESIAN_POINT ( 'NONE',  ( -8.685887942688731655, 452.2448905601784759, -2.449293598294705724E-15 ) ) ;
#13983=CARTESIAN_POINT ( 'NONE',  ( -11.93348319268871371, 279.1823905683720000, -3.332260488124732856 ) ) ;
#13984=AXIS2_PLACEMENT_3D ( 'NONE', #20039, #11815, #5316 ) ;
#13985=ORIENTED_EDGE ( 'NONE', *, *, #16976, .F. ) ;
#13986=CARTESIAN_POINT ( 'NONE',  ( -21.03221929538690560, 340.3698905601784759, 18.47759065022572500 ) ) ;
#13989=CARTESIAN_POINT ( 'NONE',  ( -28.68588794268874054, 573.2448905601785327, 0.000000000000000000 ) ) ;
#13990=CARTESIAN_POINT ( 'NONE',  ( -13.20868407381885312, 299.4948905683720568, -6.410867750099233042 ) ) ;
#13991=CARTESIAN_POINT ( 'NONE',  ( -40.53162694259543741, 364.1198905683720000, -11.84573899990672707 ) ) ;
#13992=CARTESIAN_POINT ( 'NONE',  ( -24.70764059509555821, 374.4323905601784759, -19.99999999999999289 ) ) ;
#13993=CARTESIAN_POINT ( 'NONE',  ( -32.66413529028189799, 514.1823905765656946, 19.99999999999999289 ) ) ;
#13994=CARTESIAN_POINT ( 'NONE',  ( -28.68588794268872277, 411.3698905683720568, -16.75240474999999307 ) ) ;
#13995=CARTESIAN_POINT ( 'NONE',  ( -28.68588794268870146, 232.8698905683720284, -16.75240474999999307 ) ) ;
#13997=CARTESIAN_POINT ( 'NONE',  ( -32.01814843081344719, 416.0573905683721136, 16.75240474999999307 ) ) ;
#13998=EDGE_CURVE ( 'NONE', #11378, #12297, #3264, .T. ) ;
#13999=CARTESIAN_POINT ( 'NONE',  ( -48.68588794268870856, 351.6823905765656377, -3.978247347593158345 ) ) ;
#14001=CARTESIAN_POINT ( 'NONE',  ( -25.35362745456398414, 311.0573905683720568, -16.75240474999999307 ) ) ;
#14003=CARTESIAN_POINT ( 'NONE',  ( -22.27502019258949773, 462.2448905683720568, -15.47720386886985544 ) ) ;
#14004=CARTESIAN_POINT ( 'NONE',  ( -36.33955658999053639, 513.8698905765655809, 18.47759065022572500 ) ) ;
#14007=CARTESIAN_POINT ( 'NONE',  ( -44.16309181155857289, 364.7448905683720568, -6.410867750099231266 ) ) ;
#14009=CARTESIAN_POINT ( 'NONE',  ( -8.685887942688744090, 531.9323905601785327, 3.978247347593161010 ) ) ;
#14010=CARTESIAN_POINT ( 'NONE',  ( -11.93348319268871904, 348.8698905683720568, -2.051577885510841163E-15 ) ) ;
#14011=ORIENTED_EDGE ( 'NONE', *, *, #6887, .T. ) ;
#14012=CARTESIAN_POINT ( 'NONE',  ( -11.93348319268873858, 498.5573905683720568, 3.332260488124728415 ) ) ;
#14014=( BOUNDED_CURVE ( )  B_SPLINE_CURVE ( 2, ( #19866, #5043, #3639, #10221, #16846, #7081, #3847, #5893, #20295, #20399, #8921, #18765, #3953, #17056, #17370, #7403, #14029 ),
 .UNSPECIFIED., .F., .T. ) 
 B_SPLINE_CURVE_WITH_KNOTS ( ( 3, 2, 2, 2, 2, 2, 2, 2, 3 ),
 ( 0.3125000000000001110, 0.3144531250000001110, 0.3164062500000001110, 0.3183593750000001110, 0.3203125000000001110, 0.3222656250000001110, 0.3242187500000001110, 0.3261718750000001110, 0.3281250000000001110 ),
 .UNSPECIFIED. ) 
 CURVE ( )  GEOMETRIC_REPRESENTATION_ITEM ( )  RATIONAL_B_SPLINE_CURVE ( ( 0.9999999999999988898, 0.9807852804032315408, 1.000000000000000000, 0.9807852804032304306, 1.000000000000000000, 0.9807852804032304306, 1.000000000000000000, 0.9807852804032304306, 1.000000000000000000, 0.9807852804032304306, 1.000000000000000000, 0.9807852804032304306, 1.000000000000000000, 0.9807852804032304306, 1.000000000000000000, 0.9807852804032293204, 1.000000000000001110 ) ) 
 REPRESENTATION_ITEM ( '' )  );
#14015=CARTESIAN_POINT ( 'NONE',  ( -40.01497788969913927, 380.4323905765655240, -16.95518130045146421 ) ) ;
#14016=CARTESIAN_POINT ( 'NONE',  ( -14.54375231895776110, 315.7448905765656377, 14.14213562373094568 ) ) ;
#14019=CARTESIAN_POINT ( 'NONE',  ( -11.93348319268873503, 468.8698905683720000, -2.051577885510841163E-15 ) ) ;
#14021=CARTESIAN_POINT ( 'NONE',  ( -32.01814843081345430, 466.0573905683720568, 16.75240474999999307 ) ) ;
#14023=CARTESIAN_POINT ( 'NONE',  ( -10.20829729246299067, 406.3698905765656377, 7.653668647301790529 ) ) ;
#14024=LINE ( 'NONE', #7504, #5834 ) ;
#14028=CARTESIAN_POINT ( 'NONE',  ( -10.20829729246297468, 257.6198905765656377, -7.653668647301794969 ) ) ;
#14029=CARTESIAN_POINT ( 'NONE',  ( -8.685887942688729879, 432.2448905601785327, -2.449293598294705724E-15 ) ) ;
#14031=CARTESIAN_POINT ( 'NONE',  ( -45.43829269268870519, 275.3698905683720000, 0.000000000000000000 ) ) ;
#14032=CARTESIAN_POINT ( 'NONE',  ( -24.70764059509553334, 250.0573905601785043, 19.99999999999998934 ) ) ;
#14034=CARTESIAN_POINT ( 'NONE',  ( -8.685887942688719221, 326.9948905765656377, -2.449293598294705724E-15 ) ) ;
#14035=CARTESIAN_POINT ( 'NONE',  ( -35.09675569278794427, 277.2448905683720568, 15.47720386886985366 ) ) ;
#14037=CARTESIAN_POINT ( 'NONE',  ( -17.35679799567830983, 478.5573905765656377, -16.95518130045146421 ) ) ;
#14039=CARTESIAN_POINT ( 'NONE',  ( -44.16309181155857999, 475.9948905683720000, 6.410867750099241924 ) ) ;
#14042=CARTESIAN_POINT ( 'NONE',  ( -10.20829729246300666, 526.3698905765656946, 7.653668647301790529 ) ) ;
#14043=CARTESIAN_POINT ( 'NONE',  ( -11.93348319268870661, 238.8698905683720568, -2.051577885510841163E-15 ) ) ;
#14045=LINE ( 'NONE', #747, #14547 ) ;
#14046=CARTESIAN_POINT ( 'NONE',  ( -42.82802356641967378, 463.2448905765656377, 14.14213562373094923 ) ) ;
#14049=CARTESIAN_POINT ( 'NONE',  ( -20.38821492105416056, 223.9102039777116602, -17.94255365484195508 ) ) ;
#14050=CARTESIAN_POINT ( 'NONE',  ( -45.43829269268869808, 225.6823905683720284, 3.332260488124734632 ) ) ;
#14051=CARTESIAN_POINT ( 'NONE',  ( -45.43829269268873361, 525.3698905683720568, 0.000000000000000000 ) ) ;
#14052=CARTESIAN_POINT ( 'NONE',  ( -48.68588794268887199, 372.3073905765655809, 3.978247347592742678 ) ) ;
#14053=CARTESIAN_POINT ( 'NONE',  ( -44.16309181155855157, 244.4948905683720284, 6.410867750099241924 ) ) ;
#14054=CARTESIAN_POINT ( 'NONE',  ( -19.19641293061497933, 338.8073905683720000, 14.20200298773971426 ) ) ;
#14056=CARTESIAN_POINT ( 'NONE',  ( -8.685887942688887975, 276.6823905765655809, 3.978247347593586447 ) ) ;
#14059=CARTESIAN_POINT ( 'NONE',  ( -11.93348319268872437, 389.1823905683721136, -3.332260488124732856 ) ) ;
#14061=CARTESIAN_POINT ( 'NONE',  ( -32.66413529028187668, 385.0573905601784190, -19.99999999999999289 ) ) ;
#14066=CARTESIAN_POINT ( 'NONE',  ( -35.09675569278796559, 513.4948905683720568, -15.47720386886985544 ) ) ;
#14068=ORIENTED_EDGE ( 'NONE', *, *, #4472, .T. ) ;
#14069=CARTESIAN_POINT ( 'NONE',  ( -25.35362745456398414, 312.5573905683720000, -16.75240474999999307 ) ) ;
#14071=CARTESIAN_POINT ( 'NONE',  ( -35.09675569278795138, 335.7448905683720568, 15.47720386886985366 ) ) ;
#14072=CARTESIAN_POINT ( 'NONE',  ( -28.68588794268871212, 341.3698905683720000, -16.75240474999999307 ) ) ;
#14073=EDGE_CURVE ( 'NONE', #10903, #12168, #2135, .T. ) ;
#14075=CARTESIAN_POINT ( 'NONE',  ( -14.54375231895775755, 285.7448905765655809, 14.14213562373094568 ) ) ;
#14076=CARTESIAN_POINT ( 'NONE',  ( -40.01497788969914637, 395.6823905601784190, -16.95518130045146421 ) ) ;
#14077=CARTESIAN_POINT ( 'NONE',  ( -16.84014894278197261, 237.6198905683720284, 11.84573899990672530 ) ) ;
#14079=CARTESIAN_POINT ( 'NONE',  ( -16.84014894278199037, 399.1198905683720000, 11.84573899990672530 ) ) ;
#14085=CARTESIAN_POINT ( 'NONE',  ( -44.16309181155857999, 433.2448905683720000, -6.410867750099231266 ) ) ;
#14086=ORIENTED_EDGE ( 'NONE', *, *, #6959, .T. ) ;
#14087=CARTESIAN_POINT ( 'NONE',  ( -36.33955658999052218, 439.1198905601784759, 18.47759065022572500 ) ) ;
#14090=DIRECTION ( 'NONE',  ( -1.191790137725560488E-16, 1.000000000000000000, -0.000000000000000000 ) ) ;
#14094=CARTESIAN_POINT ( 'NONE',  ( -47.16347859291443712, 317.8698905601784190, 7.653668647301805628 ) ) ;
#14095=CARTESIAN_POINT ( 'NONE',  ( -19.19641293061497578, 297.3073905683720568, 14.20200298773971426 ) ) ;
#14096=VECTOR ( 'NONE', #3477, 1000.000000000000000 ) ;
#14097=CARTESIAN_POINT ( 'NONE',  ( -45.43829269268871229, 355.6823905683720568, 3.332260488124734632 ) ) ;
#14099=CARTESIAN_POINT ( 'NONE',  ( -32.66413529028189799, 529.8073905765656946, -19.99999999999999289 ) ) ;
#14100=CARTESIAN_POINT ( 'NONE',  ( -42.88789093042844058, 404.8073905683721136, 9.489475012073736337 ) ) ;
#14101=CARTESIAN_POINT ( 'NONE',  ( -45.43829269268869808, 245.3698905683720568, 0.000000000000000000 ) ) ;
#14102=CARTESIAN_POINT ( 'NONE',  ( -11.93348319268872615, 408.5573905683721136, 3.332260488124728859 ) ) ;
#14103=CARTESIAN_POINT ( 'NONE',  ( -40.01497788969913216, 343.5573905765655809, 16.95518130045146776 ) ) ;
#14104=CARTESIAN_POINT ( 'NONE',  ( -21.03221929538691981, 324.1198905601784759, -18.47759065022572855 ) ) ;
#14105=CARTESIAN_POINT ( 'NONE',  ( -28.68588794268870501, 296.3698905683720568, 16.75240474999999307 ) ) ;
#14106=CARTESIAN_POINT ( 'NONE',  ( -45.43829269268872650, 465.3698905683720000, 0.000000000000000000 ) ) ;
#14107=CARTESIAN_POINT ( 'NONE',  ( -14.54375231895777887, 460.9948905601785327, 14.14213562373094568 ) ) ;
#14110=CARTESIAN_POINT ( 'NONE',  ( -38.17536295476245556, 373.8073905683720000, -14.20200298773971426 ) ) ;
#14111=CARTESIAN_POINT ( 'NONE',  ( -22.27502019258949417, 506.9948905683721136, 15.47720386886985189 ) ) ;
#14112=CARTESIAN_POINT ( 'NONE',  ( -28.68588794268872988, 509.7448905601784759, 19.99999999999999289 ) ) ;
#14113=CARTESIAN_POINT ( 'NONE',  ( -11.93348319268871904, 338.8698905683720000, -2.051577885510841163E-15 ) ) ;
#14115=CARTESIAN_POINT ( 'NONE',  ( -28.68588794268872988, 496.3698905683720568, 16.75240474999999307 ) ) ;
#14117=CARTESIAN_POINT ( 'NONE',  ( -45.43829269268873361, 535.3698905683720568, 0.000000000000000000 ) ) ;
#14118=CARTESIAN_POINT ( 'NONE',  ( -42.88789093042844058, 414.4323905683720000, -9.489475012073734561 ) ) ;
#14119=CARTESIAN_POINT ( 'NONE',  ( -32.66413529028186247, 289.8073905765656946, -19.99999999999999289 ) ) ;
#14120=CARTESIAN_POINT ( 'NONE',  ( -48.68588794268871567, 521.6823905765656946, -3.978247347593212080 ) ) ;
#14121=CARTESIAN_POINT ( 'NONE',  ( -16.84014894278200103, 460.1198905683720568, -11.84573899990672707 ) ) ;
#14122=ORIENTED_EDGE ( 'NONE', *, *, #18558, .F. ) ;
#14123=CARTESIAN_POINT ( 'NONE',  ( -11.93348319268873503, 469.1823905683719431, -3.332260488124732856 ) ) ;
#14124=CARTESIAN_POINT ( 'NONE',  ( -47.16347859291443001, 242.6198905765656377, 7.653668647301805628 ) ) ;
#14126=CARTESIAN_POINT ( 'NONE',  ( -47.16347859291445133, 401.3698905765656377, -7.653668647301793193 ) ) ;
#14127=CARTESIAN_POINT ( 'NONE',  ( -24.70764059509554755, 279.1823905765656377, -19.99999999999999289 ) ) ;
#14129=CARTESIAN_POINT ( 'NONE',  ( -48.68588794268872277, 467.2448905601784759, 0.000000000000000000 ) ) ;
#14132=EDGE_CURVE ( 'NONE', #126, #2082, #4766, .T. ) ;
#14134=CARTESIAN_POINT ( 'NONE',  ( -45.64106924314017988, 346.3073905601784759, -11.32908994701042538 ) ) ;
#14135=CARTESIAN_POINT ( 'NONE',  ( -35.09675569278793716, 273.4948905683720000, -15.47720386886985544 ) ) ;
#14137=CARTESIAN_POINT ( 'NONE',  ( -21.03221929538690915, 244.1198905601784759, -18.47759065022572855 ) ) ;
#14139=CARTESIAN_POINT ( 'NONE',  ( -40.53162694259544452, 436.6198905683720000, 11.84573899990672885 ) ) ;
#14140=CARTESIAN_POINT ( 'NONE',  ( -8.685887942688726326, 396.9948905765656377, -2.449293598294705724E-15 ) ) ;
#14141=CARTESIAN_POINT ( 'NONE',  ( -45.43829269268869098, 245.0573905683720000, -3.332260488124726194 ) ) ;
#14142=EDGE_CURVE ( 'NONE', #13421, #2991, #2454, .T. ) ;
#14143=ORIENTED_EDGE ( 'NONE', *, *, #15503, .T. ) ;
#14145=VERTEX_POINT ( 'NONE', #14250 ) ;
#14146=CARTESIAN_POINT ( 'NONE',  ( -16.84014894278200458, 481.6198905683720000, -11.84573899990672707 ) ) ;
#14148=CARTESIAN_POINT ( 'NONE',  ( -24.70764059509555821, 364.4323905601784759, -19.99999999999999289 ) ) ;
#14149=CARTESIAN_POINT ( 'NONE',  ( -11.93348319268870839, 238.5573905683720000, 3.332260488124728415 ) ) ;
#14151=CARTESIAN_POINT ( 'NONE',  ( -32.01814843081346140, 521.6823905683719431, -16.75240474999999307 ) ) ;
#14153=AXIS2_PLACEMENT_3D ( 'NONE', #6310, #13247, #9868 ) ;
#14154=CARTESIAN_POINT ( 'NONE',  ( -48.68588794268872277, 462.3073905765655809, 3.978247347593168115 ) ) ;
#14157=CARTESIAN_POINT ( 'NONE',  ( -30.27473451612855015, 223.9102039777116318, -18.25316008977560855 ) ) ;
#14159=CARTESIAN_POINT ( 'NONE',  ( -25.35362745456399836, 508.1823905683720568, 16.75240474999998952 ) ) ;
#14160=CARTESIAN_POINT ( 'NONE',  ( -8.685887942688902186, 376.6823905765656377, 3.978247347593586447 ) ) ;
#14162=CARTESIAN_POINT ( 'NONE',  ( -35.09675569278793716, 255.7448905683720284, 15.47720386886985366 ) ) ;
#14163=CARTESIAN_POINT ( 'NONE',  ( -42.88789093042843348, 346.3073905683720568, 9.489475012073736337 ) ) ;
#14167=CARTESIAN_POINT ( 'NONE',  ( -45.43829269268871229, 383.8698905683720000, 0.000000000000000000 ) ) ;
#14168=CARTESIAN_POINT ( 'NONE',  ( -17.35679799567828496, 325.4323905765656377, 16.95518130045146421 ) ) ;
#14169=CARTESIAN_POINT ( 'NONE',  ( -8.685887942688724550, 392.5573905601785896, -3.978247347593165895 ) ) ;
#14174=CARTESIAN_POINT ( 'NONE',  ( -28.68588794268872988, 497.8698905683720568, 16.75240474999999307 ) ) ;
#14175=CARTESIAN_POINT ( 'NONE',  ( -45.64106924314017277, 292.9323905765656377, 11.32908994701042538 ) ) ;
#14177=CARTESIAN_POINT ( 'NONE',  ( -11.93348319268871549, 310.0573905683720568, 3.332260488124728859 ) ) ;
#14179=CARTESIAN_POINT ( 'NONE',  ( -44.16309181155855867, 324.4948905683720568, 6.410867750099241924 ) ) ;
#14180=CARTESIAN_POINT ( 'NONE',  ( -44.16309181155857289, 353.2448905683720000, -6.410867750099231266 ) ) ;
#14182=CARTESIAN_POINT ( 'NONE',  ( -11.73070664223723725, 286.0573905765656377, 11.32908994701042005 ) ) ;
#14184=CARTESIAN_POINT ( 'NONE',  ( -38.17536295476244135, 242.3073905683720284, -14.20200298773971426 ) ) ;
#14186=CARTESIAN_POINT ( 'NONE',  ( -19.19641293061498644, 398.8073905683720568, 14.20200298773971426 ) ) ;
#14187=CARTESIAN_POINT ( 'NONE',  ( -32.66413529028186957, 335.0573905601785327, -19.99999999999999289 ) ) ;
#14189=ADVANCED_FACE ( 'NONE', ( #12616 ), #8042, .T. ) ;
#14190=DIRECTION ( 'NONE',  ( -1.191790137725560488E-16, 1.000000000000000000, -0.000000000000000000 ) ) ;
#14191=CARTESIAN_POINT ( 'NONE',  ( -28.68588794268872633, 451.3698905683720000, -16.75240474999999307 ) ) ;
#14193=CARTESIAN_POINT ( 'NONE',  ( -24.70764059509556176, 450.0573905601785327, 19.99999999999998934 ) ) ;
#14194=VERTEX_POINT ( 'NONE', #17792 ) ;
#14196=CARTESIAN_POINT ( 'NONE',  ( -8.685887942688742314, 573.2448905601785327, 2.449293598294706119E-15 ) ) ;
#14198=EDGE_CURVE ( 'NONE', #15181, #11055, #12358, .T. ) ;
#14199=VERTEX_POINT ( 'NONE', #13035 ) ;
#14201=CARTESIAN_POINT ( 'NONE',  ( -17.35679799567829562, 333.8073905601784759, -16.95518130045146421 ) ) ;
#14202=CARTESIAN_POINT ( 'NONE',  ( -16.84014894278198682, 369.1198905683720000, 11.84573899990672530 ) ) ;
#14205=CARTESIAN_POINT ( 'NONE',  ( -8.685887942688742314, 516.6823905765655809, 3.978247347593161010 ) ) ;
#14206=CARTESIAN_POINT ( 'NONE',  ( -14.48388495494900496, 397.9323905683719431, 9.489475012073732785 ) ) ;
#14207=CARTESIAN_POINT ( 'NONE',  ( -19.19641293061497223, 241.9323905683720284, -14.20200298773971603 ) ) ;
#14208=AXIS2_PLACEMENT_3D ( 'NONE', #18515, #3701, #19830 ) ;
#14209=CARTESIAN_POINT ( 'NONE',  ( -22.27502019258948351, 406.9948905683720000, 15.47720386886985189 ) ) ;
#14211=CARTESIAN_POINT ( 'NONE',  ( -14.54375231895776821, 338.2448905765656377, -14.14213562373094746 ) ) ;
#14213=CARTESIAN_POINT ( 'NONE',  ( -44.16309181155855867, 304.4948905683720568, 6.410867750099241924 ) ) ;
#14214=CARTESIAN_POINT ( 'NONE',  ( -13.20868407381887089, 459.7448905683720568, 6.410867750099229490 ) ) ;
#14219=CARTESIAN_POINT ( 'NONE',  ( -42.88789093042843348, 376.3073905683720000, 9.489475012073736337 ) ) ;
#14221=CARTESIAN_POINT ( 'NONE',  ( -14.48388495494901740, 509.8073905683720000, -9.489475012073736337 ) ) ;
#14222=CARTESIAN_POINT ( 'NONE',  ( -36.33955658999052929, 499.1198905601784759, 18.47759065022572500 ) ) ;
#14223=CARTESIAN_POINT ( 'NONE',  ( -13.20868407381885490, 328.2448905683720000, 6.410867750099229490 ) ) ;
#14226=CARTESIAN_POINT ( 'NONE',  ( -22.27502019258949417, 496.9948905683720568, 15.47720386886985189 ) ) ;
#14228=CARTESIAN_POINT ( 'NONE',  ( -48.68588794268870146, 311.9948905765655809, 0.000000000000000000 ) ) ;
#14229=CARTESIAN_POINT ( 'NONE',  ( -40.53162694259544452, 424.1198905683720000, -11.84573899990672707 ) ) ;
#14230=CARTESIAN_POINT ( 'NONE',  ( -8.685887942688859553, 396.6823905765656377, 3.978247347593479866 ) ) ;
#14232=CARTESIAN_POINT ( 'NONE',  ( -14.48388495494901385, 469.8073905683719431, -9.489475012073736337 ) ) ;
#14234=CARTESIAN_POINT ( 'NONE',  ( -19.19641293061498999, 457.3073905683720568, 14.20200298773971426 ) ) ;
#14235=CARTESIAN_POINT ( 'NONE',  ( -48.68588794268878672, 242.3073905765656093, 3.978247347592954952 ) ) ;
#14237=CARTESIAN_POINT ( 'NONE',  ( -42.82802356641966668, 400.7448905765656377, -14.14213562373094746 ) ) ;
#14238=CARTESIAN_POINT ( 'NONE',  ( -17.35679799567828496, 278.5573905765656377, -16.95518130045146421 ) ) ;
#14240=CARTESIAN_POINT ( 'NONE',  ( -21.03221929538692336, 368.8698905765656377, -18.47759065022572855 ) ) ;
#14246=CARTESIAN_POINT ( 'NONE',  ( -10.20829729246297291, 242.8698905601785043, -7.653668647301794969 ) ) ;
#14249=CARTESIAN_POINT ( 'NONE',  ( -38.17536295476245556, 436.9323905683720568, 14.20200298773971781 ) ) ;
#14250=CARTESIAN_POINT ( 'NONE',  ( -8.685887942688738761, 502.2448905601784190, -2.449293598294705724E-15 ) ) ;
#14251=CARTESIAN_POINT ( 'NONE',  ( -42.88789093042841927, 244.4323905683720284, -9.489475012073736337 ) ) ;
#14254=DIRECTION ( 'NONE',  ( -1.191790137725560488E-16, 1.000000000000000000, -0.000000000000000000 ) ) ;
#14256=CARTESIAN_POINT ( 'NONE',  ( -16.84014894278200103, 461.6198905683720568, -11.84573899990672707 ) ) ;
#14259=FACE_OUTER_BOUND ( 'NONE', #7733, .T. ) ;
#14260=CARTESIAN_POINT ( 'NONE',  ( -44.16309181155855157, 244.4948905683720284, 6.410867750099241924 ) ) ;
#14262=CARTESIAN_POINT ( 'NONE',  ( -22.27502019258949417, 516.9948905683720568, 15.47720386886985189 ) ) ;
#14264=CARTESIAN_POINT ( 'NONE',  ( -42.82802356641967378, 470.7448905765655809, -14.14213562373094746 ) ) ;
#14266=CARTESIAN_POINT ( 'NONE',  ( -24.70764059509554045, 284.8073905765656377, 19.99999999999998934 ) ) ;
#14267=CARTESIAN_POINT ( 'NONE',  ( -18.66797547166049753, 223.9102039777116602, -17.31025331282116397 ) ) ;
#14273=CARTESIAN_POINT ( 'NONE',  ( -16.84014894278197616, 230.1198905683720000, -11.84573899990672707 ) ) ;
#14274=( BOUNDED_CURVE ( )  B_SPLINE_CURVE ( 2, ( #8166, #21168, #21381, #11536, #9484, #18128, #17706, #9795, #2903, #16094, #6340, #9588, #12952, #21271, #16314, #19542, #1486 ),
 .UNSPECIFIED., .F., .T. ) 
 B_SPLINE_CURVE_WITH_KNOTS ( ( 3, 2, 2, 2, 2, 2, 2, 2, 3 ),
 ( 0.7656250000000001110, 0.7675781250000001110, 0.7695312500000001110, 0.7714843750000001110, 0.7734375000000001110, 0.7753906250000001110, 0.7773437500000001110, 0.7792968750000001110, 0.7812500000000001110 ),
 .UNSPECIFIED. ) 
 CURVE ( )  GEOMETRIC_REPRESENTATION_ITEM ( )  RATIONAL_B_SPLINE_CURVE ( ( 0.9999999999999988898, 0.9807852804032315408, 1.000000000000000000, 0.9807852804032304306, 1.000000000000000000, 0.9807852804032304306, 1.000000000000000000, 0.9807852804032304306, 1.000000000000000000, 0.9807852804032304306, 1.000000000000000000, 0.9807852804032304306, 1.000000000000000000, 0.9807852804032304306, 1.000000000000000000, 0.9807852804032293204, 1.000000000000001110 ) ) 
 REPRESENTATION_ITEM ( '' )  );
#14275=CARTESIAN_POINT ( 'NONE',  ( -42.88789093042843348, 334.4323905683720568, -9.489475012073736337 ) ) ;
#14276=CARTESIAN_POINT ( 'NONE',  ( -48.68588794268872277, 467.2448905601784759, 0.000000000000000000 ) ) ;
#14278=CARTESIAN_POINT ( 'NONE',  ( -11.93348319268871549, 310.3698905683720568, -2.051577885510841163E-15 ) ) ;
#14279=CARTESIAN_POINT ( 'NONE',  ( -22.27502019258949062, 380.7448905683720000, -15.47720386886985544 ) ) ;
#14283=CARTESIAN_POINT ( 'NONE',  ( -17.35679799567829562, 390.6823905601785327, 16.95518130045146421 ) ) ;
#14284=CARTESIAN_POINT ( 'NONE',  ( -36.33955658999051508, 405.3698905601785327, -18.47759065022572855 ) ) ;
#14285=EDGE_LOOP ( 'NONE', ( #240, #3306, #5991, #16692 ) ) ;
#14286=ORIENTED_EDGE ( 'NONE', *, *, #11991, .F. ) ;
#14287=CARTESIAN_POINT ( 'NONE',  ( -28.68588794268873343, 512.8698905683719431, -16.75240474999999307 ) ) ;
#14288=FACE_OUTER_BOUND ( 'NONE', #17383, .T. ) ;
#14290=CARTESIAN_POINT ( 'NONE',  ( -22.27502019258947996, 302.2448905683720000, -15.47720386886985544 ) ) ;
#14292=CARTESIAN_POINT ( 'NONE',  ( -16.84014894278198682, 330.1198905683720568, -11.84573899990672707 ) ) ;
#14294=CARTESIAN_POINT ( 'NONE',  ( -47.16347859291443712, 271.3698905765656377, -7.653668647301793193 ) ) ;
#14295=CARTESIAN_POINT ( 'NONE',  ( -47.16347859291445843, 501.3698905765655809, -7.653668647301793193 ) ) ;
#14296=CARTESIAN_POINT ( 'NONE',  ( -25.35362745456396638, 246.6823905683720568, 16.75240474999998952 ) ) ;
#14298=AXIS2_PLACEMENT_3D ( 'NONE', #18286, #1976, #13330 ) ;
#14299=CARTESIAN_POINT ( 'NONE',  ( -44.16309181155857999, 404.7448905683720568, -6.410867750099231266 ) ) ;
#14302=CARTESIAN_POINT ( 'NONE',  ( -48.68588794268872988, 511.9948905765656377, 0.000000000000000000 ) ) ;
#14303=CARTESIAN_POINT ( 'NONE',  ( -32.01814843081345430, 436.0573905683720568, 16.75240474999999307 ) ) ;
#14305=CARTESIAN_POINT ( 'NONE',  ( -8.685887942688729879, 441.9323905601784759, 3.978247347593161010 ) ) ;
#14308=ORIENTED_EDGE ( 'NONE', *, *, #16923, .F. ) ;
#14311=CARTESIAN_POINT ( 'NONE',  ( -10.20829729246298001, 321.6198905601784759, 7.653668647301790529 ) ) ;
#14315=CARTESIAN_POINT ( 'NONE',  ( -28.68588794268871212, 357.8698905683720568, 16.75240474999999307 ) ) ;
#14316=CARTESIAN_POINT ( 'NONE',  ( -28.68588794268869435, 193.9102039777116602, 0.000000000000000000 ) ) ;
#14317=EDGE_CURVE ( 'NONE', #16878, #9671, #21071, .T. ) ;
#14318=CARTESIAN_POINT ( 'NONE',  ( -24.70764059509556887, 494.8073905765656377, 19.99999999999998934 ) ) ;
#14319=CARTESIAN_POINT ( 'NONE',  ( -42.88789093042843348, 382.9323905683720568, -9.489475012073736337 ) ) ;
#14320=CARTESIAN_POINT ( 'NONE',  ( -25.35362745456396638, 248.1823905683720284, 16.75240474999998952 ) ) ;
#14321=CARTESIAN_POINT ( 'NONE',  ( -14.48388495494900674, 399.8073905683720568, -9.489475012073734561 ) ) ;
#14322=CARTESIAN_POINT ( 'NONE',  ( -8.685887942688715668, 317.3073905765656377, -3.978247347593165895 ) ) ;
#14323=CARTESIAN_POINT ( 'NONE',  ( -17.35679799567829207, 323.8073905601784190, -16.95518130045146421 ) ) ;
#14324=CARTESIAN_POINT ( 'NONE',  ( -45.43829269268870519, 303.8698905683720000, 0.000000000000000000 ) ) ;
#14325=CARTESIAN_POINT ( 'NONE',  ( -11.93348319268873148, 450.0573905683719431, 3.332260488124728415 ) ) ;
#14326=CARTESIAN_POINT ( 'NONE',  ( -48.68588794268872277, 457.2448905601784759, 0.000000000000000000 ) ) ;
#14327=CARTESIAN_POINT ( 'NONE',  ( -14.54375231895776821, 370.9948905601784759, 14.14213562373094568 ) ) ;
#14328=LINE ( 'NONE', #19071, #13362 ) ;
#14330=CARTESIAN_POINT ( 'NONE',  ( -16.84014894278198682, 359.1198905683720568, 11.84573899990672530 ) ) ;
#14331=CARTESIAN_POINT ( 'NONE',  ( -38.17536295476246977, 502.3073905683720568, -14.20200298773971426 ) ) ;
#14333=CARTESIAN_POINT ( 'NONE',  ( -28.68588794268873343, 514.7448905601784190, -19.99999999999999289 ) ) ;
#14334=CARTESIAN_POINT ( 'NONE',  ( -11.93348319268871727, 328.8698905683720000, -2.051577885510841163E-15 ) ) ;
#14337=CARTESIAN_POINT ( 'NONE',  ( -48.68588794268872988, 527.2448905601785327, 0.000000000000000000 ) ) ;
#14339=CARTESIAN_POINT ( 'NONE',  ( -35.09675569278795138, 423.4948905683720568, -15.47720386886985544 ) ) ;
#14340=CARTESIAN_POINT ( 'NONE',  ( -8.685887942688731655, 446.9948905765655809, -2.449293598294705724E-15 ) ) ;
#14341=DIRECTION ( 'NONE',  ( -1.191790137725560488E-16, 1.000000000000000000, -0.000000000000000000 ) ) ;
#14342=CARTESIAN_POINT ( 'NONE',  ( -11.93348319268873148, 449.1823905683720000, -3.332260488124732856 ) ) ;
#14344=CARTESIAN_POINT ( 'NONE',  ( -44.16309181155857999, 474.4948905683720000, 6.410867750099241924 ) ) ;
#14346=LINE ( 'NONE', #6407, #19663 ) ;
#14347=CARTESIAN_POINT ( 'NONE',  ( -45.64106924314019409, 411.0573905765656377, -11.32908994701042715 ) ) ;
#14349=CARTESIAN_POINT ( 'NONE',  ( -8.685887942688546914, 367.3073905765656377, -3.978247347592740013 ) ) ;
#14351=CARTESIAN_POINT ( 'NONE',  ( -8.685887942688710339, 256.9948905765655809, -2.449293598294705724E-15 ) ) ;
#14355=CARTESIAN_POINT ( 'NONE',  ( -17.35679799567827786, 240.6823905601784759, 16.95518130045146421 ) ) ;
#14357=CARTESIAN_POINT ( 'NONE',  ( -45.43829269268871940, 435.3698905683720000, 0.000000000000000000 ) ) ;
#14359=CARTESIAN_POINT ( 'NONE',  ( -22.27502019258946220, 258.4948905683720568, 15.47720386886985189 ) ) ;
#14361=VERTEX_POINT ( 'NONE', #4916 ) ;
#14363=CARTESIAN_POINT ( 'NONE',  ( -48.68588794268873698, 573.2448905601785327, 0.000000000000000000 ) ) ;
#14365=CARTESIAN_POINT ( 'NONE',  ( -38.17536295476246266, 456.9323905683720000, 14.20200298773971781 ) ) ;
#14366=CARTESIAN_POINT ( 'NONE',  ( -8.685887942688706786, 226.9948905765656377, -2.449293598294705724E-15 ) ) ;
#14367=ORIENTED_EDGE ( 'NONE', *, *, #11991, .T. ) ;
#14368=CARTESIAN_POINT ( 'NONE',  ( -40.01497788969913927, 365.6823905601784190, -16.95518130045146421 ) ) ;
#14369=CARTESIAN_POINT ( 'NONE',  ( -32.01814843081343298, 246.0573905683720000, 16.75240474999999307 ) ) ;
#14371=CARTESIAN_POINT ( 'NONE',  ( -16.84014894278201169, 530.1198905683720568, -11.84573899990672707 ) ) ;
#14373=CARTESIAN_POINT ( 'NONE',  ( -14.54375231895778420, 468.2448905765656377, -14.14213562373094746 ) ) ;
#14377=CARTESIAN_POINT ( 'NONE',  ( -39.74795651491226067, 224.0159561153923562, -12.62940942758988250 ) ) ;
#14379=CARTESIAN_POINT ( 'NONE',  ( -19.19641293061497223, 230.4323905683720000, -14.20200298773971603 ) ) ;
#14380=CARTESIAN_POINT ( 'NONE',  ( -22.27502019258947286, 318.4948905683720000, 15.47720386886985189 ) ) ;
#14383=CARTESIAN_POINT ( 'NONE',  ( -16.84014894278198327, 301.6198905683720000, -11.84573899990672707 ) ) ;
#14384=CARTESIAN_POINT ( 'NONE',  ( -14.48388495494899963, 377.9323905683720000, 9.489475012073732785 ) ) ;
#14385=CARTESIAN_POINT ( 'NONE',  ( -11.93348319268874036, 520.3698905683720568, -2.051577885510841163E-15 ) ) ;
#14387=CARTESIAN_POINT ( 'NONE',  ( -14.54375231895776999, 390.9948905601784759, 14.14213562373094568 ) ) ;
#14388=CARTESIAN_POINT ( 'NONE',  ( -42.82802356641964536, 230.7448905765656093, -14.14213562373094746 ) ) ;
#14391=CARTESIAN_POINT ( 'NONE',  ( -28.68588794268873343, 492.8698905683720568, -16.75240474999999307 ) ) ;
#14394=CARTESIAN_POINT ( 'NONE',  ( -38.17536295476244845, 313.8073905683720000, -14.20200298773971426 ) ) ;
#14395=CARTESIAN_POINT ( 'NONE',  ( -16.84014894278198682, 320.1198905683720568, -11.84573899990672707 ) ) ;
#14396=( BOUNDED_CURVE ( )  B_SPLINE_CURVE ( 2, ( #18304, #8457, #6731, #6834, #13450, #1557, #5218, #16488, #11817, #5112, #16701, #14760, #47, #3600, #15186, #21344, #19934 ),
 .UNSPECIFIED., .F., .T. ) 
 B_SPLINE_CURVE_WITH_KNOTS ( ( 3, 2, 2, 2, 2, 2, 2, 2, 3 ),
 ( 0.1718750000000001665, 0.1738281250000001665, 0.1757812500000001665, 0.1777343750000001665, 0.1796875000000001665, 0.1816406250000001665, 0.1835937500000001665, 0.1855468750000001665, 0.1875000000000001665 ),
 .UNSPECIFIED. ) 
 CURVE ( )  GEOMETRIC_REPRESENTATION_ITEM ( )  RATIONAL_B_SPLINE_CURVE ( ( 0.9999999999999983347, 0.9807852804032320959, 1.000000000000000000, 0.9807852804032304306, 1.000000000000000000, 0.9807852804032304306, 1.000000000000000000, 0.9807852804032304306, 1.000000000000000000, 0.9807852804032304306, 1.000000000000000000, 0.9807852804032304306, 1.000000000000000000, 0.9807852804032304306, 1.000000000000000000, 0.9807852804032287652, 1.000000000000001554 ) ) 
 REPRESENTATION_ITEM ( '' )  );
#14398=CARTESIAN_POINT ( 'NONE',  ( -48.68588794268870146, 271.6823905765656946, -3.978247347593158345 ) ) ;
#14402=CARTESIAN_POINT ( 'NONE',  ( -42.88789093042844058, 406.3073905683719431, 9.489475012073736337 ) ) ;
#14403=EDGE_CURVE ( 'NONE', #20734, #4181, #19673, .T. ) ;
#14405=CARTESIAN_POINT ( 'NONE',  ( -36.33955658999050797, 335.3698905601784759, -18.47759065022572855 ) ) ;
#14406=DIRECTION ( 'NONE',  ( -1.191790137725560488E-16, 1.000000000000000000, -0.000000000000000000 ) ) ;
#14407=CARTESIAN_POINT ( 'NONE',  ( -8.685887942688399477, 507.3073905765655809, -3.978247347592341221 ) ) ;
#14409=CARTESIAN_POINT ( 'NONE',  ( -16.84014894278200103, 440.1198905683720568, -11.84573899990672707 ) ) ;
#14412=CARTESIAN_POINT ( 'NONE',  ( -45.64106924314020119, 456.3073905601785327, -11.32908994701042715 ) ) ;
#14417=CARTESIAN_POINT ( 'NONE',  ( -11.73070664223724613, 323.1823905601784190, -11.32908994701042715 ) ) ;
#14418=CARTESIAN_POINT ( 'NONE',  ( -8.685887942688724550, 376.9948905765655809, -2.449293598294705724E-15 ) ) ;
#14419=CARTESIAN_POINT ( 'NONE',  ( -42.88789093042843348, 354.4323905683720568, -9.489475012073734561 ) ) ;
#14422=CARTESIAN_POINT ( 'NONE',  ( -8.685887942688740537, 507.3073905765656377, -3.978247347593165895 ) ) ;
#14423=CARTESIAN_POINT ( 'NONE',  ( -28.68588794268871922, 381.3698905683720568, -16.75240474999999307 ) ) ;
#14425=CARTESIAN_POINT ( 'NONE',  ( -45.43829269268871940, 414.1823905683720000, 3.332260488124734632 ) ) ;
#14427=CARTESIAN_POINT ( 'NONE',  ( -17.35679799567828852, 325.4323905765656946, 16.95518130045146421 ) ) ;
#14428=CARTESIAN_POINT ( 'NONE',  ( -28.68588794268874054, 573.2448905601785327, 0.000000000000000000 ) ) ;
#14429=CARTESIAN_POINT ( 'NONE',  ( -42.88789093042842637, 294.8073905683720000, 9.489475012073734561 ) ) ;
#14430=CARTESIAN_POINT ( 'NONE',  ( -45.43829269268871940, 455.6823905683720000, 3.332260488124734632 ) ) ;
#14431=CARTESIAN_POINT ( 'NONE',  ( -10.20829729246299777, 461.6198905601784759, 7.653668647301790529 ) ) ;
#14434=CARTESIAN_POINT ( 'NONE',  ( -45.43829269268870519, 375.6823905683720000, 3.332260488124734632 ) ) ;
#14435=CARTESIAN_POINT ( 'NONE',  ( -13.20868407381887621, 498.2448905683720000, 6.410867750099229490 ) ) ;
#14436=CARTESIAN_POINT ( 'NONE',  ( -21.03221929538692692, 510.3698905601785896, 18.47759065022572500 ) ) ;
#14437=CARTESIAN_POINT ( 'NONE',  ( -45.43829269268870519, 313.8698905683720000, 0.000000000000000000 ) ) ;
#14440=CARTESIAN_POINT ( 'NONE',  ( -14.54375231895778953, 523.4948905601785327, -14.14213562373094746 ) ) ;
#14443=CARTESIAN_POINT ( 'NONE',  ( -38.17536295476245556, 426.9323905683720000, 14.20200298773971781 ) ) ;
#14444=CARTESIAN_POINT ( 'NONE',  ( -47.16347859291445133, 392.6198905765655809, 7.653668647301805628 ) ) ;
#14446=CARTESIAN_POINT ( 'NONE',  ( -13.20868407381887089, 439.4948905683720568, -6.410867750099233042 ) ) ;
#14447=VERTEX_POINT ( 'NONE', #6637 ) ;
#14448=CARTESIAN_POINT ( 'NONE',  ( -19.19641293061499354, 467.3073905683721136, 14.20200298773971426 ) ) ;
#14450=CARTESIAN_POINT ( 'NONE',  ( -48.68588794268871567, 391.9948905765656377, 0.000000000000000000 ) ) ;
#14454=CARTESIAN_POINT ( 'NONE',  ( -14.54375231895775400, 255.7448905765656377, 14.14213562373094568 ) ) ;
#14457=CARTESIAN_POINT ( 'NONE',  ( -17.35679799567828141, 253.8073905601784759, -16.95518130045146421 ) ) ;
#14458=CARTESIAN_POINT ( 'NONE',  ( -37.43746952852602305, 223.9102039777116602, 17.72958622188000533 ) ) ;
#14459=CARTESIAN_POINT ( 'NONE',  ( -38.17536295476246266, 423.8073905683720568, -14.20200298773971426 ) ) ;
#14461=CARTESIAN_POINT ( 'NONE',  ( -16.84014894278197616, 241.6198905683720284, -11.84573899990672707 ) ) ;
#14466=CARTESIAN_POINT ( 'NONE',  ( -40.53162694259545162, 466.6198905683720000, 11.84573899990672885 ) ) ;
#14467=CARTESIAN_POINT ( 'NONE',  ( -24.70764059509553334, 234.8073905765656093, 19.99999999999998934 ) ) ;
#14471=CARTESIAN_POINT ( 'NONE',  ( -19.19641293061496512, 227.3073905683720000, 14.20200298773971426 ) ) ;
#14473=CARTESIAN_POINT ( 'NONE',  ( -11.93348319268874214, 529.1823905683720568, -3.332260488124732856 ) ) ;
#14475=CARTESIAN_POINT ( 'NONE',  ( -11.73070664223726034, 447.9323905765656946, -11.32908994701042715 ) ) ;
#14476=CARTESIAN_POINT ( 'NONE',  ( -10.20829729246298356, 351.6198905601784759, 7.653668647301790529 ) ) ;
#14479=DIRECTION ( 'NONE',  ( -1.000000000000000000, 0.000000000000000000, 0.000000000000000000 ) ) ;
#14481=EDGE_CURVE ( 'NONE', #4866, #19427, #13680, .T. ) ;
#14483=CARTESIAN_POINT ( 'NONE',  ( -32.01814843081343298, 236.0573905683720284, 16.75240474999999307 ) ) ;
#14484=CARTESIAN_POINT ( 'NONE',  ( -38.17536295476244135, 326.9323905683720568, 14.20200298773971781 ) ) ;
#14487=CARTESIAN_POINT ( 'NONE',  ( -32.01814843081344009, 313.1823905683720000, -16.75240474999999307 ) ) ;
#14488=CARTESIAN_POINT ( 'NONE',  ( -45.43829269268870519, 373.5573905683720568, -3.332260488124726194 ) ) ;
#14489=CARTESIAN_POINT ( 'NONE',  ( -16.84014894278200458, 519.1198905683720568, 11.84573899990672530 ) ) ;
#14490=CARTESIAN_POINT ( 'NONE',  ( -14.54375231895777176, 373.4948905601784759, -14.14213562373094746 ) ) ;
#14494=CARTESIAN_POINT ( 'NONE',  ( -28.68588794268872633, 487.8698905683720568, 16.75240474999999307 ) ) ;
#14496=CARTESIAN_POINT ( 'NONE',  ( -44.16309181155855867, 274.4948905683720000, 6.410867750099241924 ) ) ;
#14498=CARTESIAN_POINT ( 'NONE',  ( -44.16309181155856578, 284.7448905683720568, -6.410867750099231266 ) ) ;
#14499=CARTESIAN_POINT ( 'NONE',  ( -19.19641293061497933, 317.3073905683720000, 14.20200298773971426 ) ) ;
#14500=CARTESIAN_POINT ( 'NONE',  ( -10.20829729246297468, 256.3698905765656377, 7.653668647301790529 ) ) ;
#14501=CARTESIAN_POINT ( 'NONE',  ( -14.54375231895778420, 473.4948905601785327, -14.14213562373094746 ) ) ;
#14502=CARTESIAN_POINT ( 'NONE',  ( -19.19641293061496867, 230.4323905683720000, -14.20200298773971603 ) ) ;
#14503=CARTESIAN_POINT ( 'NONE',  ( -18.67110661049051146, 223.9107902980306619, -17.31196565581893765 ) ) ;
#14504=CARTESIAN_POINT ( 'NONE',  ( -13.20868407381886023, 379.7448905683720000, 6.410867750099229490 ) ) ;
#14508=CARTESIAN_POINT ( 'NONE',  ( -42.88789093042844058, 434.8073905683720568, 9.489475012073736337 ) ) ;
#14511=CARTESIAN_POINT ( 'NONE',  ( -36.33955658999052218, 429.1198905601784759, 18.47759065022572500 ) ) ;
#14516=CARTESIAN_POINT ( 'NONE',  ( -8.685887942688715668, 322.5573905601784759, -3.978247347593165895 ) ) ;
#14517=CARTESIAN_POINT ( 'NONE',  ( -28.68588794268874054, 573.2448905601785327, 0.000000000000000000 ) ) ;
#14518=EDGE_CURVE ( 'NONE', #14361, #6325, #4035, .T. ) ;
#14519=CARTESIAN_POINT ( 'NONE',  ( -32.01814843081344719, 343.1823905683721136, -16.75240474999999307 ) ) ;
#14520=CARTESIAN_POINT ( 'NONE',  ( -40.01497788969914637, 493.5573905765655809, 16.95518130045146776 ) ) ;
#14521=CARTESIAN_POINT ( 'NONE',  ( -14.48388495494899963, 377.9323905683720000, 9.489475012073732785 ) ) ;
#14522=CARTESIAN_POINT ( 'NONE',  ( -40.53162694259542320, 224.1198905683720000, -11.84573899990672707 ) ) ;
#14523=CARTESIAN_POINT ( 'NONE',  ( -25.35362745456399480, 391.0573905683720568, -16.75240474999999307 ) ) ;
#14524=CARTESIAN_POINT ( 'NONE',  ( -48.68588794268870146, 321.6823905765656377, -3.978247347593158345 ) ) ;
#14526=CARTESIAN_POINT ( 'NONE',  ( -38.17536295476244845, 282.3073905683720000, -14.20200298773971426 ) ) ;
#14528=CARTESIAN_POINT ( 'NONE',  ( -44.16309181155857999, 434.7448905683720000, -6.410867750099231266 ) ) ;
#14530=CARTESIAN_POINT ( 'NONE',  ( -40.01497788969913216, 285.6823905601784759, -16.95518130045146421 ) ) ;
#14533=CARTESIAN_POINT ( 'NONE',  ( -44.16309181155856578, 355.9948905683720000, 6.410867750099241924 ) ) ;
#14534=CARTESIAN_POINT ( 'NONE',  ( -28.68588794268872988, 506.3698905683720000, 16.75240474999999307 ) ) ;
#14535=CARTESIAN_POINT ( 'NONE',  ( -10.20829729246300310, 501.6198905601785327, 7.653668647301790529 ) ) ;
#14536=CARTESIAN_POINT ( 'NONE',  ( -45.43829269268869808, 324.1823905683720000, 3.332260488124734632 ) ) ;
#14537=ORIENTED_EDGE ( 'NONE', *, *, #867, .F. ) ;
#14540=EDGE_LOOP ( 'NONE', ( #16758, #4955, #5239, #18354 ) ) ;
#14542=CARTESIAN_POINT ( 'NONE',  ( -11.93348319268872970, 430.0573905683721136, 3.332260488124728859 ) ) ;
#14543=CARTESIAN_POINT ( 'NONE',  ( -8.685887942688799157, 236.6823905765655809, 3.978247347593374172 ) ) ;
#14545=CARTESIAN_POINT ( 'NONE',  ( -45.43829269268872650, 453.8698905683720000, 0.000000000000000000 ) ) ;
#14547=VECTOR ( 'NONE', #9374, 1000.000000000000000 ) ;
#14548=CARTESIAN_POINT ( 'NONE',  ( -42.88789093042844769, 454.8073905683720568, 9.489475012073734561 ) ) ;
#14551=CARTESIAN_POINT ( 'NONE',  ( -10.20829729246298712, 377.6198905765655809, -7.653668647301794969 ) ) ;
#14556=CARTESIAN_POINT ( 'NONE',  ( -45.43829269268872650, 515.6823905683720568, 3.332260488124734632 ) ) ;
#14560=CARTESIAN_POINT ( 'NONE',  ( -8.685887942688708563, 252.2448905601784475, -2.449293598294705724E-15 ) ) ;
#14561=CARTESIAN_POINT ( 'NONE',  ( -41.47555434389672513, 223.9102039777117739, 14.04716863791190917 ) ) ;
#14562=CARTESIAN_POINT ( 'NONE',  ( -11.93348319268872615, 410.6823905683720000, -3.332260488124732856 ) ) ;
#14564=CARTESIAN_POINT ( 'NONE',  ( -19.19641293061496867, 258.8073905683720000, 14.20200298773971426 ) ) ;
#14566=ORIENTED_EDGE ( 'NONE', *, *, #6009, .F. ) ;
#14569=CARTESIAN_POINT ( 'NONE',  ( -45.43829269268872650, 455.6823905683720000, 3.332260488124734632 ) ) ;
#14570=CARTESIAN_POINT ( 'NONE',  ( -28.68588794268870146, 229.4948905765656377, -19.99999999999999289 ) ) ;
#14573=DIRECTION ( 'NONE',  ( -1.191790137725560488E-16, 1.000000000000000000, -0.000000000000000000 ) ) ;
#14574=CARTESIAN_POINT ( 'NONE',  ( -38.17536295476244135, 222.3073905683720284, -14.20200298773971426 ) ) ;
#14576=CARTESIAN_POINT ( 'NONE',  ( -44.16309181155859420, 523.2448905683719431, -6.410867750099231266 ) ) ;
#14578=CARTESIAN_POINT ( 'NONE',  ( -8.685887942688731655, 446.9948905765655809, -2.449293598294705724E-15 ) ) ;
#14581=CARTESIAN_POINT ( 'NONE',  ( -45.43829269268871229, 354.1823905683720568, 3.332260488124734632 ) ) ;
#14582=CARTESIAN_POINT ( 'NONE',  ( -17.35679799567829917, 455.4323905765655809, 16.95518130045146421 ) ) ;
#14583=LINE ( 'NONE', #16202, #18051 ) ;
#14585=( BOUNDED_CURVE ( )  B_SPLINE_CURVE ( 2, ( #7951, #17909, #13053, #11418, #3106, #14582, #10007, #14692, #11534, #21166, #18126, #4822, #9900, #16631, #6338, #19972, #16312 ),
 .UNSPECIFIED., .F., .T. ) 
 B_SPLINE_CURVE_WITH_KNOTS ( ( 3, 2, 2, 2, 2, 2, 2, 2, 3 ),
 ( 0.2343750000000001943, 0.2363281250000001943, 0.2382812500000001943, 0.2402343750000001943, 0.2421875000000002220, 0.2441406250000002220, 0.2460937500000002220, 0.2480468750000002220, 0.2500000000000002220 ),
 .UNSPECIFIED. ) 
 CURVE ( )  GEOMETRIC_REPRESENTATION_ITEM ( )  RATIONAL_B_SPLINE_CURVE ( ( 0.9999999999999981126, 0.9807852804032323180, 1.000000000000000000, 0.9807852804032304306, 1.000000000000000000, 0.9807852804032304306, 1.000000000000000000, 0.9807852804032304306, 1.000000000000000000, 0.9807852804032304306, 1.000000000000000000, 0.9807852804032304306, 1.000000000000000000, 0.9807852804032304306, 1.000000000000000000, 0.9807852804032282101, 1.000000000000002220 ) ) 
 REPRESENTATION_ITEM ( '' )  );
#14588=CARTESIAN_POINT ( 'NONE',  ( -32.01814843081344009, 323.1823905683720000, -16.75240474999999307 ) ) ;
#14589=FACE_OUTER_BOUND ( 'NONE', #13528, .T. ) ;
#14590=CARTESIAN_POINT ( 'NONE',  ( -36.33955658999051508, 379.1198905601784759, 18.47759065022572500 ) ) ;
#14593=CARTESIAN_POINT ( 'NONE',  ( -13.20868407381885490, 310.9948905683720568, -6.410867750099233042 ) ) ;
#14594=CARTESIAN_POINT ( 'NONE',  ( -44.16309181155856578, 364.4948905683720568, 6.410867750099241924 ) ) ;
#14595=CARTESIAN_POINT ( 'NONE',  ( -40.53162694259545873, 516.6198905683720568, 11.84573899990672885 ) ) ;
#14596=CARTESIAN_POINT ( 'NONE',  ( -47.16347859291444422, 366.6198905601784759, -7.653668647301793193 ) ) ;
#14600=CARTESIAN_POINT ( 'NONE',  ( -11.93348319268873681, 490.6823905683720568, -3.332260488124732856 ) ) ;
#14601=CARTESIAN_POINT ( 'NONE',  ( -13.20868407381884957, 288.2448905683720000, 6.410867750099229490 ) ) ;
#14603=CARTESIAN_POINT ( 'NONE',  ( -45.43829269268870519, 285.0573905683720568, -3.332260488124726638 ) ) ;
#14604=CARTESIAN_POINT ( 'NONE',  ( -28.68588794268871212, 321.3698905683720568, -16.75240474999999307 ) ) ;
#14606=CARTESIAN_POINT ( 'NONE',  ( -28.68588794268870501, 262.8698905683720000, -16.75240474999999307 ) ) ;
#14607=CARTESIAN_POINT ( 'NONE',  ( -36.33955658999050087, 263.8698905765656377, 18.47759065022572500 ) ) ;
#14608=FACE_OUTER_BOUND ( 'NONE', #21151, .T. ) ;
#14610=FACE_OUTER_BOUND ( 'NONE', #6649, .T. ) ;
#14611=CARTESIAN_POINT ( 'NONE',  ( -13.20868407381886200, 370.9948905683720568, -6.410867750099233042 ) ) ;
#14614=CARTESIAN_POINT ( 'NONE',  ( -47.16347859291445843, 461.3698905765656377, -7.653668647301793193 ) ) ;
#14618=CARTESIAN_POINT ( 'NONE',  ( -14.48388495494900496, 419.8073905683720000, -9.489475012073736337 ) ) ;
#14619=DIRECTION ( 'NONE',  ( -1.000000000000000000, 0.000000000000000000, 0.000000000000000000 ) ) ;
#14621=CARTESIAN_POINT ( 'NONE',  ( -40.01497788969913927, 428.8073905601784759, 16.95518130045146776 ) ) ;
#14627=CARTESIAN_POINT ( 'NONE',  ( -14.54375231895776466, 313.4948905601784759, -14.14213562373094746 ) ) ;
#14629=CARTESIAN_POINT ( 'NONE',  ( -25.35362745456399125, 352.5573905683721136, -16.75240474999999307 ) ) ;
#14630=CARTESIAN_POINT ( 'NONE',  ( -36.33955658999052929, 510.1198905765655809, -18.47759065022572855 ) ) ;
#14631=CARTESIAN_POINT ( 'NONE',  ( -22.27502019258949062, 390.7448905683720000, -15.47720386886985544 ) ) ;
#14632=CARTESIAN_POINT ( 'NONE',  ( -16.84014894278196905, 229.1198905683720000, 11.84573899990672530 ) ) ;
#14634=CARTESIAN_POINT ( 'NONE',  ( -13.20868407381886023, 378.2448905683720000, 6.410867750099229490 ) ) ;
#14635=CARTESIAN_POINT ( 'NONE',  ( -11.73070664223724258, 326.0573905765656946, 11.32908994701042005 ) ) ;
#14637=CARTESIAN_POINT ( 'NONE',  ( -42.88789093042842637, 284.8073905683720568, 9.489475012073734561 ) ) ;
#14639=CARTESIAN_POINT ( 'NONE',  ( -42.88789093042844058, 444.4323905683720568, -9.489475012073736337 ) ) ;
#14644=CARTESIAN_POINT ( 'NONE',  ( -19.19641293061498288, 348.8073905683720000, 14.20200298773971426 ) ) ;
#14645=CARTESIAN_POINT ( 'NONE',  ( -13.20868407381887444, 479.4948905683720000, -6.410867750099233042 ) ) ;
#14647=CARTESIAN_POINT ( 'NONE',  ( -10.20829729246299955, 482.8698905601784759, -7.653668647301794969 ) ) ;
#14648=CARTESIAN_POINT ( 'NONE',  ( -35.09675569278794427, 315.7448905683720000, 15.47720386886985366 ) ) ;
#14649=ORIENTED_EDGE ( 'NONE', *, *, #6915, .F. ) ;
#14655=CARTESIAN_POINT ( 'NONE',  ( -11.93348319268872615, 400.3698905683720000, -2.051577885510841163E-15 ) ) ;
#14656=CARTESIAN_POINT ( 'NONE',  ( -21.03221929538691271, 395.1198905765656377, 18.47759065022572500 ) ) ;
#14658=CARTESIAN_POINT ( 'NONE',  ( -44.16309181155857999, 443.2448905683720000, -6.410867750099231266 ) ) ;
#14659=CARTESIAN_POINT ( 'NONE',  ( -40.53162694259544452, 445.1198905683720568, 11.84573899990672885 ) ) ;
#14662=CARTESIAN_POINT ( 'NONE',  ( -24.70764059509556532, 379.1823905765656946, -19.99999999999999289 ) ) ;
#14663=PLANE ( 'NONE',  #14153 ) ;
#14664=CARTESIAN_POINT ( 'NONE',  ( -24.70764059509556176, 389.1823905765656946, -19.99999999999999289 ) ) ;
#14668=CARTESIAN_POINT ( 'NONE',  ( -19.19641293061500065, 491.9323905683720000, -14.20200298773971603 ) ) ;
#14672=CARTESIAN_POINT ( 'NONE',  ( -10.20829729246300488, 521.6198905601785327, 7.653668647301790529 ) ) ;
#14674=CARTESIAN_POINT ( 'NONE',  ( -45.43829269268871229, 405.6823905683720568, 3.332260488124734632 ) ) ;
#14676=CARTESIAN_POINT ( 'NONE',  ( -48.68588794268872988, 536.9323905601785327, -3.978247347593158345 ) ) ;
#14678=CARTESIAN_POINT ( 'NONE',  ( -48.68588794268880804, 422.3073905765656377, 3.978247347592954952 ) ) ;
#14680=CARTESIAN_POINT ( 'NONE',  ( -44.16309181155858710, 454.7448905683720568, -6.410867750099231266 ) ) ;
#14681=CARTESIAN_POINT ( 'NONE',  ( -19.81322276830274731, 218.7662462910128340, -17.97266575622176532 ) ) ;
#14684=CARTESIAN_POINT ( 'NONE',  ( -43.20717515250593266, 208.4480206960199666, 3.766779594902113892 ) ) ;
#14685=CARTESIAN_POINT ( 'NONE',  ( -28.68588794268873343, 527.8698905683720568, 16.75240474999999307 ) ) ;
#14687=CARTESIAN_POINT ( 'NONE',  ( -19.19641293061500065, 510.4323905683720000, -14.20200298773971603 ) ) ;
#14689=CARTESIAN_POINT ( 'NONE',  ( -24.70764059509557242, 439.1823905765655809, -19.99999999999999289 ) ) ;
#14690=CARTESIAN_POINT ( 'NONE',  ( -17.35679799567829562, 358.5573905765655809, -16.95518130045146421 ) ) ;
#14692=CARTESIAN_POINT ( 'NONE',  ( -24.70764059509555821, 454.8073905765655809, 19.99999999999998934 ) ) ;
#14694=CARTESIAN_POINT ( 'NONE',  ( -28.68588794268874054, 573.2448905601785327, 0.000000000000000000 ) ) ;
#14695=CARTESIAN_POINT ( 'NONE',  ( -42.88789093042841927, 234.8073905683720284, 9.489475012073736337 ) ) ;
#14696=CARTESIAN_POINT ( 'NONE',  ( -28.68588794268870856, 312.8698905683720000, -16.75240474999999307 ) ) ;
#14698=CARTESIAN_POINT ( 'NONE',  ( -17.35679799567827786, 260.6823905601785327, 16.95518130045146421 ) ) ;
#14700=CARTESIAN_POINT ( 'NONE',  ( -35.09675569278794427, 307.2448905683720000, 15.47720386886985366 ) ) ;
#14701=EDGE_CURVE ( 'NONE', #19418, #7992, #16789, .T. ) ;
#14702=CARTESIAN_POINT ( 'NONE',  ( -25.35362745456400191, 528.1823905683720568, 16.75240474999998952 ) ) ;
#14703=CARTESIAN_POINT ( 'NONE',  ( -24.70764059509555111, 360.0573905601785327, 19.99999999999998934 ) ) ;
#14704=CARTESIAN_POINT ( 'NONE',  ( -8.685887942688717445, 312.2448905601784759, -2.449293598294705724E-15 ) ) ;
#14706=CARTESIAN_POINT ( 'NONE',  ( -32.01814843081346140, 477.5573905683720568, 16.75240474999999307 ) ) ;
#14708=CARTESIAN_POINT ( 'NONE',  ( -25.35362745456397349, 286.6823905683720568, 16.75240474999998952 ) ) ;
#14710=( BOUNDED_CURVE ( )  B_SPLINE_CURVE ( 2, ( #19492, #19070, #11046, #7698, #14327, #11262, #17657, #9532, #6074, #7799, #16150, #1330, #20907, #21115, #7902, #12686, #19280 ),
 .UNSPECIFIED., .F., .T. ) 
 B_SPLINE_CURVE_WITH_KNOTS ( ( 3, 2, 2, 2, 2, 2, 2, 2, 3 ),
 ( 0.5156250000000002220, 0.5175781250000002220, 0.5195312500000002220, 0.5214843750000002220, 0.5234375000000002220, 0.5253906250000003331, 0.5273437500000003331, 0.5292968750000003331, 0.5312500000000003331 ),
 .UNSPECIFIED. ) 
 CURVE ( )  GEOMETRIC_REPRESENTATION_ITEM ( )  RATIONAL_B_SPLINE_CURVE ( ( 0.9999999999999977796, 0.9807852804032326510, 1.000000000000000000, 0.9807852804032304306, 1.000000000000000000, 0.9807852804032304306, 1.000000000000000000, 0.9807852804032304306, 1.000000000000000000, 0.9807852804032304306, 1.000000000000000000, 0.9807852804032304306, 1.000000000000000000, 0.9807852804032304306, 1.000000000000000000, 0.9807852804032270999, 1.000000000000003331 ) ) 
 REPRESENTATION_ITEM ( '' )  );
#14711=CARTESIAN_POINT ( 'NONE',  ( -35.09675569278794427, 277.2448905683720568, 15.47720386886985366 ) ) ;
#14712=CARTESIAN_POINT ( 'NONE',  ( -32.01814843081344009, 311.6823905683720568, -16.75240474999999307 ) ) ;
#14713=CARTESIAN_POINT ( 'NONE',  ( -17.35679799567828852, 268.5573905765656946, -16.95518130045146421 ) ) ;
#14716=CARTESIAN_POINT ( 'NONE',  ( -45.43829269268870519, 385.6823905683720000, 3.332260488124734632 ) ) ;
#14718=DIRECTION ( 'NONE',  ( -1.191790137725560488E-16, 1.000000000000000000, -0.000000000000000000 ) ) ;
#14719=CARTESIAN_POINT ( 'NONE',  ( -36.33955658999052218, 460.1198905765655809, -18.47759065022572855 ) ) ;
#14720=CARTESIAN_POINT ( 'NONE',  ( -24.70764059509554755, 269.1823905765655809, -19.99999999999999289 ) ) ;
#14721=CARTESIAN_POINT ( 'NONE',  ( -35.09675569278795138, 421.9948905683720000, -15.47720386886985544 ) ) ;
#14724=CARTESIAN_POINT ( 'NONE',  ( -24.70764059509555821, 420.0573905601784190, 19.99999999999998934 ) ) ;
#14728=CARTESIAN_POINT ( 'NONE',  ( -10.20829729246297823, 301.6198905601784759, 7.653668647301790529 ) ) ;
#14729=CARTESIAN_POINT ( 'NONE',  ( -42.83990393396077678, 205.8064044967071879, -4.966739033517835189 ) ) ;
#14731=CARTESIAN_POINT ( 'NONE',  ( -13.20868407381885845, 340.9948905683720000, -6.410867750099233042 ) ) ;
#14732=CARTESIAN_POINT ( 'NONE',  ( -14.54375231895778775, 508.2448905765656377, -14.14213562373094746 ) ) ;
#14733=CARTESIAN_POINT ( 'NONE',  ( -42.88789093042843348, 374.8073905683720568, 9.489475012073736337 ) ) ;
#14734=CARTESIAN_POINT ( 'NONE',  ( -11.93348319268870661, 230.0573905683720284, 3.332260488124728415 ) ) ;
#14735=CARTESIAN_POINT ( 'NONE',  ( -28.68588794268871567, 386.3698905683720568, 16.75240474999999307 ) ) ;
#14737=AXIS2_PLACEMENT_3D ( 'NONE', #5755, #12366, #5545 ) ;
#14738=CARTESIAN_POINT ( 'NONE',  ( -48.68588794268870856, 332.3073905765655809, 3.978247347593168115 ) ) ;
#14740=CARTESIAN_POINT ( 'NONE',  ( -45.43829269268870519, 284.1823905683720568, 3.332260488124734632 ) ) ;
#14742=CARTESIAN_POINT ( 'NONE',  ( -44.16309181155857289, 445.9948905683720568, 6.410867750099241924 ) ) ;
#14746=CARTESIAN_POINT ( 'NONE',  ( -14.54375231895778420, 500.9948905601784190, 14.14213562373094568 ) ) ;
#14749=CARTESIAN_POINT ( 'NONE',  ( -45.43829269268870519, 345.0573905683720568, -3.332260488124726194 ) ) ;
#14750=CARTESIAN_POINT ( 'NONE',  ( -16.84014894278200103, 487.6198905683720000, 11.84573899990672530 ) ) ;
#14752=CARTESIAN_POINT ( 'NONE',  ( -21.03221929538694113, 494.1198905601784759, -18.47759065022572855 ) ) ;
#14753=CARTESIAN_POINT ( 'NONE',  ( -14.48388495494899253, 299.8073905683720000, -9.489475012073736337 ) ) ;
#14755=ORIENTED_EDGE ( 'NONE', *, *, #19444, .F. ) ;
#14759=CARTESIAN_POINT ( 'NONE',  ( -45.43829269268871940, 405.0573905683721136, -3.332260488124726638 ) ) ;
#14760=CARTESIAN_POINT ( 'NONE',  ( -40.01497788969914637, 478.8073905601785327, 16.95518130045146776 ) ) ;
#14761=CARTESIAN_POINT ( 'NONE',  ( -11.93348319268872970, 439.1823905683720000, -3.332260488124732856 ) ) ;
#14762=CARTESIAN_POINT ( 'NONE',  ( -19.19641293061499354, 440.4323905683720000, -14.20200298773971603 ) ) ;
#14763=CARTESIAN_POINT ( 'NONE',  ( -48.68588794268869435, 247.2448905601785043, 0.000000000000000000 ) ) ;
#14764=CARTESIAN_POINT ( 'NONE',  ( -21.03221929538692692, 378.8698905765656377, -18.47759065022572855 ) ) ;
#14766=CARTESIAN_POINT ( 'NONE',  ( -8.685887942688710339, 262.2448905601784759, -2.449293598294705724E-15 ) ) ;
#14769=CARTESIAN_POINT ( 'NONE',  ( -28.68588794268872633, 487.8698905683720568, 16.75240474999999307 ) ) ;
#14774=CARTESIAN_POINT ( 'NONE',  ( -44.16309181155857289, 405.9948905683720568, 6.410867750099241924 ) ) ;
#14776=CARTESIAN_POINT ( 'NONE',  ( -16.84014894278197616, 231.6198905683720000, -11.84573899990672707 ) ) ;
#14780=CARTESIAN_POINT ( 'NONE',  ( -45.43829269268871940, 435.3698905683720000, 0.000000000000000000 ) ) ;
#14781=CARTESIAN_POINT ( 'NONE',  ( -40.01497788969911795, 233.5573905765656093, 16.95518130045146776 ) ) ;
#14782=EDGE_CURVE ( 'NONE', #18799, #3040, #20250, .T. ) ;
#14786=CARTESIAN_POINT ( 'NONE',  ( -45.43829269268869808, 223.8698905683720284, 0.000000000000000000 ) ) ;
#14789=CARTESIAN_POINT ( 'NONE',  ( -42.88789093042845479, 514.8073905683720568, 9.489475012073734561 ) ) ;
#14791=DIRECTION ( 'NONE',  ( -1.191790137725560488E-16, 1.000000000000000000, -0.000000000000000000 ) ) ;
#14794=CARTESIAN_POINT ( 'NONE',  ( -21.03221929538693402, 438.8698905765656377, -18.47759065022572855 ) ) ;
#14797=CARTESIAN_POINT ( 'NONE',  ( -8.685887942688742314, 573.2448905601785327, 2.449293598294706119E-15 ) ) ;
#14800=CARTESIAN_POINT ( 'NONE',  ( -16.02813280578691391, 223.9102039777117739, 15.56881321685236763 ) ) ;
#14801=CARTESIAN_POINT ( 'NONE',  ( -43.68588794268870146, 200.1437886375729249, -0.3330356950053358633 ) ) ;
#14802=CARTESIAN_POINT ( 'NONE',  ( -45.43829269268869808, 325.6823905683721136, 3.332260488124734632 ) ) ;
#14804=FACE_BOUND ( 'NONE', #6423, .T. ) ;
#14805=CARTESIAN_POINT ( 'NONE',  ( -40.01497788969911795, 268.8073905601785327, 16.95518130045146776 ) ) ;
#14806=CARTESIAN_POINT ( 'NONE',  ( -48.68588794268870856, 341.9948905765656377, 0.000000000000000000 ) ) ;
#14807=CARTESIAN_POINT ( 'NONE',  ( -14.48388495494898898, 289.4323905683720000, 9.489475012073732785 ) ) ;
#14808=CARTESIAN_POINT ( 'NONE',  ( -42.88789093042845479, 524.4323905683720568, -9.489475012073734561 ) ) ;
#14809=CARTESIAN_POINT ( 'NONE',  ( -11.73070664223724968, 371.3073905601784759, 11.32908994701042005 ) ) ;
#14812=CARTESIAN_POINT ( 'NONE',  ( -11.93348319268873503, 480.0573905683720568, 3.332260488124728415 ) ) ;
#14814=CARTESIAN_POINT ( 'NONE',  ( -45.43829269268869808, 273.5573905683720000, -3.332260488124726194 ) ) ;
#14817=CARTESIAN_POINT ( 'NONE',  ( -44.16309181155856578, 274.7448905683720568, -6.410867750099231266 ) ) ;
#14818=CARTESIAN_POINT ( 'NONE',  ( -38.17536295476244135, 263.8073905683720568, -14.20200298773971426 ) ) ;
#14819=CARTESIAN_POINT ( 'NONE',  ( -17.35679799567828496, 248.5573905765656093, -16.95518130045146421 ) ) ;
#14821=CARTESIAN_POINT ( 'NONE',  ( -40.53162694259542320, 225.1198905683720000, 11.84573899990672885 ) ) ;
#14822=CARTESIAN_POINT ( 'NONE',  ( -28.68588794268870146, 266.3698905683720000, 16.75240474999999307 ) ) ;
#14823=CARTESIAN_POINT ( 'NONE',  ( -14.48388495494900141, 381.3073905683720568, -9.489475012073736337 ) ) ;
#14825=CARTESIAN_POINT ( 'NONE',  ( -8.685887942688580665, 457.3073905765655809, -3.978247347592792860 ) ) ;
#14828=CARTESIAN_POINT ( 'NONE',  ( -40.53162694259544452, 432.6198905683720000, -11.84573899990672707 ) ) ;
#14830=DIRECTION ( 'NONE',  ( -1.000000000000000000, 0.000000000000000000, 0.000000000000000000 ) ) ;
#14832=( BOUNDED_CURVE ( )  B_SPLINE_CURVE ( 2, ( #3350, #7985, #14614, #3245, #13085, #4854, #14719, #15043, #8198, #6579, #9931, #1409, #13308, #18153, #19780, #14825, #4967 ),
 .UNSPECIFIED., .F., .T. ) 
 B_SPLINE_CURVE_WITH_KNOTS ( ( 3, 2, 2, 2, 2, 2, 2, 2, 3 ),
 ( 0.2187500000000001943, 0.2207031250000001943, 0.2226562500000001943, 0.2246093750000001943, 0.2265625000000001943, 0.2285156250000001943, 0.2304687500000001943, 0.2324218750000001943, 0.2343750000000001943 ),
 .UNSPECIFIED. ) 
 CURVE ( )  GEOMETRIC_REPRESENTATION_ITEM ( )  RATIONAL_B_SPLINE_CURVE ( ( 0.9999999999999981126, 0.9807852804032323180, 1.000000000000000000, 0.9807852804032304306, 1.000000000000000000, 0.9807852804032304306, 1.000000000000000000, 0.9807852804032304306, 1.000000000000000000, 0.9807852804032304306, 1.000000000000000000, 0.9807852804032304306, 1.000000000000000000, 0.9807852804032304306, 1.000000000000000000, 0.9807852804032285432, 1.000000000000001998 ) ) 
 REPRESENTATION_ITEM ( '' )  );
#14833=CARTESIAN_POINT ( 'NONE',  ( -42.82802356641966668, 418.4948905601784759, 14.14213562373094923 ) ) ;
#14834=ORIENTED_EDGE ( 'NONE', *, *, #9030, .F. ) ;
#14835=ORIENTED_EDGE ( 'NONE', *, *, #9878, .T. ) ;
#14838=CARTESIAN_POINT ( 'NONE',  ( -36.33955658999050797, 299.1198905601785327, 18.47759065022572500 ) ) ;
#14841=CARTESIAN_POINT ( 'NONE',  ( -22.27502019258948351, 342.2448905683720568, -15.47720386886985544 ) ) ;
#14842=CARTESIAN_POINT ( 'NONE',  ( -47.16347859291445843, 492.6198905765656377, 7.653668647301805628 ) ) ;
#14843=CARTESIAN_POINT ( 'NONE',  ( -32.01814843081344719, 366.0573905683720000, 16.75240474999999307 ) ) ;
#14844=CARTESIAN_POINT ( 'NONE',  ( -36.33955658999050087, 310.1198905765656377, -18.47759065022572855 ) ) ;
#14846=CARTESIAN_POINT ( 'NONE',  ( -45.43829269268871229, 383.8698905683720000, 0.000000000000000000 ) ) ;
#14847=CARTESIAN_POINT ( 'NONE',  ( -47.16347859291443712, 301.3698905765655809, -7.653668647301793193 ) ) ;
#14850=CARTESIAN_POINT ( 'NONE',  ( -11.93348319268871016, 278.8698905683720000, -2.051577885510841163E-15 ) ) ;
#14851=CYLINDRICAL_SURFACE ( 'NONE', #9785, 19.99999999999999645 ) ;
#14852=CARTESIAN_POINT ( 'NONE',  ( -14.48388495494900496, 429.4323905683720000, 9.489475012073732785 ) ) ;
#14853=CARTESIAN_POINT ( 'NONE',  ( -14.54375231895776110, 283.4948905601784759, -14.14213562373094746 ) ) ;
#14854=CARTESIAN_POINT ( 'NONE',  ( -48.68588794268872988, 517.2448905601785327, 0.000000000000000000 ) ) ;
#14856=CARTESIAN_POINT ( 'NONE',  ( -48.68588794268871567, 447.2448905601785327, 0.000000000000000000 ) ) ;
#14857=CARTESIAN_POINT ( 'NONE',  ( -19.19641293061497933, 338.8073905683720000, 14.20200298773971426 ) ) ;
#14858=CARTESIAN_POINT ( 'NONE',  ( -25.35362745456399480, 486.6823905683720568, 16.75240474999998952 ) ) ;
#14859=EDGE_LOOP ( 'NONE', ( #12342, #5875, #2040, #7525 ) ) ;
#14860=CARTESIAN_POINT ( 'NONE',  ( -45.64106924314020119, 488.1823905601784759, 11.32908994701042715 ) ) ;
#14861=CARTESIAN_POINT ( 'NONE',  ( -45.43829269268869808, 304.1823905683720568, 3.332260488124734632 ) ) ;
#14868=CARTESIAN_POINT ( 'NONE',  ( -35.09675569278795848, 397.2448905683720568, 15.47720386886985366 ) ) ;
#14869=CARTESIAN_POINT ( 'NONE',  ( -47.16347859291444422, 376.6198905601784759, -7.653668647301793193 ) ) ;
#14870=CARTESIAN_POINT ( 'NONE',  ( -48.68588794268870146, 301.9948905765655809, 0.000000000000000000 ) ) ;
#14871=CARTESIAN_POINT ( 'NONE',  ( -32.01814843081345430, 416.0573905683720568, 16.75240474999999307 ) ) ;
#14872=CARTESIAN_POINT ( 'NONE',  ( -25.35362745456400191, 441.0573905683720000, -16.75240474999999307 ) ) ;
#14874=CARTESIAN_POINT ( 'NONE',  ( -24.70764059509555466, 374.8073905765656377, 19.99999999999998934 ) ) ;
#14877=CARTESIAN_POINT ( 'NONE',  ( -24.70764059509556532, 429.1823905765656946, -19.99999999999999289 ) ) ;
#14878=CARTESIAN_POINT ( 'NONE',  ( -8.685887942688742314, 573.2448905601785327, 2.449293598294706119E-15 ) ) ;
#14879=CARTESIAN_POINT ( 'NONE',  ( -19.19641293061500065, 501.9323905683720000, -14.20200298773971603 ) ) ;
#14880=LINE ( 'NONE', #4695, #9903 ) ;
#14882=CARTESIAN_POINT ( 'NONE',  ( -32.66413529028189089, 519.4323905601784190, 19.99999999999999289 ) ) ;
#14884=CARTESIAN_POINT ( 'NONE',  ( -14.48388495494900496, 401.3073905683720568, -9.489475012073736337 ) ) ;
#14886=CARTESIAN_POINT ( 'NONE',  ( -38.17536295476243424, 226.9323905683720000, 14.20200298773971781 ) ) ;
#14888=CARTESIAN_POINT ( 'NONE',  ( -28.68588794268872988, 516.3698905683720568, 16.75240474999999307 ) ) ;
#14890=CARTESIAN_POINT ( 'NONE',  ( -11.93348319268873148, 450.0573905683719431, 3.332260488124728859 ) ) ;
#14891=CARTESIAN_POINT ( 'NONE',  ( -19.19641293061500420, 520.4323905683720568, -14.20200298773971603 ) ) ;
#14895=CARTESIAN_POINT ( 'NONE',  ( -24.70764059509557597, 494.4323905601784190, -19.99999999999999289 ) ) ;
#14896=CARTESIAN_POINT ( 'NONE',  ( -11.93348319268874214, 530.3698905683720568, -2.051577885510841163E-15 ) ) ;
#14897=ORIENTED_EDGE ( 'NONE', *, *, #1250, .F. ) ;
#14898=CARTESIAN_POINT ( 'NONE',  ( -14.48388495494901562, 499.8073905683720568, -9.489475012073734561 ) ) ;
#14899=CARTESIAN_POINT ( 'NONE',  ( -36.33955658999052929, 489.1198905601785327, 18.47759065022572500 ) ) ;
#14901=CARTESIAN_POINT ( 'NONE',  ( -48.68588794268871567, 441.9948905765656377, 0.000000000000000000 ) ) ;
#14903=CARTESIAN_POINT ( 'NONE',  ( -8.685887942688456320, 357.3073905765655809, -3.978247347592526850 ) ) ;
#14906=DIRECTION ( 'NONE',  ( -1.191790137725560488E-16, 1.000000000000000000, -0.000000000000000000 ) ) ;
#14908=CARTESIAN_POINT ( 'NONE',  ( -43.60108677734861260, 200.4027425691367057, -1.621665263882683838 ) ) ;
#14910=CARTESIAN_POINT ( 'NONE',  ( -42.88789093042842637, 296.3073905683720000, 9.489475012073736337 ) ) ;
#14911=CARTESIAN_POINT ( 'NONE',  ( -24.70764059509555111, 274.4323905601784759, -19.99999999999999289 ) ) ;
#14913=CARTESIAN_POINT ( 'NONE',  ( -14.48388495494899075, 291.3073905683720568, -9.489475012073736337 ) ) ;
#14915=CARTESIAN_POINT ( 'NONE',  ( -32.01814843081345430, 497.5573905683720568, 16.75240474999999307 ) ) ;
#14916=CARTESIAN_POINT ( 'NONE',  ( -10.20829729246298534, 362.8698905601784759, -7.653668647301794969 ) ) ;
#14917=CARTESIAN_POINT ( 'NONE',  ( -47.16347859291443712, 316.6198905601784759, -7.653668647301793193 ) ) ;
#14919=CARTESIAN_POINT ( 'NONE',  ( -40.53162694259545162, 476.6198905683720000, 11.84573899990672885 ) ) ;
#14920=CARTESIAN_POINT ( 'NONE',  ( -32.01814843081344009, 276.0573905683720000, 16.75240474999999307 ) ) ;
#14922=VERTEX_POINT ( 'NONE', #10430 ) ;
#14923=CARTESIAN_POINT ( 'NONE',  ( -28.68588794268874054, 573.2448905601785327, 0.000000000000000000 ) ) ;
#14924=EDGE_CURVE ( 'NONE', #16434, #10903, #13629, .T. ) ;
#14925=CARTESIAN_POINT ( 'NONE',  ( -44.16309181155855867, 285.9948905683720000, 6.410867750099241924 ) ) ;
#14926=CARTESIAN_POINT ( 'NONE',  ( -40.01497788969912506, 240.4323905765656662, -16.95518130045146421 ) ) ;
#14931=CARTESIAN_POINT ( 'NONE',  ( -35.09675569278794427, 275.7448905683720568, 15.47720386886985366 ) ) ;
#14932=CARTESIAN_POINT ( 'NONE',  ( -35.09675569278795138, 387.2448905683720000, 15.47720386886985366 ) ) ;
#14934=CARTESIAN_POINT ( 'NONE',  ( -40.53162694259544452, 425.1198905683720000, 11.84573899990672885 ) ) ;
#14935=CARTESIAN_POINT ( 'NONE',  ( -28.68588794268871212, 339.4948905765656377, -19.99999999999999289 ) ) ;
#14937=CARTESIAN_POINT ( 'NONE',  ( -10.20829729246299244, 421.6198905601785327, 7.653668647301790529 ) ) ;
#14941=ORIENTED_EDGE ( 'NONE', *, *, #12793, .F. ) ;
#14942=CARTESIAN_POINT ( 'NONE',  ( -14.48388495494901917, 531.3073905683719431, -9.489475012073736337 ) ) ;
#14943=CARTESIAN_POINT ( 'NONE',  ( -45.64106924314017988, 308.1823905601785327, 11.32908994701042715 ) ) ;
#14945=CARTESIAN_POINT ( 'NONE',  ( -38.17536295476245556, 343.8073905683720000, -14.20200298773971426 ) ) ;
#14947=CARTESIAN_POINT ( 'NONE',  ( -45.64106924314020119, 491.0573905765655809, -11.32908994701042715 ) ) ;
#14948=CARTESIAN_POINT ( 'NONE',  ( -40.53162694259543741, 362.6198905683720000, -11.84573899990672707 ) ) ;
#14949=CARTESIAN_POINT ( 'NONE',  ( -40.53162694259544452, 392.6198905683720568, -11.84573899990672707 ) ) ;
#14950=CARTESIAN_POINT ( 'NONE',  ( -28.68588794268870856, 309.4948905765656377, -19.99999999999999289 ) ) ;
#14952=CARTESIAN_POINT ( 'NONE',  ( -13.20868407381884779, 268.2448905683720568, 6.410867750099229490 ) ) ;
#14953=CARTESIAN_POINT ( 'NONE',  ( -21.03221929538691981, 440.3698905601784759, 18.47759065022572500 ) ) ;
#14955=CARTESIAN_POINT ( 'NONE',  ( -14.48388495494900674, 431.3073905683719431, -9.489475012073736337 ) ) ;
#14956=CARTESIAN_POINT ( 'NONE',  ( -47.16347859291443712, 286.6198905601784759, -7.653668647301793193 ) ) ;
#14957=CARTESIAN_POINT ( 'NONE',  ( -42.82802356641967378, 498.4948905601784759, 14.14213562373094923 ) ) ;
#14959=( BOUNDED_CURVE ( )  B_SPLINE_CURVE ( 2, ( #2025, #8268, #6760, #10317, #511, #10427, #5251, #2123, #13273, #13694, #14899, #13595, #8593, #18338, #5350, #13485, #3526 ),
 .UNSPECIFIED., .F., .T. ) 
 B_SPLINE_CURVE_WITH_KNOTS ( ( 3, 2, 2, 2, 2, 2, 2, 2, 3 ),
 ( 0.1406250000000001388, 0.1425781250000001388, 0.1445312500000001388, 0.1464843750000001388, 0.1484375000000001388, 0.1503906250000001388, 0.1523437500000001388, 0.1542968750000001388, 0.1562500000000001388 ),
 .UNSPECIFIED. ) 
 CURVE ( )  GEOMETRIC_REPRESENTATION_ITEM ( )  RATIONAL_B_SPLINE_CURVE ( ( 0.9999999999999986677, 0.9807852804032317628, 1.000000000000000000, 0.9807852804032304306, 1.000000000000000000, 0.9807852804032304306, 1.000000000000000000, 0.9807852804032304306, 1.000000000000000000, 0.9807852804032304306, 1.000000000000000000, 0.9807852804032304306, 1.000000000000000000, 0.9807852804032304306, 1.000000000000000000, 0.9807852804032290983, 1.000000000000001332 ) ) 
 REPRESENTATION_ITEM ( '' )  );
#14961=CARTESIAN_POINT ( 'NONE',  ( -25.35362745456399125, 352.5573905683720568, -16.75240474999999307 ) ) ;
#14962=CARTESIAN_POINT ( 'NONE',  ( -35.09675569278795848, 481.9948905683720000, -15.47720386886985544 ) ) ;
#14964=CARTESIAN_POINT ( 'NONE',  ( -10.20829729246300133, 491.6198905601784759, 7.653668647301790529 ) ) ;
#14965=CARTESIAN_POINT ( 'NONE',  ( -25.35362745456397349, 296.6823905683720000, 16.75240474999998952 ) ) ;
#14967=CARTESIAN_POINT ( 'NONE',  ( -36.33955658999051508, 343.8698905765656377, 18.47759065022572500 ) ) ;
#14969=DIRECTION ( 'NONE',  ( -1.191790137725560488E-16, 1.000000000000000000, -0.000000000000000000 ) ) ;
#14972=CARTESIAN_POINT ( 'NONE',  ( -11.93348319268872615, 400.6823905683720000, -3.332260488124732856 ) ) ;
#14973=CARTESIAN_POINT ( 'NONE',  ( -42.82802356641965957, 375.9948905601784759, -14.14213562373094746 ) ) ;
#14975=CARTESIAN_POINT ( 'NONE',  ( -44.16309181155857999, 423.2448905683720568, -6.410867750099231266 ) ) ;
#14976=CARTESIAN_POINT ( 'NONE',  ( -14.48388495494898542, 259.4323905683720000, 9.489475012073732785 ) ) ;
#14977=CARTESIAN_POINT ( 'NONE',  ( -38.17536295476246977, 452.3073905683721136, -14.20200298773971426 ) ) ;
#14979=CARTESIAN_POINT ( 'NONE',  ( -28.68588794268871567, 399.7448905601784759, 19.99999999999999289 ) ) ;
#14980=CARTESIAN_POINT ( 'NONE',  ( -40.01497788969913216, 373.5573905765655809, 16.95518130045146776 ) ) ;
#14983=CARTESIAN_POINT ( 'NONE',  ( -48.68588794268871567, 431.9948905765656377, 0.000000000000000000 ) ) ;
#14985=CARTESIAN_POINT ( 'NONE',  ( -16.84014894278200458, 499.1198905683720000, 11.84573899990672530 ) ) ;
#14989=CARTESIAN_POINT ( 'NONE',  ( -36.33955658999053639, 519.1198905601785327, 18.47759065022572500 ) ) ;
#14992=CARTESIAN_POINT ( 'NONE',  ( -13.20868407381886556, 400.9948905683720568, -6.410867750099233042 ) ) ;
#14994=CARTESIAN_POINT ( 'NONE',  ( -21.25395633616651736, 222.1412455016325112, -15.05426537149049437 ) ) ;
#14995=CARTESIAN_POINT ( 'NONE',  ( -16.84014894278199037, 370.1198905683720000, -11.84573899990672707 ) ) ;
#14997=CARTESIAN_POINT ( 'NONE',  ( -42.88789093042845479, 524.8073905683720568, 9.489475012073736337 ) ) ;
#14999=CARTESIAN_POINT ( 'NONE',  ( -28.68588794268872277, 447.8698905683720000, 16.75240474999999307 ) ) ;
#15000=CARTESIAN_POINT ( 'NONE',  ( -45.43829269268873361, 523.8698905683720568, 0.000000000000000000 ) ) ;
#15003=CARTESIAN_POINT ( 'NONE',  ( -45.64106924314020119, 531.0573905765656946, -11.32908994701042538 ) ) ;
#15004=CARTESIAN_POINT ( 'NONE',  ( -32.01814843081346140, 486.0573905683721136, 16.75240474999999307 ) ) ;
#15006=CARTESIAN_POINT ( 'NONE',  ( -32.01814843081346140, 511.6823905683719431, -16.75240474999999307 ) ) ;
#15010=CARTESIAN_POINT ( 'NONE',  ( -24.70764059509556887, 429.1823905765657514, -19.99999999999999289 ) ) ;
#15017=CARTESIAN_POINT ( 'NONE',  ( -43.31820119254705759, 201.3816099220727835, -3.309203535948212149 ) ) ;
#15018=CARTESIAN_POINT ( 'NONE',  ( -14.48388495494899075, 299.4323905683720568, 9.489475012073732785 ) ) ;
#15020=CARTESIAN_POINT ( 'NONE',  ( -10.20829729246300666, 531.6198905601785327, 7.653668647301790529 ) ) ;
#15021=CARTESIAN_POINT ( 'NONE',  ( -8.685887942688710339, 262.5573905601784190, -3.978247347593165895 ) ) ;
#15024=CARTESIAN_POINT ( 'NONE',  ( -14.48388495494899075, 281.3073905683720000, -9.489475012073736337 ) ) ;
#15026=CARTESIAN_POINT ( 'NONE',  ( -13.20868407381887621, 509.7448905683720000, 6.410867750099229490 ) ) ;
#15029=CARTESIAN_POINT ( 'NONE',  ( -44.16309181155858710, 474.7448905683720568, -6.410867750099231266 ) ) ;
#15030=CARTESIAN_POINT ( 'NONE',  ( -36.33955658999051508, 410.1198905765656377, -18.47759065022572855 ) ) ;
#15031=CARTESIAN_POINT ( 'NONE',  ( -35.09675569278793716, 265.7448905683720000, 15.47720386886985366 ) ) ;
#15034=CARTESIAN_POINT ( 'NONE',  ( -11.93348319268871016, 270.6823905683719431, -3.332260488124732856 ) ) ;
#15035=CARTESIAN_POINT ( 'NONE',  ( -42.88789093042841927, 234.4323905683720000, -9.489475012073734561 ) ) ;
#15036=CARTESIAN_POINT ( 'NONE',  ( -48.68588794268869435, 241.9948905765656377, 0.000000000000000000 ) ) ;
#15037=CARTESIAN_POINT ( 'NONE',  ( -11.73070664223723902, 311.3073905601784759, 11.32908994701042005 ) ) ;
#15038=CARTESIAN_POINT ( 'NONE',  ( -45.64106924314017277, 236.3073905601784759, -11.32908994701042715 ) ) ;
#15039=DIRECTION ( 'NONE',  ( -1.191790137725560488E-16, 1.000000000000000000, -0.000000000000000000 ) ) ;
#15040=CARTESIAN_POINT ( 'NONE',  ( -14.48388495494898720, 259.8073905683720000, -9.489475012073736337 ) ) ;
#15041=CARTESIAN_POINT ( 'NONE',  ( -11.93348319268872260, 360.6823905683720568, -3.332260488124732856 ) ) ;
#15042=CARTESIAN_POINT ( 'NONE',  ( -48.68588794268872277, 507.2448905601785327, 0.000000000000000000 ) ) ;
#15043=CARTESIAN_POINT ( 'NONE',  ( -32.66413529028188378, 459.8073905765656946, -19.99999999999999289 ) ) ;
#15045=CARTESIAN_POINT ( 'NONE',  ( -28.68588794268871922, 426.3698905683720568, 16.75240474999999307 ) ) ;
#15046=CARTESIAN_POINT ( 'NONE',  ( -11.73070664223726389, 511.3073905601784759, 11.32908994701042005 ) ) ;
#15048=CARTESIAN_POINT ( 'NONE',  ( -10.20829729246299067, 401.6198905601784759, 7.653668647301790529 ) ) ;
#15051=ORIENTED_EDGE ( 'NONE', *, *, #4797, .T. ) ;
#15053=CARTESIAN_POINT ( 'NONE',  ( -14.48388495494901740, 529.4323905683720568, 9.489475012073732785 ) ) ;
#15054=CARTESIAN_POINT ( 'NONE',  ( -8.685887942688717445, 312.2448905601784759, -2.449293598294705724E-15 ) ) ;
#15057=CARTESIAN_POINT ( 'NONE',  ( -14.48388495494899431, 321.3073905683720568, -9.489475012073734561 ) ) ;
#15058=CARTESIAN_POINT ( 'NONE',  ( -45.43829269268870519, 374.1823905683720568, 3.332260488124734632 ) ) ;
#15059=ADVANCED_FACE ( 'NONE', ( #20393 ), #12282, .T. ) ;
#15060=CARTESIAN_POINT ( 'NONE',  ( -11.93348319268872082, 358.8698905683720000, -2.051577885510841163E-15 ) ) ;
#15061=EDGE_CURVE ( 'NONE', #1213, #16932, #13731, .T. ) ;
#15062=CARTESIAN_POINT ( 'NONE',  ( -8.685887942688715668, 297.3073905765655809, -3.978247347593165895 ) ) ;
#15064=CARTESIAN_POINT ( 'NONE',  ( -14.48388495494898898, 269.8073905683720000, -9.489475012073734561 ) ) ;
#15066=CARTESIAN_POINT ( 'NONE',  ( -42.88789093042844058, 416.3073905683720568, 9.489475012073736337 ) ) ;
#15072=CARTESIAN_POINT ( 'NONE',  ( -14.48388495494899431, 321.3073905683720000, -9.489475012073736337 ) ) ;
#15073=CARTESIAN_POINT ( 'NONE',  ( -19.19641293061499354, 477.3073905683720568, 14.20200298773971426 ) ) ;
#15075=CARTESIAN_POINT ( 'NONE',  ( -42.82802356641967378, 478.4948905601784759, 14.14213562373094923 ) ) ;
#15076=CARTESIAN_POINT ( 'NONE',  ( -11.93348319268871727, 308.5573905683719431, 3.332260488124728415 ) ) ;
#15078=CARTESIAN_POINT ( 'NONE',  ( -48.68588794268887199, 342.3073905765656377, 3.978247347592742678 ) ) ;
#15081=CARTESIAN_POINT ( 'NONE',  ( -25.35362745456399480, 382.5573905683720000, -16.75240474999999307 ) ) ;
#15082=CARTESIAN_POINT ( 'NONE',  ( -36.33955658999052218, 443.8698905765656377, 18.47759065022572500 ) ) ;
#15083=CARTESIAN_POINT ( 'NONE',  ( -47.16347859291444422, 382.6198905765655809, 7.653668647301805628 ) ) ;
#15084=CARTESIAN_POINT ( 'NONE',  ( -45.43829269268871940, 433.8698905683720568, 0.000000000000000000 ) ) ;
#15085=CARTESIAN_POINT ( 'NONE',  ( -25.35362745456397704, 252.5573905683720284, -16.75240474999999307 ) ) ;
#15086=CARTESIAN_POINT ( 'NONE',  ( -28.68588794268872277, 421.3698905683720568, -16.75240474999999307 ) ) ;
#15088=CARTESIAN_POINT ( 'NONE',  ( -17.35679799567829207, 400.6823905601784759, 16.95518130045146421 ) ) ;
#15089=CARTESIAN_POINT ( 'NONE',  ( -11.73070664223725146, 357.9323905765656377, -11.32908994701042715 ) ) ;
#15091=CARTESIAN_POINT ( 'NONE',  ( -11.73070664223723725, 263.1823905601784759, -11.32908994701042538 ) ) ;
#15092=CARTESIAN_POINT ( 'NONE',  ( -14.48388495494899431, 327.9323905683721136, 9.489475012073731008 ) ) ;
#15094=CARTESIAN_POINT ( 'NONE',  ( -14.48388495494900852, 469.4323905683720568, 9.489475012073732785 ) ) ;
#15096=CARTESIAN_POINT ( 'NONE',  ( -48.68588794268872988, 527.2448905601785327, 0.000000000000000000 ) ) ;
#15098=CARTESIAN_POINT ( 'NONE',  ( -13.20868407381886378, 390.9948905683720568, -6.410867750099233042 ) ) ;
#15100=CARTESIAN_POINT ( 'NONE',  ( -44.16309181155855157, 225.9948905683720284, 6.410867750099241924 ) ) ;
#15101=CARTESIAN_POINT ( 'NONE',  ( -11.93348319268872082, 358.8698905683720000, -2.051577885510841163E-15 ) ) ;
#15104=CARTESIAN_POINT ( 'NONE',  ( -40.53162694259545873, 515.1198905683720568, 11.84573899990672885 ) ) ;
#15106=CARTESIAN_POINT ( 'NONE',  ( -35.09675569278795848, 437.2448905683720000, 15.47720386886985366 ) ) ;
#15107=CARTESIAN_POINT ( 'NONE',  ( -16.84014894278201169, 530.1198905683720568, -11.84573899990672707 ) ) ;
#15109=DIRECTION ( 'NONE',  ( -1.191790137725560488E-16, 1.000000000000000000, -0.000000000000000000 ) ) ;
#15110=CARTESIAN_POINT ( 'NONE',  ( -42.88789093042844769, 482.9323905683720568, -9.489475012073736337 ) ) ;
#15112=CARTESIAN_POINT ( 'NONE',  ( -40.53162694259545873, 512.6198905683720568, -11.84573899990672707 ) ) ;
#15114=EDGE_CURVE ( 'NONE', #21365, #8857, #10832, .T. ) ;
#15116=CARTESIAN_POINT ( 'NONE',  ( -40.01497788969913927, 423.5573905765656377, 16.95518130045146776 ) ) ;
#15118=CARTESIAN_POINT ( 'NONE',  ( -48.68588794268870146, 327.2448905601785327, 0.000000000000000000 ) ) ;
#15119=DIRECTION ( 'NONE',  ( -1.191790137725560488E-16, 1.000000000000000000, -0.000000000000000000 ) ) ;
#15120=DIRECTION ( 'NONE',  ( -1.000000000000000000, 0.000000000000000000, 0.000000000000000000 ) ) ;
#15124=CARTESIAN_POINT ( 'NONE',  ( -9.816881303989697827, 223.9102039777117170, -6.855710153614462676 ) ) ;
#15125=CARTESIAN_POINT ( 'NONE',  ( -11.93348319268871194, 290.3698905683720568, -2.051577885510841163E-15 ) ) ;
#15126=CARTESIAN_POINT ( 'NONE',  ( -17.35679799567830983, 530.6823905601785327, 16.95518130045146421 ) ) ;
#15127=CARTESIAN_POINT ( 'NONE',  ( -11.73070664223723369, 261.3073905601784759, 11.32908994701042005 ) ) ;
#15129=CARTESIAN_POINT ( 'NONE',  ( -16.84014894278197971, 289.1198905683720568, 11.84573899990672530 ) ) ;
#15132=VERTEX_POINT ( 'NONE', #4487 ) ;
#15134=CARTESIAN_POINT ( 'NONE',  ( -38.17536295476247687, 513.8073905683720568, -14.20200298773971426 ) ) ;
#15135=VECTOR ( 'NONE', #3789, 1000.000000000000000 ) ;
#15137=CARTESIAN_POINT ( 'NONE',  ( -14.48388495494900852, 459.4323905683720568, 9.489475012073732785 ) ) ;
#15139=CARTESIAN_POINT ( 'NONE',  ( -22.27502019258947641, 260.7448905683720000, -15.47720386886985544 ) ) ;
#15141=CARTESIAN_POINT ( 'NONE',  ( -45.64106924314017988, 332.9323905765655809, 11.32908994701042538 ) ) ;
#15143=CARTESIAN_POINT ( 'NONE',  ( -35.09675569278793006, 253.4948905683720568, -15.47720386886985544 ) ) ;
#15144=CARTESIAN_POINT ( 'NONE',  ( -47.16347859291443001, 241.3698905765656093, -7.653668647301793193 ) ) ;
#15145=CARTESIAN_POINT ( 'NONE',  ( -8.685887942688717445, 312.2448905601784759, -2.449293598294705724E-15 ) ) ;
#15146=CARTESIAN_POINT ( 'NONE',  ( -47.16347859291443001, 226.6198905601785043, -7.653668647301793193 ) ) ;
#15147=CARTESIAN_POINT ( 'NONE',  ( -32.01814843081343298, 271.6823905683720000, -16.75240474999999307 ) ) ;
#15148=CARTESIAN_POINT ( 'NONE',  ( -19.19641293061498288, 348.8073905683720000, 14.20200298773971426 ) ) ;
#15149=CARTESIAN_POINT ( 'NONE',  ( -14.54375231895778775, 503.4948905601784759, -14.14213562373094746 ) ) ;
#15150=( BOUNDED_CURVE ( )  B_SPLINE_CURVE ( 2, ( #1678, #19946, #61, #5330, #18524, #9871, #10297, #6629, #5123, #3402, #16921, #9982, #8680, #1901, #21354, #6520, #13137 ),
 .UNSPECIFIED., .F., .T. ) 
 B_SPLINE_CURVE_WITH_KNOTS ( ( 3, 2, 2, 2, 2, 2, 2, 2, 3 ),
 ( 0.1250000000000001110, 0.1269531250000001110, 0.1289062500000001110, 0.1308593750000001110, 0.1328125000000001110, 0.1347656250000001388, 0.1367187500000001388, 0.1386718750000001388, 0.1406250000000001388 ),
 .UNSPECIFIED. ) 
 CURVE ( )  GEOMETRIC_REPRESENTATION_ITEM ( )  RATIONAL_B_SPLINE_CURVE ( ( 0.9999999999999988898, 0.9807852804032315408, 1.000000000000000000, 0.9807852804032304306, 1.000000000000000000, 0.9807852804032304306, 1.000000000000000000, 0.9807852804032304306, 1.000000000000000000, 0.9807852804032304306, 1.000000000000000000, 0.9807852804032304306, 1.000000000000000000, 0.9807852804032304306, 1.000000000000000000, 0.9807852804032290983, 1.000000000000001332 ) ) 
 REPRESENTATION_ITEM ( '' )  );
#15152=CARTESIAN_POINT ( 'NONE',  ( -22.27502019258948351, 406.9948905683720000, 15.47720386886985189 ) ) ;
#15153=CARTESIAN_POINT ( 'NONE',  ( -48.68588794268878672, 507.5573905601784759, 3.978247347593009131 ) ) ;
#15154=ORIENTED_EDGE ( 'NONE', *, *, #7561, .F. ) ;
#15155=CARTESIAN_POINT ( 'NONE',  ( -36.33955658999052218, 409.1198905601784759, 18.47759065022572500 ) ) ;
#15158=CARTESIAN_POINT ( 'NONE',  ( -11.93348319268874036, 520.6823905683719431, -3.332260488124732856 ) ) ;
#15159=CARTESIAN_POINT ( 'NONE',  ( -21.03221929538691271, 284.1198905601784759, -18.47759065022572855 ) ) ;
#15161=CARTESIAN_POINT ( 'NONE',  ( -40.53162694259543031, 324.1198905683720568, -11.84573899990672707 ) ) ;
#15162=CARTESIAN_POINT ( 'NONE',  ( -14.48388495494899963, 359.8073905683720000, -9.489475012073736337 ) ) ;
#15163=CARTESIAN_POINT ( 'NONE',  ( -44.16309181155857289, 373.2448905683720000, -6.410867750099231266 ) ) ;
#15164=CARTESIAN_POINT ( 'NONE',  ( -24.70764059509554045, 294.8073905765655809, 19.99999999999998934 ) ) ;
#15166=CARTESIAN_POINT ( 'NONE',  ( -16.84014894278197616, 257.6198905683720568, 11.84573899990672530 ) ) ;
#15167=CARTESIAN_POINT ( 'NONE',  ( -8.685887942688820473, 441.9323905601784759, 3.978247347593374172 ) ) ;
#15168=CARTESIAN_POINT ( 'NONE',  ( -13.20868407381886733, 420.9948905683720000, -6.410867750099233042 ) ) ;
#15172=CARTESIAN_POINT ( 'NONE',  ( -10.20829729246298712, 381.6198905601784759, 7.653668647301790529 ) ) ;
#15174=CARTESIAN_POINT ( 'NONE',  ( -45.43829269268869808, 325.6823905683721136, 3.332260488124734632 ) ) ;
#15175=CARTESIAN_POINT ( 'NONE',  ( -35.09675569278795848, 471.9948905683720000, -15.47720386886985544 ) ) ;
#15177=VERTEX_POINT ( 'NONE', #2871 ) ;
#15178=CARTESIAN_POINT ( 'NONE',  ( -48.68588794268872277, 457.2448905601784759, 0.000000000000000000 ) ) ;
#15179=CARTESIAN_POINT ( 'NONE',  ( -16.84014894278197971, 297.6198905683720000, 11.84573899990672530 ) ) ;
#15181=VERTEX_POINT ( 'NONE', #12607 ) ;
#15183=CARTESIAN_POINT ( 'NONE',  ( -8.685887942688719221, 341.9323905601785327, 3.978247347593161010 ) ) ;
#15185=CARTESIAN_POINT ( 'NONE',  ( -11.93348319268872260, 380.3698905683720568, -2.051577885510841163E-15 ) ) ;
#15186=CARTESIAN_POINT ( 'NONE',  ( -47.16347859291445843, 477.8698905601784759, 7.653668647301805628 ) ) ;
#15187=CARTESIAN_POINT ( 'NONE',  ( -22.27502019258949417, 420.7448905683720000, -15.47720386886985544 ) ) ;
#15188=CARTESIAN_POINT ( 'NONE',  ( -35.09675569278793716, 267.2448905683720568, 15.47720386886985366 ) ) ;
#15189=CARTESIAN_POINT ( 'NONE',  ( -44.16309181155857289, 424.4948905683720568, 6.410867750099241924 ) ) ;
#15191=CARTESIAN_POINT ( 'NONE',  ( -24.70764059509555111, 400.0573905601784759, 19.99999999999998934 ) ) ;
#15193=CARTESIAN_POINT ( 'NONE',  ( -40.01497788969913927, 370.4323905765656377, -16.95518130045146421 ) ) ;
#15196=CARTESIAN_POINT ( 'NONE',  ( -38.17536295476244135, 325.4323905683720000, 14.20200298773971781 ) ) ;
#15198=CARTESIAN_POINT ( 'NONE',  ( -45.43829269268871940, 475.0573905683720000, -3.332260488124726194 ) ) ;
#15200=CARTESIAN_POINT ( 'NONE',  ( -10.20829729246297823, 302.8698905601784759, -7.653668647301794969 ) ) ;
#15202=CARTESIAN_POINT ( 'NONE',  ( -16.84014894278199392, 391.6198905683720568, -11.84573899990672707 ) ) ;
#15204=CARTESIAN_POINT ( 'NONE',  ( -14.54375231895778953, 523.4948905601785327, -14.14213562373094746 ) ) ;
#15205=CARTESIAN_POINT ( 'NONE',  ( -25.35362745456399125, 361.0573905683720000, -16.75240474999999307 ) ) ;
#15207=ORIENTED_EDGE ( 'NONE', *, *, #867, .T. ) ;
#15208=CARTESIAN_POINT ( 'NONE',  ( -40.53162694259545873, 532.6198905683720568, -11.84573899990672707 ) ) ;
#15210=CARTESIAN_POINT ( 'NONE',  ( -44.16309181155858710, 514.4948905683720568, 6.410867750099241924 ) ) ;
#15212=CARTESIAN_POINT ( 'NONE',  ( -36.33955658999052929, 530.1198905765655809, -18.47759065022572855 ) ) ;
#15213=CARTESIAN_POINT ( 'NONE',  ( -42.88789093042844769, 492.9323905683720568, -9.489475012073736337 ) ) ;
#15215=CARTESIAN_POINT ( 'NONE',  ( -45.43829269268872650, 493.8698905683720568, 0.000000000000000000 ) ) ;
#15217=CARTESIAN_POINT ( 'NONE',  ( -28.68588794268872277, 419.4948905765656377, -19.99999999999999289 ) ) ;
#15220=FACE_OUTER_BOUND ( 'NONE', #8958, .T. ) ;
#15223=CARTESIAN_POINT ( 'NONE',  ( -48.68588794268881514, 492.3073905765656946, 3.978247347592954952 ) ) ;
#15224=CARTESIAN_POINT ( 'NONE',  ( -35.09675569278793716, 293.4948905683720000, -15.47720386886985544 ) ) ;
#15225=CARTESIAN_POINT ( 'NONE',  ( -48.68588794268875120, 527.5573905601784190, 3.978247347593114824 ) ) ;
#15226=CARTESIAN_POINT ( 'NONE',  ( -42.88789093042844769, 454.4323905683720568, -9.489475012073736337 ) ) ;
#15227=CARTESIAN_POINT ( 'NONE',  ( -28.68588794268871922, 414.4948905765656377, 19.99999999999999289 ) ) ;
#15228=CARTESIAN_POINT ( 'NONE',  ( -40.53162694259542320, 266.6198905683720568, 11.84573899990672885 ) ) ;
#15231=CARTESIAN_POINT ( 'NONE',  ( -13.20868407381887799, 500.9948905683721136, -6.410867750099233042 ) ) ;
#15232=EDGE_CURVE ( 'NONE', #232, #8850, #1247, .T. ) ;
#15233=VECTOR ( 'NONE', #19716, 1000.000000000000000 ) ;
#15236=CARTESIAN_POINT ( 'NONE',  ( -19.19641293061498999, 458.8073905683720000, 14.20200298773971426 ) ) ;
#15239=CARTESIAN_POINT ( 'NONE',  ( -16.84014894278197971, 260.1198905683720568, -11.84573899990672707 ) ) ;
#15242=CARTESIAN_POINT ( 'NONE',  ( -28.68588794268870856, 334.4948905765656377, 19.99999999999999289 ) ) ;
#15243=CARTESIAN_POINT ( 'NONE',  ( -22.27502019258946575, 268.4948905683720000, 15.47720386886985189 ) ) ;
#15245=CARTESIAN_POINT ( 'NONE',  ( -32.01814843081343298, 243.1823905683720284, -16.75240474999999307 ) ) ;
#15248=CARTESIAN_POINT ( 'NONE',  ( -28.68588794268874054, 573.2448905601785327, 0.000000000000000000 ) ) ;
#15249=CARTESIAN_POINT ( 'NONE',  ( -13.20868407381884779, 259.4948905683720568, -6.410867750099233042 ) ) ;
#15250=CARTESIAN_POINT ( 'NONE',  ( -28.68588794268871567, 362.8698905683720000, -16.75240474999999307 ) ) ;
#15254=APPLICATION_CONTEXT ( 'automotive_design' ) ;
#15257=CARTESIAN_POINT ( 'NONE',  ( -28.68588794268872277, 411.3698905683720568, -16.75240474999999307 ) ) ;
#15260=CARTESIAN_POINT ( 'NONE',  ( -48.68588794268871567, 407.5573905601784759, 3.978247347593168115 ) ) ;
#15265=CARTESIAN_POINT ( 'NONE',  ( -16.84014894278200458, 519.1198905683720568, 11.84573899990672530 ) ) ;
#15266=CARTESIAN_POINT ( 'NONE',  ( -21.03221929538690205, 280.3698905601784759, 18.47759065022572500 ) ) ;
#15267=CARTESIAN_POINT ( 'NONE',  ( -48.68588794268853803, 321.6823905765655809, -3.978247347593583783 ) ) ;
#15268=VERTEX_POINT ( 'NONE', #15963 ) ;
#15269=CARTESIAN_POINT ( 'NONE',  ( -28.68588794268871212, 332.8698905683720000, -16.75240474999999307 ) ) ;
#15271=CARTESIAN_POINT ( 'NONE',  ( -44.16309181155856578, 364.4948905683720568, 6.410867750099241924 ) ) ;
#15272=CARTESIAN_POINT ( 'NONE',  ( -11.93348319268872260, 368.5573905683719431, 3.332260488124728859 ) ) ;
#15274=CARTESIAN_POINT ( 'NONE',  ( -17.35679799567829207, 298.5573905765656377, -16.95518130045146421 ) ) ;
#15276=CARTESIAN_POINT ( 'NONE',  ( -38.17536295476244135, 262.3073905683720568, -14.20200298773971426 ) ) ;
#15278=( BOUNDED_CURVE ( )  B_SPLINE_CURVE ( 2, ( #966, #12633, #19004, #17599, #1072, #2790, #6023, #14266, #9155, #20956, #2575, #21060, #19224, #7642, #12525, #10990, #7850 ),
 .UNSPECIFIED., .F., .T. ) 
 B_SPLINE_CURVE_WITH_KNOTS ( ( 3, 2, 2, 2, 2, 2, 2, 2, 3 ),
 ( 0.7656250000000001110, 0.7675781250000001110, 0.7695312500000001110, 0.7714843750000001110, 0.7734375000000001110, 0.7753906250000001110, 0.7773437500000001110, 0.7792968750000001110, 0.7812500000000001110 ),
 .UNSPECIFIED. ) 
 CURVE ( )  GEOMETRIC_REPRESENTATION_ITEM ( )  RATIONAL_B_SPLINE_CURVE ( ( 0.9999999999999988898, 0.9807852804032315408, 1.000000000000000000, 0.9807852804032304306, 1.000000000000000000, 0.9807852804032304306, 1.000000000000000000, 0.9807852804032304306, 1.000000000000000000, 0.9807852804032304306, 1.000000000000000000, 0.9807852804032304306, 1.000000000000000000, 0.9807852804032304306, 1.000000000000000000, 0.9807852804032293204, 1.000000000000001110 ) ) 
 REPRESENTATION_ITEM ( '' )  );
#15279=CARTESIAN_POINT ( 'NONE',  ( -11.93348319268872793, 420.3698905683720568, -2.051577885510841163E-15 ) ) ;
#15281=CARTESIAN_POINT ( 'NONE',  ( -28.68588794268872633, 449.4948905765655809, -19.99999999999999289 ) ) ;
#15284=CARTESIAN_POINT ( 'NONE',  ( -11.93348319268871904, 330.6823905683721136, -3.332260488124732856 ) ) ;
#15285=CARTESIAN_POINT ( 'NONE',  ( -16.84014894278200458, 470.1198905683720568, -11.84573899990672707 ) ) ;
#15287=CARTESIAN_POINT ( 'NONE',  ( -42.82802356641967378, 458.4948905601784759, 14.14213562373094923 ) ) ;
#15288=CARTESIAN_POINT ( 'NONE',  ( -40.53162694259543031, 282.6198905683720000, -11.84573899990672707 ) ) ;
#15289=CARTESIAN_POINT ( 'NONE',  ( -17.35679799567828852, 345.4323905765656377, 16.95518130045146421 ) ) ;
#15292=CARTESIAN_POINT ( 'NONE',  ( -11.73070664223724968, 343.1823905601785327, -11.32908994701042715 ) ) ;
#15293=CARTESIAN_POINT ( 'NONE',  ( -38.17536295476244845, 302.3073905683720568, -14.20200298773971426 ) ) ;
#15294=CARTESIAN_POINT ( 'NONE',  ( -25.35362745456398414, 388.1823905683720568, 16.75240474999998952 ) ) ;
#15295=CARTESIAN_POINT ( 'NONE',  ( -8.685887942688625074, 292.5573905601784190, -3.978247347592952732 ) ) ;
#15296=DIRECTION ( 'NONE',  ( -1.000000000000000000, 0.000000000000000000, 0.000000000000000000 ) ) ;
#15297=CARTESIAN_POINT ( 'NONE',  ( -25.35362745456398770, 426.6823905683720568, 16.75240474999998952 ) ) ;
#15298=CARTESIAN_POINT ( 'NONE',  ( -28.68588794268869790, 257.8698905683720000, 16.75240474999999307 ) ) ;
#15299=CARTESIAN_POINT ( 'NONE',  ( -25.35362745456399836, 431.0573905683720000, -16.75240474999999307 ) ) ;
#15300=SHAPE_DEFINITION_REPRESENTATION ( #6125, #4206 ) ;
#15301=CARTESIAN_POINT ( 'NONE',  ( -8.685887942688722774, 367.3073905765656946, -3.978247347593165895 ) ) ;
#15303=CARTESIAN_POINT ( 'NONE',  ( -14.48388495494899608, 329.8073905683720568, -9.489475012073734561 ) ) ;
#15305=CARTESIAN_POINT ( 'NONE',  ( -45.43829269268871940, 485.6823905683721136, 3.332260488124734632 ) ) ;
#15309=CARTESIAN_POINT ( 'NONE',  ( -14.54375231895776288, 303.4948905601784759, -14.14213562373094746 ) ) ;
#15310=CARTESIAN_POINT ( 'NONE',  ( -38.17536295476246266, 393.8073905683720000, -14.20200298773971426 ) ) ;
#15314=CARTESIAN_POINT ( 'NONE',  ( -21.03221929538694468, 534.1198905601785327, -18.47759065022572855 ) ) ;
#15315=CARTESIAN_POINT ( 'NONE',  ( -16.84014894278199037, 350.1198905683720568, -11.84573899990672707 ) ) ;
#15318=CARTESIAN_POINT ( 'NONE',  ( -25.35362745456401257, 531.0573905683720568, -16.75240474999999307 ) ) ;
#15319=ORIENTED_EDGE ( 'NONE', *, *, #1933, .F. ) ;
#15320=CARTESIAN_POINT ( 'NONE',  ( -45.43829269268872650, 513.5573905683719431, -3.332260488124726194 ) ) ;
#15321=ORIENTED_EDGE ( 'NONE', *, *, #16505, .F. ) ;
#15323=CARTESIAN_POINT ( 'NONE',  ( -32.01814843081346140, 481.6823905683720568, -16.75240474999999307 ) ) ;
#15325=CARTESIAN_POINT ( 'NONE',  ( -42.88789093042844769, 482.9323905683720000, -9.489475012073734561 ) ) ;
#15327=EDGE_CURVE ( 'NONE', #13421, #9261, #5590, .T. ) ;
#15329=CARTESIAN_POINT ( 'NONE',  ( -42.82802356641966668, 430.7448905765656377, -14.14213562373094746 ) ) ;
#15332=CARTESIAN_POINT ( 'NONE',  ( -21.03221929538693402, 438.8698905765656377, -18.47759065022572855 ) ) ;
#15336=DIRECTION ( 'NONE',  ( -1.000000000000000000, 0.000000000000000000, 0.000000000000000000 ) ) ;
#15338=CARTESIAN_POINT ( 'NONE',  ( -22.27502019258947996, 302.2448905683720000, -15.47720386886985544 ) ) ;
#15340=CARTESIAN_POINT ( 'NONE',  ( -38.17536295476245556, 446.9323905683720000, 14.20200298773971781 ) ) ;
#15341=CARTESIAN_POINT ( 'NONE',  ( -24.70764059509556176, 399.1823905765656377, -19.99999999999999289 ) ) ;
#15342=CARTESIAN_POINT ( 'NONE',  ( -45.43829269268870519, 275.3698905683720000, 0.000000000000000000 ) ) ;
#15343=ADVANCED_FACE ( 'NONE', ( #17990 ), #8135, .T. ) ;
#15346=CARTESIAN_POINT ( 'NONE',  ( -24.70764059509557953, 534.4323905601784190, -19.99999999999999289 ) ) ;
#15347=CARTESIAN_POINT ( 'NONE',  ( -45.43829269268872650, 485.3698905683720568, 0.000000000000000000 ) ) ;
#15350=CARTESIAN_POINT ( 'NONE',  ( -35.09675569278796559, 457.2448905683720568, 15.47720386886985366 ) ) ;
#15351=CARTESIAN_POINT ( 'NONE',  ( -32.66413529028187668, 409.8073905765656377, -19.99999999999999289 ) ) ;
#15352=CARTESIAN_POINT ( 'NONE',  ( -19.19641293061496867, 257.3073905683720568, 14.20200298773971426 ) ) ;
#15354=CARTESIAN_POINT ( 'NONE',  ( -47.16347859291444422, 332.6198905765656377, 7.653668647301805628 ) ) ;
#15355=CARTESIAN_POINT ( 'NONE',  ( -8.685887942688736985, 477.3073905765656377, -3.978247347593165895 ) ) ;
#15356=CARTESIAN_POINT ( 'NONE',  ( -8.685887942688726326, 392.2448905601784759, -2.449293598294705724E-15 ) ) ;
#15357=CARTESIAN_POINT ( 'NONE',  ( -44.16309181155855157, 235.9948905683720284, 6.410867750099241924 ) ) ;
#15358=CARTESIAN_POINT ( 'NONE',  ( -36.33955658999051508, 420.1198905765656377, -18.47759065022572855 ) ) ;
#15359=CARTESIAN_POINT ( 'NONE',  ( -45.64106924314017277, 238.1823905601785043, 11.32908994701042715 ) ) ;
#15360=CARTESIAN_POINT ( 'NONE',  ( -35.09675569278793006, 241.9948905683720284, -15.47720386886985544 ) ) ;
#15362=CARTESIAN_POINT ( 'NONE',  ( -40.53162694259543741, 366.6198905683720000, 11.84573899990672885 ) ) ;
#15365=CARTESIAN_POINT ( 'NONE',  ( -14.48388495494900496, 409.8073905683720568, -9.489475012073736337 ) ) ;
#15366=CARTESIAN_POINT ( 'NONE',  ( -36.33955658999050797, 340.1198905765655809, -18.47759065022572855 ) ) ;
#15367=CARTESIAN_POINT ( 'NONE',  ( -45.64106924314019409, 406.3073905601784759, -11.32908994701042715 ) ) ;
#15369=CARTESIAN_POINT ( 'NONE',  ( -42.82802356641965957, 350.7448905765655809, -14.14213562373094746 ) ) ;
#15372=CARTESIAN_POINT ( 'NONE',  ( -40.53162694259545873, 524.1198905683720568, -11.84573899990672707 ) ) ;
#15373=CARTESIAN_POINT ( 'NONE',  ( -14.54375231895775578, 280.9948905601785327, 14.14213562373094568 ) ) ;
#15375=CARTESIAN_POINT ( 'NONE',  ( -13.20868407381885490, 329.7448905683720568, 6.410867750099229490 ) ) ;
#15376=EDGE_LOOP ( 'NONE', ( #8959, #7116, #17948, #12939 ) ) ;
#15377=CARTESIAN_POINT ( 'NONE',  ( -28.68588794268871212, 341.3698905683720000, -16.75240474999999307 ) ) ;
#15378=CARTESIAN_POINT ( 'NONE',  ( -19.19641293061497933, 357.3073905683720000, 14.20200298773971426 ) ) ;
#15379=EDGE_CURVE ( 'NONE', #573, #502, #13057, .T. ) ;
#15380=CARTESIAN_POINT ( 'NONE',  ( -28.68588794268870146, 274.4948905765656377, 19.99999999999999289 ) ) ;
#15382=CARTESIAN_POINT ( 'NONE',  ( -25.35362745456396993, 266.6823905683720568, 16.75240474999998952 ) ) ;
#15383=CARTESIAN_POINT ( 'NONE',  ( -43.31864445205426506, 201.3798797254112856, 3.307266650052995693 ) ) ;
#15384=CARTESIAN_POINT ( 'NONE',  ( -32.01814843081345430, 417.5573905683720568, 16.75240474999999307 ) ) ;
#15387=CARTESIAN_POINT ( 'NONE',  ( -44.16309181155855867, 325.9948905683720000, 6.410867750099241924 ) ) ;
#15388=CARTESIAN_POINT ( 'NONE',  ( -28.68588794268872633, 466.3698905683720000, 16.75240474999999307 ) ) ;
#15390=CARTESIAN_POINT ( 'NONE',  ( -47.16347859291445843, 476.6198905601785327, -7.653668647301793193 ) ) ;
#15391=CARTESIAN_POINT ( 'NONE',  ( -25.35362745456397349, 286.6823905683720568, 16.75240474999998952 ) ) ;
#15393=ORIENTED_EDGE ( 'NONE', *, *, #12854, .T. ) ;
#15396=CARTESIAN_POINT ( 'NONE',  ( -25.35362745456397349, 296.6823905683720000, 16.75240474999998952 ) ) ;
#15397=CARTESIAN_POINT ( 'NONE',  ( -44.16309181155856578, 375.9948905683720568, 6.410867750099241924 ) ) ;
#15399=CARTESIAN_POINT ( 'NONE',  ( -10.20829729246300666, 526.3698905765656946, 7.653668647301790529 ) ) ;
#15400=CARTESIAN_POINT ( 'NONE',  ( -14.48388495494900496, 399.8073905683720568, -9.489475012073736337 ) ) ;
#15401=CARTESIAN_POINT ( 'NONE',  ( -44.16309181155855157, 255.9948905683720568, 6.410867750099241924 ) ) ;
#15402=CARTESIAN_POINT ( 'NONE',  ( -35.09675569278795848, 435.7448905683720000, 15.47720386886985366 ) ) ;
#15404=( BOUNDED_CURVE ( )  B_SPLINE_CURVE ( 2, ( #11906, #7346, #5409, #13549, #13865, #7238, #15703, #13979, #15281, #12013, #2182, #3999, #2287, #2500, #465, #5728, #17109 ),
 .UNSPECIFIED., .F., .T. ) 
 B_SPLINE_CURVE_WITH_KNOTS ( ( 3, 2, 2, 2, 2, 2, 2, 2, 3 ),
 ( 0.2500000000000002220, 0.2519531250000002220, 0.2539062500000002220, 0.2558593750000002220, 0.2578125000000002220, 0.2597656250000002220, 0.2617187500000002220, 0.2636718750000002220, 0.2656250000000002220 ),
 .UNSPECIFIED. ) 
 CURVE ( )  GEOMETRIC_REPRESENTATION_ITEM ( )  RATIONAL_B_SPLINE_CURVE ( ( 0.9999999999999977796, 0.9807852804032326510, 1.000000000000000000, 0.9807852804032304306, 1.000000000000000000, 0.9807852804032304306, 1.000000000000000000, 0.9807852804032304306, 1.000000000000000000, 0.9807852804032304306, 1.000000000000000000, 0.9807852804032304306, 1.000000000000000000, 0.9807852804032304306, 1.000000000000000000, 0.9807852804032282101, 1.000000000000002220 ) ) 
 REPRESENTATION_ITEM ( '' )  );
#15405=ADVANCED_FACE ( 'NONE', ( #18421 ), #8572, .T. ) ;
#15406=CARTESIAN_POINT ( 'NONE',  ( -45.64106924314018698, 362.9323905765656377, 11.32908994701042715 ) ) ;
#15407=EDGE_CURVE ( 'NONE', #9092, #8857, #2004, .T. ) ;
#15408=CARTESIAN_POINT ( 'NONE',  ( -40.01497788969913216, 275.6823905601784759, -16.95518130045146421 ) ) ;
#15409=CARTESIAN_POINT ( 'NONE',  ( -35.09675569278794427, 325.7448905683720000, 15.47720386886985366 ) ) ;
#15410=CARTESIAN_POINT ( 'NONE',  ( -40.01497788969913927, 433.5573905765656946, 16.95518130045146776 ) ) ;
#15413=CARTESIAN_POINT ( 'NONE',  ( -28.68588794268871567, 387.8698905683720000, 16.75240474999999307 ) ) ;
#15415=CARTESIAN_POINT ( 'NONE',  ( -32.66413529028189799, 519.4323905601784190, 19.99999999999999289 ) ) ;
#15416=CARTESIAN_POINT ( 'NONE',  ( -35.09675569278795138, 345.7448905683720568, 15.47720386886985366 ) ) ;
#15418=CARTESIAN_POINT ( 'NONE',  ( -40.53162694259545873, 505.1198905683720568, 11.84573899990672885 ) ) ;
#15421=CARTESIAN_POINT ( 'NONE',  ( -40.01497788969913216, 315.6823905601785327, -16.95518130045146421 ) ) ;
#15424=CARTESIAN_POINT ( 'NONE',  ( -28.68588794268872277, 456.3698905683720000, 16.75240474999999307 ) ) ;
#15426=CARTESIAN_POINT ( 'NONE',  ( -25.35362745456400901, 491.0573905683720568, -16.75240474999999307 ) ) ;
#15428=CARTESIAN_POINT ( 'NONE',  ( -36.33955658999051508, 430.1198905765656377, -18.47759065022572855 ) ) ;
#15429=CARTESIAN_POINT ( 'NONE',  ( -48.68588794268872277, 471.9948905765656377, 0.000000000000000000 ) ) ;
#15432=CARTESIAN_POINT ( 'NONE',  ( -47.16347859291445843, 482.6198905765656377, 7.653668647301805628 ) ) ;
#15433=CARTESIAN_POINT ( 'NONE',  ( -28.68588794268873698, 548.2448905601784190, 0.000000000000000000 ) ) ;
#15436=CARTESIAN_POINT ( 'NONE',  ( -25.35362745456398059, 282.5573905683720568, -16.75240474999999307 ) ) ;
#15437=CARTESIAN_POINT ( 'NONE',  ( -40.01497788969911795, 248.8073905601784759, 16.95518130045146776 ) ) ;
#15438=CARTESIAN_POINT ( 'NONE',  ( -14.54375231895777176, 405.7448905765656377, 14.14213562373094568 ) ) ;
#15439=CARTESIAN_POINT ( 'NONE',  ( -19.19641293061499354, 451.9323905683720568, -14.20200298773971603 ) ) ;
#15441=CARTESIAN_POINT ( 'NONE',  ( -35.09675569278793006, 263.4948905683720000, -15.47720386886985544 ) ) ;
#15444=CARTESIAN_POINT ( 'NONE',  ( -32.66413529028189089, 535.0573905601784190, -19.99999999999999289 ) ) ;
#15445=CARTESIAN_POINT ( 'NONE',  ( -42.88789093042844769, 476.3073905683719431, 9.489475012073734561 ) ) ;
#15446=EDGE_CURVE ( 'NONE', #21369, #1587, #12232, .T. ) ;
#15449=ORIENTED_EDGE ( 'NONE', *, *, #13259, .T. ) ;
#15451=CARTESIAN_POINT ( 'NONE',  ( -45.43829269268869808, 263.8698905683720000, 0.000000000000000000 ) ) ;
#15454=CARTESIAN_POINT ( 'NONE',  ( -11.73070664223726212, 486.0573905765656946, 11.32908994701042005 ) ) ;
#15455=CARTESIAN_POINT ( 'NONE',  ( -42.82802356641965957, 388.4948905601784759, 14.14213562373094923 ) ) ;
#15456=CARTESIAN_POINT ( 'NONE',  ( -32.89526592549250950, 223.9102039777117170, -17.42271427295905184 ) ) ;
#15457=CARTESIAN_POINT ( 'NONE',  ( -14.48388495494898365, 239.4323905683720000, 9.489475012073731008 ) ) ;
#15459=CARTESIAN_POINT ( 'NONE',  ( -22.27502019258950483, 522.2448905683720568, -15.47720386886985544 ) ) ;
#15461=CARTESIAN_POINT ( 'NONE',  ( -13.20868407381884779, 249.4948905683720284, -6.410867750099233042 ) ) ;
#15462=CARTESIAN_POINT ( 'NONE',  ( -11.93348319268871904, 340.3698905683720000, -2.051577885510841163E-15 ) ) ;
#15466=CARTESIAN_POINT ( 'NONE',  ( -45.43829269268871229, 404.1823905683720568, 3.332260488124734632 ) ) ;
#15468=CARTESIAN_POINT ( 'NONE',  ( -8.685887942688726326, 412.5573905601785327, -3.978247347593165895 ) ) ;
#15473=CARTESIAN_POINT ( 'NONE',  ( -19.19641293061500065, 511.9323905683721136, -14.20200298773971603 ) ) ;
#15474=CARTESIAN_POINT ( 'NONE',  ( -32.66413529028186957, 285.0573905601784759, -19.99999999999999289 ) ) ;
#15475=CARTESIAN_POINT ( 'NONE',  ( -24.70764059509555466, 319.1823905765656377, -19.99999999999999289 ) ) ;
#15476=EDGE_LOOP ( 'NONE', ( #5086, #16801, #13148, #1266, #7221 ) ) ;
#15477=CARTESIAN_POINT ( 'NONE',  ( -45.43829269268870519, 325.3698905683720000, 0.000000000000000000 ) ) ;
#15479=CARTESIAN_POINT ( 'NONE',  ( -45.43829269268870519, 343.5573905683720000, -3.332260488124726194 ) ) ;
#15480=CARTESIAN_POINT ( 'NONE',  ( -16.84014894278198682, 367.6198905683720000, 11.84573899990672530 ) ) ;
#15481=CARTESIAN_POINT ( 'NONE',  ( -42.82802356641965247, 290.7448905765655809, -14.14213562373094746 ) ) ;
#15482=DIRECTION ( 'NONE',  ( -1.191790137725560488E-16, 1.000000000000000000, -0.000000000000000000 ) ) ;
#15483=CARTESIAN_POINT ( 'NONE',  ( -45.43829269268869808, 244.1823905683720568, 3.332260488124734632 ) ) ;
#15485=CARTESIAN_POINT ( 'NONE',  ( -32.01814843081345430, 413.1823905683719431, -16.75240474999999307 ) ) ;
#15486=CARTESIAN_POINT ( 'NONE',  ( -42.82802356641965957, 335.9948905601784759, -14.14213562373094746 ) ) ;
#15489=CARTESIAN_POINT ( 'NONE',  ( -25.35362745456398770, 322.5573905683720000, -16.75240474999999307 ) ) ;
#15490=CARTESIAN_POINT ( 'NONE',  ( -35.09675569278796559, 455.7448905683720568, 15.47720386886985366 ) ) ;
#15492=CARTESIAN_POINT ( 'NONE',  ( -11.73070664223725856, 471.3073905601784759, 11.32908994701042005 ) ) ;
#15493=CARTESIAN_POINT ( 'NONE',  ( -11.93348319268871371, 289.1823905683720000, -3.332260488124732856 ) ) ;
#15495=ORIENTED_EDGE ( 'NONE', *, *, #6915, .T. ) ;
#15496=CARTESIAN_POINT ( 'NONE',  ( -28.68588794268872633, 442.8698905683720568, -16.75240474999999307 ) ) ;
#15498=CARTESIAN_POINT ( 'NONE',  ( -48.68588794268872988, 511.9948905765656377, 0.000000000000000000 ) ) ;
#15499=CARTESIAN_POINT ( 'NONE',  ( -45.64106924314018698, 336.3073905601784759, -11.32908994701042715 ) ) ;
#15500=CARTESIAN_POINT ( 'NONE',  ( -13.20868407381885135, 298.2448905683720000, 6.410867750099229490 ) ) ;
#15501=CARTESIAN_POINT ( 'NONE',  ( -45.43829269268871229, 385.3698905683720568, 0.000000000000000000 ) ) ;
#15502=CARTESIAN_POINT ( 'NONE',  ( -32.66413529028185536, 229.4323905601785043, 19.99999999999999289 ) ) ;
#15503=EDGE_CURVE ( 'NONE', #20007, #19138, #19668, .T. ) ;
#15504=CARTESIAN_POINT ( 'NONE',  ( -10.20829729246300488, 517.6198905765656946, -7.653668647301794969 ) ) ;
#15505=CARTESIAN_POINT ( 'NONE',  ( -11.93348319268872615, 398.8698905683720000, -2.051577885510841163E-15 ) ) ;
#15506=CARTESIAN_POINT ( 'NONE',  ( -38.17536295476243424, 246.9323905683720284, 14.20200298773971781 ) ) ;
#15507=CARTESIAN_POINT ( 'NONE',  ( -32.01814843081344719, 431.6823905683720000, -16.75240474999999307 ) ) ;
#15510=CARTESIAN_POINT ( 'NONE',  ( -17.35679799567829207, 345.4323905765656377, 16.95518130045146421 ) ) ;
#15512=CARTESIAN_POINT ( 'NONE',  ( -35.09675569278795138, 335.7448905683720568, 15.47720386886985366 ) ) ;
#15513=CARTESIAN_POINT ( 'NONE',  ( -11.93348319268873503, 470.6823905683720568, -3.332260488124732856 ) ) ;
#15516=CARTESIAN_POINT ( 'NONE',  ( -32.66413529028186247, 305.0573905601784190, -19.99999999999999289 ) ) ;
#15517=CARTESIAN_POINT ( 'NONE',  ( -40.53162694259544452, 394.1198905683720000, -11.84573899990672707 ) ) ;
#15519=CARTESIAN_POINT ( 'NONE',  ( -8.685887942688742314, 521.9323905601785327, 3.978247347593161010 ) ) ;
#15520=CARTESIAN_POINT ( 'NONE',  ( -16.84014894278198682, 340.1198905683720568, -11.84573899990672707 ) ) ;
#15524=CARTESIAN_POINT ( 'NONE',  ( -19.19641293061500065, 510.4323905683720000, -14.20200298773971603 ) ) ;
#15525=ORIENTED_EDGE ( 'NONE', *, *, #10344, .T. ) ;
#15526=CARTESIAN_POINT ( 'NONE',  ( -8.685887942688719221, 352.5573905601784759, -3.978247347593165895 ) ) ;
#15527=( BOUNDED_CURVE ( )  B_SPLINE_CURVE ( 2, ( #3425, #12949, #19538, #11313, #19861, #10005, #17907, #1818, #18018, #3212, #9790, #1591, #8162, #720, #10320, #6975, #12060 ),
 .UNSPECIFIED., .F., .T. ) 
 B_SPLINE_CURVE_WITH_KNOTS ( ( 3, 2, 2, 2, 2, 2, 2, 2, 3 ),
 ( 0.7187500000000002220, 0.7207031250000002220, 0.7226562500000002220, 0.7246093750000002220, 0.7265625000000002220, 0.7285156250000003331, 0.7304687500000003331, 0.7324218750000003331, 0.7343750000000003331 ),
 .UNSPECIFIED. ) 
 CURVE ( )  GEOMETRIC_REPRESENTATION_ITEM ( )  RATIONAL_B_SPLINE_CURVE ( ( 0.9999999999999977796, 0.9807852804032326510, 1.000000000000000000, 0.9807852804032304306, 1.000000000000000000, 0.9807852804032304306, 1.000000000000000000, 0.9807852804032304306, 1.000000000000000000, 0.9807852804032304306, 1.000000000000000000, 0.9807852804032304306, 1.000000000000000000, 0.9807852804032304306, 1.000000000000000000, 0.9807852804032270999, 1.000000000000003331 ) ) 
 REPRESENTATION_ITEM ( '' )  );
#15528=CARTESIAN_POINT ( 'NONE',  ( -21.03221929538692692, 378.8698905765656377, -18.47759065022572855 ) ) ;
#15529=CARTESIAN_POINT ( 'NONE',  ( -17.35679799567828496, 315.4323905765656946, 16.95518130045146421 ) ) ;
#15531=CARTESIAN_POINT ( 'NONE',  ( -8.685887942688736985, 492.2448905601785327, -2.449293598294705724E-15 ) ) ;
#15532=CARTESIAN_POINT ( 'NONE',  ( -14.48388495494900852, 467.9323905683721136, 9.489475012073732785 ) ) ;
#15534=CARTESIAN_POINT ( 'NONE',  ( -11.93348319268873503, 479.1823905683720568, -3.332260488124732856 ) ) ;
#15535=CARTESIAN_POINT ( 'NONE',  ( -14.54375231895775222, 250.9948905601784759, 14.14213562373094568 ) ) ;
#15536=CARTESIAN_POINT ( 'NONE',  ( -8.685887942688726326, 406.9948905765656377, -2.449293598294705724E-15 ) ) ;
#15539=CARTESIAN_POINT ( 'NONE',  ( -32.66413529028188378, 485.0573905601785327, -19.99999999999999289 ) ) ;
#15542=VECTOR ( 'NONE', #10270, 1000.000000000000000 ) ;
#15547=CARTESIAN_POINT ( 'NONE',  ( -40.53162694259543031, 286.6198905683720000, 11.84573899990672885 ) ) ;
#15548=CARTESIAN_POINT ( 'NONE',  ( -45.64106924314017277, 256.3073905601784759, -11.32908994701042715 ) ) ;
#15549=CARTESIAN_POINT ( 'NONE',  ( -8.685887942688859553, 406.6823905765655809, 3.978247347593479866 ) ) ;
#15550=CARTESIAN_POINT ( 'NONE',  ( -25.35362745456399125, 448.1823905683719431, 16.75240474999998952 ) ) ;
#15551=CARTESIAN_POINT ( 'NONE',  ( -32.66413529028186957, 329.8073905765655809, -19.99999999999999289 ) ) ;
#15552=CARTESIAN_POINT ( 'NONE',  ( -16.84014894278197971, 261.6198905683720568, -11.84573899990672707 ) ) ;
#15555=CARTESIAN_POINT ( 'NONE',  ( -24.70764059509557242, 479.1823905765656377, -19.99999999999999289 ) ) ;
#15557=CARTESIAN_POINT ( 'NONE',  ( -22.27502019258949062, 488.4948905683720568, 15.47720386886985189 ) ) ;
#15560=CARTESIAN_POINT ( 'NONE',  ( -13.20868407381884779, 249.4948905683720284, -6.410867750099233042 ) ) ;
#15563=CARTESIAN_POINT ( 'NONE',  ( -21.03221929538692336, 465.1198905765655809, 18.47759065022572500 ) ) ;
#15567=CARTESIAN_POINT ( 'NONE',  ( -14.48388495494901740, 521.3073905683720568, -9.489475012073736337 ) ) ;
#15569=CARTESIAN_POINT ( 'NONE',  ( -38.17536295476244135, 242.3073905683720284, -14.20200298773971426 ) ) ;
#15570=CARTESIAN_POINT ( 'NONE',  ( -13.20868407381885667, 339.7448905683720568, 6.410867750099229490 ) ) ;
#15571=CARTESIAN_POINT ( 'NONE',  ( -32.66413529028186247, 319.4323905601785327, 19.99999999999999289 ) ) ;
#15573=CARTESIAN_POINT ( 'NONE',  ( -45.64106924314017277, 272.9323905765655809, 11.32908994701042538 ) ) ;
#15574=CARTESIAN_POINT ( 'NONE',  ( -16.84014894278199748, 410.1198905683720000, -11.84573899990672707 ) ) ;
#15575=CARTESIAN_POINT ( 'NONE',  ( -32.66413529028186247, 324.1823905765655809, 19.99999999999999289 ) ) ;
#15577=CARTESIAN_POINT ( 'NONE',  ( -42.82802356641966668, 395.9948905601784759, -14.14213562373094746 ) ) ;
#15583=CARTESIAN_POINT ( 'NONE',  ( -38.17536295476246977, 503.8073905683721136, -14.20200298773971426 ) ) ;
#15586=ORIENTED_EDGE ( 'NONE', *, *, #5509, .T. ) ;
#15587=CARTESIAN_POINT ( 'NONE',  ( -45.43829269268870519, 305.0573905683720000, -3.332260488124726638 ) ) ;
#15590=CARTESIAN_POINT ( 'NONE',  ( -22.27502019258947641, 346.9948905683720000, 15.47720386886985189 ) ) ;
#15591=CARTESIAN_POINT ( 'NONE',  ( -35.09675569278795138, 345.7448905683720568, 15.47720386886985366 ) ) ;
#15593=CARTESIAN_POINT ( 'NONE',  ( -40.01497788969913216, 280.4323905765655809, -16.95518130045146421 ) ) ;
#15595=CARTESIAN_POINT ( 'NONE',  ( -40.53162694259542320, 255.1198905683720284, 11.84573899990672885 ) ) ;
#15596=CARTESIAN_POINT ( 'NONE',  ( -43.59942232657301986, 200.4092789822994405, 1.616039188923344083 ) ) ;
#15597=CARTESIAN_POINT ( 'NONE',  ( -35.09675569278795138, 393.4948905683720000, -15.47720386886985544 ) ) ;
#15601=CARTESIAN_POINT ( 'NONE',  ( -28.68588794268870856, 312.8698905683720000, -16.75240474999999307 ) ) ;
#15602=CARTESIAN_POINT ( 'NONE',  ( -44.16309181155858710, 463.2448905683720568, -6.410867750099231266 ) ) ;
#15604=CARTESIAN_POINT ( 'NONE',  ( -48.68588794268871567, 447.5573905601784759, 3.978247347593168115 ) ) ;
#15605=CARTESIAN_POINT ( 'NONE',  ( -25.35362745456398059, 281.0573905683720568, -16.75240474999999307 ) ) ;
#15608=VERTEX_POINT ( 'NONE', #223 ) ;
#15610=CARTESIAN_POINT ( 'NONE',  ( -22.27502019258947996, 300.7448905683720568, -15.47720386886985544 ) ) ;
#15611=CARTESIAN_POINT ( 'NONE',  ( -42.88789093042843348, 366.3073905683720000, 9.489475012073734561 ) ) ;
#15612=CARTESIAN_POINT ( 'NONE',  ( -47.16347859291443712, 296.6198905601784759, -7.653668647301793193 ) ) ;
#15613=CARTESIAN_POINT ( 'NONE',  ( -11.73070664223726567, 516.0573905765655809, 11.32908994701042005 ) ) ;
#15614=CARTESIAN_POINT ( 'NONE',  ( -44.16309181155857289, 394.4948905683720000, 6.410867750099241924 ) ) ;
#15615=CARTESIAN_POINT ( 'NONE',  ( -35.09675569278793716, 237.2448905683720000, 15.47720386886985366 ) ) ;
#15616=CARTESIAN_POINT ( 'NONE',  ( -45.43829269268871940, 413.5573905683720000, -3.332260488124726638 ) ) ;
#15617=CARTESIAN_POINT ( 'NONE',  ( -14.54375231895776821, 348.2448905765656377, -14.14213562373094746 ) ) ;
#15619=CARTESIAN_POINT ( 'NONE',  ( -40.53162694259543031, 315.1198905683720568, 11.84573899990672885 ) ) ;
#15620=( NAMED_UNIT ( * ) SI_UNIT ( $, .STERADIAN. ) SOLID_ANGLE_UNIT ( ) );
#15621=CARTESIAN_POINT ( 'NONE',  ( -42.88789093042844769, 466.3073905683720568, 9.489475012073736337 ) ) ;
#15625=CARTESIAN_POINT ( 'NONE',  ( -10.20829729246297113, 226.3698905765656377, 7.653668647301790529 ) ) ;
#15626=CIRCLE ( 'NONE', #1461, 15.00000000000000355 ) ;
#15627=CARTESIAN_POINT ( 'NONE',  ( -44.16309181155857289, 374.7448905683720568, -6.410867750099231266 ) ) ;
#15630=EDGE_CURVE ( 'NONE', #9671, #4636, #18722, .T. ) ;
#15631=CARTESIAN_POINT ( 'NONE',  ( -48.68588794268872988, 516.9323905601784190, -3.978247347593158345 ) ) ;
#15632=CARTESIAN_POINT ( 'NONE',  ( -45.43829269268870519, 334.1823905683720000, 3.332260488124734632 ) ) ;
#15633=ORIENTED_EDGE ( 'NONE', *, *, #923, .T. ) ;
#15634=CARTESIAN_POINT ( 'NONE',  ( -16.84014894278200813, 500.1198905683720000, -11.84573899990672707 ) ) ;
#15635=VERTEX_POINT ( 'NONE', #2239 ) ;
#15636=CARTESIAN_POINT ( 'NONE',  ( -48.68588794268854514, 381.6823905765656377, -3.978247347593583783 ) ) ;
#15639=CARTESIAN_POINT ( 'NONE',  ( -48.68588794268869435, 231.9948905765656377, 0.000000000000000000 ) ) ;
#15640=CARTESIAN_POINT ( 'NONE',  ( -38.17536295476246266, 465.4323905683720000, 14.20200298773971781 ) ) ;
#15641=AXIS2_PLACEMENT_3D ( 'NONE', #15248, #434, #7001 ) ;
#15642=VERTEX_POINT ( 'NONE', #12064 ) ;
#15643=CARTESIAN_POINT ( 'NONE',  ( -40.53162694259545162, 492.6198905683720000, -11.84573899990672707 ) ) ;
#15644=CARTESIAN_POINT ( 'NONE',  ( -14.54375231895775222, 245.7448905765656093, 14.14213562373094568 ) ) ;
#15645=CARTESIAN_POINT ( 'NONE',  ( -47.16347859291445133, 412.6198905765656377, 7.653668647301805628 ) ) ;
#15646=CARTESIAN_POINT ( 'NONE',  ( -11.73070664223724080, 277.9323905765655809, -11.32908994701042538 ) ) ;
#15647=DIRECTION ( 'NONE',  ( -1.191790137725560488E-16, 1.000000000000000000, -0.000000000000000000 ) ) ;
#15650=EDGE_CURVE ( 'NONE', #15664, #16862, #5436, .T. ) ;
#15651=CARTESIAN_POINT ( 'NONE',  ( -14.54375231895775755, 258.2448905765656377, -14.14213562373094746 ) ) ;
#15655=CARTESIAN_POINT ( 'NONE',  ( -44.16309181155856578, 284.7448905683720568, -6.410867750099231266 ) ) ;
#15657=CARTESIAN_POINT ( 'NONE',  ( -32.01814843081345430, 437.5573905683720000, 16.75240474999999307 ) ) ;
#15658=CARTESIAN_POINT ( 'NONE',  ( -45.43829269268869808, 265.3698905683720000, 0.000000000000000000 ) ) ;
#15660=LINE ( 'NONE', #5583, #19818 ) ;
#15662=CARTESIAN_POINT ( 'NONE',  ( -14.48388495494901029, 479.4323905683720568, 9.489475012073731008 ) ) ;
#15664=VERTEX_POINT ( 'NONE', #13701 ) ;
#15665=DIRECTION ( 'NONE',  ( -1.000000000000000000, 0.000000000000000000, 0.000000000000000000 ) ) ;
#15666=CARTESIAN_POINT ( 'NONE',  ( -16.84014894278197261, 247.6198905683720284, 11.84573899990672530 ) ) ;
#15669=LINE ( 'NONE', #10986, #16276 ) ;
#15670=CARTESIAN_POINT ( 'NONE',  ( -24.70764059509557597, 469.1823905765656377, -19.99999999999999289 ) ) ;
#15673=CARTESIAN_POINT ( 'NONE',  ( -25.35362745456396283, 228.1823905683720284, 16.75240474999998952 ) ) ;
#15675=CARTESIAN_POINT ( 'NONE',  ( -19.19641293061500065, 511.9323905683721136, -14.20200298773971603 ) ) ;
#15676=DIRECTION ( 'NONE',  ( -1.191790137725560488E-16, 1.000000000000000000, -0.000000000000000000 ) ) ;
#15677=CARTESIAN_POINT ( 'NONE',  ( -14.48388495494898542, 239.8073905683720284, -9.489475012073736337 ) ) ;
#15678=CARTESIAN_POINT ( 'NONE',  ( -44.16309181155857289, 334.7448905683720568, -6.410867750099231266 ) ) ;
#15680=CARTESIAN_POINT ( 'NONE',  ( -36.33955658999050797, 303.8698905765656377, 18.47759065022572500 ) ) ;
#15682=CARTESIAN_POINT ( 'NONE',  ( -45.43829269268871229, 393.5573905683720568, -3.332260488124726194 ) ) ;
#15683=CARTESIAN_POINT ( 'NONE',  ( -45.43829269268873361, 535.3698905683720568, 0.000000000000000000 ) ) ;
#15684=CARTESIAN_POINT ( 'NONE',  ( -47.16347859291444422, 386.6198905601784759, -7.653668647301793193 ) ) ;
#15689=CARTESIAN_POINT ( 'NONE',  ( -11.93348319268873858, 510.6823905683720000, -3.332260488124732856 ) ) ;
#15690=CARTESIAN_POINT ( 'NONE',  ( -48.68588794268870146, 291.9948905765656377, 0.000000000000000000 ) ) ;
#15692=CARTESIAN_POINT ( 'NONE',  ( -22.27502019258946930, 298.4948905683720568, 15.47720386886985189 ) ) ;
#15693=ORIENTED_EDGE ( 'NONE', *, *, #12732, .F. ) ;
#15694=CARTESIAN_POINT ( 'NONE',  ( -28.68588794268870856, 336.3698905683720000, 16.75240474999999307 ) ) ;
#15695=CARTESIAN_POINT ( 'NONE',  ( -38.17536295476245556, 342.3073905683721136, -14.20200298773971426 ) ) ;
#15697=CARTESIAN_POINT ( 'NONE',  ( -32.66413529028186957, 279.8073905765655809, -19.99999999999999289 ) ) ;
#15699=CARTESIAN_POINT ( 'NONE',  ( -11.93348319268870661, 239.1823905683720284, -3.332260488124732856 ) ) ;
#15700=CARTESIAN_POINT ( 'NONE',  ( -42.93765923600279422, 203.3731313234726201, 4.678819197459195500 ) ) ;
#15701=CARTESIAN_POINT ( 'NONE',  ( -44.16309181155857999, 394.7448905683720568, -6.410867750099231266 ) ) ;
#15703=CARTESIAN_POINT ( 'NONE',  ( -36.33955658999052218, 450.1198905765655809, -18.47759065022572855 ) ) ;
#15704=CARTESIAN_POINT ( 'NONE',  ( -40.01497788969916058, 510.4323905765656377, -16.95518130045146421 ) ) ;
#15705=CARTESIAN_POINT ( 'NONE',  ( -45.43829269268871229, 433.5573905683719431, -3.332260488124726194 ) ) ;
#15707=CARTESIAN_POINT ( 'NONE',  ( -8.685887942688731655, 451.9323905601784759, 3.978247347593161010 ) ) ;
#15714=CARTESIAN_POINT ( 'NONE',  ( -45.64106924314017988, 318.1823905601784759, 11.32908994701042715 ) ) ;
#15715=ADVANCED_FACE ( 'NONE', ( #11561 ), #3846, .T. ) ;
#15716=CARTESIAN_POINT ( 'NONE',  ( -38.17536295476244135, 295.4323905683720000, 14.20200298773971781 ) ) ;
#15718=CARTESIAN_POINT ( 'NONE',  ( -35.09675569278795138, 357.2448905683720000, 15.47720386886985366 ) ) ;
#15720=CARTESIAN_POINT ( 'NONE',  ( -40.01497788969915348, 523.5573905765655809, 16.95518130045146776 ) ) ;
#15721=CARTESIAN_POINT ( 'NONE',  ( -22.27502019258947996, 396.9948905683720568, 15.47720386886985189 ) ) ;
#15722=CARTESIAN_POINT ( 'NONE',  ( -38.17536295476244135, 243.8073905683720284, -14.20200298773971426 ) ) ;
#15723=CARTESIAN_POINT ( 'NONE',  ( -45.43829269268871940, 413.8698905683720568, 0.000000000000000000 ) ) ;
#15724=CARTESIAN_POINT ( 'NONE',  ( -28.68588794268871567, 349.4948905765656377, -19.99999999999999289 ) ) ;
#15726=CARTESIAN_POINT ( 'NONE',  ( -45.43829269268870519, 304.1823905683720568, 3.332260488124734632 ) ) ;
#15727=SHAPE_REPRESENTATION_RELATIONSHIP ( 'NONE' , 'NONE' ,  #4206, #11515 ) ;
#15728=CARTESIAN_POINT ( 'NONE',  ( -42.88789093042844769, 464.4323905683720000, -9.489475012073736337 ) ) ;
#15730=CARTESIAN_POINT ( 'NONE',  ( -48.68588794268878672, 512.3073905765656946, 3.978247347593061978 ) ) ;
#15733=CARTESIAN_POINT ( 'NONE',  ( -28.68588794268871567, 362.8698905683720000, -16.75240474999999307 ) ) ;
#15735=CARTESIAN_POINT ( 'NONE',  ( -45.64106924314020119, 508.1823905601784759, 11.32908994701042715 ) ) ;
#15736=CARTESIAN_POINT ( 'NONE',  ( -11.93348319268872260, 348.5573905683720000, 3.332260488124728415 ) ) ;
#15738=CARTESIAN_POINT ( 'NONE',  ( -38.17536295476246977, 505.4323905683720568, 14.20200298773971781 ) ) ;
#15740=CARTESIAN_POINT ( 'NONE',  ( -24.70764059509556176, 354.4323905601784759, -19.99999999999999289 ) ) ;
#15741=CARTESIAN_POINT ( 'NONE',  ( -10.20829729246298001, 316.3698905765656377, 7.653668647301790529 ) ) ;
#15742=CARTESIAN_POINT ( 'NONE',  ( -19.19641293061498999, 421.9323905683720000, -14.20200298773971603 ) ) ;
#15743=CARTESIAN_POINT ( 'NONE',  ( -36.33955658999050087, 290.1198905765656377, -18.47759065022572855 ) ) ;
#15745=CARTESIAN_POINT ( 'NONE',  ( -35.09675569278796559, 465.7448905683720568, 15.47720386886985366 ) ) ;
#15746=ORIENTED_EDGE ( 'NONE', *, *, #2098, .F. ) ;
#15747=CARTESIAN_POINT ( 'NONE',  ( -28.68588794268872988, 471.3698905683720568, -16.75240474999999307 ) ) ;
#15749=CARTESIAN_POINT ( 'NONE',  ( -28.68588794268871567, 394.4948905765656377, 19.99999999999999289 ) ) ;
#15751=CARTESIAN_POINT ( 'NONE',  ( -17.35679799567829562, 368.5573905765655809, -16.95518130045146421 ) ) ;
#15752=CARTESIAN_POINT ( 'NONE',  ( -8.685887942688728103, 416.9948905765656377, -2.449293598294705724E-15 ) ) ;
#15757=CARTESIAN_POINT ( 'NONE',  ( -13.20868407381885135, 280.9948905683720000, -6.410867750099233042 ) ) ;
#15758=CARTESIAN_POINT ( 'NONE',  ( -10.20829729246297291, 252.8698905601785043, -7.653668647301794969 ) ) ;
#15760=CARTESIAN_POINT ( 'NONE',  ( -45.43829269268871229, 435.0573905683720568, -3.332260488124726194 ) ) ;
#15761=CARTESIAN_POINT ( 'NONE',  ( -21.03221929538692692, 398.8698905765656377, -18.47759065022572855 ) ) ;
#15762=CARTESIAN_POINT ( 'NONE',  ( -11.93348319268871016, 260.0573905683720000, 3.332260488124728415 ) ) ;
#15764=CARTESIAN_POINT ( 'NONE',  ( -8.685887942688605534, 477.3073905765656377, -3.978247347592846594 ) ) ;
#15765=ORIENTED_EDGE ( 'NONE', *, *, #3408, .T. ) ;
#15766=CARTESIAN_POINT ( 'NONE',  ( -45.43829269268872650, 485.6823905683721136, 3.332260488124734632 ) ) ;
#15769=CARTESIAN_POINT ( 'NONE',  ( -8.685887942688456320, 362.5573905601784190, -3.978247347592526850 ) ) ;
#15770=CARTESIAN_POINT ( 'NONE',  ( -38.17536295476244135, 232.3073905683720568, -14.20200298773971426 ) ) ;
#15772=CARTESIAN_POINT ( 'NONE',  ( -28.68588794268873698, 521.3698905683720568, -16.75240474999999307 ) ) ;
#15775=CARTESIAN_POINT ( 'NONE',  ( -45.64106924314020119, 471.0573905765656377, -11.32908994701042715 ) ) ;
#15776=CARTESIAN_POINT ( 'NONE',  ( -8.685887942688809815, 351.9323905601785327, 3.978247347593374172 ) ) ;
#15779=CARTESIAN_POINT ( 'NONE',  ( -10.20829729246299600, 452.8698905601785327, -7.653668647301794969 ) ) ;
#15780=CARTESIAN_POINT ( 'NONE',  ( -40.53162694259542320, 226.6198905683720000, 11.84573899990672885 ) ) ;
#15782=CARTESIAN_POINT ( 'NONE',  ( -19.19641293061499709, 508.8073905683720000, 14.20200298773971426 ) ) ;
#15784=CARTESIAN_POINT ( 'NONE',  ( -45.43829269268869098, 244.1823905683720568, 3.332260488124734632 ) ) ;
#15785=CARTESIAN_POINT ( 'NONE',  ( -32.01814843081344719, 337.5573905683720000, 16.75240474999999307 ) ) ;
#15787=CARTESIAN_POINT ( 'NONE',  ( -48.68588794268880093, 357.5573905601784190, 3.978247347592954952 ) ) ;
#15789=CARTESIAN_POINT ( 'NONE',  ( -25.35362745456398414, 386.6823905683720568, 16.75240474999998952 ) ) ;
#15790=CARTESIAN_POINT ( 'NONE',  ( -8.685887942688713892, 223.9102039777116886, 2.449293598294704541E-15 ) ) ;
#15791=CARTESIAN_POINT ( 'NONE',  ( -14.54375231895777176, 383.4948905601784759, -14.14213562373094746 ) ) ;
#15794=ORIENTED_EDGE ( 'NONE', *, *, #7094, .T. ) ;
#15795=CARTESIAN_POINT ( 'NONE',  ( -40.01497788969914637, 405.6823905601785327, -16.95518130045146421 ) ) ;
#15798=CARTESIAN_POINT ( 'NONE',  ( -16.84014894278200458, 499.1198905683720000, 11.84573899990672530 ) ) ;
#15801=CARTESIAN_POINT ( 'NONE',  ( -44.16309181155856578, 304.7448905683720568, -6.410867750099231266 ) ) ;
#15803=CARTESIAN_POINT ( 'NONE',  ( -40.53162694259543741, 332.6198905683720000, -11.84573899990672707 ) ) ;
#15804=CARTESIAN_POINT ( 'NONE',  ( -42.88789093042843348, 352.9323905683721136, -9.489475012073734561 ) ) ;
#15806=CARTESIAN_POINT ( 'NONE',  ( -36.33955658999050797, 283.8698905765656377, 18.47759065022572500 ) ) ;
#15808=CARTESIAN_POINT ( 'NONE',  ( -13.20868407381884602, 238.2448905683720000, 6.410867750099229490 ) ) ;
#15810=CARTESIAN_POINT ( 'NONE',  ( -13.20868407381886200, 389.7448905683720000, 6.410867750099229490 ) ) ;
#15812=AXIS2_PLACEMENT_3D ( 'NONE', #810, #7378, #12364 ) ;
#15815=CARTESIAN_POINT ( 'NONE',  ( -21.03221929538690915, 244.1198905601784759, -18.47759065022572855 ) ) ;
#15816=CARTESIAN_POINT ( 'NONE',  ( -32.01814843081345430, 446.0573905683720568, 16.75240474999999307 ) ) ;
#15818=CARTESIAN_POINT ( 'NONE',  ( -48.68588794268871567, 437.5573905601785327, 3.978247347593168115 ) ) ;
#15821=VERTEX_POINT ( 'NONE', #17576 ) ;
#15824=CARTESIAN_POINT ( 'NONE',  ( -14.54375231895776466, 323.4948905601784759, -14.14213562373094746 ) ) ;
#15826=CARTESIAN_POINT ( 'NONE',  ( -44.16309181155856578, 365.9948905683720568, 6.410867750099241924 ) ) ;
#15828=CARTESIAN_POINT ( 'NONE',  ( -42.82802356641968089, 523.2448905765656946, 14.14213562373094923 ) ) ;
#15829=CARTESIAN_POINT ( 'NONE',  ( -28.68588794268871922, 401.3698905683720000, -16.75240474999999307 ) ) ;
#15830=CARTESIAN_POINT ( 'NONE',  ( -14.48388495494898365, 239.4323905683720000, 9.489475012073732785 ) ) ;
#15831=CARTESIAN_POINT ( 'NONE',  ( -40.53162694259544452, 405.1198905683720000, 11.84573899990672885 ) ) ;
#15832=CARTESIAN_POINT ( 'NONE',  ( -8.685887942688719221, 347.3073905765656377, -3.978247347593165895 ) ) ;
#15833=CARTESIAN_POINT ( 'NONE',  ( -19.19641293061497578, 310.4323905683720568, -14.20200298773971603 ) ) ;
#15834=CARTESIAN_POINT ( 'NONE',  ( -28.68588794268872633, 452.8698905683720000, -16.75240474999999307 ) ) ;
#15838=CARTESIAN_POINT ( 'NONE',  ( -35.09675569278794427, 373.4948905683720568, -15.47720386886985544 ) ) ;
#15839=CARTESIAN_POINT ( 'NONE',  ( -42.88789093042844769, 494.8073905683720000, 9.489475012073736337 ) ) ;
#15841=CARTESIAN_POINT ( 'NONE',  ( -32.66413529028189089, 499.4323905601784759, 19.99999999999999289 ) ) ;
#15842=CARTESIAN_POINT ( 'NONE',  ( -44.16309181155856578, 323.2448905683720000, -6.410867750099231266 ) ) ;
#15844=CARTESIAN_POINT ( 'NONE',  ( -11.93348319268873858, 508.8698905683719431, -2.051577885510841163E-15 ) ) ;
#15847=CARTESIAN_POINT ( 'NONE',  ( -42.82802356641965247, 313.2448905765656377, 14.14213562373094923 ) ) ;
#15850=CARTESIAN_POINT ( 'NONE',  ( -45.43829269268871940, 425.3698905683720568, 0.000000000000000000 ) ) ;
#15851=CARTESIAN_POINT ( 'NONE',  ( -24.70764059509555111, 289.1823905765656377, -19.99999999999999289 ) ) ;
#15852=CARTESIAN_POINT ( 'NONE',  ( -42.82802356641968089, 520.7448905765656946, -14.14213562373094746 ) ) ;
#15853=CARTESIAN_POINT ( 'NONE',  ( -44.16309181155857999, 464.4948905683720000, 6.410867750099241924 ) ) ;
#15855=CARTESIAN_POINT ( 'NONE',  ( -28.68588794268872633, 466.3698905683720000, 16.75240474999999307 ) ) ;
#15856=CARTESIAN_POINT ( 'NONE',  ( -48.68588794268871567, 401.9948905765656377, 0.000000000000000000 ) ) ;
#15859=CARTESIAN_POINT ( 'NONE',  ( -24.70764059509555821, 369.1823905765655240, -19.99999999999999289 ) ) ;
#15861=CARTESIAN_POINT ( 'NONE',  ( -10.20829729246300133, 486.3698905765655809, 7.653668647301790529 ) ) ;
#15863=CARTESIAN_POINT ( 'NONE',  ( -43.27177863848956463, 223.9102039777116033, 11.41195197239935233 ) ) ;
#15865=CARTESIAN_POINT ( 'NONE',  ( -8.685887942688708563, 252.2448905601784475, -2.449293598294705724E-15 ) ) ;
#15866=CARTESIAN_POINT ( 'NONE',  ( -10.20829729246298712, 366.3698905765655809, 7.653668647301790529 ) ) ;
#15867=CARTESIAN_POINT ( 'NONE',  ( -35.09675569278795138, 433.4948905683720568, -15.47720386886985544 ) ) ;
#15869=CARTESIAN_POINT ( 'NONE',  ( -40.53162694259542320, 256.6198905683720568, 11.84573899990672885 ) ) ;
#15870=EDGE_LOOP ( 'NONE', ( #18035, #19258, #6970, #5286, #13210, #4781 ) ) ;
#15872=CARTESIAN_POINT ( 'NONE',  ( -28.68588794268872988, 479.4948905765656377, -19.99999999999999289 ) ) ;
#15874=CARTESIAN_POINT ( 'NONE',  ( -32.01814843081345430, 473.1823905683720000, -16.75240474999999307 ) ) ;
#15875=ORIENTED_EDGE ( 'NONE', *, *, #1041, .F. ) ;
#15876=CARTESIAN_POINT ( 'NONE',  ( -14.54375231895776999, 363.4948905601784759, -14.14213562373094746 ) ) ;
#15877=CARTESIAN_POINT ( 'NONE',  ( -32.01814843081343298, 231.6823905683720568, -16.75240474999999307 ) ) ;
#15878=VERTEX_POINT ( 'NONE', #20931 ) ;
#15879=CARTESIAN_POINT ( 'NONE',  ( -35.09675569278796559, 521.9948905683720568, -15.47720386886985544 ) ) ;
#15882=CARTESIAN_POINT ( 'NONE',  ( -40.01497788969915348, 470.4323905765656377, -16.95518130045146421 ) ) ;
#15884=FACE_OUTER_BOUND ( 'NONE', #21053, .T. ) ;
#15888=CARTESIAN_POINT ( 'NONE',  ( -28.68588794268869790, 221.3698905683720284, -16.75240474999999307 ) ) ;
#15889=CARTESIAN_POINT ( 'NONE',  ( -11.93348319268872260, 340.6823905683720000, -3.332260488124732856 ) ) ;
#15893=CARTESIAN_POINT ( 'NONE',  ( -11.93348319268872437, 388.5573905683720000, 3.332260488124728415 ) ) ;
#15895=DIRECTION ( 'NONE',  ( 0.000000000000000000, -0.000000000000000000, 1.000000000000000000 ) ) ;
#15896=CARTESIAN_POINT ( 'NONE',  ( -48.68588794268870856, 376.9323905601785327, -3.978247347593158345 ) ) ;
#15900=CARTESIAN_POINT ( 'NONE',  ( -19.19641293061499709, 508.8073905683720000, 14.20200298773971426 ) ) ;
#15902=VERTEX_POINT ( 'NONE', #4491 ) ;
#15903=CARTESIAN_POINT ( 'NONE',  ( -40.53162694259543031, 304.1198905683720000, -11.84573899990672707 ) ) ;
#15905=CARTESIAN_POINT ( 'NONE',  ( -42.88789093042842637, 322.9323905683720000, -9.489475012073736337 ) ) ;
#15906=CARTESIAN_POINT ( 'NONE',  ( -28.68588794268870501, 259.4948905765655809, -19.99999999999999289 ) ) ;
#15908=CARTESIAN_POINT ( 'NONE',  ( -44.16309181155855867, 253.2448905683720284, -6.410867750099231266 ) ) ;
#15909=CARTESIAN_POINT ( 'NONE',  ( -11.93348319268872437, 390.6823905683720568, -3.332260488124732856 ) ) ;
#15914=CARTESIAN_POINT ( 'NONE',  ( -48.68588794268867304, 511.6823905765656377, -3.978247347593264927 ) ) ;
#15915=CARTESIAN_POINT ( 'NONE',  ( -14.48388495494900496, 437.9323905683720000, 9.489475012073732785 ) ) ;
#15916=ORIENTED_EDGE ( 'NONE', *, *, #18023, .F. ) ;
#15917=CARTESIAN_POINT ( 'NONE',  ( -14.54375231895778064, 443.4948905601784759, -14.14213562373094746 ) ) ;
#15918=ORIENTED_EDGE ( 'NONE', *, *, #12797, .T. ) ;
#15919=ORIENTED_EDGE ( 'NONE', *, *, #1555, .T. ) ;
#15922=CARTESIAN_POINT ( 'NONE',  ( -8.685887942688715668, 321.9323905601784759, 3.978247347593161010 ) ) ;
#15924=CARTESIAN_POINT ( 'NONE',  ( -38.17536295476244845, 366.9323905683721136, 14.20200298773971781 ) ) ;
#15926=DIRECTION ( 'NONE',  ( -1.191790137725560488E-16, 1.000000000000000000, -0.000000000000000000 ) ) ;
#15928=CARTESIAN_POINT ( 'NONE',  ( -14.54375231895778420, 505.7448905765655809, 14.14213562373094568 ) ) ;
#15929=CARTESIAN_POINT ( 'NONE',  ( -16.84014894278199037, 387.6198905683720568, 11.84573899990672530 ) ) ;
#15930=CARTESIAN_POINT ( 'NONE',  ( -40.53162694259542320, 236.6198905683720284, 11.84573899990672885 ) ) ;
#15931=AXIS2_PLACEMENT_3D ( 'NONE', #19504, #16166, #3179 ) ;
#15932=CARTESIAN_POINT ( 'NONE',  ( -28.68588794268871922, 406.3698905683720000, 16.75240474999999307 ) ) ;
#15933=CARTESIAN_POINT ( 'NONE',  ( -48.68588794268870856, 331.6823905765655809, -3.978247347593158345 ) ) ;
#15934=CARTESIAN_POINT ( 'NONE',  ( -47.16347859291443712, 326.6198905601784759, -7.653668647301793193 ) ) ;
#15935=CARTESIAN_POINT ( 'NONE',  ( -44.16309181155856578, 303.2448905683720000, -6.410867750099231266 ) ) ;
#15937=CARTESIAN_POINT ( 'NONE',  ( -13.20868407381887089, 450.9948905683720000, -6.410867750099233042 ) ) ;
#15943=CARTESIAN_POINT ( 'NONE',  ( -45.43829269268870519, 365.0573905683720568, -3.332260488124726194 ) ) ;
#15945=CARTESIAN_POINT ( 'NONE',  ( -38.17536295476246266, 495.4323905683720000, 14.20200298773971781 ) ) ;
#15947=CARTESIAN_POINT ( 'NONE',  ( -47.16347859291445843, 497.8698905601784759, 7.653668647301805628 ) ) ;
#15948=CARTESIAN_POINT ( 'NONE',  ( -13.20868407381885490, 319.4948905683720000, -6.410867750099233042 ) ) ;
#15952=CARTESIAN_POINT ( 'NONE',  ( -47.16347859291443712, 312.6198905765655809, 7.653668647301805628 ) ) ;
#15953=CARTESIAN_POINT ( 'NONE',  ( -45.43829269268871940, 415.3698905683720568, 0.000000000000000000 ) ) ;
#15954=CARTESIAN_POINT ( 'NONE',  ( -28.68588794268871567, 394.4948905765656377, 19.99999999999999289 ) ) ;
#15956=CARTESIAN_POINT ( 'NONE',  ( -13.20868407381887089, 449.4948905683720568, -6.410867750099233042 ) ) ;
#15957=ORIENTED_EDGE ( 'NONE', *, *, #13008, .F. ) ;
#15958=CARTESIAN_POINT ( 'NONE',  ( -45.43829269268872650, 463.5573905683720568, -3.332260488124726638 ) ) ;
#15960=CARTESIAN_POINT ( 'NONE',  ( -8.685887942688726326, 396.9948905765656377, -2.449293598294705724E-15 ) ) ;
#15963=CARTESIAN_POINT ( 'NONE',  ( -48.68588794268872277, 491.9948905765656377, 0.000000000000000000 ) ) ;
#15968=CARTESIAN_POINT ( 'NONE',  ( -38.53300430798842058, 223.9102039777116602, 16.90666462915203638 ) ) ;
#15970=( BOUNDED_CURVE ( )  B_SPLINE_CURVE ( 2, ( #7960, #1936, #13287, #6667, #16530, #1715, #18353, #19872, #15227, #11964, #5263, #420, #11649, #3435, #8282, #9909, #6986 ),
 .UNSPECIFIED., .F., .T. ) 
 B_SPLINE_CURVE_WITH_KNOTS ( ( 3, 2, 2, 2, 2, 2, 2, 2, 3 ),
 ( 0.3593750000000001110, 0.3613281250000001110, 0.3632812500000001110, 0.3652343750000001110, 0.3671875000000001110, 0.3691406250000001665, 0.3710937500000001665, 0.3730468750000001665, 0.3750000000000001665 ),
 .UNSPECIFIED. ) 
 CURVE ( )  GEOMETRIC_REPRESENTATION_ITEM ( )  RATIONAL_B_SPLINE_CURVE ( ( 0.9999999999999988898, 0.9807852804032315408, 1.000000000000000000, 0.9807852804032304306, 1.000000000000000000, 0.9807852804032304306, 1.000000000000000000, 0.9807852804032304306, 1.000000000000000000, 0.9807852804032304306, 1.000000000000000000, 0.9807852804032304306, 1.000000000000000000, 0.9807852804032304306, 1.000000000000000000, 0.9807852804032287652, 1.000000000000001554 ) ) 
 REPRESENTATION_ITEM ( '' )  );
#15972=CARTESIAN_POINT ( 'NONE',  ( -11.73070664223723192, 241.3073905601784759, 11.32908994701042005 ) ) ;
#15974=CARTESIAN_POINT ( 'NONE',  ( -22.27502019258949417, 422.2448905683720568, -15.47720386886985544 ) ) ;
#15975=CARTESIAN_POINT ( 'NONE',  ( -47.16347859291444422, 386.6198905601784759, -7.653668647301793193 ) ) ;
#15976=CARTESIAN_POINT ( 'NONE',  ( -44.16309181155855157, 255.9948905683720568, 6.410867750099241924 ) ) ;
#15978=ORIENTED_EDGE ( 'NONE', *, *, #19227, .F. ) ;
#15979=CARTESIAN_POINT ( 'NONE',  ( -21.03221929538693757, 478.8698905765656377, -18.47759065022572855 ) ) ;
#15980=ORIENTED_EDGE ( 'NONE', *, *, #15503, .F. ) ;
#15981=CARTESIAN_POINT ( 'NONE',  ( -40.53162694259545162, 464.1198905683720568, -11.84573899990672707 ) ) ;
#15982=CARTESIAN_POINT ( 'NONE',  ( -42.82802356641964536, 230.7448905765656093, -14.14213562373094746 ) ) ;
#15984=VERTEX_POINT ( 'NONE', #2874 ) ;
#15985=CARTESIAN_POINT ( 'NONE',  ( -8.685887942689042518, 526.6823905765655809, 3.978247347593879546 ) ) ;
#15986=CARTESIAN_POINT ( 'NONE',  ( -45.43829269268869808, 233.8698905683720284, 0.000000000000000000 ) ) ;
#15989=CARTESIAN_POINT ( 'NONE',  ( -40.53162694259545873, 532.6198905683720568, -11.84573899990672707 ) ) ;
#15992=CARTESIAN_POINT ( 'NONE',  ( -8.685887942688735208, 457.3073905765655809, -3.978247347593165895 ) ) ;
#15993=PRODUCT ( 'Coarse Pitch Steep Screw Shaft', 'Coarse Pitch Steep Screw Shaft', '', ( #8676 ) ) ;
#15994=CARTESIAN_POINT ( 'NONE',  ( -40.01497788969913216, 348.8073905601784759, 16.95518130045146776 ) ) ;
#15996=CARTESIAN_POINT ( 'NONE',  ( -24.70764059509554755, 239.1823905765656093, -19.99999999999999289 ) ) ;
#15998=CARTESIAN_POINT ( 'NONE',  ( -10.23462588383483762, 223.9102039777117454, 7.884011575492554158 ) ) ;
#15999=CARTESIAN_POINT ( 'NONE',  ( -35.09675569278793716, 225.7448905683720568, 15.47720386886985366 ) ) ;
#16000=CARTESIAN_POINT ( 'NONE',  ( -19.19641293061497933, 318.8073905683720568, 14.20200298773971426 ) ) ;
#16002=CARTESIAN_POINT ( 'NONE',  ( -32.66413529028185536, 235.0573905601785043, -19.99999999999999289 ) ) ;
#16004=CARTESIAN_POINT ( 'NONE',  ( -38.17536295476244845, 313.8073905683720000, -14.20200298773971426 ) ) ;
#16005=CARTESIAN_POINT ( 'NONE',  ( -28.68588794268871922, 381.3698905683720568, -16.75240474999999307 ) ) ;
#16006=CARTESIAN_POINT ( 'NONE',  ( -32.01814843081346140, 527.5573905683720568, 16.75240474999999307 ) ) ;
#16008=CARTESIAN_POINT ( 'NONE',  ( -36.33955658999050797, 385.3698905601785327, -18.47759065022572855 ) ) ;
#16009=CARTESIAN_POINT ( 'NONE',  ( -48.68588794268869435, 231.9948905765656377, 0.000000000000000000 ) ) ;
#16012=CARTESIAN_POINT ( 'NONE',  ( -44.16309181155858710, 494.7448905683720000, -6.410867750099231266 ) ) ;
#16015=CARTESIAN_POINT ( 'NONE',  ( -35.09675569278794427, 307.2448905683720000, 15.47720386886985366 ) ) ;
#16016=CARTESIAN_POINT ( 'NONE',  ( -22.27502019258948351, 320.7448905683720000, -15.47720386886985544 ) ) ;
#16017=AXIS2_PLACEMENT_3D ( 'NONE', #17408, #4092, #10573 ) ;
#16018=CARTESIAN_POINT ( 'NONE',  ( -24.70764059509553690, 264.8073905765656377, 19.99999999999998934 ) ) ;
#16021=VECTOR ( 'NONE', #15119, 1000.000000000000000 ) ;
#16022=CARTESIAN_POINT ( 'NONE',  ( -19.19641293061498644, 388.8073905683720568, 14.20200298773971426 ) ) ;
#16023=CARTESIAN_POINT ( 'NONE',  ( -11.73070664223724613, 333.1823905601784190, -11.32908994701042538 ) ) ;
#16025=CARTESIAN_POINT ( 'NONE',  ( -8.685887942688617969, 242.5573905601784759, -3.978247347592952732 ) ) ;
#16026=CARTESIAN_POINT ( 'NONE',  ( -38.17536295476246266, 442.3073905683721136, -14.20200298773971426 ) ) ;
#16029=CARTESIAN_POINT ( 'NONE',  ( -48.68588794268871567, 446.9323905601784759, -3.978247347593158345 ) ) ;
#16034=CARTESIAN_POINT ( 'NONE',  ( -17.35679799567828852, 320.6823905601784759, 16.95518130045146421 ) ) ;
#16039=CARTESIAN_POINT ( 'NONE',  ( -44.16309181155857289, 354.7448905683720568, -6.410867750099231266 ) ) ;
#16041=CARTESIAN_POINT ( 'NONE',  ( -40.01497788969915348, 500.4323905765656946, -16.95518130045146421 ) ) ;
#16042=CARTESIAN_POINT ( 'NONE',  ( -11.93348319268872260, 378.8698905683720000, -2.051577885510841163E-15 ) ) ;
#16043=CARTESIAN_POINT ( 'NONE',  ( -32.66413529028186247, 309.8073905765656377, -19.99999999999999289 ) ) ;
#16044=CARTESIAN_POINT ( 'NONE',  ( -40.53162694259544452, 412.6198905683720568, -11.84573899990672707 ) ) ;
#16045=CARTESIAN_POINT ( 'NONE',  ( -8.685887942688719221, 326.9948905765656377, -2.449293598294705724E-15 ) ) ;
#16047=CARTESIAN_POINT ( 'NONE',  ( -13.20868407381885312, 299.4948905683720568, -6.410867750099233042 ) ) ;
#16048=CARTESIAN_POINT ( 'NONE',  ( -14.48388495494900674, 449.4323905683720568, 9.489475012073732785 ) ) ;
#16049=FACE_OUTER_BOUND ( 'NONE', #14859, .T. ) ;
#16051=DIRECTION ( 'NONE',  ( -1.000000000000000000, 0.000000000000000000, 0.000000000000000000 ) ) ;
#16053=CARTESIAN_POINT ( 'NONE',  ( -16.84014894278199037, 371.6198905683720000, -11.84573899990672707 ) ) ;
#16054=CARTESIAN_POINT ( 'NONE',  ( -11.93348319268873858, 498.8698905683720000, -2.051577885510841163E-15 ) ) ;
#16055=CARTESIAN_POINT ( 'NONE',  ( -48.68588794268872277, 507.2448905601785327, 0.000000000000000000 ) ) ;
#16056=CARTESIAN_POINT ( 'NONE',  ( -40.53162694259543031, 315.1198905683720568, 11.84573899990672885 ) ) ;
#16058=CARTESIAN_POINT ( 'NONE',  ( -14.54375231895775400, 260.9948905601784759, 14.14213562373094568 ) ) ;
#16062=CARTESIAN_POINT ( 'NONE',  ( -16.84014894278199748, 431.6198905683720000, -11.84573899990672707 ) ) ;
#16065=CARTESIAN_POINT ( 'NONE',  ( -45.43829269268871940, 443.8698905683720568, 0.000000000000000000 ) ) ;
#16067=CARTESIAN_POINT ( 'NONE',  ( -28.68588794268872277, 456.3698905683720000, 16.75240474999999307 ) ) ;
#16068=CARTESIAN_POINT ( 'NONE',  ( -14.54375231895777532, 413.4948905601784759, -14.14213562373094746 ) ) ;
#16069=CARTESIAN_POINT ( 'NONE',  ( -17.35679799567830273, 388.5573905765656377, -16.95518130045146421 ) ) ;
#16070=CARTESIAN_POINT ( 'NONE',  ( -42.82802356641965957, 370.7448905765656377, -14.14213562373094746 ) ) ;
#16075=CARTESIAN_POINT ( 'NONE',  ( -11.93348319268872793, 420.6823905683720000, -3.332260488124732856 ) ) ;
#16077=CARTESIAN_POINT ( 'NONE',  ( -40.53162694259542320, 254.1198905683720284, -11.84573899990672707 ) ) ;
#16080=CARTESIAN_POINT ( 'NONE',  ( -10.20829729246299422, 426.3698905765656377, 7.653668647301790529 ) ) ;
#16082=CARTESIAN_POINT ( 'NONE',  ( -28.68588794268872988, 472.8698905683720568, -16.75240474999999307 ) ) ;
#16083=CARTESIAN_POINT ( 'NONE',  ( -47.16347859291443001, 231.3698905765656093, -7.653668647301793193 ) ) ;
#16085=CARTESIAN_POINT ( 'NONE',  ( -47.16347859291446554, 522.6198905765655809, 7.653668647301805628 ) ) ;
#16086=CARTESIAN_POINT ( 'NONE',  ( -11.93348319268870661, 228.5573905683720568, 3.332260488124728415 ) ) ;
#16088=CARTESIAN_POINT ( 'NONE',  ( -19.19641293061500420, 530.4323905683720568, -14.20200298773971603 ) ) ;
#16090=CARTESIAN_POINT ( 'NONE',  ( -28.68588794268872277, 434.4948905765655809, 19.99999999999999289 ) ) ;
#16094=CARTESIAN_POINT ( 'NONE',  ( -32.66413529028186247, 289.4323905601784190, 19.99999999999999289 ) ) ;
#16095=( BOUNDED_CURVE ( )  B_SPLINE_CURVE ( 2, ( #7634, #10659, #2356, #12518, #20735, #14368, #17591, #12298, #17277, #14148, #10769, #2567, #15876, #2463, #2783, #15769, #9371 ),
 .UNSPECIFIED., .F., .T. ) 
 B_SPLINE_CURVE_WITH_KNOTS ( ( 3, 2, 2, 2, 2, 2, 2, 2, 3 ),
 ( 0.5312500000000003331, 0.5332031250000003331, 0.5351562500000003331, 0.5371093750000003331, 0.5390625000000003331, 0.5410156250000003331, 0.5429687500000003331, 0.5449218750000003331, 0.5468750000000003331 ),
 .UNSPECIFIED. ) 
 CURVE ( )  GEOMETRIC_REPRESENTATION_ITEM ( )  RATIONAL_B_SPLINE_CURVE ( ( 0.9999999999999966693, 0.9807852804032337612, 1.000000000000000000, 0.9807852804032304306, 1.000000000000000000, 0.9807852804032304306, 1.000000000000000000, 0.9807852804032304306, 1.000000000000000000, 0.9807852804032304306, 1.000000000000000000, 0.9807852804032304306, 1.000000000000000000, 0.9807852804032304306, 1.000000000000000000, 0.9807852804032270999, 1.000000000000003331 ) ) 
 REPRESENTATION_ITEM ( '' )  );
#16097=CARTESIAN_POINT ( 'NONE',  ( -25.35362745456397349, 221.0573905683720284, -16.75240474999999307 ) ) ;
#16098=CARTESIAN_POINT ( 'NONE',  ( -32.01814843081344009, 313.1823905683720000, -16.75240474999999307 ) ) ;
#16103=CARTESIAN_POINT ( 'NONE',  ( -35.09675569278793716, 303.4948905683720568, -15.47720386886985544 ) ) ;
#16105=CARTESIAN_POINT ( 'NONE',  ( -44.16309181155856578, 374.4948905683720000, 6.410867750099241924 ) ) ;
#16106=CARTESIAN_POINT ( 'NONE',  ( -13.20868407381888154, 530.9948905683720568, -6.410867750099233042 ) ) ;
#16107=CARTESIAN_POINT ( 'NONE',  ( -21.03221929538690915, 370.3698905601784759, 18.47759065022572500 ) ) ;
#16110=CARTESIAN_POINT ( 'NONE',  ( -32.01814843081346140, 483.1823905683720000, -16.75240474999999307 ) ) ;
#16112=CARTESIAN_POINT ( 'NONE',  ( -11.93348319268871371, 289.1823905683720000, -3.332260488124732856 ) ) ;
#16115=CARTESIAN_POINT ( 'NONE',  ( -11.93348319268871194, 290.6823905683720568, -3.332260488124732856 ) ) ;
#16116=CARTESIAN_POINT ( 'NONE',  ( -28.68588794268870856, 326.3698905683720000, 16.75240474999999307 ) ) ;
#16117=CARTESIAN_POINT ( 'NONE',  ( -14.48388495494898542, 259.4323905683720568, 9.489475012073731008 ) ) ;
#16118=CARTESIAN_POINT ( 'NONE',  ( -47.16347859291443001, 261.3698905765656377, -7.653668647301793193 ) ) ;
#16119=DIRECTION ( 'NONE',  ( -1.191790137725560488E-16, 1.000000000000000000, -0.000000000000000000 ) ) ;
#16121=CARTESIAN_POINT ( 'NONE',  ( -40.53162694259543741, 374.1198905683720000, -11.84573899990672707 ) ) ;
#16127=CARTESIAN_POINT ( 'NONE',  ( -16.84014894278200103, 450.1198905683720568, -11.84573899990672707 ) ) ;
#16130=CARTESIAN_POINT ( 'NONE',  ( -11.73070664223725856, 433.1823905601785327, -11.32908994701042715 ) ) ;
#16131=VERTEX_POINT ( 'NONE', #3300 ) ;
#16135=CARTESIAN_POINT ( 'NONE',  ( -48.68588794268870146, 326.9323905601784759, -3.978247347593158345 ) ) ;
#16137=CARTESIAN_POINT ( 'NONE',  ( -16.84014894278199037, 351.6198905683720000, -11.84573899990672707 ) ) ;
#16140=CARTESIAN_POINT ( 'NONE',  ( -36.33955658999053639, 503.8698905765656377, 18.47759065022572500 ) ) ;
#16141=CARTESIAN_POINT ( 'NONE',  ( -35.09675569278795138, 391.9948905683720568, -15.47720386886985544 ) ) ;
#16142=CARTESIAN_POINT ( 'NONE',  ( -38.17536295476244135, 223.8073905683720284, -14.20200298773971426 ) ) ;
#16143=CARTESIAN_POINT ( 'NONE',  ( -44.16309181155856578, 384.4948905683720000, 6.410867750099241924 ) ) ;
#16145=CARTESIAN_POINT ( 'NONE',  ( -48.68588794268870856, 331.9948905765656377, 0.000000000000000000 ) ) ;
#16146=CARTESIAN_POINT ( 'NONE',  ( -8.685887942688641061, 422.5573905601784759, -3.978247347592952732 ) ) ;
#16147=CARTESIAN_POINT ( 'NONE',  ( -14.48388495494898720, 277.9323905683720568, 9.489475012073731008 ) ) ;
#16148=CARTESIAN_POINT ( 'NONE',  ( -38.17536295476245556, 446.9323905683720000, 14.20200298773971781 ) ) ;
#16149=CARTESIAN_POINT ( 'NONE',  ( -8.685887942688536256, 282.5573905601784190, -3.978247347592740013 ) ) ;
#16150=CARTESIAN_POINT ( 'NONE',  ( -36.33955658999051508, 369.1198905601785327, 18.47759065022572500 ) ) ;
#16151=DIRECTION ( 'NONE',  ( -1.191790137725560488E-16, 1.000000000000000000, -0.000000000000000000 ) ) ;
#16154=CARTESIAN_POINT ( 'NONE',  ( -42.88789093042843348, 346.3073905683720568, 9.489475012073736337 ) ) ;
#16155=CARTESIAN_POINT ( 'NONE',  ( -44.16309181155858710, 493.2448905683720000, -6.410867750099231266 ) ) ;
#16156=CARTESIAN_POINT ( 'NONE',  ( -28.68588794268873343, 504.7448905601785896, -19.99999999999999289 ) ) ;
#16157=CARTESIAN_POINT ( 'NONE',  ( -11.93348319268871549, 318.8698905683720000, -2.051577885510841163E-15 ) ) ;
#16160=CARTESIAN_POINT ( 'NONE',  ( -8.685887942688422569, 522.5573905601784190, -3.978247347592394068 ) ) ;
#16163=EDGE_CURVE ( 'NONE', #11848, #9040, #14880, .T. ) ;
#16165=CARTESIAN_POINT ( 'NONE',  ( -28.68588794268871922, 427.8698905683720568, 16.75240474999999307 ) ) ;
#16166=DIRECTION ( 'NONE',  ( -1.000000000000000000, -0.000000000000000000, -0.000000000000000000 ) ) ;
#16168=CARTESIAN_POINT ( 'NONE',  ( -38.17536295476245556, 445.4323905683720568, 14.20200298773971781 ) ) ;
#16170=CARTESIAN_POINT ( 'NONE',  ( -35.09675569278796559, 455.7448905683720568, 15.47720386886985366 ) ) ;
#16172=CARTESIAN_POINT ( 'NONE',  ( -36.33955658999050797, 380.1198905765656377, -18.47759065022572855 ) ) ;
#16173=DIRECTION ( 'NONE',  ( -1.191790137725560488E-16, 1.000000000000000000, -0.000000000000000000 ) ) ;
#16175=CARTESIAN_POINT ( 'NONE',  ( -11.73070664223725856, 427.9323905765656377, -11.32908994701042538 ) ) ;
#16176=CARTESIAN_POINT ( 'NONE',  ( -28.68588794268869790, 254.4948905765656093, 19.99999999999999289 ) ) ;
#16177=CARTESIAN_POINT ( 'NONE',  ( -14.48388495494901740, 519.4323905683720568, 9.489475012073732785 ) ) ;
#16180=CARTESIAN_POINT ( 'NONE',  ( -8.685887942688720997, 342.2448905601784759, -2.449293598294705724E-15 ) ) ;
#16182=CARTESIAN_POINT ( 'NONE',  ( -44.16309181155857999, 434.7448905683720000, -6.410867750099231266 ) ) ;
#16183=CARTESIAN_POINT ( 'NONE',  ( -10.20829729246297646, 266.3698905765656377, 7.653668647301790529 ) ) ;
#16184=CARTESIAN_POINT ( 'NONE',  ( -35.09675569278793006, 253.4948905683720568, -15.47720386886985544 ) ) ;
#16189=CARTESIAN_POINT ( 'NONE',  ( -25.35362745456400546, 472.5573905683720568, -16.75240474999999307 ) ) ;
#16190=CARTESIAN_POINT ( 'NONE',  ( -21.03221929538690560, 218.8698905765656377, -18.47759065022572855 ) ) ;
#16191=ORIENTED_EDGE ( 'NONE', *, *, #9621, .T. ) ;
#16193=CARTESIAN_POINT ( 'NONE',  ( -11.93348319268874214, 530.6823905683721705, -3.332260488124732856 ) ) ;
#16194=ORIENTED_EDGE ( 'NONE', *, *, #20462, .T. ) ;
#16195=CARTESIAN_POINT ( 'NONE',  ( -32.01814843081346140, 526.0573905683720568, 16.75240474999999307 ) ) ;
#16197=ADVANCED_FACE ( 'NONE', ( #6632 ), #19729, .T. ) ;
#16198=CARTESIAN_POINT ( 'NONE',  ( -45.64106924314019409, 441.0573905765656377, -11.32908994701042715 ) ) ;
#16200=CARTESIAN_POINT ( 'NONE',  ( -25.35362745456399125, 351.0573905683720000, -16.75240474999999307 ) ) ;
#16202=CARTESIAN_POINT ( 'NONE',  ( -8.685887942688742314, 573.2448905601785327, 2.449293598294706119E-15 ) ) ;
#16203=CARTESIAN_POINT ( 'NONE',  ( -48.68588794268872277, 507.2448905601785327, 0.000000000000000000 ) ) ;
#16204=AXIS2_PLACEMENT_3D ( 'NONE', #18111, #6324, #3307 ) ;
#16206=CARTESIAN_POINT ( 'NONE',  ( -28.68588794268869435, 226.3698905683720284, 16.75240474999999307 ) ) ;
#16207=CARTESIAN_POINT ( 'NONE',  ( -44.16309181155856578, 314.7448905683720000, -6.410867750099231266 ) ) ;
#16209=CARTESIAN_POINT ( 'NONE',  ( -24.70764059509556887, 444.4323905601784759, -19.99999999999999289 ) ) ;
#16211=CARTESIAN_POINT ( 'NONE',  ( -42.88789093042842637, 306.3073905683719431, 9.489475012073736337 ) ) ;
#16212=CARTESIAN_POINT ( 'NONE',  ( -40.53162694259543741, 372.6198905683720000, -11.84573899990672707 ) ) ;
#16213=CARTESIAN_POINT ( 'NONE',  ( -28.68588794268872988, 517.8698905683720568, 16.75240474999999307 ) ) ;
#16214=CARTESIAN_POINT ( 'NONE',  ( -10.20829729246298712, 371.6198905601784759, 7.653668647301790529 ) ) ;
#16216=CARTESIAN_POINT ( 'NONE',  ( -17.35679799567829917, 403.8073905601785327, -16.95518130045146421 ) ) ;
#16218=CARTESIAN_POINT ( 'NONE',  ( -14.48388495494901385, 481.3073905683720000, -9.489475012073736337 ) ) ;
#16220=CARTESIAN_POINT ( 'NONE',  ( -19.19641293061497578, 280.4323905683720568, -14.20200298773971603 ) ) ;
#16222=( BOUNDED_CURVE ( )  B_SPLINE_CURVE ( 2, ( #3165, #2076, #18710, #20453, #2393, #12338, #565, #7133, #10697, #10275, #10592, #20138, #12121, #16895, #8974, #784, #5305 ),
 .UNSPECIFIED., .F., .T. ) 
 B_SPLINE_CURVE_WITH_KNOTS ( ( 3, 2, 2, 2, 2, 2, 2, 2, 3 ),
 ( 0.5625000000000001110, 0.5644531250000001110, 0.5664062500000001110, 0.5683593750000001110, 0.5703125000000001110, 0.5722656250000001110, 0.5742187500000001110, 0.5761718750000001110, 0.5781250000000001110 ),
 .UNSPECIFIED. ) 
 CURVE ( )  GEOMETRIC_REPRESENTATION_ITEM ( )  RATIONAL_B_SPLINE_CURVE ( ( 0.9999999999999988898, 0.9807852804032315408, 1.000000000000000000, 0.9807852804032304306, 1.000000000000000000, 0.9807852804032304306, 1.000000000000000000, 0.9807852804032304306, 1.000000000000000000, 0.9807852804032304306, 1.000000000000000000, 0.9807852804032304306, 1.000000000000000000, 0.9807852804032304306, 1.000000000000000000, 0.9807852804032293204, 1.000000000000001110 ) ) 
 REPRESENTATION_ITEM ( '' )  );
#16223=CARTESIAN_POINT ( 'NONE',  ( -11.93348319268871194, 290.0573905683720000, 3.332260488124728859 ) ) ;
#16224=CARTESIAN_POINT ( 'NONE',  ( -42.88789093042842637, 314.8073905683721136, 9.489475012073736337 ) ) ;
#16225=CARTESIAN_POINT ( 'NONE',  ( -40.53162694259542320, 266.6198905683720568, 11.84573899990672885 ) ) ;
#16226=CARTESIAN_POINT ( 'NONE',  ( -8.685887942688710339, 257.3073905765656377, -3.978247347593165895 ) ) ;
#16228=CARTESIAN_POINT ( 'NONE',  ( -42.88789093042841927, 232.9323905683720000, -9.489475012073734561 ) ) ;
#16229=CARTESIAN_POINT ( 'NONE',  ( -22.27502019258948707, 372.2448905683720000, -15.47720386886985544 ) ) ;
#16236=CARTESIAN_POINT ( 'NONE',  ( -44.16309181155857289, 414.4948905683720000, 6.410867750099241924 ) ) ;
#16237=CARTESIAN_POINT ( 'NONE',  ( -48.68588794268873698, 573.2448905601785327, 0.000000000000000000 ) ) ;
#16238=ORIENTED_EDGE ( 'NONE', *, *, #21255, .T. ) ;
#16239=CARTESIAN_POINT ( 'NONE',  ( -47.16347859291445133, 417.8698905601784759, 7.653668647301805628 ) ) ;
#16244=CARTESIAN_POINT ( 'NONE',  ( -21.03221929538690205, 310.3698905601784759, 18.47759065022572500 ) ) ;
#16246=CARTESIAN_POINT ( 'NONE',  ( -16.84014894278198327, 339.1198905683720568, 11.84573899990672530 ) ) ;
#16247=CARTESIAN_POINT ( 'NONE',  ( -42.82802356641968089, 510.7448905765656946, -14.14213562373094746 ) ) ;
#16248=CARTESIAN_POINT ( 'NONE',  ( -45.43829269268871229, 383.8698905683720000, 0.000000000000000000 ) ) ;
#16250=CARTESIAN_POINT ( 'NONE',  ( -28.68588794268871922, 391.3698905683720000, -16.75240474999999307 ) ) ;
#16251=CARTESIAN_POINT ( 'NONE',  ( -24.70764059509554755, 314.8073905765655809, 19.99999999999998934 ) ) ;
#16252=CARTESIAN_POINT ( 'NONE',  ( -14.54375231895777709, 423.4948905601784759, -14.14213562373094746 ) ) ;
#16253=CARTESIAN_POINT ( 'NONE',  ( -25.35362745456397349, 286.6823905683720000, 16.75240474999998952 ) ) ;
#16257=CARTESIAN_POINT ( 'NONE',  ( -40.53162694259544452, 436.6198905683720000, 11.84573899990672885 ) ) ;
#16262=CARTESIAN_POINT ( 'NONE',  ( -45.43829269268870519, 355.6823905683720000, 3.332260488124734632 ) ) ;
#16263=CARTESIAN_POINT ( 'NONE',  ( -13.20868407381887799, 499.4948905683720568, -6.410867750099233042 ) ) ;
#16264=CARTESIAN_POINT ( 'NONE',  ( -36.33955658999052929, 479.1198905601785327, 18.47759065022572500 ) ) ;
#16265=CARTESIAN_POINT ( 'NONE',  ( -28.68588794268871212, 321.3698905683720568, -16.75240474999999307 ) ) ;
#16266=EDGE_LOOP ( 'NONE', ( #12453, #9935, #3207, #15633, #14011 ) ) ;
#16267=AXIS2_PLACEMENT_3D ( 'NONE', #4151, #20497, #1036 ) ;
#16269=CARTESIAN_POINT ( 'NONE',  ( -28.68588794268873698, 524.7448905601785327, -19.99999999999999289 ) ) ;
#16273=CARTESIAN_POINT ( 'NONE',  ( -35.09675569278795138, 403.4948905683720000, -15.47720386886985544 ) ) ;
#16275=CARTESIAN_POINT ( 'NONE',  ( -45.43829269268871229, 443.5573905683720000, -3.332260488124726194 ) ) ;
#16276=VECTOR ( 'NONE', #2787, 1000.000000000000000 ) ;
#16277=CARTESIAN_POINT ( 'NONE',  ( -16.84014894278199748, 447.6198905683720568, 11.84573899990672530 ) ) ;
#16280=CARTESIAN_POINT ( 'NONE',  ( -25.35362745456400546, 482.5573905683720000, -16.75240474999999307 ) ) ;
#16281=CARTESIAN_POINT ( 'NONE',  ( -42.82802356641966668, 390.7448905765656377, -14.14213562373094746 ) ) ;
#16284=CARTESIAN_POINT ( 'NONE',  ( -21.03221929538693047, 428.8698905765655809, -18.47759065022572855 ) ) ;
#16285=FACE_OUTER_BOUND ( 'NONE', #10877, .T. ) ;
#16286=CARTESIAN_POINT ( 'NONE',  ( -45.43829269268871940, 495.0573905683719431, -3.332260488124726194 ) ) ;
#16290=CARTESIAN_POINT ( 'NONE',  ( -40.01497788969912506, 255.6823905601785043, -16.95518130045146421 ) ) ;
#16293=CARTESIAN_POINT ( 'NONE',  ( -42.88789093042844058, 406.3073905683719431, 9.489475012073736337 ) ) ;
#16294=CARTESIAN_POINT ( 'NONE',  ( -21.03221929538692692, 384.1198905601784759, -18.47759065022572855 ) ) ;
#16295=CARTESIAN_POINT ( 'NONE',  ( -11.93348319268870483, 230.3698905683720284, -2.051577885510841163E-15 ) ) ;
#16296=ORIENTED_EDGE ( 'NONE', *, *, #923, .F. ) ;
#16299=CARTESIAN_POINT ( 'NONE',  ( -32.01814843081345430, 457.5573905683719431, 16.75240474999999307 ) ) ;
#16300=CARTESIAN_POINT ( 'NONE',  ( -45.64106924314017277, 232.9323905765656093, 11.32908994701042715 ) ) ;
#16303=CARTESIAN_POINT ( 'NONE',  ( -36.33955658999053639, 523.8698905765655809, 18.47759065022572500 ) ) ;
#16304=CARTESIAN_POINT ( 'NONE',  ( -44.16309181155855867, 223.2448905683720568, -6.410867750099231266 ) ) ;
#16305=ORIENTED_EDGE ( 'NONE', *, *, #8300, .F. ) ;
#16306=CARTESIAN_POINT ( 'NONE',  ( -38.17536295476247687, 512.3073905683720568, -14.20200298773971426 ) ) ;
#16309=CARTESIAN_POINT ( 'NONE',  ( -14.54375231895777709, 445.7448905765656377, 14.14213562373094568 ) ) ;
#16311=CARTESIAN_POINT ( 'NONE',  ( -11.93348319268872260, 349.1823905683720000, -3.332260488124732856 ) ) ;
#16312=CARTESIAN_POINT ( 'NONE',  ( -48.68588794268872277, 451.9948905765656377, 0.000000000000000000 ) ) ;
#16314=CARTESIAN_POINT ( 'NONE',  ( -47.16347859291443712, 287.8698905601784759, 7.653668647301805628 ) ) ;
#16315=CARTESIAN_POINT ( 'NONE',  ( -22.27502019258946930, 220.7448905683720568, -15.47720386886985544 ) ) ;
#16316=CARTESIAN_POINT ( 'NONE',  ( -28.68588794268870856, 317.8698905683720000, 16.75240474999999307 ) ) ;
#16318=CARTESIAN_POINT ( 'NONE',  ( -32.66413529028186247, 265.0573905601784759, -19.99999999999999289 ) ) ;
#16319=CARTESIAN_POINT ( 'NONE',  ( -48.68588794268887199, 377.5573905601785327, 3.978247347592742678 ) ) ;
#16320=CARTESIAN_POINT ( 'NONE',  ( -25.35362745456398414, 312.5573905683720000, -16.75240474999999307 ) ) ;
#16322=CARTESIAN_POINT ( 'NONE',  ( -22.27502019258950483, 532.2448905683720568, -15.47720386886985544 ) ) ;
#16323=CARTESIAN_POINT ( 'NONE',  ( -28.68588794268871567, 364.7448905601784759, -19.99999999999999289 ) ) ;
#16324=CARTESIAN_POINT ( 'NONE',  ( -17.35679799567828852, 313.8073905601784190, -16.95518130045146421 ) ) ;
#16325=VERTEX_POINT ( 'NONE', #2009 ) ;
#16326=CARTESIAN_POINT ( 'NONE',  ( -22.27502019258949062, 478.4948905683720000, 15.47720386886985189 ) ) ;
#16327=CYLINDRICAL_SURFACE ( 'NONE', #10069, 19.99999999999999645 ) ;
#16328=CARTESIAN_POINT ( 'NONE',  ( -45.43829269268869808, 283.5573905683720568, -3.332260488124726194 ) ) ;
#16331=CARTESIAN_POINT ( 'NONE',  ( -32.01814843081344009, 277.5573905683720568, 16.75240474999999307 ) ) ;
#16332=CARTESIAN_POINT ( 'NONE',  ( -38.17536295476244845, 312.3073905683720000, -14.20200298773971426 ) ) ;
#16333=CARTESIAN_POINT ( 'NONE',  ( -19.19641293061496512, 258.8073905683720568, 14.20200298773971426 ) ) ;
#16335=CARTESIAN_POINT ( 'NONE',  ( -32.66413529028186247, 254.1823905765655809, 19.99999999999999289 ) ) ;
#16336=CARTESIAN_POINT ( 'NONE',  ( -17.35679799567830983, 473.8073905601784759, -16.95518130045146421 ) ) ;
#16337=CARTESIAN_POINT ( 'NONE',  ( -40.53162694259542320, 232.6198905683720000, -11.84573899990672707 ) ) ;
#16338=CARTESIAN_POINT ( 'NONE',  ( -25.35362745456399480, 382.5573905683720568, -16.75240474999999307 ) ) ;
#16342=CARTESIAN_POINT ( 'NONE',  ( -8.685887942688742314, 573.2448905601785327, 2.449293598294706119E-15 ) ) ;
#16343=CARTESIAN_POINT ( 'NONE',  ( -22.27502019258949417, 430.7448905683720000, -15.47720386886985544 ) ) ;
#16346=( BOUNDED_CURVE ( )  B_SPLINE_CURVE ( 2, ( #12377, #14120, #10526, #712, #15852, #8910, #13907, #17253, #7284, #10635, #12275, #9017, #7600, #4266, #9122, #825, #7173 ),
 .UNSPECIFIED., .F., .T. ) 
 B_SPLINE_CURVE_WITH_KNOTS ( ( 3, 2, 2, 2, 2, 2, 2, 2, 3 ),
 ( 0.03125000000000002776, 0.03320312500000007633, 0.03515625000000012490, 0.03710937500000016653, 0.03906250000000021511, 0.04101562500000026368, 0.04296875000000030531, 0.04492187500000035388, 0.04687500000000040246 ),
 .UNSPECIFIED. ) 
 CURVE ( )  GEOMETRIC_REPRESENTATION_ITEM ( )  RATIONAL_B_SPLINE_CURVE ( ( 0.9999999999999997780, 0.9807852804032306526, 1.000000000000000000, 0.9807852804032304306, 1.000000000000000000, 0.9807852804032304306, 1.000000000000000000, 0.9807852804032304306, 1.000000000000000000, 0.9807852804032304306, 1.000000000000000000, 0.9807852804032304306, 1.000000000000000000, 0.9807852804032304306, 1.000000000000000000, 0.9807852804032264338, 1.000000000000003997 ) ) 
 REPRESENTATION_ITEM ( '' )  );
#16347=CARTESIAN_POINT ( 'NONE',  ( -24.70764059509556887, 424.4323905601784759, -19.99999999999999289 ) ) ;
#16351=CARTESIAN_POINT ( 'NONE',  ( -42.82802356641965957, 353.2448905765656377, 14.14213562373094923 ) ) ;
#16352=CARTESIAN_POINT ( 'NONE',  ( -32.66413529028186957, 299.4323905601784759, 19.99999999999999289 ) ) ;
#16354=CARTESIAN_POINT ( 'NONE',  ( -32.01814843081344719, 337.5573905683720568, 16.75240474999999307 ) ) ;
#16355=CARTESIAN_POINT ( 'NONE',  ( -10.20829729246300310, 506.3698905765656946, 7.653668647301790529 ) ) ;
#16356=CARTESIAN_POINT ( 'NONE',  ( -44.16309181155856578, 384.4948905683720000, 6.410867750099241924 ) ) ;
#16357=CARTESIAN_POINT ( 'NONE',  ( -35.09675569278795848, 395.7448905683720568, 15.47720386886985366 ) ) ;
#16358=CARTESIAN_POINT ( 'NONE',  ( -42.82802356641965247, 320.7448905765656377, -14.14213562373094746 ) ) ;
#16359=CARTESIAN_POINT ( 'NONE',  ( -48.68588794268862330, 426.9323905601784759, -3.978247347593371508 ) ) ;
#16360=CARTESIAN_POINT ( 'NONE',  ( -13.20868407381884957, 288.2448905683720000, 6.410867750099229490 ) ) ;
#16362=CARTESIAN_POINT ( 'NONE',  ( -32.01814843081345430, 433.1823905683721136, -16.75240474999999307 ) ) ;
#16367=EDGE_CURVE ( 'NONE', #14199, #15635, #6401, .T. ) ;
#16369=CARTESIAN_POINT ( 'NONE',  ( -28.68588794268871212, 357.8698905683720568, 16.75240474999999307 ) ) ;
#16370=CARTESIAN_POINT ( 'NONE',  ( -19.19641293061499354, 487.3073905683719431, 14.20200298773971426 ) ) ;
#16374=CARTESIAN_POINT ( 'NONE',  ( -24.70764059509556532, 490.0573905601784759, 19.99999999999998934 ) ) ;
#16375=CARTESIAN_POINT ( 'NONE',  ( -11.93348319268871727, 309.1823905683719431, -3.332260488124732856 ) ) ;
#16379=VERTEX_POINT ( 'NONE', #5543 ) ;
#16381=CARTESIAN_POINT ( 'NONE',  ( -45.43829269268871940, 405.6823905683720568, 3.332260488124734632 ) ) ;
#16382=CARTESIAN_POINT ( 'NONE',  ( -10.20829729246299600, 446.3698905765656377, 7.653668647301790529 ) ) ;
#16384=CARTESIAN_POINT ( 'NONE',  ( -35.09675569278795138, 441.9948905683720568, -15.47720386886985544 ) ) ;
#16385=CARTESIAN_POINT ( 'NONE',  ( -40.53162694259544452, 442.6198905683720568, -11.84573899990672707 ) ) ;
#16386=CARTESIAN_POINT ( 'NONE',  ( -47.16347859291445133, 416.6198905601785327, -7.653668647301793193 ) ) ;
#16388=CARTESIAN_POINT ( 'NONE',  ( -8.685887942688726326, 386.9948905765655809, -2.449293598294705724E-15 ) ) ;
#16390=CARTESIAN_POINT ( 'NONE',  ( -36.33955658999049376, 265.3698905601784759, -18.47759065022572855 ) ) ;
#16394=CARTESIAN_POINT ( 'NONE',  ( -19.19641293061499709, 498.8073905683720000, 14.20200298773971426 ) ) ;
#16396=CARTESIAN_POINT ( 'NONE',  ( -32.66413529028188378, 465.0573905601784190, -19.99999999999999289 ) ) ;
#16397=CARTESIAN_POINT ( 'NONE',  ( -48.68588794268878672, 517.5573905601784190, 3.978247347593061978 ) ) ;
#16398=CARTESIAN_POINT ( 'NONE',  ( -25.35362745456398770, 408.1823905683720568, 16.75240474999998952 ) ) ;
#16399=CARTESIAN_POINT ( 'NONE',  ( -8.685887942688735208, 466.9948905765656377, -2.449293598294705724E-15 ) ) ;
#16400=CARTESIAN_POINT ( 'NONE',  ( -16.84014894278197261, 239.1198905683720284, 11.84573899990672530 ) ) ;
#16402=CARTESIAN_POINT ( 'NONE',  ( -11.73070664223725501, 426.0573905765655809, 11.32908994701042005 ) ) ;
#16404=CARTESIAN_POINT ( 'NONE',  ( -22.27502019258948707, 438.4948905683720568, 15.47720386886985189 ) ) ;
#16405=CARTESIAN_POINT ( 'NONE',  ( -48.68588794268869435, 222.3073905765656093, 3.978247347593168115 ) ) ;
#16406=ORIENTED_EDGE ( 'NONE', *, *, #14403, .F. ) ;
#16408=CARTESIAN_POINT ( 'NONE',  ( -22.27502019258945865, 226.9948905683720284, 15.47720386886985189 ) ) ;
#16410=CARTESIAN_POINT ( 'NONE',  ( -44.16309181155858710, 503.2448905683719431, -6.410867750099231266 ) ) ;
#16412=CARTESIAN_POINT ( 'NONE',  ( -21.03221929538691981, 445.1198905765655809, 18.47759065022572500 ) ) ;
#16414=CARTESIAN_POINT ( 'NONE',  ( -42.82802356641965247, 328.4948905601784759, 14.14213562373094923 ) ) ;
#16416=CARTESIAN_POINT ( 'NONE',  ( -40.01497788969912506, 240.4323905765656662, -16.95518130045146421 ) ) ;
#16417=CYLINDRICAL_SURFACE ( 'NONE', #11186, 19.99999999999999645 ) ;
#16419=CARTESIAN_POINT ( 'NONE',  ( -43.04611869048239470, 202.6362012587621280, -4.338193544061892837 ) ) ;
#16420=CARTESIAN_POINT ( 'NONE',  ( -14.48388495494899075, 309.4323905683720568, 9.489475012073732785 ) ) ;
#16421=CARTESIAN_POINT ( 'NONE',  ( -11.73070664223726034, 443.1823905601784759, -11.32908994701042538 ) ) ;
#16422=CARTESIAN_POINT ( 'NONE',  ( -36.33955658999049376, 265.3698905601784759, -18.47759065022572855 ) ) ;
#16424=CARTESIAN_POINT ( 'NONE',  ( -35.09675569278793716, 293.4948905683720000, -15.47720386886985544 ) ) ;
#16426=CARTESIAN_POINT ( 'NONE',  ( -11.93348319268874036, 520.6823905683719431, -3.332260488124732856 ) ) ;
#16427=CARTESIAN_POINT ( 'NONE',  ( -48.68588794268870856, 357.2448905601784759, 0.000000000000000000 ) ) ;
#16430=CARTESIAN_POINT ( 'NONE',  ( -16.84014894278200458, 481.6198905683720000, -11.84573899990672707 ) ) ;
#16433=CARTESIAN_POINT ( 'NONE',  ( -11.93348319268871194, 278.5573905683720000, 3.332260488124728415 ) ) ;
#16434=VERTEX_POINT ( 'NONE', #5653 ) ;
#16435=CARTESIAN_POINT ( 'NONE',  ( -38.17536295476244845, 283.8073905683720568, -14.20200298773971426 ) ) ;
#16436=CARTESIAN_POINT ( 'NONE',  ( -45.43829269268869808, 255.3698905683720000, 0.000000000000000000 ) ) ;
#16437=CARTESIAN_POINT ( 'NONE',  ( -21.03221929538690915, 238.8698905765656093, -18.47759065022572855 ) ) ;
#16440=CARTESIAN_POINT ( 'NONE',  ( -11.93348319268870661, 229.1823905683720568, -3.332260488124732856 ) ) ;
#16441=CARTESIAN_POINT ( 'NONE',  ( -14.48388495494898898, 269.8073905683720000, -9.489475012073736337 ) ) ;
#16442=CARTESIAN_POINT ( 'NONE',  ( -44.16309181155857289, 384.7448905683720000, -6.410867750099231266 ) ) ;
#16445=CARTESIAN_POINT ( 'NONE',  ( -48.68588794268870146, 271.9948905765656377, 0.000000000000000000 ) ) ;
#16446=EDGE_CURVE ( 'NONE', #9649, #3515, #5463, .T. ) ;
#16447=CARTESIAN_POINT ( 'NONE',  ( -38.17536295476245556, 415.4323905683720568, 14.20200298773971781 ) ) ;
#16450=CARTESIAN_POINT ( 'NONE',  ( -10.20829729246299244, 422.8698905601784759, -7.653668647301794969 ) ) ;
#16451=ORIENTED_EDGE ( 'NONE', *, *, #17469, .T. ) ;
#16455=CARTESIAN_POINT ( 'NONE',  ( -8.685887942688985675, 356.6823905765654672, 3.978247347593800054 ) ) ;
#16456=CARTESIAN_POINT ( 'NONE',  ( -17.35679799567829207, 303.8073905601784759, -16.95518130045146421 ) ) ;
#16458=CARTESIAN_POINT ( 'NONE',  ( -44.16309181155857289, 334.7448905683720568, -6.410867750099231266 ) ) ;
#16459=CARTESIAN_POINT ( 'NONE',  ( -42.82802356641967378, 493.2448905765656377, 14.14213562373094923 ) ) ;
#16460=CARTESIAN_POINT ( 'NONE',  ( -25.35362745456399125, 371.0573905683720000, -16.75240474999999307 ) ) ;
#16462=CARTESIAN_POINT ( 'NONE',  ( -11.93348319268872260, 378.8698905683720000, -2.051577885510841163E-15 ) ) ;
#16464=CARTESIAN_POINT ( 'NONE',  ( -47.16347859291443712, 302.6198905765656377, 7.653668647301805628 ) ) ;
#16466=CARTESIAN_POINT ( 'NONE',  ( -19.19641293061497223, 280.4323905683720568, -14.20200298773971603 ) ) ;
#16467=CYLINDRICAL_SURFACE ( 'NONE', #14298, 19.99999999999999645 ) ;
#16468=CARTESIAN_POINT ( 'NONE',  ( -35.09675569278795848, 437.2448905683720000, 15.47720386886985366 ) ) ;
#16472=CARTESIAN_POINT ( 'NONE',  ( -48.68588794268872277, 481.9948905765656377, 0.000000000000000000 ) ) ;
#16473=( BOUNDED_CURVE ( )  B_SPLINE_CURVE ( 2, ( #12776, #16455, #12887, #19369, #21309, #8098, #1746, #8210, #2937, #4657, #9624, #11461, #16351, #9941, #9517, #19793, #3147 ),
 .UNSPECIFIED., .F., .T. ) 
 B_SPLINE_CURVE_WITH_KNOTS ( ( 3, 2, 2, 2, 2, 2, 2, 2, 3 ),
 ( 0.5468750000000003331, 0.5488281250000003331, 0.5507812500000002220, 0.5527343750000002220, 0.5546875000000002220, 0.5566406250000002220, 0.5585937500000002220, 0.5605468750000001110, 0.5625000000000001110 ),
 .UNSPECIFIED. ) 
 CURVE ( )  GEOMETRIC_REPRESENTATION_ITEM ( )  RATIONAL_B_SPLINE_CURVE ( ( 0.9999999999999966693, 0.9807852804032337612, 1.000000000000000000, 0.9807852804032304306, 1.000000000000000000, 0.9807852804032304306, 1.000000000000000000, 0.9807852804032304306, 1.000000000000000000, 0.9807852804032304306, 1.000000000000000000, 0.9807852804032304306, 1.000000000000000000, 0.9807852804032304306, 1.000000000000000000, 0.9807852804032293204, 1.000000000000001110 ) ) 
 REPRESENTATION_ITEM ( '' )  );
#16475=EDGE_CURVE ( 'NONE', #15642, #7137, #11396, .T. ) ;
#16476=CARTESIAN_POINT ( 'NONE',  ( -40.53162694259543741, 356.6198905683720000, 11.84573899990672885 ) ) ;
#16477=CARTESIAN_POINT ( 'NONE',  ( -16.84014894278200458, 480.1198905683720000, -11.84573899990672707 ) ) ;
#16479=CARTESIAN_POINT ( 'NONE',  ( -48.68588794268872277, 486.9323905601785327, -3.978247347593158345 ) ) ;
#16480=CARTESIAN_POINT ( 'NONE',  ( -45.43829269268869808, 294.1823905683720000, 3.332260488124734632 ) ) ;
#16483=CARTESIAN_POINT ( 'NONE',  ( -10.20829729246298356, 346.3698905765655809, 7.653668647301790529 ) ) ;
#16484=ORIENTED_EDGE ( 'NONE', *, *, #12363, .F. ) ;
#16486=AXIS2_PLACEMENT_3D ( 'NONE', #20509, #10433, #17055 ) ;
#16487=CARTESIAN_POINT ( 'NONE',  ( -22.27502019258948351, 408.4948905683720000, 15.47720386886985189 ) ) ;
#16488=CARTESIAN_POINT ( 'NONE',  ( -24.70764059509556176, 480.0573905601784759, 19.99999999999998934 ) ) ;
#16489=CARTESIAN_POINT ( 'NONE',  ( -40.53162694259544452, 425.1198905683720000, 11.84573899990672885 ) ) ;
#16490=CARTESIAN_POINT ( 'NONE',  ( -19.19641293061498999, 447.3073905683720568, 14.20200298773971426 ) ) ;
#16492=CARTESIAN_POINT ( 'NONE',  ( -14.54375231895776821, 375.7448905765656377, 14.14213562373094568 ) ) ;
#16494=CARTESIAN_POINT ( 'NONE',  ( -42.82802356641966668, 390.7448905765656377, -14.14213562373094746 ) ) ;
#16497=CARTESIAN_POINT ( 'NONE',  ( -35.09675569278795848, 503.4948905683720568, -15.47720386886985544 ) ) ;
#16501=CARTESIAN_POINT ( 'NONE',  ( -28.68588794268871922, 419.7448905601784759, 19.99999999999999289 ) ) ;
#16503=CARTESIAN_POINT ( 'NONE',  ( -45.43829269268871940, 415.3698905683720568, 0.000000000000000000 ) ) ;
#16504=CARTESIAN_POINT ( 'NONE',  ( -28.68588794268872988, 469.4948905765656377, -19.99999999999999289 ) ) ;
#16505=EDGE_CURVE ( 'NONE', #19523, #20734, #21012, .T. ) ;
#16506=CARTESIAN_POINT ( 'NONE',  ( -25.35362745456397704, 232.5573905683720568, -16.75240474999999307 ) ) ;
#16511=CARTESIAN_POINT ( 'NONE',  ( -45.43829269268871940, 435.0573905683720568, -3.332260488124726638 ) ) ;
#16512=CARTESIAN_POINT ( 'NONE',  ( -42.88789093042845479, 532.9323905683720568, -9.489475012073736337 ) ) ;
#16515=CARTESIAN_POINT ( 'NONE',  ( -42.88789093042841927, 224.8073905683720284, 9.489475012073736337 ) ) ;
#16517=CARTESIAN_POINT ( 'NONE',  ( -35.09675569278796559, 511.9948905683720000, -15.47720386886985544 ) ) ;
#16519=CARTESIAN_POINT ( 'NONE',  ( -21.03221929538691981, 435.1198905765656377, 18.47759065022572500 ) ) ;
#16520=CARTESIAN_POINT ( 'NONE',  ( -14.54375231895776999, 358.2448905765656377, -14.14213562373094746 ) ) ;
#16521=CARTESIAN_POINT ( 'NONE',  ( -36.33955658999049376, 250.1198905765656377, -18.47759065022572855 ) ) ;
#16526=CARTESIAN_POINT ( 'NONE',  ( -48.68588794268872277, 477.2448905601784759, 0.000000000000000000 ) ) ;
#16527=CARTESIAN_POINT ( 'NONE',  ( -44.16309181155856578, 304.7448905683720568, -6.410867750099231266 ) ) ;
#16529=CARTESIAN_POINT ( 'NONE',  ( -21.03221929538689849, 260.3698905601785327, 18.47759065022572500 ) ) ;
#16530=CARTESIAN_POINT ( 'NONE',  ( -14.54375231895777354, 415.7448905765655809, 14.14213562373094568 ) ) ;
#16531=CARTESIAN_POINT ( 'NONE',  ( -38.17536295476246977, 503.8073905683721136, -14.20200298773971426 ) ) ;
#16532=( BOUNDED_CURVE ( )  B_SPLINE_CURVE ( 2, ( #14983, #9870, #17786, #17991, #8359, #19725, #11184, #170, #1352, #14877, #16284, #13025, #6312, #16175, #4692, #1459, #3401 ),
 .UNSPECIFIED., .F., .T. ) 
 B_SPLINE_CURVE_WITH_KNOTS ( ( 3, 2, 2, 2, 2, 2, 2, 2, 3 ),
 ( 0.3125000000000001110, 0.3144531250000001110, 0.3164062500000001110, 0.3183593750000001110, 0.3203125000000001110, 0.3222656250000001110, 0.3242187500000001110, 0.3261718750000001110, 0.3281250000000001110 ),
 .UNSPECIFIED. ) 
 CURVE ( )  GEOMETRIC_REPRESENTATION_ITEM ( )  RATIONAL_B_SPLINE_CURVE ( ( 0.9999999999999988898, 0.9807852804032315408, 1.000000000000000000, 0.9807852804032304306, 1.000000000000000000, 0.9807852804032304306, 1.000000000000000000, 0.9807852804032304306, 1.000000000000000000, 0.9807852804032304306, 1.000000000000000000, 0.9807852804032304306, 1.000000000000000000, 0.9807852804032304306, 1.000000000000000000, 0.9807852804032293204, 1.000000000000001110 ) ) 
 REPRESENTATION_ITEM ( '' )  );
#16533=CARTESIAN_POINT ( 'NONE',  ( -48.68588794268870856, 366.9323905601785327, -3.978247347593158345 ) ) ;
#16534=CARTESIAN_POINT ( 'NONE',  ( -48.68588794268873698, 573.2448905601785327, 0.000000000000000000 ) ) ;
#16536=CARTESIAN_POINT ( 'NONE',  ( -19.19641293061499709, 471.9323905683720568, -14.20200298773971603 ) ) ;
#16538=CARTESIAN_POINT ( 'NONE',  ( -19.19641293061497578, 287.3073905683720000, 14.20200298773971426 ) ) ;
#16540=DIRECTION ( 'NONE',  ( -1.191790137725560488E-16, 1.000000000000000000, -0.000000000000000000 ) ) ;
#16541=CARTESIAN_POINT ( 'NONE',  ( -45.43829269268870519, 285.6823905683720000, 3.332260488124734632 ) ) ;
#16542=CARTESIAN_POINT ( 'NONE',  ( -14.48388495494898720, 261.3073905683720568, -9.489475012073734561 ) ) ;
#16543=CARTESIAN_POINT ( 'NONE',  ( -47.16347859291443001, 242.6198905765656377, 7.653668647301805628 ) ) ;
#16544=CARTESIAN_POINT ( 'NONE',  ( -17.35679799567830273, 418.5573905765655809, -16.95518130045146421 ) ) ;
#16545=CARTESIAN_POINT ( 'NONE',  ( -48.68588794268869435, 237.2448905601785043, 0.000000000000000000 ) ) ;
#16547=CARTESIAN_POINT ( 'NONE',  ( -38.17536295476243424, 265.4323905683720568, 14.20200298773971781 ) ) ;
#16548=CARTESIAN_POINT ( 'NONE',  ( -11.93348319268872260, 370.3698905683720568, -2.051577885510841163E-15 ) ) ;
#16549=CARTESIAN_POINT ( 'NONE',  ( -28.68588794268874054, 573.2448905601785327, 0.000000000000000000 ) ) ;
#16552=CARTESIAN_POINT ( 'NONE',  ( -17.35679799567828496, 268.5573905765656377, -16.95518130045146421 ) ) ;
#16553=CARTESIAN_POINT ( 'NONE',  ( -38.17536295476246266, 432.3073905683720000, -14.20200298773971426 ) ) ;
#16554=UNCERTAINTY_MEASURE_WITH_UNIT (LENGTH_MEASURE( 1.000000000000000082E-05 ), #1343, 'distance_accuracy_value', 'NONE');
#16557=CARTESIAN_POINT ( 'NONE',  ( -8.685887942688729879, 432.2448905601785327, -2.449293598294705724E-15 ) ) ;
#16563=CARTESIAN_POINT ( 'NONE',  ( -28.68588794268870501, 309.7448905601785327, 19.99999999999999289 ) ) ;
#16565=CARTESIAN_POINT ( 'NONE',  ( -13.20868407381885667, 349.7448905683720568, 6.410867750099229490 ) ) ;
#16567=CARTESIAN_POINT ( 'NONE',  ( -8.685887942688736985, 486.9948905765656377, -2.449293598294705724E-15 ) ) ;
#16568=CARTESIAN_POINT ( 'NONE',  ( -16.84014894278199037, 370.1198905683720000, -11.84573899990672707 ) ) ;
#16569=CARTESIAN_POINT ( 'NONE',  ( -38.17536295476245556, 395.4323905683720000, 14.20200298773971781 ) ) ;
#16572=CARTESIAN_POINT ( 'NONE',  ( -8.685887942688715668, 307.3073905765655809, -3.978247347593165895 ) ) ;
#16574=CARTESIAN_POINT ( 'NONE',  ( -11.93348319268871194, 289.1823905683720000, -3.332260488124732856 ) ) ;
#16575=CARTESIAN_POINT ( 'NONE',  ( -8.685887942688729879, 442.2448905601785327, -2.449293598294705724E-15 ) ) ;
#16576=CARTESIAN_POINT ( 'NONE',  ( -22.27502019258948351, 428.4948905683720568, 15.47720386886985189 ) ) ;
#16578=CARTESIAN_POINT ( 'NONE',  ( -10.20829729246300310, 501.6198905601785327, 7.653668647301790529 ) ) ;
#16581=CARTESIAN_POINT ( 'NONE',  ( -14.48388495494899786, 351.3073905683721136, -9.489475012073736337 ) ) ;
#16582=CARTESIAN_POINT ( 'NONE',  ( -45.43829269268872650, 473.8698905683720568, 0.000000000000000000 ) ) ;
#16584=CARTESIAN_POINT ( 'NONE',  ( -8.685887942688736985, 482.5573905601784759, -3.978247347593165895 ) ) ;
#16585=CARTESIAN_POINT ( 'NONE',  ( -32.01814843081344009, 311.6823905683720568, -16.75240474999999307 ) ) ;
#16591=CARTESIAN_POINT ( 'NONE',  ( -28.68588794268871567, 397.8698905683720000, 16.75240474999999307 ) ) ;
#16592=CARTESIAN_POINT ( 'NONE',  ( -42.82802356641966668, 443.2448905765656377, 14.14213562373094923 ) ) ;
#16593=CARTESIAN_POINT ( 'NONE',  ( -28.68588794268871567, 384.4948905765656377, 19.99999999999999289 ) ) ;
#16594=CARTESIAN_POINT ( 'NONE',  ( -38.17536295476245556, 415.4323905683720568, 14.20200298773971781 ) ) ;
#16595=CARTESIAN_POINT ( 'NONE',  ( -19.19641293061497223, 268.8073905683720568, 14.20200298773971426 ) ) ;
#16596=CARTESIAN_POINT ( 'NONE',  ( -11.93348319268872970, 438.5573905683720000, 3.332260488124728859 ) ) ;
#16598=DIRECTION ( 'NONE',  ( -1.191790137725560488E-16, 1.000000000000000000, -0.000000000000000000 ) ) ;
#16600=CARTESIAN_POINT ( 'NONE',  ( -45.64106924314018698, 361.0573905765656946, -11.32908994701042715 ) ) ;
#16604=( BOUNDED_CURVE ( )  B_SPLINE_CURVE ( 2, ( #5666, #10525, #930, #17147, #10421, #18855, #15743, #14119, #2224, #15851, #10852, #5879, #10742, #13906, #5451, #2435, #12376 ),
 .UNSPECIFIED., .F., .T. ) 
 B_SPLINE_CURVE_WITH_KNOTS ( ( 3, 2, 2, 2, 2, 2, 2, 2, 3 ),
 ( 0.7500000000000001110, 0.7519531250000001110, 0.7539062500000001110, 0.7558593750000001110, 0.7578125000000001110, 0.7597656250000001110, 0.7617187500000001110, 0.7636718750000001110, 0.7656250000000001110 ),
 .UNSPECIFIED. ) 
 CURVE ( )  GEOMETRIC_REPRESENTATION_ITEM ( )  RATIONAL_B_SPLINE_CURVE ( ( 0.9999999999999988898, 0.9807852804032315408, 1.000000000000000000, 0.9807852804032304306, 1.000000000000000000, 0.9807852804032304306, 1.000000000000000000, 0.9807852804032304306, 1.000000000000000000, 0.9807852804032304306, 1.000000000000000000, 0.9807852804032304306, 1.000000000000000000, 0.9807852804032304306, 1.000000000000000000, 0.9807852804032293204, 1.000000000000001110 ) ) 
 REPRESENTATION_ITEM ( '' )  );
#16605=CARTESIAN_POINT ( 'NONE',  ( -16.84014894278200813, 501.6198905683720000, -11.84573899990672707 ) ) ;
#16608=CARTESIAN_POINT ( 'NONE',  ( -40.01497788969915348, 518.8073905601785327, 16.95518130045146776 ) ) ;
#16610=CARTESIAN_POINT ( 'NONE',  ( -13.20868407381886556, 410.9948905683720000, -6.410867750099233042 ) ) ;
#16612=CARTESIAN_POINT ( 'NONE',  ( -22.27502019258946220, 238.4948905683720284, 15.47720386886985189 ) ) ;
#16613=CARTESIAN_POINT ( 'NONE',  ( -25.35362745456398059, 356.6823905683720568, 16.75240474999998952 ) ) ;
#16614=EDGE_LOOP ( 'NONE', ( #5446, #6831, #20067, #13962 ) ) ;
#16615=CARTESIAN_POINT ( 'NONE',  ( -11.93348319268874036, 518.5573905683720568, 3.332260488124728415 ) ) ;
#16617=CARTESIAN_POINT ( 'NONE',  ( -11.93348319268872970, 440.3698905683720000, -2.051577885510841163E-15 ) ) ;
#16619=CARTESIAN_POINT ( 'NONE',  ( -14.48388495494901917, 529.8073905683720568, -9.489475012073736337 ) ) ;
#16621=CARTESIAN_POINT ( 'NONE',  ( -8.685887942688820473, 431.9323905601784190, 3.978247347593374172 ) ) ;
#16622=CARTESIAN_POINT ( 'NONE',  ( -40.53162694259545162, 492.6198905683720000, -11.84573899990672707 ) ) ;
#16624=CARTESIAN_POINT ( 'NONE',  ( -45.43829269268872650, 503.5573905683720000, -3.332260488124726638 ) ) ;
#16627=CARTESIAN_POINT ( 'NONE',  ( -45.64106924314019409, 431.0573905765655809, -11.32908994701042715 ) ) ;
#16631=CARTESIAN_POINT ( 'NONE',  ( -45.64106924314019409, 452.9323905765656377, 11.32908994701042538 ) ) ;
#16633=ADVANCED_FACE ( 'NONE', ( #16049 ), #17761, .T. ) ;
#16636=CARTESIAN_POINT ( 'NONE',  ( -43.37414277151795261, 201.1719893629813498, -3.054701555947804792 ) ) ;
#16638=CARTESIAN_POINT ( 'NONE',  ( -14.48388495494899075, 291.3073905683720568, -9.489475012073736337 ) ) ;
#16640=CARTESIAN_POINT ( 'NONE',  ( -28.68588794268870501, 264.7448905601784759, -19.99999999999999289 ) ) ;
#16642=CARTESIAN_POINT ( 'NONE',  ( -45.43829269268870519, 285.3698905683720568, 0.000000000000000000 ) ) ;
#16645=CARTESIAN_POINT ( 'NONE',  ( -45.64106924314020119, 536.3073905601785327, -11.32908994701042538 ) ) ;
#16646=CARTESIAN_POINT ( 'NONE',  ( -35.09675569278796559, 497.2448905683720000, 15.47720386886985366 ) ) ;
#16648=EDGE_CURVE ( 'NONE', #18441, #8749, #1067, .T. ) ;
#16649=DIRECTION ( 'NONE',  ( -1.191790137725560488E-16, 1.000000000000000000, -0.000000000000000000 ) ) ;
#16651=CARTESIAN_POINT ( 'NONE',  ( -16.84014894278200103, 469.1198905683720568, 11.84573899990672530 ) ) ;
#16652=CARTESIAN_POINT ( 'NONE',  ( -24.70764059509556532, 409.1823905765656377, -19.99999999999999289 ) ) ;
#16653=CARTESIAN_POINT ( 'NONE',  ( -16.84014894278197616, 267.6198905683720568, 11.84573899990672530 ) ) ;
#16656=CARTESIAN_POINT ( 'NONE',  ( -14.48388495494898542, 241.3073905683720568, -9.489475012073734561 ) ) ;
#16658=CARTESIAN_POINT ( 'NONE',  ( -40.01497788969911795, 253.5573905765656093, 16.95518130045146776 ) ) ;
#16660=CARTESIAN_POINT ( 'NONE',  ( -47.16347859291443001, 227.8698905601784759, 7.653668647301805628 ) ) ;
#16661=CARTESIAN_POINT ( 'NONE',  ( -47.16347859291443001, 261.3698905765656377, -7.653668647301793193 ) ) ;
#16662=CARTESIAN_POINT ( 'NONE',  ( -25.35362745456398059, 261.0573905683720000, -16.75240474999999307 ) ) ;
#16663=CARTESIAN_POINT ( 'NONE',  ( -11.93348319268872260, 350.0573905683720000, 3.332260488124728415 ) ) ;
#16664=CARTESIAN_POINT ( 'NONE',  ( -47.16347859291443712, 277.8698905601784759, 7.653668647301805628 ) ) ;
#16665=( BOUNDED_CURVE ( )  B_SPLINE_CURVE ( 2, ( #13760, #16794, #2079, #5307, #361, #3587, #6822, #8553, #11803, #20140, #11908, #20346, #20455, #5206, #12123, #10173, #13438 ),
 .UNSPECIFIED., .F., .T. ) 
 B_SPLINE_CURVE_WITH_KNOTS ( ( 3, 2, 2, 2, 2, 2, 2, 2, 3 ),
 ( 0.3906250000000001665, 0.3925781250000001665, 0.3945312500000001665, 0.3964843750000001665, 0.3984375000000001665, 0.4003906250000001665, 0.4023437500000001665, 0.4042968750000001665, 0.4062500000000001665 ),
 .UNSPECIFIED. ) 
 CURVE ( )  GEOMETRIC_REPRESENTATION_ITEM ( )  RATIONAL_B_SPLINE_CURVE ( ( 0.9999999999999983347, 0.9807852804032320959, 1.000000000000000000, 0.9807852804032304306, 1.000000000000000000, 0.9807852804032304306, 1.000000000000000000, 0.9807852804032304306, 1.000000000000000000, 0.9807852804032304306, 1.000000000000000000, 0.9807852804032304306, 1.000000000000000000, 0.9807852804032304306, 1.000000000000000000, 0.9807852804032287652, 1.000000000000001554 ) ) 
 REPRESENTATION_ITEM ( '' )  );
#16666=CARTESIAN_POINT ( 'NONE',  ( -32.01814843081345430, 421.6823905683720568, -16.75240474999999307 ) ) ;
#16669=CARTESIAN_POINT ( 'NONE',  ( -21.03221929538693047, 414.1198905601785327, -18.47759065022572855 ) ) ;
#16672=ORIENTED_EDGE ( 'NONE', *, *, #18440, .F. ) ;
#16673=CARTESIAN_POINT ( 'NONE',  ( -19.19641293061500420, 521.9323905683720568, -14.20200298773971603 ) ) ;
#16674=CARTESIAN_POINT ( 'NONE',  ( -47.16347859291443712, 307.8698905601784759, 7.653668647301805628 ) ) ;
#16677=CARTESIAN_POINT ( 'NONE',  ( -25.35362745456398770, 322.5573905683720000, -16.75240474999999307 ) ) ;
#16678=CARTESIAN_POINT ( 'NONE',  ( -28.68588794268871212, 356.3698905683720568, 16.75240474999999307 ) ) ;
#16679=CARTESIAN_POINT ( 'NONE',  ( -28.68588794268871567, 361.3698905683720568, -16.75240474999999307 ) ) ;
#16680=CARTESIAN_POINT ( 'NONE',  ( -11.73070664223724258, 297.9323905765655240, -11.32908994701042715 ) ) ;
#16682=CARTESIAN_POINT ( 'NONE',  ( -45.43829269268870519, 274.1823905683720000, 3.332260488124734632 ) ) ;
#16683=CARTESIAN_POINT ( 'NONE',  ( -28.68588794268872277, 439.7448905601784759, 19.99999999999999289 ) ) ;
#16685=CARTESIAN_POINT ( 'NONE',  ( -38.17536295476245556, 426.9323905683720000, 14.20200298773971781 ) ) ;
#16686=CYLINDRICAL_SURFACE ( 'NONE', #18903, 19.99999999999999645 ) ;
#16688=DIRECTION ( 'NONE',  ( -1.191790137725560488E-16, 1.000000000000000000, -0.000000000000000000 ) ) ;
#16690=CARTESIAN_POINT ( 'NONE',  ( -38.17536295476244845, 323.8073905683719431, -14.20200298773971426 ) ) ;
#16691=CARTESIAN_POINT ( 'NONE',  ( -40.53162694259545162, 485.1198905683720000, 11.84573899990672885 ) ) ;
#16692=ORIENTED_EDGE ( 'NONE', *, *, #19748, .T. ) ;
#16693=CARTESIAN_POINT ( 'NONE',  ( -8.685887942688738761, 492.5573905601785327, -3.978247347593165895 ) ) ;
#16694=CARTESIAN_POINT ( 'NONE',  ( -16.84014894278198327, 310.1198905683720000, -11.84573899990672707 ) ) ;
#16696=CARTESIAN_POINT ( 'NONE',  ( -8.685887942688720997, 342.2448905601784759, -2.449293598294705724E-15 ) ) ;
#16698=CARTESIAN_POINT ( 'NONE',  ( -48.68588794268873698, 573.2448905601785327, 0.000000000000000000 ) ) ;
#16700=CARTESIAN_POINT ( 'NONE',  ( -22.27502019258949062, 402.2448905683720568, -15.47720386886985544 ) ) ;
#16701=CARTESIAN_POINT ( 'NONE',  ( -36.33955658999052929, 479.1198905601785327, 18.47759065022572500 ) ) ;
#16702=CARTESIAN_POINT ( 'NONE',  ( -40.01497788969913216, 383.5573905765656377, 16.95518130045146776 ) ) ;
#16703=CARTESIAN_POINT ( 'NONE',  ( -22.27502019258949417, 430.7448905683720000, -15.47720386886985544 ) ) ;
#16704=CARTESIAN_POINT ( 'NONE',  ( -42.88789093042841927, 256.3073905683720568, 9.489475012073736337 ) ) ;
#16706=CARTESIAN_POINT ( 'NONE',  ( -42.88789093042844058, 424.8073905683719431, 9.489475012073734561 ) ) ;
#16707=LINE ( 'NONE', #19834, #8035 ) ;
#16708=CARTESIAN_POINT ( 'NONE',  ( -14.54375231895777176, 368.2448905765656377, -14.14213562373094746 ) ) ;
#16709=CARTESIAN_POINT ( 'NONE',  ( -42.82802356641965247, 275.9948905601785327, -14.14213562373094746 ) ) ;
#16711=CARTESIAN_POINT ( 'NONE',  ( -38.17536295476244845, 335.4323905683720000, 14.20200298773971781 ) ) ;
#16713=CARTESIAN_POINT ( 'NONE',  ( -11.93348319268873681, 490.0573905683720568, 3.332260488124728415 ) ) ;
#16719=CARTESIAN_POINT ( 'NONE',  ( -25.35362745456398414, 398.1823905683720568, 16.75240474999998952 ) ) ;
#16720=CARTESIAN_POINT ( 'NONE',  ( -48.68588794268869435, 261.9948905765655809, 0.000000000000000000 ) ) ;
#16721=CARTESIAN_POINT ( 'NONE',  ( -44.16309181155855867, 224.7448905683720568, -6.410867750099231266 ) ) ;
#16722=CARTESIAN_POINT ( 'NONE',  ( -19.19641293061498644, 360.4323905683720000, -14.20200298773971603 ) ) ;
#16724=ORIENTED_EDGE ( 'NONE', *, *, #4648, .T. ) ;
#16725=CARTESIAN_POINT ( 'NONE',  ( -13.20868407381887977, 519.4948905683720568, -6.410867750099233042 ) ) ;
#16726=ORIENTED_EDGE ( 'NONE', *, *, #13647, .T. ) ;
#16727=CARTESIAN_POINT ( 'NONE',  ( -35.09675569278795138, 443.4948905683720568, -15.47720386886985544 ) ) ;
#16728=CARTESIAN_POINT ( 'NONE',  ( -38.17536295476246977, 515.4323905683720568, 14.20200298773971781 ) ) ;
#16732=CARTESIAN_POINT ( 'NONE',  ( -25.35362745456400901, 491.0573905683720000, -16.75240474999999307 ) ) ;
#16733=ORIENTED_EDGE ( 'NONE', *, *, #10344, .F. ) ;
#16734=CARTESIAN_POINT ( 'NONE',  ( -22.27502019258949417, 506.9948905683721136, 15.47720386886985189 ) ) ;
#16737=CARTESIAN_POINT ( 'NONE',  ( -17.35679799567830628, 428.5573905765656377, -16.95518130045146421 ) ) ;
#16738=CARTESIAN_POINT ( 'NONE',  ( -32.66413529028186957, 359.8073905765656946, -19.99999999999999289 ) ) ;
#16741=DIRECTION ( 'NONE',  ( -1.191790137725560488E-16, 1.000000000000000000, -0.000000000000000000 ) ) ;
#16744=CARTESIAN_POINT ( 'NONE',  ( -42.93756312153262655, 203.3739285472156268, -4.679109617540635924 ) ) ;
#16745=CARTESIAN_POINT ( 'NONE',  ( -25.35362745456397349, 288.1823905683720000, 16.75240474999998952 ) ) ;
#16746=CARTESIAN_POINT ( 'NONE',  ( -42.82802356641968089, 528.4948905601785327, 14.14213562373094923 ) ) ;
#16747=CARTESIAN_POINT ( 'NONE',  ( -47.16347859291443001, 266.6198905601784759, -7.653668647301793193 ) ) ;
#16748=LINE ( 'NONE', #20092, #20622 ) ;
#16750=CARTESIAN_POINT ( 'NONE',  ( -40.53162694259543031, 284.1198905683720000, -11.84573899990672707 ) ) ;
#16753=CARTESIAN_POINT ( 'NONE',  ( -14.48388495494901385, 509.4323905683720000, 9.489475012073731008 ) ) ;
#16755=CARTESIAN_POINT ( 'NONE',  ( -11.93348319268873325, 460.3698905683720000, -2.051577885510841163E-15 ) ) ;
#16756=CARTESIAN_POINT ( 'NONE',  ( -11.73070664223725501, 407.9323905765656377, -11.32908994701042538 ) ) ;
#16757=CARTESIAN_POINT ( 'NONE',  ( -32.01814843081343298, 261.6823905683720568, -16.75240474999999307 ) ) ;
#16758=ORIENTED_EDGE ( 'NONE', *, *, #14701, .F. ) ;
#16759=CARTESIAN_POINT ( 'NONE',  ( -21.03221929538690560, 335.1198905765655809, 18.47759065022572500 ) ) ;
#16760=CARTESIAN_POINT ( 'NONE',  ( -25.35362745456397704, 252.5573905683720000, -16.75240474999999307 ) ) ;
#16761=CARTESIAN_POINT ( 'NONE',  ( -21.03221929538689849, 245.1198905765656377, 18.47759065022572500 ) ) ;
#16763=CARTESIAN_POINT ( 'NONE',  ( -42.82802356641964536, 235.9948905601784759, -14.14213562373094746 ) ) ;
#16764=CARTESIAN_POINT ( 'NONE',  ( -22.27502019258946575, 276.9948905683720000, 15.47720386886985189 ) ) ;
#16765=EDGE_CURVE ( 'NONE', #20871, #20201, #9743, .T. ) ;
#16766=CARTESIAN_POINT ( 'NONE',  ( -38.17536295476245556, 353.8073905683720568, -14.20200298773971426 ) ) ;
#16767=CARTESIAN_POINT ( 'NONE',  ( -28.68588794268873343, 504.7448905601785896, -19.99999999999999289 ) ) ;
#16769=CARTESIAN_POINT ( 'NONE',  ( -16.84014894278199037, 397.6198905683720568, 11.84573899990672530 ) ) ;
#16772=CARTESIAN_POINT ( 'NONE',  ( -42.82802356641966668, 398.4948905601784759, 14.14213562373094923 ) ) ;
#16774=VERTEX_POINT ( 'NONE', #8333 ) ;
#16775=B_SPLINE_CURVE_WITH_KNOTS ( 'NONE', 3,
 ( #2771, #12611, #4281, #19203, #4385, #3082, #1154, #21039, #1252, #10970, #6003, #15863, #7616, #17686, #17578, #14561, #11292, #4596, #21146, #9353, #15968, #14458, #12716, #944 ),
 .UNSPECIFIED., .F., .F.,
 ( 4, 2, 2, 2, 2, 2, 2, 2, 2, 2, 2, 4 ),
 ( 0.000000000000000000, 0.002720743832753576025, 0.005441487665507152051, 0.006801859581883942449, 0.008162231498260731979, 0.01088297533101431798, 0.01224334724739110924, 0.01360371916376789878, 0.01632446299652147784, 0.01768483491289826390, 0.01904520682927505343, 0.02176595066202864637 ),
 .UNSPECIFIED. ) ;
#16778=CARTESIAN_POINT ( 'NONE',  ( -28.68588794268873698, 522.8698905683719431, -16.75240474999999307 ) ) ;
#16779=CARTESIAN_POINT ( 'NONE',  ( -8.685887942688713892, 292.5573905601784759, -3.978247347593165895 ) ) ;
#16780=CARTESIAN_POINT ( 'NONE',  ( -43.31958977256851995, 208.9114094701607485, -3.303159798271271708 ) ) ;
#16781=CARTESIAN_POINT ( 'NONE',  ( -38.17536295476244845, 323.8073905683720000, -14.20200298773971426 ) ) ;
#16783=CARTESIAN_POINT ( 'NONE',  ( -38.17536295476244845, 355.4323905683720568, 14.20200298773971781 ) ) ;
#16784=CARTESIAN_POINT ( 'NONE',  ( -16.84014894278199037, 370.1198905683720000, -11.84573899990672707 ) ) ;
#16785=CARTESIAN_POINT ( 'NONE',  ( -40.01497788969912506, 303.5573905765656377, 16.95518130045146776 ) ) ;
#16787=CARTESIAN_POINT ( 'NONE',  ( -11.93348319268870839, 258.5573905683720000, 3.332260488124728859 ) ) ;
#16789=( BOUNDED_CURVE ( )  B_SPLINE_CURVE ( 2, ( #7484, #3319, #13164, #6438, #6869, #3426, #8272, #1704, #196, #1819, #19751, #6546, #16414, #1592, #18234, #4934, #15118 ),
 .UNSPECIFIED., .F., .T. ) 
 B_SPLINE_CURVE_WITH_KNOTS ( ( 3, 2, 2, 2, 2, 2, 2, 2, 3 ),
 ( 0.6406250000000002220, 0.6425781250000002220, 0.6445312500000002220, 0.6464843750000001110, 0.6484375000000001110, 0.6503906250000001110, 0.6523437500000000000, 0.6542968750000000000, 0.6562500000000000000 ),
 .UNSPECIFIED. ) 
 CURVE ( )  GEOMETRIC_REPRESENTATION_ITEM ( )  RATIONAL_B_SPLINE_CURVE ( ( 0.9999999999999977796, 0.9807852804032326510, 1.000000000000000000, 0.9807852804032304306, 1.000000000000000000, 0.9807852804032304306, 1.000000000000000000, 0.9807852804032304306, 1.000000000000000000, 0.9807852804032304306, 1.000000000000000000, 0.9807852804032304306, 1.000000000000000000, 0.9807852804032304306, 1.000000000000000000, 0.9807852804032304306, 1.000000000000000000 ) ) 
 REPRESENTATION_ITEM ( '' )  );
#16790=CARTESIAN_POINT ( 'NONE',  ( -19.19641293061498999, 421.9323905683720000, -14.20200298773971603 ) ) ;
#16791=CARTESIAN_POINT ( 'NONE',  ( -48.68588794268873698, 573.2448905601785327, 0.000000000000000000 ) ) ;
#16793=CARTESIAN_POINT ( 'NONE',  ( -8.685887942688722774, 362.2448905601784190, -2.449293598294705724E-15 ) ) ;
#16794=CARTESIAN_POINT ( 'NONE',  ( -8.685887942688859553, 411.9323905601784190, 3.978247347593479866 ) ) ;
#16795=CARTESIAN_POINT ( 'NONE',  ( -13.20868407381885312, 319.7448905683720000, 6.410867750099229490 ) ) ;
#16796=CARTESIAN_POINT ( 'NONE',  ( -38.17536295476246266, 475.4323905683720568, 14.20200298773971781 ) ) ;
#16798=CARTESIAN_POINT ( 'NONE',  ( -47.16347859291445843, 457.8698905601785327, 7.653668647301805628 ) ) ;
#16799=CARTESIAN_POINT ( 'NONE',  ( -45.43829269268869808, 313.5573905683720000, -3.332260488124726194 ) ) ;
#16801=ORIENTED_EDGE ( 'NONE', *, *, #1134, .T. ) ;
#16803=CARTESIAN_POINT ( 'NONE',  ( -36.33955658999050797, 345.3698905601784759, -18.47759065022572855 ) ) ;
#16804=CARTESIAN_POINT ( 'NONE',  ( -28.68588794268871922, 392.8698905683720000, -16.75240474999999307 ) ) ;
#16806=CYLINDRICAL_SURFACE ( 'NONE', #16978, 19.99999999999999645 ) ;
#16807=CARTESIAN_POINT ( 'NONE',  ( -45.43829269268871229, 424.1823905683721136, 3.332260488124734632 ) ) ;
#16808=CARTESIAN_POINT ( 'NONE',  ( -32.01814843081343298, 263.1823905683720000, -16.75240474999999307 ) ) ;
#16809=CARTESIAN_POINT ( 'NONE',  ( -16.84014894278199748, 430.1198905683720000, -11.84573899990672707 ) ) ;
#16813=CARTESIAN_POINT ( 'NONE',  ( -11.73070664223724968, 366.0573905765655809, 11.32908994701042005 ) ) ;
#16814=CARTESIAN_POINT ( 'NONE',  ( -8.685887942688720997, 346.9948905765656377, -2.449293598294705724E-15 ) ) ;
#16816=CARTESIAN_POINT ( 'NONE',  ( -42.88789093042842637, 324.8073905683720000, 9.489475012073734561 ) ) ;
#16818=CARTESIAN_POINT ( 'NONE',  ( -21.03221929538691981, 435.1198905765656377, 18.47759065022572500 ) ) ;
#16820=CARTESIAN_POINT ( 'NONE',  ( -45.64106924314017277, 306.3073905601784190, -11.32908994701042538 ) ) ;
#16822=CARTESIAN_POINT ( 'NONE',  ( -38.17536295476245556, 383.8073905683720568, -14.20200298773971426 ) ) ;
#16825=CARTESIAN_POINT ( 'NONE',  ( -32.66413529028189799, 529.4323905601785327, 19.99999999999999289 ) ) ;
#16826=CARTESIAN_POINT ( 'NONE',  ( -16.84014894278198682, 357.6198905683720000, 11.84573899990672530 ) ) ;
#16829=CARTESIAN_POINT ( 'NONE',  ( -22.27502019258949773, 526.9948905683720568, 15.47720386886985189 ) ) ;
#16831=CARTESIAN_POINT ( 'NONE',  ( -16.84014894278201169, 520.1198905683720568, -11.84573899990672707 ) ) ;
#16833=CARTESIAN_POINT ( 'NONE',  ( -21.03221929538694113, 494.1198905601784759, -18.47759065022572855 ) ) ;
#16834=CARTESIAN_POINT ( 'NONE',  ( -40.53162694259545162, 485.1198905683720000, 11.84573899990672885 ) ) ;
#16836=CARTESIAN_POINT ( 'NONE',  ( -22.27502019258949062, 486.9948905683720568, 15.47720386886985189 ) ) ;
#16838=VECTOR ( 'NONE', #20726, 1000.000000000000000 ) ;
#16839=CARTESIAN_POINT ( 'NONE',  ( -32.66413529028188378, 429.8073905765656946, -19.99999999999999289 ) ) ;
#16842=CARTESIAN_POINT ( 'NONE',  ( -32.66413529028187668, 439.8073905765656946, -19.99999999999999289 ) ) ;
#16846=CARTESIAN_POINT ( 'NONE',  ( -42.82802356641966668, 435.9948905601784759, -14.14213562373094746 ) ) ;
#16847=CARTESIAN_POINT ( 'NONE',  ( -10.20829729246300310, 496.3698905765655809, 7.653668647301790529 ) ) ;
#16848=CARTESIAN_POINT ( 'NONE',  ( -25.35362745456397349, 298.1823905683720000, 16.75240474999998952 ) ) ;
#16850=CARTESIAN_POINT ( 'NONE',  ( -14.48388495494900852, 441.3073905683720568, -9.489475012073736337 ) ) ;
#16851=CARTESIAN_POINT ( 'NONE',  ( -22.27502019258946930, 288.4948905683720000, 15.47720386886985189 ) ) ;
#16853=ORIENTED_EDGE ( 'NONE', *, *, #20462, .F. ) ;
#16855=CARTESIAN_POINT ( 'NONE',  ( -14.48388495494901562, 501.3073905683720568, -9.489475012073734561 ) ) ;
#16859=CARTESIAN_POINT ( 'NONE',  ( -11.93348319268873503, 470.6823905683720568, -3.332260488124732856 ) ) ;
#16861=CARTESIAN_POINT ( 'NONE',  ( -45.43829269268869098, 254.1823905683719715, 3.332260488124734632 ) ) ;
#16862=VERTEX_POINT ( 'NONE', #20344 ) ;
#16865=CARTESIAN_POINT ( 'NONE',  ( -44.16309181155855157, 245.9948905683720284, 6.410867750099241924 ) ) ;
#16867=CARTESIAN_POINT ( 'NONE',  ( -10.20829729246297823, 311.6198905601784759, 7.653668647301790529 ) ) ;
#16869=CARTESIAN_POINT ( 'NONE',  ( -13.20868407381884779, 268.2448905683720568, 6.410867750099229490 ) ) ;
#16870=CARTESIAN_POINT ( 'NONE',  ( -14.48388495494899786, 359.4323905683719431, 9.489475012073732785 ) ) ;
#16871=CARTESIAN_POINT ( 'NONE',  ( -17.35679799567831338, 503.8073905601785327, -16.95518130045146421 ) ) ;
#16872=CARTESIAN_POINT ( 'NONE',  ( -16.84014894278199392, 407.6198905683720568, 11.84573899990672530 ) ) ;
#16873=CARTESIAN_POINT ( 'NONE',  ( -10.20829729246300310, 511.6198905601785327, 7.653668647301790529 ) ) ;
#16874=CARTESIAN_POINT ( 'NONE',  ( -48.68588794268871567, 396.9323905601785327, -3.978247347593158345 ) ) ;
#16875=ORIENTED_EDGE ( 'NONE', *, *, #18846, .F. ) ;
#16878=VERTEX_POINT ( 'NONE', #10171 ) ;
#16879=CARTESIAN_POINT ( 'NONE',  ( -11.93348319268874214, 530.0573905683720568, 3.332260488124728415 ) ) ;
#16880=CARTESIAN_POINT ( 'NONE',  ( -36.33955658999050087, 285.3698905601784759, -18.47759065022572855 ) ) ;
#16882=CARTESIAN_POINT ( 'NONE',  ( -32.01814843081344009, 317.5573905683720568, 16.75240474999999307 ) ) ;
#16884=CARTESIAN_POINT ( 'NONE',  ( -13.20868407381886023, 368.2448905683720000, 6.410867750099229490 ) ) ;
#16885=CARTESIAN_POINT ( 'NONE',  ( -19.19641293061498288, 370.4323905683719431, -14.20200298773971603 ) ) ;
#16886=CARTESIAN_POINT ( 'NONE',  ( -14.54375231895776466, 308.2448905765656377, -14.14213562373094746 ) ) ;
#16888=CARTESIAN_POINT ( 'NONE',  ( -19.19641293061496867, 267.3073905683720568, 14.20200298773971426 ) ) ;
#16889=CARTESIAN_POINT ( 'NONE',  ( -21.03221929538692336, 465.1198905765655809, 18.47759065022572500 ) ) ;
#16891=ADVANCED_FACE ( 'NONE', ( #5408 ), #16686, .T. ) ;
#16892=CARTESIAN_POINT ( 'NONE',  ( -25.35362745456399836, 412.5573905683719431, -16.75240474999999307 ) ) ;
#16895=CARTESIAN_POINT ( 'NONE',  ( -11.73070664223724791, 353.1823905601785327, -11.32908994701042538 ) ) ;
#16896=CARTESIAN_POINT ( 'NONE',  ( -17.35679799567828141, 305.4323905765655809, 16.95518130045146421 ) ) ;
#16898=CARTESIAN_POINT ( 'NONE',  ( -32.01814843081344009, 323.1823905683720000, -16.75240474999999307 ) ) ;
#16899=CARTESIAN_POINT ( 'NONE',  ( -40.53162694259545162, 472.6198905683720000, -11.84573899990672707 ) ) ;
#16901=CARTESIAN_POINT ( 'NONE',  ( -45.64106924314020119, 466.3073905601785327, -11.32908994701042715 ) ) ;
#16902=CARTESIAN_POINT ( 'NONE',  ( -28.68588794268870856, 291.3698905683720568, -16.75240474999999307 ) ) ;
#16903=EDGE_CURVE ( 'NONE', #7992, #126, #3688, .T. ) ;
#16907=CARTESIAN_POINT ( 'NONE',  ( -48.68588794268870856, 347.5573905601784759, 3.978247347593168115 ) ) ;
#16908=EDGE_CURVE ( 'NONE', #11409, #12297, #13758, .T. ) ;
#16909=CARTESIAN_POINT ( 'NONE',  ( -13.20868407381886200, 389.7448905683720000, 6.410867750099229490 ) ) ;
#16910=CARTESIAN_POINT ( 'NONE',  ( -36.33955658999050087, 295.3698905601784759, -18.47759065022572855 ) ) ;
#16911=CYLINDRICAL_SURFACE ( 'NONE', #5546, 19.99999999999999645 ) ;
#16912=CARTESIAN_POINT ( 'NONE',  ( -13.20868407381886733, 419.4948905683720000, -6.410867750099233042 ) ) ;
#16913=CARTESIAN_POINT ( 'NONE',  ( -35.09675569278793006, 263.4948905683720000, -15.47720386886985544 ) ) ;
#16914=CARTESIAN_POINT ( 'NONE',  ( -14.48388495494900674, 417.9323905683720568, 9.489475012073731008 ) ) ;
#16916=( BOUNDED_CURVE ( )  B_SPLINE_CURVE ( 2, ( #20648, #12428, #4631, #19341, #9495, #15795, #14284, #17822, #19448, #4421, #11225, #16216, #17508, #12543, #7863, #17718, #982 ),
 .UNSPECIFIED., .F., .T. ) 
 B_SPLINE_CURVE_WITH_KNOTS ( ( 3, 2, 2, 2, 2, 2, 2, 2, 3 ),
 ( 0.4062500000000001665, 0.4082031250000001665, 0.4101562500000001665, 0.4121093750000001665, 0.4140625000000001665, 0.4160156250000001665, 0.4179687500000001665, 0.4199218750000001665, 0.4218750000000001665 ),
 .UNSPECIFIED. ) 
 CURVE ( )  GEOMETRIC_REPRESENTATION_ITEM ( )  RATIONAL_B_SPLINE_CURVE ( ( 0.9999999999999983347, 0.9807852804032320959, 1.000000000000000000, 0.9807852804032304306, 1.000000000000000000, 0.9807852804032304306, 1.000000000000000000, 0.9807852804032304306, 1.000000000000000000, 0.9807852804032304306, 1.000000000000000000, 0.9807852804032304306, 1.000000000000000000, 0.9807852804032304306, 1.000000000000000000, 0.9807852804032287652, 1.000000000000001554 ) ) 
 REPRESENTATION_ITEM ( '' )  );
#16917=CARTESIAN_POINT ( 'NONE',  ( -28.68588794268871212, 354.4948905765656377, 19.99999999999999289 ) ) ;
#16918=CARTESIAN_POINT ( 'NONE',  ( -36.33955658999050087, 275.3698905601784759, -18.47759065022572855 ) ) ;
#16920=CARTESIAN_POINT ( 'NONE',  ( -16.84014894278198682, 320.1198905683720568, -11.84573899990672707 ) ) ;
#16921=CARTESIAN_POINT ( 'NONE',  ( -21.03221929538694113, 488.8698905765655809, -18.47759065022572855 ) ) ;
#16922=CARTESIAN_POINT ( 'NONE',  ( -13.20868407381887089, 469.7448905683720568, 6.410867750099229490 ) ) ;
#16923=EDGE_CURVE ( 'NONE', #18084, #21047, #252, .T. ) ;
#16924=CARTESIAN_POINT ( 'NONE',  ( -45.64106924314018698, 432.9323905765656946, 11.32908994701042538 ) ) ;
#16928=CARTESIAN_POINT ( 'NONE',  ( -14.48388495494900141, 389.4323905683720568, 9.489475012073732785 ) ) ;
#16929=CARTESIAN_POINT ( 'NONE',  ( -48.68588794268873698, 573.2448905601785327, 0.000000000000000000 ) ) ;
#16930=CARTESIAN_POINT ( 'NONE',  ( -36.33955658999053639, 529.1198905601785327, 18.47759065022572500 ) ) ;
#16931=CARTESIAN_POINT ( 'NONE',  ( -35.09675569278795138, 355.7448905683720568, 15.47720386886985366 ) ) ;
#16932=VERTEX_POINT ( 'NONE', #5518 ) ;
#16933=CARTESIAN_POINT ( 'NONE',  ( -40.53162694259545873, 525.1198905683720568, 11.84573899990672885 ) ) ;
#16935=CARTESIAN_POINT ( 'NONE',  ( -13.20868407381887799, 518.2448905683720568, 6.410867750099229490 ) ) ;
#16937=CARTESIAN_POINT ( 'NONE',  ( -48.68588794268872988, 531.9948905765656946, 0.000000000000000000 ) ) ;
#16938=CARTESIAN_POINT ( 'NONE',  ( -25.35362745456399480, 476.6823905683720000, 16.75240474999998952 ) ) ;
#16940=CARTESIAN_POINT ( 'NONE',  ( -42.88789093042844769, 484.8073905683720000, 9.489475012073734561 ) ) ;
#16942=CARTESIAN_POINT ( 'NONE',  ( -47.16347859291445133, 431.3698905765655809, -7.653668647301793193 ) ) ;
#16943=CARTESIAN_POINT ( 'NONE',  ( -48.68588794268885778, 472.3073905765656377, 3.978247347592849259 ) ) ;
#16950=CARTESIAN_POINT ( 'NONE',  ( -28.68588794268870856, 302.8698905683720000, -16.75240474999999307 ) ) ;
#16952=CARTESIAN_POINT ( 'NONE',  ( -19.19641293061498999, 448.8073905683720568, 14.20200298773971426 ) ) ;
#16954=CARTESIAN_POINT ( 'NONE',  ( -14.48388495494898720, 269.4323905683720568, 9.489475012073732785 ) ) ;
#16957=CARTESIAN_POINT ( 'NONE',  ( -42.82802356641964536, 268.4948905601784759, 14.14213562373094923 ) ) ;
#16958=CARTESIAN_POINT ( 'NONE',  ( -25.35362745456400901, 502.5573905683720000, -16.75240474999999307 ) ) ;
#16963=CARTESIAN_POINT ( 'NONE',  ( -42.88789093042844769, 476.3073905683720000, 9.489475012073736337 ) ) ;
#16965=CARTESIAN_POINT ( 'NONE',  ( -45.43829269268869098, 253.5573905683720284, -3.332260488124726194 ) ) ;
#16969=CARTESIAN_POINT ( 'NONE',  ( -17.35679799567830983, 478.5573905765656377, -16.95518130045146421 ) ) ;
#16970=CYLINDRICAL_SURFACE ( 'NONE', #13776, 19.99999999999999645 ) ;
#16971=CARTESIAN_POINT ( 'NONE',  ( -40.53162694259542320, 244.1198905683720284, -11.84573899990672707 ) ) ;
#16973=CARTESIAN_POINT ( 'NONE',  ( -28.68588794268869790, 224.7448905601784759, -19.99999999999999289 ) ) ;
#16974=CARTESIAN_POINT ( 'NONE',  ( -32.01814843081343298, 251.6823905683720568, -16.75240474999999307 ) ) ;
#16975=CARTESIAN_POINT ( 'NONE',  ( -42.88789093042843348, 364.4323905683720568, -9.489475012073736337 ) ) ;
#16976=EDGE_CURVE ( 'NONE', #368, #18118, #12012, .T. ) ;
#16978=AXIS2_PLACEMENT_3D ( 'NONE', #2091, #8672, #15296 ) ;
#16980=CARTESIAN_POINT ( 'NONE',  ( -11.93348319268872615, 398.8698905683720000, -2.051577885510841163E-15 ) ) ;
#16981=CARTESIAN_POINT ( 'NONE',  ( -21.03221929538691981, 338.8698905765656377, -18.47759065022572855 ) ) ;
#16982=CARTESIAN_POINT ( 'NONE',  ( -42.82802356641966668, 405.9948905601785327, -14.14213562373094746 ) ) ;
#16983=EDGE_CURVE ( 'NONE', #15984, #19418, #17471, .T. ) ;
#16987=ORIENTED_EDGE ( 'NONE', *, *, #9889, .T. ) ;
#16988=CARTESIAN_POINT ( 'NONE',  ( -45.43829269268873361, 535.3698905683720568, 0.000000000000000000 ) ) ;
#16989=CARTESIAN_POINT ( 'NONE',  ( -10.20829729246297646, 281.6198905601784759, 7.653668647301790529 ) ) ;
#16990=CARTESIAN_POINT ( 'NONE',  ( -43.52372910701232911, 209.6355236139544331, -2.220491386914098531 ) ) ;
#16991=CARTESIAN_POINT ( 'NONE',  ( -44.16309181155856578, 314.7448905683720000, -6.410867750099231266 ) ) ;
#16993=VERTEX_POINT ( 'NONE', #2821 ) ;
#16994=CARTESIAN_POINT ( 'NONE',  ( -22.27502019258948351, 340.7448905683720568, -15.47720386886985544 ) ) ;
#16995=CARTESIAN_POINT ( 'NONE',  ( -45.43829269268871229, 374.1823905683720568, 3.332260488124734632 ) ) ;
#16996=CARTESIAN_POINT ( 'NONE',  ( -45.64106924314017988, 292.9323905765656377, 11.32908994701042715 ) ) ;
#16998=CARTESIAN_POINT ( 'NONE',  ( -45.43829269268869808, 263.8698905683720000, 0.000000000000000000 ) ) ;
#16999=CARTESIAN_POINT ( 'NONE',  ( -48.68588794268872277, 461.9948905765656377, 0.000000000000000000 ) ) ;
#17000=CARTESIAN_POINT ( 'NONE',  ( -11.93348319268872615, 410.6823905683720000, -3.332260488124732856 ) ) ;
#17002=CARTESIAN_POINT ( 'NONE',  ( -17.35679799567830628, 505.4323905765656377, 16.95518130045146421 ) ) ;
#17004=CARTESIAN_POINT ( 'NONE',  ( -22.27502019258948351, 322.2448905683720000, -15.47720386886985544 ) ) ;
#17005=CARTESIAN_POINT ( 'NONE',  ( -38.17536295476246977, 472.3073905683720568, -14.20200298773971426 ) ) ;
#17008=CARTESIAN_POINT ( 'NONE',  ( -11.73070664223726389, 473.1823905601784190, -11.32908994701042715 ) ) ;
#17009=CARTESIAN_POINT ( 'NONE',  ( -44.16309181155855867, 284.4948905683720000, 6.410867750099241924 ) ) ;
#17010=ORIENTED_EDGE ( 'NONE', *, *, #13008, .T. ) ;
#17012=CARTESIAN_POINT ( 'NONE',  ( -48.68588794268870856, 336.9323905601784759, -3.978247347593158345 ) ) ;
#17013=CARTESIAN_POINT ( 'NONE',  ( -40.53162694259543031, 302.6198905683720000, -11.84573899990672707 ) ) ;
#17014=CARTESIAN_POINT ( 'NONE',  ( -19.19641293061498288, 388.8073905683720568, 14.20200298773971426 ) ) ;
#17015=CARTESIAN_POINT ( 'NONE',  ( -48.68588794268870146, 297.2448905601784759, 0.000000000000000000 ) ) ;
#17016=CARTESIAN_POINT ( 'NONE',  ( -24.70764059509558308, 519.1823905765655809, -19.99999999999999289 ) ) ;
#17017=CARTESIAN_POINT ( 'NONE',  ( -35.09675569278795848, 405.7448905683720568, 15.47720386886985366 ) ) ;
#17018=CARTESIAN_POINT ( 'NONE',  ( -16.84014894278197616, 269.1198905683720568, 11.84573899990672530 ) ) ;
#17020=CARTESIAN_POINT ( 'NONE',  ( -25.35362745456398770, 416.6823905683720568, 16.75240474999998952 ) ) ;
#17021=CARTESIAN_POINT ( 'NONE',  ( -47.16347859291444422, 372.6198905765655809, 7.653668647301805628 ) ) ;
#17023=CARTESIAN_POINT ( 'NONE',  ( -35.09675569278793716, 321.9948905683720568, -15.47720386886985544 ) ) ;
#17025=CARTESIAN_POINT ( 'NONE',  ( -42.88789093042844769, 484.4323905683719431, -9.489475012073736337 ) ) ;
#17026=ADVANCED_FACE ( 'NONE', ( #20985 ), #19253, .T. ) ;
#17032=CARTESIAN_POINT ( 'NONE',  ( -11.93348319268872260, 380.3698905683720568, -2.051577885510841163E-15 ) ) ;
#17033=CARTESIAN_POINT ( 'NONE',  ( -8.685887942688742314, 573.2448905601785327, 2.449293598294706119E-15 ) ) ;
#17034=CARTESIAN_POINT ( 'NONE',  ( -8.685887942688740537, 522.2448905601784190, -2.449293598294705724E-15 ) ) ;
#17035=CARTESIAN_POINT ( 'NONE',  ( -38.17536295476245556, 352.3073905683720000, -14.20200298773971426 ) ) ;
#17037=CARTESIAN_POINT ( 'NONE',  ( -25.35362745456399836, 516.6823905683720568, 16.75240474999998952 ) ) ;
#17039=( BOUNDED_CURVE ( )  B_SPLINE_CURVE ( 2, ( #12270, #15636, #7281, #2433, #7388, #14015, #12163, #1216, #17249, #18750, #15528, #17040, #20594, #20494, #6165, #12051, #14418 ),
 .UNSPECIFIED., .F., .T. ) 
 B_SPLINE_CURVE_WITH_KNOTS ( ( 3, 2, 2, 2, 2, 2, 2, 2, 3 ),
 ( 0.4687500000000002220, 0.4707031250000002220, 0.4726562500000002220, 0.4746093750000002220, 0.4765625000000002220, 0.4785156250000002220, 0.4804687500000002220, 0.4824218750000002220, 0.4843750000000002220 ),
 .UNSPECIFIED. ) 
 CURVE ( )  GEOMETRIC_REPRESENTATION_ITEM ( )  RATIONAL_B_SPLINE_CURVE ( ( 0.9999999999999977796, 0.9807852804032326510, 1.000000000000000000, 0.9807852804032304306, 1.000000000000000000, 0.9807852804032304306, 1.000000000000000000, 0.9807852804032304306, 1.000000000000000000, 0.9807852804032304306, 1.000000000000000000, 0.9807852804032304306, 1.000000000000000000, 0.9807852804032304306, 1.000000000000000000, 0.9807852804032282101, 1.000000000000002220 ) ) 
 REPRESENTATION_ITEM ( '' )  );
#17040=CARTESIAN_POINT ( 'NONE',  ( -17.35679799567829917, 378.5573905765656946, -16.95518130045146421 ) ) ;
#17044=CARTESIAN_POINT ( 'NONE',  ( -32.66413529028188378, 495.0573905601784759, -19.99999999999999289 ) ) ;
#17045=CARTESIAN_POINT ( 'NONE',  ( -38.17536295476246977, 492.3073905683720000, -14.20200298773971426 ) ) ;
#17047=CARTESIAN_POINT ( 'NONE',  ( -45.43829269268872650, 493.5573905683720000, -3.332260488124726638 ) ) ;
#17050=CARTESIAN_POINT ( 'NONE',  ( -8.685887942688729879, 426.6823905765655809, 3.978247347593161010 ) ) ;
#17054=CARTESIAN_POINT ( 'NONE',  ( -36.33955658999052929, 483.8698905765656377, 18.47759065022572500 ) ) ;
#17055=DIRECTION ( 'NONE',  ( -1.000000000000000000, 0.000000000000000000, 0.000000000000000000 ) ) ;
#17056=CARTESIAN_POINT ( 'NONE',  ( -11.73070664223725856, 433.1823905601784759, -11.32908994701042538 ) ) ;
#17058=CARTESIAN_POINT ( 'NONE',  ( -25.35362745456396993, 278.1823905683720000, 16.75240474999998952 ) ) ;
#17059=CARTESIAN_POINT ( 'NONE',  ( -47.16347859291443001, 256.6198905601784759, -7.653668647301793193 ) ) ;
#17060=CARTESIAN_POINT ( 'NONE',  ( -11.73070664223724968, 406.0573905765655240, 11.32908994701042005 ) ) ;
#17061=CARTESIAN_POINT ( 'NONE',  ( -40.53162694259544452, 444.1198905683720568, -11.84573899990672707 ) ) ;
#17062=CARTESIAN_POINT ( 'NONE',  ( -48.68588794268871567, 401.9948905765656377, 0.000000000000000000 ) ) ;
#17063=CARTESIAN_POINT ( 'NONE',  ( -44.16309181155855867, 275.9948905683720000, 6.410867750099241924 ) ) ;
#17065=ORIENTED_EDGE ( 'NONE', *, *, #13854, .T. ) ;
#17067=CARTESIAN_POINT ( 'NONE',  ( -38.17536295476246266, 476.9323905683720568, 14.20200298773971781 ) ) ;
#17071=CARTESIAN_POINT ( 'NONE',  ( -11.93348319268871194, 269.1823905683720000, -3.332260488124732856 ) ) ;
#17074=CARTESIAN_POINT ( 'NONE',  ( -14.54375231895778242, 485.7448905765656377, 14.14213562373094568 ) ) ;
#17075=CARTESIAN_POINT ( 'NONE',  ( -48.68588794268887199, 387.5573905601784190, 3.978247347592742678 ) ) ;
#17076=CARTESIAN_POINT ( 'NONE',  ( -35.09675569278793006, 243.4948905683720284, -15.47720386886985544 ) ) ;
#17077=CARTESIAN_POINT ( 'NONE',  ( -13.20868407381887621, 509.7448905683720000, 6.410867750099229490 ) ) ;
#17078=CARTESIAN_POINT ( 'NONE',  ( -11.73070664223724791, 376.0573905765655809, 11.32908994701042005 ) ) ;
#17079=CARTESIAN_POINT ( 'NONE',  ( -40.53162694259542320, 252.6198905683720284, -11.84573899990672707 ) ) ;
#17081=CARTESIAN_POINT ( 'NONE',  ( -25.35362745456399125, 352.5573905683720568, -16.75240474999999307 ) ) ;
#17084=CARTESIAN_POINT ( 'NONE',  ( -44.16309181155857289, 394.4948905683720000, 6.410867750099241924 ) ) ;
#17087=CARTESIAN_POINT ( 'NONE',  ( -36.33955658999051508, 405.3698905601785327, -18.47759065022572855 ) ) ;
#17091=VERTEX_POINT ( 'NONE', #12234 ) ;
#17092=CARTESIAN_POINT ( 'NONE',  ( -35.09675569278797269, 517.2448905683719431, 15.47720386886985366 ) ) ;
#17093=CARTESIAN_POINT ( 'NONE',  ( -48.68588794268870146, 287.2448905601784759, 0.000000000000000000 ) ) ;
#17095=VERTEX_POINT ( 'NONE', #10591 ) ;
#17097=CARTESIAN_POINT ( 'NONE',  ( -14.48388495494899608, 331.3073905683720000, -9.489475012073734561 ) ) ;
#17099=CARTESIAN_POINT ( 'NONE',  ( -40.53162694259543741, 345.1198905683720568, 11.84573899990672885 ) ) ;
#17100=CARTESIAN_POINT ( 'NONE',  ( -38.17536295476244845, 365.4323905683720568, 14.20200298773971781 ) ) ;
#17101=CARTESIAN_POINT ( 'NONE',  ( -32.66413529028186957, 284.1823905765655809, 19.99999999999999289 ) ) ;
#17103=CARTESIAN_POINT ( 'NONE',  ( -42.88789093042841927, 264.8073905683721136, 9.489475012073734561 ) ) ;
#17104=CARTESIAN_POINT ( 'NONE',  ( -48.68588794268869435, 227.2448905601785043, 0.000000000000000000 ) ) ;
#17105=CARTESIAN_POINT ( 'NONE',  ( -45.43829269268871229, 425.0573905683720568, -3.332260488124726194 ) ) ;
#17109=CARTESIAN_POINT ( 'NONE',  ( -8.685887942688731655, 446.9948905765655809, -2.449293598294705724E-15 ) ) ;
#17111=CARTESIAN_POINT ( 'NONE',  ( -16.84014894278198682, 321.6198905683720568, -11.84573899990672707 ) ) ;
#17112=CARTESIAN_POINT ( 'NONE',  ( -16.84014894278200103, 460.1198905683720568, -11.84573899990672707 ) ) ;
#17114=CARTESIAN_POINT ( 'NONE',  ( -21.03221929538693757, 474.1198905601784759, -18.47759065022572855 ) ) ;
#17115=CARTESIAN_POINT ( 'NONE',  ( -42.88789093042842637, 284.8073905683720568, 9.489475012073736337 ) ) ;
#17117=CARTESIAN_POINT ( 'NONE',  ( -42.82802356641965957, 338.4948905601785327, 14.14213562373094923 ) ) ;
#17118=CARTESIAN_POINT ( 'NONE',  ( -14.48388495494901029, 441.3073905683721136, -9.489475012073734561 ) ) ;
#17120=FACE_OUTER_BOUND ( 'NONE', #20668, .T. ) ;
#17121=CARTESIAN_POINT ( 'NONE',  ( -32.01814843081344009, 291.6823905683720568, -16.75240474999999307 ) ) ;
#17123=CARTESIAN_POINT ( 'NONE',  ( -40.53162694259543741, 374.1198905683720000, -11.84573899990672707 ) ) ;
#17124=DIRECTION ( 'NONE',  ( -1.191790137725560488E-16, 1.000000000000000000, -0.000000000000000000 ) ) ;
#17125=CARTESIAN_POINT ( 'NONE',  ( -28.68588794268873698, 519.4948905765655809, -19.99999999999999289 ) ) ;
#17126=CARTESIAN_POINT ( 'NONE',  ( -16.84014894278199037, 397.6198905683720568, 11.84573899990672530 ) ) ;
#17127=CARTESIAN_POINT ( 'NONE',  ( -35.09675569278793716, 247.2448905683720000, 15.47720386886985366 ) ) ;
#17128=CARTESIAN_POINT ( 'NONE',  ( -19.19641293061498644, 427.3073905683720568, 14.20200298773971426 ) ) ;
#17130=CARTESIAN_POINT ( 'NONE',  ( -45.64106924314018698, 351.0573905765656377, -11.32908994701042715 ) ) ;
#17131=CARTESIAN_POINT ( 'NONE',  ( -48.68588794268870146, 277.2448905601784759, 0.000000000000000000 ) ) ;
#17132=CARTESIAN_POINT ( 'NONE',  ( -16.84014894278198327, 317.6198905683720568, 11.84573899990672530 ) ) ;
#17133=CARTESIAN_POINT ( 'NONE',  ( -42.88789093042844769, 474.4323905683721136, -9.489475012073736337 ) ) ;
#17137=CARTESIAN_POINT ( 'NONE',  ( -32.39665892562713623, 224.2034014279912526, 19.99999999999999289 ) ) ;
#17138=CARTESIAN_POINT ( 'NONE',  ( -45.43829269268871229, 395.6823905683719431, 3.332260488124734632 ) ) ;
#17140=CARTESIAN_POINT ( 'NONE',  ( -40.01497788969916058, 525.6823905601785327, -16.95518130045146421 ) ) ;
#17141=CARTESIAN_POINT ( 'NONE',  ( -44.16309181155857289, 343.2448905683720000, -6.410867750099231266 ) ) ;
#17143=CARTESIAN_POINT ( 'NONE',  ( -13.20868407381887621, 498.2448905683720000, 6.410867750099229490 ) ) ;
#17145=CARTESIAN_POINT ( 'NONE',  ( -10.20829729246299244, 417.6198905765656377, -7.653668647301794969 ) ) ;
#17147=CARTESIAN_POINT ( 'NONE',  ( -45.64106924314017277, 291.0573905765656377, -11.32908994701042538 ) ) ;
#17149=CARTESIAN_POINT ( 'NONE',  ( -38.17536295476246266, 455.4323905683720000, 14.20200298773971781 ) ) ;
#17151=CARTESIAN_POINT ( 'NONE',  ( -28.68588794268872988, 481.3698905683720568, -16.75240474999999307 ) ) ;
#17152=CARTESIAN_POINT ( 'NONE',  ( -40.01497788969911795, 243.5573905765656377, 16.95518130045146776 ) ) ;
#17153=CARTESIAN_POINT ( 'NONE',  ( -28.68588794268871922, 404.4948905765656377, 19.99999999999999289 ) ) ;
#17159=CARTESIAN_POINT ( 'NONE',  ( -21.03221929538691271, 258.8698905765656377, -18.47759065022572855 ) ) ;
#17162=CARTESIAN_POINT ( 'NONE',  ( -13.20868407381884957, 270.9948905683720000, -6.410867750099233042 ) ) ;
#17164=CARTESIAN_POINT ( 'NONE',  ( -28.68588794268870146, 254.7448905601784475, -19.99999999999999289 ) ) ;
#17166=CARTESIAN_POINT ( 'NONE',  ( -48.68588794268870856, 361.9948905765655809, 0.000000000000000000 ) ) ;
#17167=CARTESIAN_POINT ( 'NONE',  ( -25.35362745456399125, 438.1823905683720000, 16.75240474999998952 ) ) ;
#17169=( BOUNDED_CURVE ( )  B_SPLINE_CURVE ( 2, ( #1455, #6624, #8569, #8243, #5118, #15088, #11823, #15191, #14979, #1673, #13245, #11500, #18418, #11609, #11718, #6947, #13569 ),
 .UNSPECIFIED., .F., .T. ) 
 B_SPLINE_CURVE_WITH_KNOTS ( ( 3, 2, 2, 2, 2, 2, 2, 2, 3 ),
 ( 0.4218750000000001665, 0.4238281250000001665, 0.4257812500000001665, 0.4277343750000001665, 0.4296875000000002220, 0.4316406250000002220, 0.4335937500000002220, 0.4355468750000002220, 0.4375000000000002220 ),
 .UNSPECIFIED. ) 
 CURVE ( )  GEOMETRIC_REPRESENTATION_ITEM ( )  RATIONAL_B_SPLINE_CURVE ( ( 0.9999999999999983347, 0.9807852804032320959, 1.000000000000000000, 0.9807852804032304306, 1.000000000000000000, 0.9807852804032304306, 1.000000000000000000, 0.9807852804032304306, 1.000000000000000000, 0.9807852804032304306, 1.000000000000000000, 0.9807852804032304306, 1.000000000000000000, 0.9807852804032304306, 1.000000000000000000, 0.9807852804032282101, 1.000000000000002220 ) ) 
 REPRESENTATION_ITEM ( '' )  );
#17170=CARTESIAN_POINT ( 'NONE',  ( -45.43829269268869808, 275.6823905683720568, 3.332260488124734632 ) ) ;
#17173=CARTESIAN_POINT ( 'NONE',  ( -11.93348319268873681, 490.0573905683720568, 3.332260488124728859 ) ) ;
#17177=CARTESIAN_POINT ( 'NONE',  ( -42.88789093042841927, 244.8073905683720568, 9.489475012073736337 ) ) ;
#17181=CARTESIAN_POINT ( 'NONE',  ( -36.33955658999052218, 480.1198905765656377, -18.47759065022572855 ) ) ;
#17182=CARTESIAN_POINT ( 'NONE',  ( -10.20829729246298001, 307.6198905765656377, -7.653668647301794969 ) ) ;
#17183=CARTESIAN_POINT ( 'NONE',  ( -22.14532378356892295, 223.9102039777116318, -18.39083598434388733 ) ) ;
#17184=CARTESIAN_POINT ( 'NONE',  ( -32.01814843081343298, 227.5573905683720284, 16.75240474999999307 ) ) ;
#17185=CARTESIAN_POINT ( 'NONE',  ( -16.84014894278200458, 519.1198905683720568, 11.84573899990672530 ) ) ;
#17187=CARTESIAN_POINT ( 'NONE',  ( -45.43829269268869808, 243.8698905683720568, 0.000000000000000000 ) ) ;
#17188=CARTESIAN_POINT ( 'NONE',  ( -35.09675569278794427, 343.4948905683720000, -15.47720386886985544 ) ) ;
#17190=LINE ( 'NONE', #2475, #18520 ) ;
#17192=CARTESIAN_POINT ( 'NONE',  ( -45.43829269268871940, 393.8698905683720000, 0.000000000000000000 ) ) ;
#17194=CARTESIAN_POINT ( 'NONE',  ( -28.68588794268871567, 379.7448905601785327, 19.99999999999999289 ) ) ;
#17196=CARTESIAN_POINT ( 'NONE',  ( -48.68588794268870856, 351.9948905765656377, 0.000000000000000000 ) ) ;
#17198=ORIENTED_EDGE ( 'NONE', *, *, #13398, .T. ) ;
#17199=CARTESIAN_POINT ( 'NONE',  ( -25.35362745456399836, 508.1823905683720568, 16.75240474999998952 ) ) ;
#17200=CARTESIAN_POINT ( 'NONE',  ( -48.68588794268870146, 311.9948905765655809, 0.000000000000000000 ) ) ;
#17202=CARTESIAN_POINT ( 'NONE',  ( -44.16309181155855867, 305.9948905683720568, 6.410867750099241924 ) ) ;
#17204=CARTESIAN_POINT ( 'NONE',  ( -42.88789093042843348, 352.9323905683721136, -9.489475012073736337 ) ) ;
#17205=CARTESIAN_POINT ( 'NONE',  ( -16.84014894278199037, 350.1198905683720568, -11.84573899990672707 ) ) ;
#17206=CARTESIAN_POINT ( 'NONE',  ( -47.16347859291443712, 281.3698905765656377, -7.653668647301793193 ) ) ;
#17207=DIRECTION ( 'NONE',  ( -1.191790137725560488E-16, 1.000000000000000000, -0.000000000000000000 ) ) ;
#17208=CARTESIAN_POINT ( 'NONE',  ( -45.43829269268869808, 253.8698905683720000, 0.000000000000000000 ) ) ;
#17209=CARTESIAN_POINT ( 'NONE',  ( -48.68588794268887909, 462.3073905765656377, 3.978247347592795524 ) ) ;
#17210=CARTESIAN_POINT ( 'NONE',  ( -16.84014894278199392, 391.6198905683720568, -11.84573899990672707 ) ) ;
#17213=CARTESIAN_POINT ( 'NONE',  ( -28.68588794268873698, 548.2448905601784190, 0.000000000000000000 ) ) ;
#17214=CARTESIAN_POINT ( 'NONE',  ( -44.16309181155856578, 304.7448905683720568, -6.410867750099231266 ) ) ;
#17215=CARTESIAN_POINT ( 'NONE',  ( -19.19641293061499354, 467.3073905683721136, 14.20200298773971426 ) ) ;
#17216=ORIENTED_EDGE ( 'NONE', *, *, #7274, .F. ) ;
#17217=CARTESIAN_POINT ( 'NONE',  ( -21.03221929538691981, 460.3698905601784759, 18.47759065022572500 ) ) ;
#17218=CARTESIAN_POINT ( 'NONE',  ( -38.17536295476244845, 282.3073905683720568, -14.20200298773971426 ) ) ;
#17224=CARTESIAN_POINT ( 'NONE',  ( -24.70764059509555821, 344.4323905601784759, -19.99999999999999289 ) ) ;
#17225=CARTESIAN_POINT ( 'NONE',  ( -45.43829269268870519, 303.8698905683720000, 0.000000000000000000 ) ) ;
#17227=CARTESIAN_POINT ( 'NONE',  ( -44.16309181155856578, 385.9948905683720568, 6.410867750099241924 ) ) ;
#17228=CARTESIAN_POINT ( 'NONE',  ( -32.66413529028186957, 375.0573905601784759, -19.99999999999999289 ) ) ;
#17229=CARTESIAN_POINT ( 'NONE',  ( -8.685887942688742314, 517.3073905765655809, -3.978247347593165895 ) ) ;
#17230=CARTESIAN_POINT ( 'NONE',  ( -45.43829269268871229, 413.5573905683720000, -3.332260488124726194 ) ) ;
#17231=CARTESIAN_POINT ( 'NONE',  ( -16.84014894278197616, 241.6198905683720284, -11.84573899990672707 ) ) ;
#17232=CARTESIAN_POINT ( 'NONE',  ( -16.84014894278199392, 407.6198905683720568, 11.84573899990672530 ) ) ;
#17233=CARTESIAN_POINT ( 'NONE',  ( -24.70764059509555821, 339.1823905765656377, -19.99999999999999289 ) ) ;
#17235=CARTESIAN_POINT ( 'NONE',  ( -22.27502019258947996, 300.7448905683720568, -15.47720386886985544 ) ) ;
#17236=CARTESIAN_POINT ( 'NONE',  ( -44.16309181155858710, 474.7448905683720568, -6.410867750099231266 ) ) ;
#17239=CARTESIAN_POINT ( 'NONE',  ( -8.685887942688715668, 302.2448905601784190, -2.449293598294705724E-15 ) ) ;
#17241=CARTESIAN_POINT ( 'NONE',  ( -14.48388495494900496, 391.3073905683720000, -9.489475012073736337 ) ) ;
#17243=CARTESIAN_POINT ( 'NONE',  ( -17.35679799567830983, 520.6823905601785327, 16.95518130045146421 ) ) ;
#17244=CARTESIAN_POINT ( 'NONE',  ( -11.93348319268872260, 349.1823905683720000, -3.332260488124732856 ) ) ;
#17247=CARTESIAN_POINT ( 'NONE',  ( -40.53162694259545873, 512.6198905683720568, -11.84573899990672707 ) ) ;
#17249=CARTESIAN_POINT ( 'NONE',  ( -28.68588794268871922, 379.4948905765656377, -19.99999999999999289 ) ) ;
#17250=CARTESIAN_POINT ( 'NONE',  ( -8.685887942688717445, 316.9948905765655809, -2.449293598294705724E-15 ) ) ;
#17251=EDGE_CURVE ( 'NONE', #16862, #15664, #19252, .T. ) ;
#17252=CARTESIAN_POINT ( 'NONE',  ( -28.68588794268869790, 223.9102039777116602, 0.000000000000000000 ) ) ;
#17253=CARTESIAN_POINT ( 'NONE',  ( -32.66413529028189089, 519.8073905765655809, -19.99999999999999289 ) ) ;
#17254=CARTESIAN_POINT ( 'NONE',  ( -11.93348319268873503, 468.5573905683720000, 3.332260488124728415 ) ) ;
#17256=CARTESIAN_POINT ( 'NONE',  ( -22.27502019258949062, 476.9948905683720000, 15.47720386886985189 ) ) ;
#17257=CARTESIAN_POINT ( 'NONE',  ( -32.66413529028185536, 249.4323905601784759, 19.99999999999999289 ) ) ;
#17258=CARTESIAN_POINT ( 'NONE',  ( -21.03221929538691271, 395.1198905765656377, 18.47759065022572500 ) ) ;
#17262=CYLINDRICAL_SURFACE ( 'NONE', #11133, 19.99999999999999645 ) ;
#17266=CARTESIAN_POINT ( 'NONE',  ( -35.09675569278793716, 283.4948905683720000, -15.47720386886985544 ) ) ;
#17267=CARTESIAN_POINT ( 'NONE',  ( -40.01497788969912506, 245.6823905601784759, -16.95518130045146421 ) ) ;
#17268=CARTESIAN_POINT ( 'NONE',  ( -48.68588794268885067, 402.3073905765656377, 3.978247347592849259 ) ) ;
#17270=CARTESIAN_POINT ( 'NONE',  ( -32.01814843081345430, 443.1823905683720568, -16.75240474999999307 ) ) ;
#17271=CARTESIAN_POINT ( 'NONE',  ( -8.685887942688541585, 327.3073905765655240, -3.978247347592740013 ) ) ;
#17272=CARTESIAN_POINT ( 'NONE',  ( -22.27502019258946575, 268.4948905683720000, 15.47720386886985189 ) ) ;
#17275=CARTESIAN_POINT ( 'NONE',  ( -16.84014894278200103, 489.1198905683720000, 11.84573899990672530 ) ) ;
#17277=CARTESIAN_POINT ( 'NONE',  ( -28.68588794268871567, 364.7448905601784759, -19.99999999999999289 ) ) ;
#17278=CARTESIAN_POINT ( 'NONE',  ( -35.09675569278793006, 241.9948905683720284, -15.47720386886985544 ) ) ;
#17280=ORIENTED_EDGE ( 'NONE', *, *, #20876, .T. ) ;
#17282=CARTESIAN_POINT ( 'NONE',  ( -47.16347859291445843, 471.3698905765656377, -7.653668647301793193 ) ) ;
#17285=CARTESIAN_POINT ( 'NONE',  ( -8.685887942688731655, 452.2448905601784759, -2.449293598294705724E-15 ) ) ;
#17286=CARTESIAN_POINT ( 'NONE',  ( -14.48388495494898187, 229.4323905683720000, 9.489475012073731008 ) ) ;
#17287=CARTESIAN_POINT ( 'NONE',  ( -45.43829269268872650, 525.6823905683719431, 3.332260488124734632 ) ) ;
#17288=CARTESIAN_POINT ( 'NONE',  ( -32.01814843081343298, 241.6823905683720568, -16.75240474999999307 ) ) ;
#17289=CARTESIAN_POINT ( 'NONE',  ( -45.43829269268870519, 345.0573905683720568, -3.332260488124726194 ) ) ;
#17291=CARTESIAN_POINT ( 'NONE',  ( -17.35679799567828496, 320.6823905601784190, 16.95518130045146421 ) ) ;
#17292=CARTESIAN_POINT ( 'NONE',  ( -14.54375231895775933, 305.7448905765656377, 14.14213562373094568 ) ) ;
#17294=ADVANCED_FACE ( 'NONE', ( #19779 ), #1305, .T. ) ;
#17296=CARTESIAN_POINT ( 'NONE',  ( -40.53162694259543741, 375.1198905683720000, 11.84573899990672885 ) ) ;
#17297=CARTESIAN_POINT ( 'NONE',  ( -42.82802356641965957, 388.4948905601784759, 14.14213562373094923 ) ) ;
#17299=ORIENTED_EDGE ( 'NONE', *, *, #20112, .T. ) ;
#17301=CARTESIAN_POINT ( 'NONE',  ( -16.84014894278200458, 509.1198905683720568, 11.84573899990672530 ) ) ;
#17305=CARTESIAN_POINT ( 'NONE',  ( -11.93348319268871371, 300.3698905683720568, -2.051577885510841163E-15 ) ) ;
#17306=ORIENTED_EDGE ( 'NONE', *, *, #18262, .F. ) ;
#17307=CARTESIAN_POINT ( 'NONE',  ( -45.43829269268871229, 353.8698905683720568, 0.000000000000000000 ) ) ;
#17308=CARTESIAN_POINT ( 'NONE',  ( -45.43829269268871229, 344.1823905683719431, 3.332260488124734632 ) ) ;
#17309=( GEOMETRIC_REPRESENTATION_CONTEXT ( 3 ) GLOBAL_UNCERTAINTY_ASSIGNED_CONTEXT ( ( #16554 ) ) GLOBAL_UNIT_ASSIGNED_CONTEXT ( ( #1343, #13129, #11278 ) ) REPRESENTATION_CONTEXT ( 'NONE', 'WORKASPACE' ) );
#17310=CARTESIAN_POINT ( 'NONE',  ( -45.64106924314017988, 282.9323905765656377, 11.32908994701042715 ) ) ;
#17312=CARTESIAN_POINT ( 'NONE',  ( -45.64106924314018698, 396.3073905601784759, -11.32908994701042538 ) ) ;
#17313=CARTESIAN_POINT ( 'NONE',  ( -14.48388495494898542, 239.8073905683720284, -9.489475012073734561 ) ) ;
#17314=CARTESIAN_POINT ( 'NONE',  ( -42.82802356641964536, 205.1437886375728965, 5.000000000000001776 ) ) ;
#17315=CARTESIAN_POINT ( 'NONE',  ( -35.09675569278795848, 397.2448905683720568, 15.47720386886985366 ) ) ;
#17317=CARTESIAN_POINT ( 'NONE',  ( -42.82802356641968089, 503.2448905765656377, 14.14213562373094923 ) ) ;
#17318=CARTESIAN_POINT ( 'NONE',  ( -40.01497788969912506, 245.6823905601784759, -16.95518130045146421 ) ) ;
#17319=CARTESIAN_POINT ( 'NONE',  ( -14.48388495494900674, 447.9323905683720000, 9.489475012073732785 ) ) ;
#17321=CARTESIAN_POINT ( 'NONE',  ( -28.68588794268872633, 454.7448905601784759, -19.99999999999999289 ) ) ;
#17328=CARTESIAN_POINT ( 'NONE',  ( -42.82802356641965247, 328.4948905601784759, 14.14213562373094923 ) ) ;
#17329=CARTESIAN_POINT ( 'NONE',  ( -32.01814843081344009, 296.0573905683720000, 16.75240474999999307 ) ) ;
#17330=CARTESIAN_POINT ( 'NONE',  ( -16.84014894278199037, 361.6198905683720000, -11.84573899990672707 ) ) ;
#17332=CARTESIAN_POINT ( 'NONE',  ( -24.70764059509557242, 524.8073905765655809, 19.99999999999998934 ) ) ;
#17333=CARTESIAN_POINT ( 'NONE',  ( -16.84014894278199748, 410.1198905683720000, -11.84573899990672707 ) ) ;
#17334=CARTESIAN_POINT ( 'NONE',  ( -32.01814843081343298, 243.1823905683720568, -16.75240474999999307 ) ) ;
#17335=CARTESIAN_POINT ( 'NONE',  ( -35.09675569278795848, 405.7448905683720568, 15.47720386886985366 ) ) ;
#17336=CARTESIAN_POINT ( 'NONE',  ( -42.82802356641965957, 343.2448905765656377, 14.14213562373094923 ) ) ;
#17337=CARTESIAN_POINT ( 'NONE',  ( -42.82802356641965247, 325.9948905601784759, -14.14213562373094746 ) ) ;
#17338=CARTESIAN_POINT ( 'NONE',  ( -32.01814843081344009, 311.6823905683720568, -16.75240474999999307 ) ) ;
#17339=CARTESIAN_POINT ( 'NONE',  ( -40.53162694259545162, 456.6198905683720568, 11.84573899990672885 ) ) ;
#17342=FACE_OUTER_BOUND ( 'NONE', #5732, .T. ) ;
#17345=CARTESIAN_POINT ( 'NONE',  ( -13.20868407381886200, 370.9948905683720568, -6.410867750099233042 ) ) ;
#17347=( BOUNDED_CURVE ( )  B_SPLINE_CURVE ( 2, ( #2797, #4414, #5601, #4310, #7323, #17291, #10566, #20428, #8949, #15571, #7650, #4086, #757, #9058, #7212, #10997, #17401 ),
 .UNSPECIFIED., .F., .T. ) 
 B_SPLINE_CURVE_WITH_KNOTS ( ( 3, 2, 2, 2, 2, 2, 2, 2, 3 ),
 ( 0.6718750000000002220, 0.6738281250000002220, 0.6757812500000002220, 0.6777343750000002220, 0.6796875000000002220, 0.6816406250000002220, 0.6835937500000002220, 0.6855468750000002220, 0.6875000000000002220 ),
 .UNSPECIFIED. ) 
 CURVE ( )  GEOMETRIC_REPRESENTATION_ITEM ( )  RATIONAL_B_SPLINE_CURVE ( ( 0.9999999999999977796, 0.9807852804032326510, 1.000000000000000000, 0.9807852804032304306, 1.000000000000000000, 0.9807852804032304306, 1.000000000000000000, 0.9807852804032304306, 1.000000000000000000, 0.9807852804032304306, 1.000000000000000000, 0.9807852804032304306, 1.000000000000000000, 0.9807852804032304306, 1.000000000000000000, 0.9807852804032282101, 1.000000000000002220 ) ) 
 REPRESENTATION_ITEM ( '' )  );
#17348=CARTESIAN_POINT ( 'NONE',  ( -36.33955658999053639, 509.1198905601784759, 18.47759065022572500 ) ) ;
#17349=CARTESIAN_POINT ( 'NONE',  ( -32.01814843081344719, 346.0573905683720568, 16.75240474999999307 ) ) ;
#17351=CARTESIAN_POINT ( 'NONE',  ( -35.09675569278796559, 511.9948905683720000, -15.47720386886985544 ) ) ;
#17355=CARTESIAN_POINT ( 'NONE',  ( -35.09675569278795848, 417.2448905683720568, 15.47720386886985366 ) ) ;
#17358=CARTESIAN_POINT ( 'NONE',  ( -13.20868407381887089, 468.2448905683720568, 6.410867750099229490 ) ) ;
#17361=CARTESIAN_POINT ( 'NONE',  ( -11.93348319268873503, 468.5573905683720000, 3.332260488124728859 ) ) ;
#17364=CARTESIAN_POINT ( 'NONE',  ( -14.54375231895777176, 395.7448905765656377, 14.14213562373094568 ) ) ;
#17365=CARTESIAN_POINT ( 'NONE',  ( -10.20829729246297646, 277.6198905765655809, -7.653668647301794969 ) ) ;
#17368=CARTESIAN_POINT ( 'NONE',  ( -8.685887942688736985, 486.9948905765656377, -2.449293598294705724E-15 ) ) ;
#17370=CARTESIAN_POINT ( 'NONE',  ( -10.20829729246299422, 432.8698905601784759, -7.653668647301794969 ) ) ;
#17373=CARTESIAN_POINT ( 'NONE',  ( -38.17536295476244845, 283.8073905683720568, -14.20200298773971426 ) ) ;
#17375=CARTESIAN_POINT ( 'NONE',  ( -42.82802356641966668, 403.2448905765655809, 14.14213562373094923 ) ) ;
#17376=CARTESIAN_POINT ( 'NONE',  ( -22.27502019258948351, 418.4948905683720000, 15.47720386886985189 ) ) ;
#17378=CARTESIAN_POINT ( 'NONE',  ( -35.09675569278793716, 273.4948905683720000, -15.47720386886985544 ) ) ;
#17380=CARTESIAN_POINT ( 'NONE',  ( -14.54375231895778420, 478.2448905765655809, -14.14213562373094746 ) ) ;
#17382=CARTESIAN_POINT ( 'NONE',  ( -40.53162694259545162, 474.1198905683720568, -11.84573899990672707 ) ) ;
#17383=EDGE_LOOP ( 'NONE', ( #18361, #15449, #1469, #16296 ) ) ;
#17384=FACE_OUTER_BOUND ( 'NONE', #3282, .T. ) ;
#17385=CARTESIAN_POINT ( 'NONE',  ( -28.68588794268870146, 241.3698905683720568, -16.75240474999999307 ) ) ;
#17388=CARTESIAN_POINT ( 'NONE',  ( -45.43829269268873361, 524.1823905683721705, 3.332260488124734632 ) ) ;
#17391=CARTESIAN_POINT ( 'NONE',  ( -45.64106924314020119, 472.9323905765655809, 11.32908994701042715 ) ) ;
#17394=CARTESIAN_POINT ( 'NONE',  ( -36.09149475953510233, 223.9102039777116033, -15.70829946160876034 ) ) ;
#17395=CARTESIAN_POINT ( 'NONE',  ( -48.68588794268873698, 573.2448905601785327, 0.000000000000000000 ) ) ;
#17396=CARTESIAN_POINT ( 'NONE',  ( -14.48388495494901562, 509.4323905683719431, 9.489475012073732785 ) ) ;
#17398=CARTESIAN_POINT ( 'NONE',  ( -19.19641293061496867, 257.3073905683720568, 14.20200298773971426 ) ) ;
#17399=CARTESIAN_POINT ( 'NONE',  ( -22.27502019258947286, 338.4948905683720568, 15.47720386886985189 ) ) ;
#17401=CARTESIAN_POINT ( 'NONE',  ( -48.68588794268870146, 317.2448905601784759, 0.000000000000000000 ) ) ;
#17402=CARTESIAN_POINT ( 'NONE',  ( -36.33955658999050797, 273.8698905765656377, 18.47759065022572500 ) ) ;
#17404=CARTESIAN_POINT ( 'NONE',  ( -14.48388495494900496, 389.8073905683721136, -9.489475012073736337 ) ) ;
#17405=CARTESIAN_POINT ( 'NONE',  ( -47.16347859291443712, 322.6198905765655809, 7.653668647301805628 ) ) ;
#17406=CARTESIAN_POINT ( 'NONE',  ( -36.33955658999051508, 395.3698905601785327, -18.47759065022572855 ) ) ;
#17408=CARTESIAN_POINT ( 'NONE',  ( -28.68588794268874054, 573.2448905601785327, 0.000000000000000000 ) ) ;
#17409=ORIENTED_EDGE ( 'NONE', *, *, #15379, .T. ) ;
#17411=CARTESIAN_POINT ( 'NONE',  ( -11.93348319268873858, 500.0573905683720568, 3.332260488124728415 ) ) ;
#17412=FACE_OUTER_BOUND ( 'NONE', #13642, .T. ) ;
#17413=ORIENTED_EDGE ( 'NONE', *, *, #11556, .T. ) ;
#17414=CARTESIAN_POINT ( 'NONE',  ( -14.48388495494899431, 311.3073905683720568, -9.489475012073734561 ) ) ;
#17416=CARTESIAN_POINT ( 'NONE',  ( -44.16309181155856578, 334.4948905683720568, 6.410867750099241924 ) ) ;
#17417=CARTESIAN_POINT ( 'NONE',  ( -35.09675569278795138, 355.7448905683720568, 15.47720386886985366 ) ) ;
#17419=CARTESIAN_POINT ( 'NONE',  ( -32.66413529028186957, 289.8073905765656946, -19.99999999999999289 ) ) ;
#17420=CARTESIAN_POINT ( 'NONE',  ( -28.68588794268874054, 573.2448905601785327, 0.000000000000000000 ) ) ;
#17421=CARTESIAN_POINT ( 'NONE',  ( -25.35362745456397704, 241.0573905683720000, -16.75240474999999307 ) ) ;
#17422=CARTESIAN_POINT ( 'NONE',  ( -16.84014894278199392, 401.6198905683720568, -11.84573899990672707 ) ) ;
#17423=CARTESIAN_POINT ( 'NONE',  ( -28.68588794268874054, 573.2448905601785327, 0.000000000000000000 ) ) ;
#17427=CARTESIAN_POINT ( 'NONE',  ( -35.09675569278795848, 451.9948905683720000, -15.47720386886985544 ) ) ;
#17428=ORIENTED_EDGE ( 'NONE', *, *, #9999, .F. ) ;
#17429=CARTESIAN_POINT ( 'NONE',  ( -42.82802356641966668, 438.4948905601784759, 14.14213562373094923 ) ) ;
#17431=ORIENTED_EDGE ( 'NONE', *, *, #15114, .T. ) ;
#17434=CARTESIAN_POINT ( 'NONE',  ( -11.73070664223724258, 331.3073905601785327, 11.32908994701042005 ) ) ;
#17435=CARTESIAN_POINT ( 'NONE',  ( -28.68588794268871567, 372.8698905683720000, -16.75240474999999307 ) ) ;
#17437=CARTESIAN_POINT ( 'NONE',  ( -40.01497788969916058, 520.4323905765656946, -16.95518130045146421 ) ) ;
#17438=CARTESIAN_POINT ( 'NONE',  ( -14.48388495494900496, 407.9323905683720000, 9.489475012073732785 ) ) ;
#17439=CARTESIAN_POINT ( 'NONE',  ( -14.48388495494898542, 241.3073905683720852, -9.489475012073736337 ) ) ;
#17440=CARTESIAN_POINT ( 'NONE',  ( -14.48388495494900674, 397.9323905683720000, 9.489475012073731008 ) ) ;
#17441=CARTESIAN_POINT ( 'NONE',  ( -8.685887942688719221, 337.3073905765655809, -3.978247347593165895 ) ) ;
#17442=CARTESIAN_POINT ( 'NONE',  ( -13.20868407381885135, 298.2448905683720000, 6.410867750099229490 ) ) ;
#17443=CARTESIAN_POINT ( 'NONE',  ( -38.17536295476246977, 453.8073905683720568, -14.20200298773971426 ) ) ;
#17444=DIRECTION ( 'NONE',  ( -1.191790137725560488E-16, 1.000000000000000000, -0.000000000000000000 ) ) ;
#17447=CARTESIAN_POINT ( 'NONE',  ( -40.53162694259543741, 366.6198905683720000, 11.84573899990672885 ) ) ;
#17448=CARTESIAN_POINT ( 'NONE',  ( -32.01814843081346140, 496.0573905683720568, 16.75240474999999307 ) ) ;
#17449=CARTESIAN_POINT ( 'NONE',  ( -32.66413529028189799, 515.0573905601785327, -19.99999999999999289 ) ) ;
#17450=CARTESIAN_POINT ( 'NONE',  ( -40.53162694259543741, 335.1198905683720568, 11.84573899990672885 ) ) ;
#17452=CARTESIAN_POINT ( 'NONE',  ( -38.17536295476246266, 495.4323905683720000, 14.20200298773971781 ) ) ;
#17455=CARTESIAN_POINT ( 'NONE',  ( -25.35362745456399836, 432.5573905683719431, -16.75240474999999307 ) ) ;
#17457=CARTESIAN_POINT ( 'NONE',  ( -10.20829729246300133, 492.8698905601784759, -7.653668647301794969 ) ) ;
#17458=CARTESIAN_POINT ( 'NONE',  ( -45.43829269268871940, 474.1823905683720000, 3.332260488124734632 ) ) ;
#17460=CARTESIAN_POINT ( 'NONE',  ( -11.93348319268873503, 468.8698905683720000, -2.051577885510841163E-15 ) ) ;
#17461=CARTESIAN_POINT ( 'NONE',  ( -45.64106924314016567, 248.1823905601784759, 11.32908994701042538 ) ) ;
#17462=CARTESIAN_POINT ( 'NONE',  ( -40.01497788969913927, 413.5573905765656946, 16.95518130045146776 ) ) ;
#17464=CARTESIAN_POINT ( 'NONE',  ( -10.20829729246298712, 367.6198905765656377, -7.653668647301794969 ) ) ;
#17465=CARTESIAN_POINT ( 'NONE',  ( -8.685887942688729879, 436.9948905765656377, -2.449293598294705724E-15 ) ) ;
#17469=EDGE_CURVE ( 'NONE', #8749, #17095, #499, .T. ) ;
#17470=CARTESIAN_POINT ( 'NONE',  ( -48.68588794268854514, 346.9323905601784190, -3.978247347593583783 ) ) ;
#17471=( BOUNDED_CURVE ( )  B_SPLINE_CURVE ( 2, ( #2286, #564, #7132, #3897, #15486, #672, #14405, #14187, #4330, #1102, #1204, #3998, #17525, #16023, #10913, #18816, #12443 ),
 .UNSPECIFIED., .F., .T. ) 
 B_SPLINE_CURVE_WITH_KNOTS ( ( 3, 2, 2, 2, 2, 2, 2, 2, 3 ),
 ( 0.6250000000000002220, 0.6269531250000002220, 0.6289062500000002220, 0.6308593750000002220, 0.6328125000000002220, 0.6347656250000002220, 0.6367187500000002220, 0.6386718750000002220, 0.6406250000000002220 ),
 .UNSPECIFIED. ) 
 CURVE ( )  GEOMETRIC_REPRESENTATION_ITEM ( )  RATIONAL_B_SPLINE_CURVE ( ( 0.9999999999999977796, 0.9807852804032326510, 1.000000000000000000, 0.9807852804032304306, 1.000000000000000000, 0.9807852804032304306, 1.000000000000000000, 0.9807852804032304306, 1.000000000000000000, 0.9807852804032304306, 1.000000000000000000, 0.9807852804032304306, 1.000000000000000000, 0.9807852804032304306, 1.000000000000000000, 0.9807852804032282101, 1.000000000000002220 ) ) 
 REPRESENTATION_ITEM ( '' )  );
#17472=CARTESIAN_POINT ( 'NONE',  ( -11.73070664223723547, 243.1823905601784759, -11.32908994701042715 ) ) ;
#17473=CARTESIAN_POINT ( 'NONE',  ( -47.16347859291444422, 362.6198905765656377, 7.653668647301805628 ) ) ;
#17474=CARTESIAN_POINT ( 'NONE',  ( -28.68588794268872277, 432.8698905683720568, -16.75240474999999307 ) ) ;
#17476=CARTESIAN_POINT ( 'NONE',  ( -14.48388495494898542, 251.3073905683720284, -9.489475012073736337 ) ) ;
#17477=ORIENTED_EDGE ( 'NONE', *, *, #14198, .T. ) ;
#17479=CARTESIAN_POINT ( 'NONE',  ( -8.685887942688735208, 476.9948905765656377, -2.449293598294705724E-15 ) ) ;
#17481=CARTESIAN_POINT ( 'NONE',  ( -42.88789093042844769, 486.3073905683720568, 9.489475012073734561 ) ) ;
#17484=CARTESIAN_POINT ( 'NONE',  ( -45.43829269268869098, 243.5573905683720000, -3.332260488124726194 ) ) ;
#17486=CARTESIAN_POINT ( 'NONE',  ( -22.27502019258949773, 526.9948905683720568, 15.47720386886985189 ) ) ;
#17490=CARTESIAN_POINT ( 'NONE',  ( -21.03221929538693757, 468.8698905765656377, -18.47759065022572855 ) ) ;
#17491=CARTESIAN_POINT ( 'NONE',  ( -36.33955658999051508, 349.1198905601784759, 18.47759065022572500 ) ) ;
#17493=CARTESIAN_POINT ( 'NONE',  ( -16.84014894278197616, 231.6198905683720000, -11.84573899990672707 ) ) ;
#17495=CARTESIAN_POINT ( 'NONE',  ( -25.35362745456401257, 522.5573905683720568, -16.75240474999999307 ) ) ;
#17497=CARTESIAN_POINT ( 'NONE',  ( -16.84014894278196905, 227.6198905683720000, 11.84573899990672530 ) ) ;
#17498=CARTESIAN_POINT ( 'NONE',  ( -32.01814843081344719, 347.5573905683720568, 16.75240474999999307 ) ) ;
#17500=CARTESIAN_POINT ( 'NONE',  ( -21.03221929538690205, 305.1198905765656377, 18.47759065022572500 ) ) ;
#17503=CARTESIAN_POINT ( 'NONE',  ( -25.35362745456398414, 376.6823905683720000, 16.75240474999998952 ) ) ;
#17504=CARTESIAN_POINT ( 'NONE',  ( -21.03221929538690560, 325.1198905765655809, 18.47759065022572500 ) ) ;
#17505=CARTESIAN_POINT ( 'NONE',  ( -11.73070664223725146, 391.3073905601784759, 11.32908994701042005 ) ) ;
#17508=CARTESIAN_POINT ( 'NONE',  ( -14.54375231895777532, 403.4948905601784759, -14.14213562373094746 ) ) ;
#17509=ORIENTED_EDGE ( 'NONE', *, *, #115, .F. ) ;
#17511=CARTESIAN_POINT ( 'NONE',  ( -28.68588794268872988, 507.8698905683720568, 16.75240474999999307 ) ) ;
#17515=CARTESIAN_POINT ( 'NONE',  ( -45.43829269268870519, 295.6823905683720000, 3.332260488124734632 ) ) ;
#17517=CARTESIAN_POINT ( 'NONE',  ( -19.19641293061498288, 330.4323905683720000, -14.20200298773971603 ) ) ;
#17518=CARTESIAN_POINT ( 'NONE',  ( -32.01814843081344719, 351.6823905683720000, -16.75240474999999307 ) ) ;
#17520=CARTESIAN_POINT ( 'NONE',  ( -45.64106924314017277, 262.9323905765656377, 11.32908994701042715 ) ) ;
#17522=CARTESIAN_POINT ( 'NONE',  ( -45.43829269268869808, 243.8698905683720568, 0.000000000000000000 ) ) ;
#17523=CARTESIAN_POINT ( 'NONE',  ( -38.17536295476246266, 403.8073905683721136, -14.20200298773971426 ) ) ;
#17525=CARTESIAN_POINT ( 'NONE',  ( -14.54375231895776643, 333.4948905601784759, -14.14213562373094746 ) ) ;
#17528=CARTESIAN_POINT ( 'NONE',  ( -13.20868407381886911, 448.2448905683720000, 6.410867750099229490 ) ) ;
#17529=ORIENTED_EDGE ( 'NONE', *, *, #12715, .F. ) ;
#17530=CARTESIAN_POINT ( 'NONE',  ( -11.73070664223726034, 443.1823905601784759, -11.32908994701042715 ) ) ;
#17536=CARTESIAN_POINT ( 'NONE',  ( -24.70764059509555821, 334.4323905601784759, -19.99999999999999289 ) ) ;
#17538=CARTESIAN_POINT ( 'NONE',  ( -35.09675569278795138, 367.2448905683720000, 15.47720386886985366 ) ) ;
#17540=CARTESIAN_POINT ( 'NONE',  ( -14.54375231895778775, 498.2448905765656377, -14.14213562373094746 ) ) ;
#17541=CARTESIAN_POINT ( 'NONE',  ( -35.09675569278795138, 385.7448905683720000, 15.47720386886985366 ) ) ;
#17542=CARTESIAN_POINT ( 'NONE',  ( -13.20868407381884602, 239.7448905683720000, 6.410867750099229490 ) ) ;
#17544=CARTESIAN_POINT ( 'NONE',  ( -40.53162694259544452, 415.1198905683720000, 11.84573899990672885 ) ) ;
#17546=CARTESIAN_POINT ( 'NONE',  ( -45.64106924314018698, 341.0573905765656946, -11.32908994701042715 ) ) ;
#17548=CARTESIAN_POINT ( 'NONE',  ( -35.09675569278793716, 301.9948905683720568, -15.47720386886985544 ) ) ;
#17549=CARTESIAN_POINT ( 'NONE',  ( -16.84014894278200103, 451.6198905683720568, -11.84573899990672707 ) ) ;
#17553=EDGE_CURVE ( 'NONE', #18972, #4317, #13521, .T. ) ;
#17554=CARTESIAN_POINT ( 'NONE',  ( -19.19641293061498644, 361.9323905683721136, -14.20200298773971603 ) ) ;
#17555=CARTESIAN_POINT ( 'NONE',  ( -42.88789093042845479, 504.8073905683720568, 9.489475012073736337 ) ) ;
#17556=CARTESIAN_POINT ( 'NONE',  ( -42.82802356641967378, 505.9948905601785327, -14.14213562373094746 ) ) ;
#17557=CARTESIAN_POINT ( 'NONE',  ( -22.27502019258947286, 316.9948905683720568, 15.47720386886985189 ) ) ;
#17560=CARTESIAN_POINT ( 'NONE',  ( -44.16309181155857999, 494.4948905683720568, 6.410867750099241924 ) ) ;
#17564=CARTESIAN_POINT ( 'NONE',  ( -13.20868407381886733, 429.7448905683720000, 6.410867750099229490 ) ) ;
#17565=DIRECTION ( 'NONE',  ( -1.191790137725560488E-16, 1.000000000000000000, -0.000000000000000000 ) ) ;
#17566=CARTESIAN_POINT ( 'NONE',  ( -25.35362745456399125, 456.6823905683720000, 16.75240474999998952 ) ) ;
#17568=CARTESIAN_POINT ( 'NONE',  ( -42.88789093042844769, 464.8073905683720000, 9.489475012073734561 ) ) ;
#17569=CARTESIAN_POINT ( 'NONE',  ( -40.01497788969914637, 415.6823905601785327, -16.95518130045146421 ) ) ;
#17571=CARTESIAN_POINT ( 'NONE',  ( -14.54375231895777532, 398.2448905765655809, -14.14213562373094746 ) ) ;
#17576=CARTESIAN_POINT ( 'NONE',  ( -8.685887942688729879, 426.9948905765656377, -2.449293598294705724E-15 ) ) ;
#17577=CARTESIAN_POINT ( 'NONE',  ( -42.82802356641964536, 255.9948905601784759, -14.14213562373094746 ) ) ;
#17578=CARTESIAN_POINT ( 'NONE',  ( -42.29072086064468294, 223.9102039777117170, 12.95568915141013200 ) ) ;
#17580=CARTESIAN_POINT ( 'NONE',  ( -42.82802356641964536, 238.4948905601784759, 14.14213562373094923 ) ) ;
#17581=CARTESIAN_POINT ( 'NONE',  ( -45.64106924314018698, 448.1823905601785327, 11.32908994701042538 ) ) ;
#17582=CARTESIAN_POINT ( 'NONE',  ( -13.20868407381886733, 429.7448905683720000, 6.410867750099229490 ) ) ;
#17583=CARTESIAN_POINT ( 'NONE',  ( -11.73070664223724968, 383.1823905601784190, -11.32908994701042538 ) ) ;
#17584=CARTESIAN_POINT ( 'NONE',  ( -35.09675569278793716, 257.2448905683720000, 15.47720386886985366 ) ) ;
#17586=CARTESIAN_POINT ( 'NONE',  ( -48.68588794268872277, 481.9948905765656377, 0.000000000000000000 ) ) ;
#17587=ORIENTED_EDGE ( 'NONE', *, *, #7274, .T. ) ;
#17588=CARTESIAN_POINT ( 'NONE',  ( -19.19641293061498999, 458.8073905683720000, 14.20200298773971426 ) ) ;
#17589=CARTESIAN_POINT ( 'NONE',  ( -32.66413529028186247, 234.1823905765656662, 19.99999999999999289 ) ) ;
#17591=CARTESIAN_POINT ( 'NONE',  ( -36.33955658999050797, 365.3698905601784759, -18.47759065022572855 ) ) ;
#17592=CARTESIAN_POINT ( 'NONE',  ( -11.93348319268870839, 249.1823905683720568, -3.332260488124732856 ) ) ;
#17594=CARTESIAN_POINT ( 'NONE',  ( -32.01814843081346140, 516.0573905683720568, 16.75240474999999307 ) ) ;
#17597=CARTESIAN_POINT ( 'NONE',  ( -40.01497788969914637, 463.5573905765656377, 16.95518130045146776 ) ) ;
#17599=CARTESIAN_POINT ( 'NONE',  ( -11.73070664223723725, 286.0573905765655809, 11.32908994701042005 ) ) ;
#17600=CARTESIAN_POINT ( 'NONE',  ( -37.18636649280855977, 223.9102039777115465, -14.87251219269597335 ) ) ;
#17601=CARTESIAN_POINT ( 'NONE',  ( -42.88789093042841927, 224.4323905683720000, -9.489475012073734561 ) ) ;
#17602=( BOUNDED_CURVE ( )  B_SPLINE_CURVE ( 2, ( #18870, #943, #19096, #7185, #726, #5465, #7296, #838, #4059, #13920, #5679, #12388, #10864, #18982, #10756, #7510, #2553 ),
 .UNSPECIFIED., .F., .T. ) 
 B_SPLINE_CURVE_WITH_KNOTS ( ( 3, 2, 2, 2, 2, 2, 2, 2, 3 ),
 ( 0.9218750000000001110, 0.9238281250000001110, 0.9257812500000001110, 0.9277343750000001110, 0.9296875000000001110, 0.9316406250000001110, 0.9335937500000001110, 0.9355468750000001110, 0.9375000000000001110 ),
 .UNSPECIFIED. ) 
 CURVE ( )  GEOMETRIC_REPRESENTATION_ITEM ( )  RATIONAL_B_SPLINE_CURVE ( ( 0.9999999999999988898, 0.9807852804032315408, 1.000000000000000000, 0.9807852804032304306, 1.000000000000000000, 0.9807852804032304306, 1.000000000000000000, 0.9807852804032304306, 1.000000000000000000, 0.9807852804032304306, 1.000000000000000000, 0.9807852804032304306, 1.000000000000000000, 0.9807852804032304306, 1.000000000000000000, 0.9807852804032293204, 1.000000000000001110 ) ) 
 REPRESENTATION_ITEM ( '' )  );
#17603=CARTESIAN_POINT ( 'NONE',  ( -20.13121767714597610, 223.9102039777117739, 18.15005032320406642 ) ) ;
#17604=CARTESIAN_POINT ( 'NONE',  ( -13.20868407381884602, 229.4948905683720284, -6.410867750099233042 ) ) ;
#17605=CARTESIAN_POINT ( 'NONE',  ( -25.35362745456397704, 328.1823905683720568, 16.75240474999998952 ) ) ;
#17606=CARTESIAN_POINT ( 'NONE',  ( -32.66413529028188378, 469.4323905601784759, 19.99999999999999289 ) ) ;
#17608=CARTESIAN_POINT ( 'NONE',  ( -45.43829269268869808, 305.0573905683720000, -3.332260488124726194 ) ) ;
#17610=EDGE_CURVE ( 'NONE', #2934, #14145, #10140, .T. ) ;
#17611=CARTESIAN_POINT ( 'NONE',  ( -19.19641293061498999, 380.4323905683720568, -14.20200298773971603 ) ) ;
#17612=CARTESIAN_POINT ( 'NONE',  ( -16.84014894278201169, 521.6198905683719431, -11.84573899990672707 ) ) ;
#17613=CARTESIAN_POINT ( 'NONE',  ( -17.35679799567830273, 393.8073905601785896, -16.95518130045146421 ) ) ;
#17617=CARTESIAN_POINT ( 'NONE',  ( -40.53162694259545162, 496.6198905683720000, 11.84573899990672885 ) ) ;
#17619=DIRECTION ( 'NONE',  ( -1.000000000000000000, 0.000000000000000000, 0.000000000000000000 ) ) ;
#17620=ORIENTED_EDGE ( 'NONE', *, *, #17553, .T. ) ;
#17621=CARTESIAN_POINT ( 'NONE',  ( -28.68588794268870501, 297.8698905683720000, 16.75240474999999307 ) ) ;
#17622=CARTESIAN_POINT ( 'NONE',  ( -40.53162694259543031, 322.6198905683720568, -11.84573899990672707 ) ) ;
#17623=EDGE_CURVE ( 'NONE', #368, #19523, #7671, .T. ) ;
#17624=CARTESIAN_POINT ( 'NONE',  ( -8.685887942688712116, 266.9948905765656377, -2.449293598294705724E-15 ) ) ;
#17627=CARTESIAN_POINT ( 'NONE',  ( -28.68588794268871922, 392.8698905683720000, -16.75240474999999307 ) ) ;
#17628=DIRECTION ( 'NONE',  ( -1.191790137725560488E-16, 1.000000000000000000, -0.000000000000000000 ) ) ;
#17632=CARTESIAN_POINT ( 'NONE',  ( -11.73070664223726745, 507.9323905765655809, -11.32908994701042538 ) ) ;
#17633=EDGE_CURVE ( 'NONE', #13900, #18327, #17347, .T. ) ;
#17634=CARTESIAN_POINT ( 'NONE',  ( -45.43829269268871229, 434.1823905683720568, 3.332260488124734632 ) ) ;
#17636=CARTESIAN_POINT ( 'NONE',  ( -11.73070664223725501, 441.3073905601784759, 11.32908994701042005 ) ) ;
#17641=CARTESIAN_POINT ( 'NONE',  ( -17.35679799567829562, 323.8073905601784190, -16.95518130045146421 ) ) ;
#17642=CARTESIAN_POINT ( 'NONE',  ( -45.42716650061694139, 223.9102039777116886, -0.8991096741133857151 ) ) ;
#17643=CARTESIAN_POINT ( 'NONE',  ( -45.43829269268871229, 355.3698905683720568, 0.000000000000000000 ) ) ;
#17647=CARTESIAN_POINT ( 'NONE',  ( -17.35679799567830983, 505.4323905765656377, 16.95518130045146421 ) ) ;
#17648=CARTESIAN_POINT ( 'NONE',  ( -19.19641293061498999, 380.4323905683720568, -14.20200298773971603 ) ) ;
#17650=CARTESIAN_POINT ( 'NONE',  ( -19.19641293061498288, 397.3073905683720000, 14.20200298773971426 ) ) ;
#17651=CARTESIAN_POINT ( 'NONE',  ( -21.03221929538691981, 328.8698905765656377, -18.47759065022572855 ) ) ;
#17653=CARTESIAN_POINT ( 'NONE',  ( -42.88789093042842637, 304.8073905683720000, 9.489475012073734561 ) ) ;
#17654=CARTESIAN_POINT ( 'NONE',  ( -22.27502019258948707, 448.4948905683720568, 15.47720386886985189 ) ) ;
#17657=CARTESIAN_POINT ( 'NONE',  ( -21.03221929538690915, 370.3698905601784759, 18.47759065022572500 ) ) ;
#17660=CARTESIAN_POINT ( 'NONE',  ( -11.93348319268872260, 370.6823905683719431, -3.332260488124732856 ) ) ;
#17661=CARTESIAN_POINT ( 'NONE',  ( -19.19641293061499709, 507.3073905683720568, 14.20200298773971426 ) ) ;
#17662=CARTESIAN_POINT ( 'NONE',  ( -48.68588794268872277, 497.2448905601785327, 0.000000000000000000 ) ) ;
#17663=CARTESIAN_POINT ( 'NONE',  ( -38.17536295476244845, 322.3073905683720568, -14.20200298773971426 ) ) ;
#17668=CARTESIAN_POINT ( 'NONE',  ( -42.88789093042844058, 416.3073905683720568, 9.489475012073734561 ) ) ;
#17670=CARTESIAN_POINT ( 'NONE',  ( -16.84014894278199748, 437.6198905683720000, 11.84573899990672530 ) ) ;
#17672=CARTESIAN_POINT ( 'NONE',  ( -44.16309181155858710, 463.2448905683720568, -6.410867750099231266 ) ) ;
#17674=EDGE_CURVE ( 'NONE', #17091, #14922, #17190, .T. ) ;
#17675=CARTESIAN_POINT ( 'NONE',  ( -45.64106924314019409, 391.0573905765655809, -11.32908994701042715 ) ) ;
#17686=CARTESIAN_POINT ( 'NONE',  ( -42.54924018682451958, 223.9102039777117454, 12.58112014037532411 ) ) ;
#17687=CARTESIAN_POINT ( 'NONE',  ( -25.35362745456399836, 422.5573905683721136, -16.75240474999999307 ) ) ;
#17688=CARTESIAN_POINT ( 'NONE',  ( -8.685887942688724550, 382.2448905601784759, -2.449293598294705724E-15 ) ) ;
#17689=CARTESIAN_POINT ( 'NONE',  ( -32.01814843081343298, 243.1823905683720568, -16.75240474999999307 ) ) ;
#17693=ORIENTED_EDGE ( 'NONE', *, *, #4299, .T. ) ;
#17694=CARTESIAN_POINT ( 'NONE',  ( -13.20868407381887089, 459.7448905683720568, 6.410867750099229490 ) ) ;
#17695=CARTESIAN_POINT ( 'NONE',  ( -32.66413529028186247, 229.8073905765656377, -19.99999999999999289 ) ) ;
#17698=CARTESIAN_POINT ( 'NONE',  ( -45.43829269268869098, 223.5573905683720284, -3.332260488124726194 ) ) ;
#17699=EDGE_LOOP ( 'NONE', ( #20433, #17587, #10255, #17778 ) ) ;
#17700=CARTESIAN_POINT ( 'NONE',  ( -38.17536295476246977, 525.4323905683720568, 14.20200298773971781 ) ) ;
#17702=CARTESIAN_POINT ( 'NONE',  ( -24.70764059509556176, 454.8073905765655809, 19.99999999999998934 ) ) ;
#17705=CARTESIAN_POINT ( 'NONE',  ( -45.64106924314016567, 241.0573905765656093, -11.32908994701042538 ) ) ;
#17706=CARTESIAN_POINT ( 'NONE',  ( -21.03221929538690205, 290.3698905601784759, 18.47759065022572500 ) ) ;
#17708=CARTESIAN_POINT ( 'NONE',  ( -18.68939845611674144, 223.9102039777117170, 17.39761213591845390 ) ) ;
#17709=CARTESIAN_POINT ( 'NONE',  ( -44.16309181155855867, 223.2448905683720568, -6.410867750099231266 ) ) ;
#17710=CARTESIAN_POINT ( 'NONE',  ( -16.84014894278198327, 311.6198905683720000, -11.84573899990672707 ) ) ;
#17711=CARTESIAN_POINT ( 'NONE',  ( -47.16347859291445133, 446.6198905601784759, -7.653668647301793193 ) ) ;
#17712=CARTESIAN_POINT ( 'NONE',  ( -42.82802356641965957, 378.4948905601784759, 14.14213562373094923 ) ) ;
#17713=CARTESIAN_POINT ( 'NONE',  ( -11.93348319268871727, 310.0573905683720568, 3.332260488124728415 ) ) ;
#17714=CARTESIAN_POINT ( 'NONE',  ( -13.20868407381886023, 378.2448905683720000, 6.410867750099229490 ) ) ;
#17715=CARTESIAN_POINT ( 'NONE',  ( -11.93348319268874214, 530.6823905683720568, -3.332260488124732856 ) ) ;
#17717=CARTESIAN_POINT ( 'NONE',  ( -10.20829729246298534, 361.6198905601784759, 7.653668647301790529 ) ) ;
#17718=CARTESIAN_POINT ( 'NONE',  ( -8.685887942688594876, 402.5573905601784190, -3.978247347592846594 ) ) ;
#17719=VERTEX_POINT ( 'NONE', #3977 ) ;
#17720=CARTESIAN_POINT ( 'NONE',  ( -38.17536295476246977, 483.8073905683720000, -14.20200298773971426 ) ) ;
#17722=CARTESIAN_POINT ( 'NONE',  ( -14.48388495494899075, 297.9323905683720000, 9.489475012073732785 ) ) ;
#17725=( BOUNDED_CURVE ( )  B_SPLINE_CURVE ( 2, ( #6385, #16359, #8003, #3160, #2948, #3374, #1326, #9527, #19692, #21321, #12787, #19380, #16252, #4667, #19486, #16146, #11584 ),
 .UNSPECIFIED., .F., .T. ) 
 B_SPLINE_CURVE_WITH_KNOTS ( ( 3, 2, 2, 2, 2, 2, 2, 2, 3 ),
 ( 0.3437500000000001110, 0.3457031250000001110, 0.3476562500000001110, 0.3496093750000001110, 0.3515625000000001110, 0.3535156250000001110, 0.3554687500000001110, 0.3574218750000001110, 0.3593750000000001110 ),
 .UNSPECIFIED. ) 
 CURVE ( )  GEOMETRIC_REPRESENTATION_ITEM ( )  RATIONAL_B_SPLINE_CURVE ( ( 0.9999999999999988898, 0.9807852804032315408, 1.000000000000000000, 0.9807852804032304306, 1.000000000000000000, 0.9807852804032304306, 1.000000000000000000, 0.9807852804032304306, 1.000000000000000000, 0.9807852804032304306, 1.000000000000000000, 0.9807852804032304306, 1.000000000000000000, 0.9807852804032304306, 1.000000000000000000, 0.9807852804032293204, 1.000000000000001110 ) ) 
 REPRESENTATION_ITEM ( '' )  );
#17726=CARTESIAN_POINT ( 'NONE',  ( -40.53162694259543031, 284.1198905683720000, -11.84573899990672707 ) ) ;
#17727=CARTESIAN_POINT ( 'NONE',  ( -11.93348319268871549, 318.8698905683720000, -2.051577885510841163E-15 ) ) ;
#17729=CARTESIAN_POINT ( 'NONE',  ( -42.82802356641964536, 263.2448905765656377, 14.14213562373094923 ) ) ;
#17730=CARTESIAN_POINT ( 'NONE',  ( -48.68588794268858777, 476.9323905601784759, -3.978247347593477201 ) ) ;
#17731=CARTESIAN_POINT ( 'NONE',  ( -25.35362745456397704, 231.0573905683720568, -16.75240474999999307 ) ) ;
#17733=CARTESIAN_POINT ( 'NONE',  ( -45.43829269268871229, 375.3698905683720568, 0.000000000000000000 ) ) ;
#17737=CARTESIAN_POINT ( 'NONE',  ( -48.68588794268869435, 251.9948905765656093, 0.000000000000000000 ) ) ;
#17738=CARTESIAN_POINT ( 'NONE',  ( -11.93348319268872970, 438.8698905683720568, -2.051577885510841163E-15 ) ) ;
#17740=ORIENTED_EDGE ( 'NONE', *, *, #11864, .T. ) ;
#17741=CARTESIAN_POINT ( 'NONE',  ( -24.70764059509557242, 454.4323905601784759, -19.99999999999999289 ) ) ;
#17743=ORIENTED_EDGE ( 'NONE', *, *, #2411, .F. ) ;
#17747=CARTESIAN_POINT ( 'NONE',  ( -40.01497788969912506, 328.8073905601784759, 16.95518130045146776 ) ) ;
#17750=CARTESIAN_POINT ( 'NONE',  ( -28.68588794268871212, 367.8698905683720000, 16.75240474999999307 ) ) ;
#17752=CARTESIAN_POINT ( 'NONE',  ( -36.33955658999052929, 493.8698905765655809, 18.47759065022572500 ) ) ;
#17753=CARTESIAN_POINT ( 'NONE',  ( -44.16309181155857289, 383.2448905683720000, -6.410867750099231266 ) ) ;
#17754=CARTESIAN_POINT ( 'NONE',  ( -44.16309181155855157, 225.9948905683720284, 6.410867750099241924 ) ) ;
#17755=CARTESIAN_POINT ( 'NONE',  ( -45.43829269268871940, 393.5573905683720000, -3.332260488124726638 ) ) ;
#17757=CARTESIAN_POINT ( 'NONE',  ( -42.82802356641965957, 333.2448905765656377, 14.14213562373094923 ) ) ;
#17759=CARTESIAN_POINT ( 'NONE',  ( -22.27502019258947641, 280.7448905683720568, -15.47720386886985544 ) ) ;
#17760=CARTESIAN_POINT ( 'NONE',  ( -28.68588794268872277, 447.8698905683720000, 16.75240474999999307 ) ) ;
#17761=CYLINDRICAL_SURFACE ( 'NONE', #15812, 19.99999999999999645 ) ;
#17765=CARTESIAN_POINT ( 'NONE',  ( -25.35362745456398059, 348.1823905683720000, 16.75240474999998952 ) ) ;
#17766=CARTESIAN_POINT ( 'NONE',  ( -14.48388495494901562, 507.9323905683720568, 9.489475012073732785 ) ) ;
#17767=CARTESIAN_POINT ( 'NONE',  ( -10.20829729246300310, 511.6198905601785327, 7.653668647301790529 ) ) ;
#17768=CARTESIAN_POINT ( 'NONE',  ( -19.19641293061497933, 317.3073905683720000, 14.20200298773971426 ) ) ;
#17770=ORIENTED_EDGE ( 'NONE', *, *, #21255, .F. ) ;
#17771=CARTESIAN_POINT ( 'NONE',  ( -45.64106924314020119, 526.3073905601785327, -11.32908994701042538 ) ) ;
#17772=ORIENTED_EDGE ( 'NONE', *, *, #13604, .F. ) ;
#17774=CARTESIAN_POINT ( 'NONE',  ( -16.84014894278199392, 429.1198905683720000, 11.84573899990672530 ) ) ;
#17775=CARTESIAN_POINT ( 'NONE',  ( -8.685887942688708563, 236.9948905765656377, -2.449293598294705724E-15 ) ) ;
#17777=CARTESIAN_POINT ( 'NONE',  ( -38.17536295476245556, 435.4323905683720568, 14.20200298773971781 ) ) ;
#17778=ORIENTED_EDGE ( 'NONE', *, *, #7481, .F. ) ;
#17779=CARTESIAN_POINT ( 'NONE',  ( -16.84014894278200458, 470.1198905683720568, -11.84573899990672707 ) ) ;
#17781=CARTESIAN_POINT ( 'NONE',  ( -28.68588794268872277, 414.7448905601784759, -19.99999999999999289 ) ) ;
#17783=CARTESIAN_POINT ( 'NONE',  ( -48.68588794268871567, 391.6823905765655809, -3.978247347593158345 ) ) ;
#17784=DIRECTION ( 'NONE',  ( -1.191790137725560488E-16, 1.000000000000000000, -0.000000000000000000 ) ) ;
#17786=CARTESIAN_POINT ( 'NONE',  ( -47.16347859291445133, 431.3698905765655809, -7.653668647301793193 ) ) ;
#17787=CARTESIAN_POINT ( 'NONE',  ( -48.68588794268869435, 251.9948905765656093, 0.000000000000000000 ) ) ;
#17789=CARTESIAN_POINT ( 'NONE',  ( -47.16347859291443001, 256.6198905601784759, -7.653668647301793193 ) ) ;
#17790=CARTESIAN_POINT ( 'NONE',  ( -21.03221929538691981, 344.1198905601784759, -18.47759065022572855 ) ) ;
#17791=CARTESIAN_POINT ( 'NONE',  ( -25.35362745456398770, 418.1823905683720568, 16.75240474999998952 ) ) ;
#17792=CARTESIAN_POINT ( 'NONE',  ( -8.685887942688720997, 336.9948905765656377, -2.449293598294705724E-15 ) ) ;
#17793=CARTESIAN_POINT ( 'NONE',  ( -14.48388495494898365, 249.4323905683720000, 9.489475012073732785 ) ) ;
#17797=CARTESIAN_POINT ( 'NONE',  ( -8.685887942688729879, 426.9948905765656377, -2.449293598294705724E-15 ) ) ;
#17798=EDGE_LOOP ( 'NONE', ( #19449, #11708, #1315, #18536 ) ) ;
#17799=CARTESIAN_POINT ( 'NONE',  ( -45.43829269268872650, 465.3698905683720000, 0.000000000000000000 ) ) ;
#17800=CARTESIAN_POINT ( 'NONE',  ( -45.64106924314017277, 221.0573905765656093, -11.32908994701042715 ) ) ;
#17801=VERTEX_POINT ( 'NONE', #7753 ) ;
#17803=CARTESIAN_POINT ( 'NONE',  ( -45.43829269268869098, 224.1823905683720284, 3.332260488124734632 ) ) ;
#17805=CARTESIAN_POINT ( 'NONE',  ( -14.48388495494901917, 529.8073905683720568, -9.489475012073734561 ) ) ;
#17806=CARTESIAN_POINT ( 'NONE',  ( -28.68588794268874054, 573.2448905601785327, 0.000000000000000000 ) ) ;
#17807=CARTESIAN_POINT ( 'NONE',  ( -11.73070664223725679, 446.0573905765656377, 11.32908994701042005 ) ) ;
#17810=CARTESIAN_POINT ( 'NONE',  ( -28.68588794268870146, 239.4948905765656377, -19.99999999999999289 ) ) ;
#17815=CARTESIAN_POINT ( 'NONE',  ( -45.43829269268869098, 233.5573905683720568, -3.332260488124726194 ) ) ;
#17816=CARTESIAN_POINT ( 'NONE',  ( -35.09675569278794427, 327.2448905683720000, 15.47720386886985366 ) ) ;
#17818=CARTESIAN_POINT ( 'NONE',  ( -13.20868407381885135, 299.7448905683720568, 6.410867750099229490 ) ) ;
#17819=CARTESIAN_POINT ( 'NONE',  ( -11.93348319268872260, 369.1823905683720000, -3.332260488124732856 ) ) ;
#17820=CARTESIAN_POINT ( 'NONE',  ( -32.01814843081346140, 523.1823905683720568, -16.75240474999999307 ) ) ;
#17821=CARTESIAN_POINT ( 'NONE',  ( -14.54375231895776643, 360.9948905601784759, 14.14213562373094568 ) ) ;
#17822=CARTESIAN_POINT ( 'NONE',  ( -32.66413529028187668, 405.0573905601785327, -19.99999999999999289 ) ) ;
#17824=CARTESIAN_POINT ( 'NONE',  ( -22.27502019258949773, 482.2448905683720568, -15.47720386886985544 ) ) ;
#17826=CARTESIAN_POINT ( 'NONE',  ( -44.16309181155855867, 284.4948905683720000, 6.410867750099241924 ) ) ;
#17827=ORIENTED_EDGE ( 'NONE', *, *, #13398, .F. ) ;
#17828=CARTESIAN_POINT ( 'NONE',  ( -25.35362745456398414, 292.5573905683720568, -16.75240474999999307 ) ) ;
#17829=CARTESIAN_POINT ( 'NONE',  ( -38.17536295476244135, 315.4323905683720000, 14.20200298773971781 ) ) ;
#17830=CARTESIAN_POINT ( 'NONE',  ( -21.03221929538691271, 258.8698905765656377, -18.47759065022572855 ) ) ;
#17832=CARTESIAN_POINT ( 'NONE',  ( -35.09675569278793716, 235.7448905683720000, 15.47720386886985366 ) ) ;
#17833=CARTESIAN_POINT ( 'NONE',  ( -24.70764059509554045, 224.4323905601785043, -19.99999999999999289 ) ) ;
#17834=CARTESIAN_POINT ( 'NONE',  ( -45.43829269268870519, 385.0573905683720000, -3.332260488124726194 ) ) ;
#17837=LINE ( 'NONE', #16342, #12894 ) ;
#17838=CARTESIAN_POINT ( 'NONE',  ( -14.48388495494900496, 417.9323905683720568, 9.489475012073732785 ) ) ;
#17841=CARTESIAN_POINT ( 'NONE',  ( -45.64106924314019409, 418.1823905601784759, 11.32908994701042715 ) ) ;
#17843=ORIENTED_EDGE ( 'NONE', *, *, #9944, .T. ) ;
#17846=CARTESIAN_POINT ( 'NONE',  ( -42.82802356641965247, 315.9948905601784759, -14.14213562373094746 ) ) ;
#17847=DIRECTION ( 'NONE',  ( -1.000000000000000000, 0.000000000000000000, 0.000000000000000000 ) ) ;
#17848=CARTESIAN_POINT ( 'NONE',  ( -19.19641293061497933, 348.8073905683720000, 14.20200298773971426 ) ) ;
#17849=VECTOR ( 'NONE', #20171, 1000.000000000000000 ) ;
#17850=ADVANCED_FACE ( 'NONE', ( #14804, #14589 ), #21387, .F. ) ;
#17851=CARTESIAN_POINT ( 'NONE',  ( -8.685887942688740537, 496.6823905765656377, 3.978247347593161010 ) ) ;
#17852=CARTESIAN_POINT ( 'NONE',  ( -28.68588794268871567, 376.3698905683720568, 16.75240474999999307 ) ) ;
#17853=CARTESIAN_POINT ( 'NONE',  ( -38.17536295476243424, 226.9323905683720000, 14.20200298773971781 ) ) ;
#17854=CARTESIAN_POINT ( 'NONE',  ( -11.93348319268872437, 389.1823905683720568, -3.332260488124732856 ) ) ;
#17855=VECTOR ( 'NONE', #17444, 1000.000000000000000 ) ;
#17856=CARTESIAN_POINT ( 'NONE',  ( -14.54375231895776110, 315.7448905765656377, 14.14213562373094568 ) ) ;
#17858=CARTESIAN_POINT ( 'NONE',  ( -28.68588794268870146, 286.3698905683720568, 16.75240474999999307 ) ) ;
#17859=CARTESIAN_POINT ( 'NONE',  ( -32.01814843081345430, 443.1823905683720568, -16.75240474999999307 ) ) ;
#17862=DIRECTION ( 'NONE',  ( -1.191790137725560488E-16, 1.000000000000000000, -0.000000000000000000 ) ) ;
#17864=CARTESIAN_POINT ( 'NONE',  ( -38.17536295476244845, 356.9323905683720000, 14.20200298773971781 ) ) ;
#17865=CARTESIAN_POINT ( 'NONE',  ( -28.68588794268873343, 501.3698905683721136, -16.75240474999999307 ) ) ;
#17866=CARTESIAN_POINT ( 'NONE',  ( -10.20829729246299955, 481.6198905601785327, 7.653668647301790529 ) ) ;
#17867=CARTESIAN_POINT ( 'NONE',  ( -45.43829269268870519, 333.5573905683720568, -3.332260488124726194 ) ) ;
#17869=AXIS2_PLACEMENT_3D ( 'NONE', #11020, #17628, #9404 ) ;
#17870=VERTEX_POINT ( 'NONE', #6344 ) ;
#17873=EDGE_LOOP ( 'NONE', ( #2916, #3655, #7229, #17529, #18694 ) ) ;
#17875=CARTESIAN_POINT ( 'NONE',  ( -11.93348319268872615, 410.0573905683720568, 3.332260488124728859 ) ) ;
#17876=CYLINDRICAL_SURFACE ( 'NONE', #5895, 19.99999999999999645 ) ;
#17877=CARTESIAN_POINT ( 'NONE',  ( -25.35362745456400191, 451.0573905683719431, -16.75240474999999307 ) ) ;
#17878=CARTESIAN_POINT ( 'NONE',  ( -38.17536295476246266, 455.4323905683720568, 14.20200298773971781 ) ) ;
#17881=CARTESIAN_POINT ( 'NONE',  ( -11.73070664223725323, 387.9323905765656377, -11.32908994701042715 ) ) ;
#17882=CARTESIAN_POINT ( 'NONE',  ( -8.685887942688724550, 366.9948905765655809, -2.449293598294705724E-15 ) ) ;
#17883=CARTESIAN_POINT ( 'NONE',  ( -45.64106924314018698, 391.0573905765656377, -11.32908994701042538 ) ) ;
#17885=CARTESIAN_POINT ( 'NONE',  ( -47.16347859291443001, 252.6198905765656377, 7.653668647301805628 ) ) ;
#17886=CARTESIAN_POINT ( 'NONE',  ( -22.27502019258949062, 488.4948905683720568, 15.47720386886985189 ) ) ;
#17887=EDGE_CURVE ( 'NONE', #16993, #16325, #2697, .T. ) ;
#17890=CARTESIAN_POINT ( 'NONE',  ( -28.68588794268871212, 344.7448905601784759, -19.99999999999999289 ) ) ;
#17891=CARTESIAN_POINT ( 'NONE',  ( -13.20868407381886378, 409.7448905683720000, 6.410867750099229490 ) ) ;
#17893=CARTESIAN_POINT ( 'NONE',  ( -28.68588794268870146, 252.8698905683720000, -16.75240474999999307 ) ) ;
#17898=CARTESIAN_POINT ( 'NONE',  ( -16.84014894278200458, 471.6198905683720000, -11.84573899990672707 ) ) ;
#17899=CARTESIAN_POINT ( 'NONE',  ( -10.20829729246297113, 226.3698905765656377, 7.653668647301790529 ) ) ;
#17900=ORIENTED_EDGE ( 'NONE', *, *, #10318, .F. ) ;
#17901=CARTESIAN_POINT ( 'NONE',  ( -42.82802356641968089, 523.2448905765656946, 14.14213562373094923 ) ) ;
#17902=CARTESIAN_POINT ( 'NONE',  ( -42.88789093042845479, 534.4323905683720568, -9.489475012073736337 ) ) ;
#17904=CARTESIAN_POINT ( 'NONE',  ( -28.68588794268873343, 501.3698905683721136, -16.75240474999999307 ) ) ;
#17906=CARTESIAN_POINT ( 'NONE',  ( -48.68588794268871567, 441.6823905765656377, -3.978247347593158345 ) ) ;
#17907=CARTESIAN_POINT ( 'NONE',  ( -36.33955658999050087, 300.1198905765656377, -18.47759065022572855 ) ) ;
#17908=CARTESIAN_POINT ( 'NONE',  ( -22.27502019258947641, 346.9948905683720000, 15.47720386886985189 ) ) ;
#17909=CARTESIAN_POINT ( 'NONE',  ( -8.685887942688886199, 456.6823905765655809, 3.978247347593533600 ) ) ;
#17913=CARTESIAN_POINT ( 'NONE',  ( -23.15340224802397273, 223.9102039777117739, 19.28725776582380647 ) ) ;
#17914=CARTESIAN_POINT ( 'NONE',  ( -42.88789093042841927, 222.9323905683720284, -9.489475012073736337 ) ) ;
#17915=CARTESIAN_POINT ( 'NONE',  ( -11.93348319268871549, 320.3698905683720568, -2.051577885510841163E-15 ) ) ;
#17917=CARTESIAN_POINT ( 'NONE',  ( -36.33955658999050797, 279.1198905601784759, 18.47759065022572500 ) ) ;
#17919=CARTESIAN_POINT ( 'NONE',  ( -28.68588794268870501, 307.8698905683720000, 16.75240474999999307 ) ) ;
#17920=CARTESIAN_POINT ( 'NONE',  ( -42.88789093042845479, 514.4323905683720568, -9.489475012073734561 ) ) ;
#17921=CARTESIAN_POINT ( 'NONE',  ( -32.66413529028187668, 375.0573905601784759, -19.99999999999999289 ) ) ;
#17923=CARTESIAN_POINT ( 'NONE',  ( -21.03221929538690915, 228.8698905765655809, -18.47759065022572855 ) ) ;
#17925=CARTESIAN_POINT ( 'NONE',  ( -13.20868407381887266, 479.7448905683720568, 6.410867750099229490 ) ) ;
#17927=CARTESIAN_POINT ( 'NONE',  ( -40.53162694259543031, 272.6198905683720568, -11.84573899990672707 ) ) ;
#17928=VERTEX_POINT ( 'NONE', #18027 ) ;
#17929=CARTESIAN_POINT ( 'NONE',  ( -16.84014894278197971, 281.6198905683720000, -11.84573899990672707 ) ) ;
#17931=CARTESIAN_POINT ( 'NONE',  ( -14.48388495494899431, 319.8073905683720568, -9.489475012073736337 ) ) ;
#17933=CARTESIAN_POINT ( 'NONE',  ( -32.66413529028186247, 259.8073905765655809, -19.99999999999999289 ) ) ;
#17935=CARTESIAN_POINT ( 'NONE',  ( -38.17536295476244135, 232.3073905683720568, -14.20200298773971426 ) ) ;
#17936=EDGE_CURVE ( 'NONE', #20007, #8266, #8496, .T. ) ;
#17937=CARTESIAN_POINT ( 'NONE',  ( -44.16309181155856578, 375.9948905683720568, 6.410867750099241924 ) ) ;
#17942=CARTESIAN_POINT ( 'NONE',  ( -42.88789093042844058, 422.9323905683720000, -9.489475012073736337 ) ) ;
#17945=CARTESIAN_POINT ( 'NONE',  ( -21.03221929538693047, 434.1198905601784759, -18.47759065022572855 ) ) ;
#17948=ORIENTED_EDGE ( 'NONE', *, *, #7630, .T. ) ;
#17949=ORIENTED_EDGE ( 'NONE', *, *, #4677, .F. ) ;
#17951=CARTESIAN_POINT ( 'NONE',  ( -45.64106924314017988, 298.1823905601784759, 11.32908994701042715 ) ) ;
#17953=CARTESIAN_POINT ( 'NONE',  ( -32.01814843081344719, 353.1823905683720568, -16.75240474999999307 ) ) ;
#17954=CARTESIAN_POINT ( 'NONE',  ( -17.35679799567830983, 495.4323905765656377, 16.95518130045146421 ) ) ;
#17955=CARTESIAN_POINT ( 'NONE',  ( -32.01814843081344719, 381.6823905683719431, -16.75240474999999307 ) ) ;
#17957=CARTESIAN_POINT ( 'NONE',  ( -28.68588794268871567, 376.3698905683720568, 16.75240474999999307 ) ) ;
#17958=CARTESIAN_POINT ( 'NONE',  ( -36.33955658999050797, 330.1198905765655809, -18.47759065022572855 ) ) ;
#17960=CARTESIAN_POINT ( 'NONE',  ( -42.88789093042842637, 282.9323905683720568, -9.489475012073734561 ) ) ;
#17961=CARTESIAN_POINT ( 'NONE',  ( -19.19641293061498999, 438.8073905683720000, 14.20200298773971426 ) ) ;
#17964=( BOUNDED_CURVE ( )  B_SPLINE_CURVE ( 2, ( #8914, #3945, #10530, #5993, #15535, #12381, #9126, #19088, #716, #17257, #7288, #5671, #20711, #17461, #5884, #9236, #14763 ),
 .UNSPECIFIED., .F., .T. ) 
 B_SPLINE_CURVE_WITH_KNOTS ( ( 3, 2, 2, 2, 2, 2, 2, 2, 3 ),
 ( 0.8906250000000002220, 0.8925781250000002220, 0.8945312500000002220, 0.8964843750000002220, 0.8984375000000002220, 0.9003906250000001110, 0.9023437500000001110, 0.9042968750000001110, 0.9062500000000001110 ),
 .UNSPECIFIED. ) 
 CURVE ( )  GEOMETRIC_REPRESENTATION_ITEM ( )  RATIONAL_B_SPLINE_CURVE ( ( 0.9999999999999977796, 0.9807852804032326510, 1.000000000000000000, 0.9807852804032304306, 1.000000000000000000, 0.9807852804032304306, 1.000000000000000000, 0.9807852804032304306, 1.000000000000000000, 0.9807852804032304306, 1.000000000000000000, 0.9807852804032304306, 1.000000000000000000, 0.9807852804032304306, 1.000000000000000000, 0.9807852804032293204, 1.000000000000001110 ) ) 
 REPRESENTATION_ITEM ( '' )  );
#17965=CARTESIAN_POINT ( 'NONE',  ( -40.01497788969913927, 448.8073905601785327, 16.95518130045146776 ) ) ;
#17966=CARTESIAN_POINT ( 'NONE',  ( -16.84014894278198682, 341.6198905683720000, -11.84573899990672707 ) ) ;
#17967=CARTESIAN_POINT ( 'NONE',  ( -40.53162694259545162, 482.6198905683720000, -11.84573899990672707 ) ) ;
#17969=CARTESIAN_POINT ( 'NONE',  ( -36.33955658999052218, 495.3698905601784759, -18.47759065022572855 ) ) ;
#17970=CARTESIAN_POINT ( 'NONE',  ( -11.93348319268871549, 308.8698905683720000, -2.051577885510841163E-15 ) ) ;
#17975=ORIENTED_EDGE ( 'NONE', *, *, #17469, .F. ) ;
#17979=CARTESIAN_POINT ( 'NONE',  ( -28.68588794268872277, 412.8698905683720568, -16.75240474999999307 ) ) ;
#17980=CARTESIAN_POINT ( 'NONE',  ( -17.35679799567827786, 235.4323905765656093, 16.95518130045146421 ) ) ;
#17982=CARTESIAN_POINT ( 'NONE',  ( -22.27502019258949773, 440.7448905683720000, -15.47720386886985544 ) ) ;
#17984=CARTESIAN_POINT ( 'NONE',  ( -44.16309181155857999, 443.2448905683720000, -6.410867750099231266 ) ) ;
#17988=CARTESIAN_POINT ( 'NONE',  ( -42.82802356641965957, 380.7448905765656377, -14.14213562373094746 ) ) ;
#17989=CARTESIAN_POINT ( 'NONE',  ( -48.68588794268870856, 381.9948905765655809, 0.000000000000000000 ) ) ;
#17990=FACE_OUTER_BOUND ( 'NONE', #13441, .T. ) ;
#17991=CARTESIAN_POINT ( 'NONE',  ( -45.64106924314018698, 431.0573905765655809, -11.32908994701042538 ) ) ;
#17993=CARTESIAN_POINT ( 'NONE',  ( -45.43829269268871940, 495.6823905683720568, 3.332260488124734632 ) ) ;
#17994=EDGE_CURVE ( 'NONE', #17870, #4866, #4896, .T. ) ;
#18000=CARTESIAN_POINT ( 'NONE',  ( -28.68588794268871922, 402.8698905683720000, -16.75240474999999307 ) ) ;
#18001=CARTESIAN_POINT ( 'NONE',  ( -17.35679799567830983, 468.5573905765655240, -16.95518130045146421 ) ) ;
#18003=CARTESIAN_POINT ( 'NONE',  ( -28.68588794268869435, 227.8698905683720284, 16.75240474999999307 ) ) ;
#18004=ORIENTED_EDGE ( 'NONE', *, *, #16983, .F. ) ;
#18007=CARTESIAN_POINT ( 'NONE',  ( -19.19641293061499709, 471.9323905683720568, -14.20200298773971603 ) ) ;
#18008=CARTESIAN_POINT ( 'NONE',  ( -47.16347859291443001, 232.6198905765656377, 7.653668647301805628 ) ) ;
#18013=CARTESIAN_POINT ( 'NONE',  ( -28.68588794268869790, 221.3698905683720284, -16.75240474999999307 ) ) ;
#18015=CARTESIAN_POINT ( 'NONE',  ( -45.43829269268872650, 503.8698905683720568, 0.000000000000000000 ) ) ;
#18017=CARTESIAN_POINT ( 'NONE',  ( -8.685887942688729879, 437.3073905765655809, -3.978247347593165895 ) ) ;
#18018=CARTESIAN_POINT ( 'NONE',  ( -28.68588794268870856, 299.4948905765656377, -19.99999999999999289 ) ) ;
#18023=EDGE_CURVE ( 'NONE', #1107, #17719, #308, .T. ) ;
#18025=CARTESIAN_POINT ( 'NONE',  ( -48.68588794268873698, 573.2448905601785327, 0.000000000000000000 ) ) ;
#18026=CARTESIAN_POINT ( 'NONE',  ( -13.20868407381885135, 309.7448905683720568, 6.410867750099229490 ) ) ;
#18027=CARTESIAN_POINT ( 'NONE',  ( -8.685887942688731655, 446.9948905765655809, -2.449293598294705724E-15 ) ) ;
#18028=CARTESIAN_POINT ( 'NONE',  ( -8.685887942688712116, 272.5573905601785327, -3.978247347593165895 ) ) ;
#18029=CARTESIAN_POINT ( 'NONE',  ( -43.68588794268873698, 548.2448905601784190, 0.000000000000000000 ) ) ;
#18031=CARTESIAN_POINT ( 'NONE',  ( -19.19641293061497578, 281.9323905683720568, -14.20200298773971603 ) ) ;
#18032=CARTESIAN_POINT ( 'NONE',  ( -45.43829269268873361, 525.0573905683720568, -3.332260488124726638 ) ) ;
#18033=CARTESIAN_POINT ( 'NONE',  ( -45.64106924314018698, 358.1823905601784759, 11.32908994701042715 ) ) ;
#18035=ORIENTED_EDGE ( 'NONE', *, *, #17994, .F. ) ;
#18036=CARTESIAN_POINT ( 'NONE',  ( -42.88789093042844769, 484.4323905683719431, -9.489475012073736337 ) ) ;
#18038=CARTESIAN_POINT ( 'NONE',  ( -28.68588794268870146, 286.3698905683720568, 16.75240474999999307 ) ) ;
#18040=CARTESIAN_POINT ( 'NONE',  ( -38.17536295476244845, 293.8073905683720000, -14.20200298773971426 ) ) ;
#18041=CARTESIAN_POINT ( 'NONE',  ( -35.09675569278793716, 311.9948905683720568, -15.47720386886985544 ) ) ;
#18043=CARTESIAN_POINT ( 'NONE',  ( -42.88789093042841927, 256.3073905683720568, 9.489475012073734561 ) ) ;
#18045=CARTESIAN_POINT ( 'NONE',  ( -8.685887942688708563, 247.3073905765656377, -3.978247347593165895 ) ) ;
#18047=CARTESIAN_POINT ( 'NONE',  ( -22.27502019258945865, 226.9948905683720284, 15.47720386886985189 ) ) ;
#18048=CARTESIAN_POINT ( 'NONE',  ( -11.93348319268872260, 370.6823905683719431, -3.332260488124732856 ) ) ;
#18051=VECTOR ( 'NONE', #1380, 1000.000000000000000 ) ;
#18053=CARTESIAN_POINT ( 'NONE',  ( -19.19641293061498999, 417.3073905683720568, 14.20200298773971426 ) ) ;
#18054=DIRECTION ( 'NONE',  ( -1.191790137725560488E-16, 1.000000000000000000, -0.000000000000000000 ) ) ;
#18056=CARTESIAN_POINT ( 'NONE',  ( -21.03221929538693047, 424.1198905601784759, -18.47759065022572855 ) ) ;
#18061=CARTESIAN_POINT ( 'NONE',  ( -17.35679799567829207, 313.8073905601784190, -16.95518130045146421 ) ) ;
#18064=CARTESIAN_POINT ( 'NONE',  ( -45.43829269268871229, 335.3698905683720000, 0.000000000000000000 ) ) ;
#18065=CARTESIAN_POINT ( 'NONE',  ( -17.35679799567830628, 475.4323905765655809, 16.95518130045146421 ) ) ;
#18066=CARTESIAN_POINT ( 'NONE',  ( -11.93348319268872260, 359.1823905683720000, -3.332260488124732856 ) ) ;
#18067=CARTESIAN_POINT ( 'NONE',  ( -42.82802356641965247, 310.7448905765656377, -14.14213562373094746 ) ) ;
#18068=CARTESIAN_POINT ( 'NONE',  ( -16.84014894278199037, 387.6198905683720568, 11.84573899990672530 ) ) ;
#18069=CARTESIAN_POINT ( 'NONE',  ( -8.685887942688717445, 316.9948905765655809, -2.449293598294705724E-15 ) ) ;
#18071=CARTESIAN_POINT ( 'NONE',  ( -35.09675569278794427, 295.7448905683720568, 15.47720386886985366 ) ) ;
#18074=CARTESIAN_POINT ( 'NONE',  ( -40.53162694259544452, 434.1198905683720000, -11.84573899990672707 ) ) ;
#18077=CARTESIAN_POINT ( 'NONE',  ( -17.35679799567831338, 513.8073905601785327, -16.95518130045146421 ) ) ;
#18080=VECTOR ( 'NONE', #4476, 1000.000000000000000 ) ;
#18081=CARTESIAN_POINT ( 'NONE',  ( -22.27502019258948351, 342.2448905683720568, -15.47720386886985544 ) ) ;
#18082=CARTESIAN_POINT ( 'NONE',  ( -13.20868407381887444, 488.2448905683720000, 6.410867750099229490 ) ) ;
#18084=VERTEX_POINT ( 'NONE', #523 ) ;
#18085=CARTESIAN_POINT ( 'NONE',  ( -17.35679799567831338, 493.8073905601785327, -16.95518130045146421 ) ) ;
#18086=CARTESIAN_POINT ( 'NONE',  ( -11.93348319268871549, 299.1823905683720000, -3.332260488124732856 ) ) ;
#18090=DIRECTION ( 'NONE',  ( -1.000000000000000000, 0.000000000000000000, 0.000000000000000000 ) ) ;
#18091=CARTESIAN_POINT ( 'NONE',  ( -35.09675569278795138, 413.4948905683720000, -15.47720386886985544 ) ) ;
#18092=CARTESIAN_POINT ( 'NONE',  ( -32.66413529028187668, 444.1823905765656377, 19.99999999999999289 ) ) ;
#18093=DIRECTION ( 'NONE',  ( -1.191790137725560488E-16, 1.000000000000000000, -0.000000000000000000 ) ) ;
#18094=CARTESIAN_POINT ( 'NONE',  ( -40.53162694259544452, 445.1198905683720568, 11.84573899990672885 ) ) ;
#18095=CARTESIAN_POINT ( 'NONE',  ( -42.88789093042844058, 444.8073905683720568, 9.489475012073734561 ) ) ;
#18098=CARTESIAN_POINT ( 'NONE',  ( -8.685887942688724550, 376.9948905765655809, -2.449293598294705724E-15 ) ) ;
#18100=CARTESIAN_POINT ( 'NONE',  ( -45.64106924314016567, 266.3073905601784190, -11.32908994701042538 ) ) ;
#18104=CARTESIAN_POINT ( 'NONE',  ( -35.09675569278796559, 487.2448905683720000, 15.47720386886985366 ) ) ;
#18105=DIRECTION ( 'NONE',  ( -1.000000000000000000, 0.000000000000000000, 0.000000000000000000 ) ) ;
#18106=CARTESIAN_POINT ( 'NONE',  ( -11.73070664223726567, 521.3073905601785327, 11.32908994701042005 ) ) ;
#18107=CARTESIAN_POINT ( 'NONE',  ( -44.16309181155857999, 404.7448905683720568, -6.410867750099231266 ) ) ;
#18109=CARTESIAN_POINT ( 'NONE',  ( -45.43829269268869098, 225.6823905683720568, 3.332260488124734632 ) ) ;
#18111=CARTESIAN_POINT ( 'NONE',  ( -28.68588794268874054, 573.2448905601785327, 0.000000000000000000 ) ) ;
#18113=CARTESIAN_POINT ( 'NONE',  ( -44.16309181155857999, 444.7448905683720000, -6.410867750099231266 ) ) ;
#18114=CARTESIAN_POINT ( 'NONE',  ( -38.17536295476246977, 525.4323905683720568, 14.20200298773971781 ) ) ;
#18117=CARTESIAN_POINT ( 'NONE',  ( -16.84014894278196905, 227.6198905683720000, 11.84573899990672530 ) ) ;
#18118=VERTEX_POINT ( 'NONE', #2661 ) ;
#18120=CARTESIAN_POINT ( 'NONE',  ( -42.88789093042845479, 512.9323905683720568, -9.489475012073734561 ) ) ;
#18122=CARTESIAN_POINT ( 'NONE',  ( -17.35679799567830983, 438.5573905765655809, -16.95518130045146421 ) ) ;
#18124=EDGE_CURVE ( 'NONE', #8857, #8848, #12932, .T. ) ;
#18126=CARTESIAN_POINT ( 'NONE',  ( -36.33955658999052929, 453.8698905765656377, 18.47759065022572500 ) ) ;
#18128=CARTESIAN_POINT ( 'NONE',  ( -17.35679799567828141, 290.6823905601785327, 16.95518130045146421 ) ) ;
#18130=CARTESIAN_POINT ( 'NONE',  ( -17.35679799567830628, 495.4323905765656946, 16.95518130045146421 ) ) ;
#18131=CARTESIAN_POINT ( 'NONE',  ( -42.88789093042842637, 314.4323905683720000, -9.489475012073736337 ) ) ;
#18132=CARTESIAN_POINT ( 'NONE',  ( -40.01497788969912506, 235.6823905601784759, -16.95518130045146421 ) ) ;
#18133=CARTESIAN_POINT ( 'NONE',  ( -24.70764059509553334, 260.0573905601784190, 19.99999999999998934 ) ) ;
#18135=CARTESIAN_POINT ( 'NONE',  ( -28.68588794268870501, 297.8698905683720000, 16.75240474999999307 ) ) ;
#18136=CARTESIAN_POINT ( 'NONE',  ( -25.35362745456399836, 508.1823905683720000, 16.75240474999998952 ) ) ;
#18137=CARTESIAN_POINT ( 'NONE',  ( -36.33955658999050797, 375.3698905601784759, -18.47759065022572855 ) ) ;
#18141=CARTESIAN_POINT ( 'NONE',  ( -38.17536295476246266, 476.9323905683720568, 14.20200298773971781 ) ) ;
#18142=CARTESIAN_POINT ( 'NONE',  ( -40.53162694259543031, 282.6198905683720000, -11.84573899990672707 ) ) ;
#18145=CARTESIAN_POINT ( 'NONE',  ( -14.48388495494899075, 291.3073905683720568, -9.489475012073734561 ) ) ;
#18146=CARTESIAN_POINT ( 'NONE',  ( -36.33955658999049376, 240.1198905765656377, -18.47759065022572855 ) ) ;
#18147=CARTESIAN_POINT ( 'NONE',  ( -21.03221929538693047, 418.8698905765655809, -18.47759065022572855 ) ) ;
#18149=CARTESIAN_POINT ( 'NONE',  ( -35.09675569278793716, 271.9948905683720000, -15.47720386886985544 ) ) ;
#18150=CARTESIAN_POINT ( 'NONE',  ( -35.09675569278794427, 373.4948905683720568, -15.47720386886985544 ) ) ;
#18153=CARTESIAN_POINT ( 'NONE',  ( -11.73070664223726212, 457.9323905765655809, -11.32908994701042538 ) ) ;
#18155=CARTESIAN_POINT ( 'NONE',  ( -28.68588794268870501, 269.4948905765656377, -19.99999999999999289 ) ) ;
#18156=CARTESIAN_POINT ( 'NONE',  ( -19.19641293061498999, 420.4323905683720000, -14.20200298773971603 ) ) ;
#18159=CARTESIAN_POINT ( 'NONE',  ( -10.20829729246299422, 431.6198905601785327, 7.653668647301790529 ) ) ;
#18160=EDGE_CURVE ( 'NONE', #4322, #11378, #19549, .T. ) ;
#18166=CARTESIAN_POINT ( 'NONE',  ( -48.68588794268870146, 296.9323905601784759, -3.978247347593158345 ) ) ;
#18168=CARTESIAN_POINT ( 'NONE',  ( -11.93348319268871904, 350.3698905683720568, -2.051577885510841163E-15 ) ) ;
#18170=CARTESIAN_POINT ( 'NONE',  ( -10.20829729246300133, 486.3698905765655809, 7.653668647301790529 ) ) ;
#18171=CARTESIAN_POINT ( 'NONE',  ( -14.48388495494899963, 367.9323905683720000, 9.489475012073732785 ) ) ;
#18173=CARTESIAN_POINT ( 'NONE',  ( -42.88789093042843348, 384.8073905683720568, 9.489475012073734561 ) ) ;
#18175=CARTESIAN_POINT ( 'NONE',  ( -8.685887942688715668, 296.9948905765655809, -2.449293598294705724E-15 ) ) ;
#18177=CARTESIAN_POINT ( 'NONE',  ( -14.48388495494899075, 289.8073905683719431, -9.489475012073734561 ) ) ;
#18179=CARTESIAN_POINT ( 'NONE',  ( -28.68588794268872633, 442.8698905683720568, -16.75240474999999307 ) ) ;
#18182=CARTESIAN_POINT ( 'NONE',  ( -47.16347859291446554, 516.6198905601784190, -7.653668647301793193 ) ) ;
#18185=CARTESIAN_POINT ( 'NONE',  ( -40.53162694259543741, 346.6198905683720000, 11.84573899990672885 ) ) ;
#18186=CARTESIAN_POINT ( 'NONE',  ( -44.16309181155857999, 474.4948905683720000, 6.410867750099241924 ) ) ;
#18187=EDGE_LOOP ( 'NONE', ( #5340, #13444, #7072, #8452 ) ) ;
#18188=CARTESIAN_POINT ( 'NONE',  ( -47.16347859291445843, 496.6198905601784759, -7.653668647301793193 ) ) ;
#18189=CARTESIAN_POINT ( 'NONE',  ( -38.17536295476244135, 305.4323905683720000, 14.20200298773971781 ) ) ;
#18195=CARTESIAN_POINT ( 'NONE',  ( -44.16309181155857999, 394.7448905683720568, -6.410867750099231266 ) ) ;
#18198=CARTESIAN_POINT ( 'NONE',  ( -19.19641293061498999, 430.4323905683720000, -14.20200298773971603 ) ) ;
#18199=CARTESIAN_POINT ( 'NONE',  ( -35.09675569278795848, 451.9948905683720000, -15.47720386886985544 ) ) ;
#18202=CARTESIAN_POINT ( 'NONE',  ( -21.03221929538692336, 368.8698905765656377, -18.47759065022572855 ) ) ;
#18207=CARTESIAN_POINT ( 'NONE',  ( -32.01814843081346140, 493.1823905683721136, -16.75240474999999307 ) ) ;
#18212=CARTESIAN_POINT ( 'NONE',  ( -24.70764059509556532, 520.0573905601784190, 19.99999999999998934 ) ) ;
#18216=CARTESIAN_POINT ( 'NONE',  ( -32.01814843081345430, 397.5573905683721136, 16.75240474999999307 ) ) ;
#18217=CARTESIAN_POINT ( 'NONE',  ( -45.64106924314016567, 262.9323905765656377, 11.32908994701042538 ) ) ;
#18218=CARTESIAN_POINT ( 'NONE',  ( -25.35362745456396638, 238.1823905683720852, 16.75240474999998952 ) ) ;
#18219=CARTESIAN_POINT ( 'NONE',  ( -22.27502019258948707, 360.7448905683720568, -15.47720386886985544 ) ) ;
#18220=EDGE_LOOP ( 'NONE', ( #13209, #5953, #11677, #295, #20226, #3461, #15393, #1667, #19736, #4835, #2491, #17740, #15919, #19745, #10679, #6615, #746, #15051, #9414, #9256, #1744, #7393, #11139, #14068, #8504, #20307, #15918, #10923, #1060, #10949, #18638, #4979, #1740, #17477, #13743, #10797, #9363, #17413, #12486, #20098, #12980, #4214, #5636, #10556, #18748, #7628, #853, #15495, #11844, #17010, #12917, #20914, #5737, #6212, #16451, #9174, #10134, #20178, #11740, #16724, #76, #12132, #19139, #7969, #737, #7548 ) ) ;
#18221=CARTESIAN_POINT ( 'NONE',  ( -25.35362745456401257, 521.0573905683720568, -16.75240474999999307 ) ) ;
#18222=ORIENTED_EDGE ( 'NONE', *, *, #16505, .T. ) ;
#18223=CARTESIAN_POINT ( 'NONE',  ( -25.35362745456400191, 442.5573905683720568, -16.75240474999999307 ) ) ;
#18224=CARTESIAN_POINT ( 'NONE',  ( -13.20868407381888154, 529.4948905683720568, -6.410867750099233042 ) ) ;
#18227=CARTESIAN_POINT ( 'NONE',  ( -42.82802356641966668, 428.4948905601784759, 14.14213562373094923 ) ) ;
#18228=CARTESIAN_POINT ( 'NONE',  ( -35.09675569278796559, 475.7448905683720568, 15.47720386886985366 ) ) ;
#18230=CARTESIAN_POINT ( 'NONE',  ( -19.19641293061499709, 507.3073905683720568, 14.20200298773971426 ) ) ;
#18232=CARTESIAN_POINT ( 'NONE',  ( -47.16347859291445133, 442.6198905765656377, 7.653668647301805628 ) ) ;
#18233=CARTESIAN_POINT ( 'NONE',  ( -21.03221929538692336, 358.8698905765656377, -18.47759065022572855 ) ) ;
#18234=CARTESIAN_POINT ( 'NONE',  ( -47.16347859291443712, 327.8698905601785327, 7.653668647301805628 ) ) ;
#18235=DIRECTION ( 'NONE',  ( -1.191790137725560488E-16, 1.000000000000000000, -0.000000000000000000 ) ) ;
#18239=CARTESIAN_POINT ( 'NONE',  ( -43.47648769733579854, 200.8087914445877971, -2.512805286998617049 ) ) ;
#18240=CARTESIAN_POINT ( 'NONE',  ( -35.09675569278793716, 303.4948905683720568, -15.47720386886985544 ) ) ;
#18242=CARTESIAN_POINT ( 'NONE',  ( -47.16347859291443001, 267.8698905601784759, 7.653668647301805628 ) ) ;
#18244=CARTESIAN_POINT ( 'NONE',  ( -11.93348319268871194, 290.3698905683720568, -2.051577885510841163E-15 ) ) ;
#18246=CARTESIAN_POINT ( 'NONE',  ( -13.20868407381887799, 510.9948905683721136, -6.410867750099233042 ) ) ;
#18249=CARTESIAN_POINT ( 'NONE',  ( -45.43829269268872650, 465.3698905683720000, 0.000000000000000000 ) ) ;
#18250=CARTESIAN_POINT ( 'NONE',  ( -8.685887942688717445, 316.9948905765655809, -2.449293598294705724E-15 ) ) ;
#18251=CARTESIAN_POINT ( 'NONE',  ( -45.43829269268869098, 264.1823905683720000, 3.332260488124734632 ) ) ;
#18253=DIRECTION ( 'NONE',  ( -1.191790137725560488E-16, 1.000000000000000000, -0.000000000000000000 ) ) ;
#18255=CARTESIAN_POINT ( 'NONE',  ( -44.16309181155855867, 264.7448905683720000, -6.410867750099231266 ) ) ;
#18256=CARTESIAN_POINT ( 'NONE',  ( -32.66413529028186247, 244.1823905765655809, 19.99999999999999289 ) ) ;
#18258=CARTESIAN_POINT ( 'NONE',  ( -14.54375231895775400, 233.4948905601784759, -14.14213562373094746 ) ) ;
#18259=CARTESIAN_POINT ( 'NONE',  ( -24.70764059509554755, 259.1823905765656377, -19.99999999999999289 ) ) ;
#18260=CARTESIAN_POINT ( 'NONE',  ( -22.27502019258946575, 266.9948905683720000, 15.47720386886985189 ) ) ;
#18261=CARTESIAN_POINT ( 'NONE',  ( -16.84014894278199037, 351.6198905683720000, -11.84573899990672707 ) ) ;
#18262=EDGE_CURVE ( 'NONE', #15902, #16993, #9184, .T. ) ;
#18266=CARTESIAN_POINT ( 'NONE',  ( -38.17536295476245556, 425.4323905683720000, 14.20200298773971781 ) ) ;
#18268=CARTESIAN_POINT ( 'NONE',  ( -11.73070664223725323, 421.3073905601784190, 11.32908994701042005 ) ) ;
#18272=EDGE_LOOP ( 'NONE', ( #19313, #12102 ) ) ;
#18273=CARTESIAN_POINT ( 'NONE',  ( -42.88789093042845479, 524.4323905683720568, -9.489475012073736337 ) ) ;
#18274=CARTESIAN_POINT ( 'NONE',  ( -8.685887942688715668, 302.2448905601784190, -2.449293598294705724E-15 ) ) ;
#18277=CARTESIAN_POINT ( 'NONE',  ( -35.09675569278793716, 323.4948905683720000, -15.47720386886985544 ) ) ;
#18278=ORIENTED_EDGE ( 'NONE', *, *, #18866, .F. ) ;
#18279=CARTESIAN_POINT ( 'NONE',  ( -42.82802356641967378, 483.2448905765656377, 14.14213562373094923 ) ) ;
#18280=CARTESIAN_POINT ( 'NONE',  ( -13.20868407381886200, 369.4948905683720568, -6.410867750099233042 ) ) ;
#18281=CARTESIAN_POINT ( 'NONE',  ( -40.53162694259543741, 362.6198905683720000, -11.84573899990672707 ) ) ;
#18282=VECTOR ( 'NONE', #7233, 1000.000000000000000 ) ;
#18283=CARTESIAN_POINT ( 'NONE',  ( -10.20829729246298001, 307.6198905765656377, -7.653668647301794969 ) ) ;
#18285=CARTESIAN_POINT ( 'NONE',  ( -38.17536295476244135, 275.4323905683720568, 14.20200298773971781 ) ) ;
#18286=CARTESIAN_POINT ( 'NONE',  ( -28.68588794268874054, 573.2448905601785327, 0.000000000000000000 ) ) ;
#18287=( BOUNDED_CURVE ( )  B_SPLINE_CURVE ( 2, ( #17196, #12216, #7329, #5389, #15369, #8849, #9065, #13960, #10359, #19024, #13841, #2165, #11995, #8748, #20545, #5711, #5498 ),
 .UNSPECIFIED., .F., .T. ) 
 B_SPLINE_CURVE_WITH_KNOTS ( ( 3, 2, 2, 2, 2, 2, 2, 2, 3 ),
 ( 0.5625000000000001110, 0.5644531250000001110, 0.5664062500000001110, 0.5683593750000001110, 0.5703125000000001110, 0.5722656250000001110, 0.5742187500000001110, 0.5761718750000001110, 0.5781250000000001110 ),
 .UNSPECIFIED. ) 
 CURVE ( )  GEOMETRIC_REPRESENTATION_ITEM ( )  RATIONAL_B_SPLINE_CURVE ( ( 0.9999999999999988898, 0.9807852804032315408, 1.000000000000000000, 0.9807852804032304306, 1.000000000000000000, 0.9807852804032304306, 1.000000000000000000, 0.9807852804032304306, 1.000000000000000000, 0.9807852804032304306, 1.000000000000000000, 0.9807852804032304306, 1.000000000000000000, 0.9807852804032304306, 1.000000000000000000, 0.9807852804032293204, 1.000000000000001110 ) ) 
 REPRESENTATION_ITEM ( '' )  );
#18288=CARTESIAN_POINT ( 'NONE',  ( -42.88789093042844058, 424.4323905683720568, -9.489475012073736337 ) ) ;
#18290=CARTESIAN_POINT ( 'NONE',  ( -8.685887942688742314, 573.2448905601785327, 2.449293598294706119E-15 ) ) ;
#18291=CARTESIAN_POINT ( 'NONE',  ( -40.01497788969916058, 515.6823905601785327, -16.95518130045146421 ) ) ;
#18292=DIRECTION ( 'NONE',  ( -1.191790137725560488E-16, 1.000000000000000000, -0.000000000000000000 ) ) ;
#18294=CARTESIAN_POINT ( 'NONE',  ( -45.43829269268871229, 335.3698905683720000, 0.000000000000000000 ) ) ;
#18295=CARTESIAN_POINT ( 'NONE',  ( -25.35362745456400546, 481.0573905683720568, -16.75240474999999307 ) ) ;
#18296=VERTEX_POINT ( 'NONE', #6606 ) ;
#18297=CARTESIAN_POINT ( 'NONE',  ( -11.73070664223726389, 483.1823905601784759, -11.32908994701042715 ) ) ;
#18298=CARTESIAN_POINT ( 'NONE',  ( -32.01814843081344009, 296.0573905683720000, 16.75240474999999307 ) ) ;
#18303=CARTESIAN_POINT ( 'NONE',  ( -40.53162694259544452, 406.6198905683720568, 11.84573899990672885 ) ) ;
#18304=CARTESIAN_POINT ( 'NONE',  ( -8.685887942688735208, 482.2448905601784759, -2.449293598294705724E-15 ) ) ;
#18305=CARTESIAN_POINT ( 'NONE',  ( -28.68588794268874054, 573.2448905601785327, 0.000000000000000000 ) ) ;
#18306=CARTESIAN_POINT ( 'NONE',  ( -28.68588794268872277, 421.3698905683720568, -16.75240474999999307 ) ) ;
#18307=CARTESIAN_POINT ( 'NONE',  ( -14.48388495494898720, 269.4323905683720568, 9.489475012073732785 ) ) ;
#18308=CARTESIAN_POINT ( 'NONE',  ( -28.68588794268872277, 436.3698905683720000, 16.75240474999999307 ) ) ;
#18311=CARTESIAN_POINT ( 'NONE',  ( -14.54375231895776821, 365.7448905765656377, 14.14213562373094568 ) ) ;
#18312=CARTESIAN_POINT ( 'NONE',  ( -10.20829729246297646, 272.8698905601784759, -7.653668647301794969 ) ) ;
#18313=CARTESIAN_POINT ( 'NONE',  ( -14.54375231895775755, 263.4948905601784759, -14.14213562373094746 ) ) ;
#18314=CARTESIAN_POINT ( 'NONE',  ( -16.84014894278198682, 330.1198905683720568, -11.84573899990672707 ) ) ;
#18316=CARTESIAN_POINT ( 'NONE',  ( -44.16309181155858710, 494.7448905683720000, -6.410867750099231266 ) ) ;
#18321=CARTESIAN_POINT ( 'NONE',  ( -13.20868407381886378, 399.7448905683720568, 6.410867750099229490 ) ) ;
#18323=CARTESIAN_POINT ( 'NONE',  ( -42.88789093042841927, 226.3073905683720000, 9.489475012073736337 ) ) ;
#18324=CARTESIAN_POINT ( 'NONE',  ( -28.68588794268871567, 371.3698905683720568, -16.75240474999999307 ) ) ;
#18326=CARTESIAN_POINT ( 'NONE',  ( -11.93348319268874036, 518.8698905683719431, -2.051577885510841163E-15 ) ) ;
#18327=VERTEX_POINT ( 'NONE', #8115 ) ;
#18328=CARTESIAN_POINT ( 'NONE',  ( -28.68588794268872633, 452.8698905683720000, -16.75240474999999307 ) ) ;
#18329=CARTESIAN_POINT ( 'NONE',  ( -35.09675569278797269, 515.7448905683720568, 15.47720386886985366 ) ) ;
#18332=CARTESIAN_POINT ( 'NONE',  ( -32.66413529028189089, 529.8073905765656946, -19.99999999999999289 ) ) ;
#18333=CARTESIAN_POINT ( 'NONE',  ( -19.19641293061500065, 490.4323905683720000, -14.20200298773971603 ) ) ;
#18336=CARTESIAN_POINT ( 'NONE',  ( -45.43829269268873361, 513.8698905683720568, 0.000000000000000000 ) ) ;
#18337=ADVANCED_FACE ( 'NONE', ( #19205 ), #1157, .T. ) ;
#18338=CARTESIAN_POINT ( 'NONE',  ( -45.64106924314019409, 488.1823905601784759, 11.32908994701042538 ) ) ;
#18340=CARTESIAN_POINT ( 'NONE',  ( -40.01497788969913927, 433.5573905765656377, 16.95518130045146776 ) ) ;
#18342=CARTESIAN_POINT ( 'NONE',  ( -40.01497788969913927, 360.4323905765656946, -16.95518130045146421 ) ) ;
#18348=CARTESIAN_POINT ( 'NONE',  ( -13.30084729135444377, 223.9102039777116886, -12.89731357292796510 ) ) ;
#18349=CARTESIAN_POINT ( 'NONE',  ( -19.19641293061497578, 288.8073905683719431, 14.20200298773971426 ) ) ;
#18351=CARTESIAN_POINT ( 'NONE',  ( -8.685887942689042518, 531.9323905601784190, 3.978247347593879546 ) ) ;
#18352=CARTESIAN_POINT ( 'NONE',  ( -45.64106924314017988, 278.1823905601784759, 11.32908994701042715 ) ) ;
#18353=CARTESIAN_POINT ( 'NONE',  ( -21.03221929538691626, 415.1198905765656377, 18.47759065022572500 ) ) ;
#18354=ORIENTED_EDGE ( 'NONE', *, *, #16903, .F. ) ;
#18355=CARTESIAN_POINT ( 'NONE',  ( -47.16347859291446554, 536.6198905601784190, -7.653668647301793193 ) ) ;
#18356=CARTESIAN_POINT ( 'NONE',  ( -16.84014894278200813, 511.6198905683720000, -11.84573899990672707 ) ) ;
#18358=CARTESIAN_POINT ( 'NONE',  ( -44.16309181155858710, 464.7448905683720568, -6.410867750099231266 ) ) ;
#18359=CARTESIAN_POINT ( 'NONE',  ( -10.20829729246299067, 407.6198905765656377, -7.653668647301794969 ) ) ;
#18360=CARTESIAN_POINT ( 'NONE',  ( -28.68588794268869790, 256.3698905683720000, 16.75240474999999307 ) ) ;
#18361=ORIENTED_EDGE ( 'NONE', *, *, #646, .F. ) ;
#18362=CARTESIAN_POINT ( 'NONE',  ( -11.73070664223724613, 336.0573905765656377, 11.32908994701042005 ) ) ;
#18363=CARTESIAN_POINT ( 'NONE',  ( -16.84014894278197616, 269.1198905683720568, 11.84573899990672530 ) ) ;
#18364=CARTESIAN_POINT ( 'NONE',  ( -44.16309181155855867, 234.7448905683720000, -6.410867750099231266 ) ) ;
#18365=CARTESIAN_POINT ( 'NONE',  ( -48.68588794268869435, 242.3073905765656377, 3.978247347593168115 ) ) ;
#18367=CARTESIAN_POINT ( 'NONE',  ( -48.68588794268869435, 227.5573905601784759, 3.978247347593168115 ) ) ;
#18369=CARTESIAN_POINT ( 'NONE',  ( -11.93348319268871016, 268.8698905683720000, -2.051577885510841163E-15 ) ) ;
#18371=CARTESIAN_POINT ( 'NONE',  ( -45.43829269268870519, 355.6823905683720000, 3.332260488124734632 ) ) ;
#18372=CARTESIAN_POINT ( 'NONE',  ( -45.64106924314017277, 278.1823905601785327, 11.32908994701042538 ) ) ;
#18374=CARTESIAN_POINT ( 'NONE',  ( -19.19641293061498999, 410.4323905683720568, -14.20200298773971603 ) ) ;
#18377=CARTESIAN_POINT ( 'NONE',  ( -40.01497788969913927, 398.8073905601784759, 16.95518130045146776 ) ) ;
#18380=EDGE_LOOP ( 'NONE', ( #20417, #3145 ) ) ;
#18381=CARTESIAN_POINT ( 'NONE',  ( -11.93348319268874214, 530.6823905683721705, -3.332260488124732856 ) ) ;
#18382=CARTESIAN_POINT ( 'NONE',  ( -32.66413529028186957, 295.0573905601784759, -19.99999999999999289 ) ) ;
#18383=CARTESIAN_POINT ( 'NONE',  ( -43.15150032496258348, 208.1972798037766950, -3.972578417695637576 ) ) ;
#18384=VECTOR ( 'NONE', #15676, 1000.000000000000000 ) ;
#18385=CARTESIAN_POINT ( 'NONE',  ( -19.19641293061497578, 328.8073905683720568, 14.20200298773971426 ) ) ;
#18387=CARTESIAN_POINT ( 'NONE',  ( -14.48388495494899786, 357.9323905683720568, 9.489475012073732785 ) ) ;
#18388=CARTESIAN_POINT ( 'NONE',  ( -13.20868407381886023, 359.4948905683720000, -6.410867750099233042 ) ) ;
#18389=CARTESIAN_POINT ( 'NONE',  ( -14.54375231895775933, 295.7448905765656377, 14.14213562373094568 ) ) ;
#18392=CARTESIAN_POINT ( 'NONE',  ( -40.53162694259542320, 265.1198905683720568, 11.84573899990672885 ) ) ;
#18395=CARTESIAN_POINT ( 'NONE',  ( -44.16309181155857999, 414.7448905683720568, -6.410867750099231266 ) ) ;
#18397=CARTESIAN_POINT ( 'NONE',  ( -8.685887942688738761, 512.2448905601784190, -2.449293598294705724E-15 ) ) ;
#18398=CARTESIAN_POINT ( 'NONE',  ( -45.64106924314017988, 358.1823905601784190, 11.32908994701042538 ) ) ;
#18399=DIRECTION ( 'NONE',  ( -1.191790137725560488E-16, 1.000000000000000000, -0.000000000000000000 ) ) ;
#18400=CARTESIAN_POINT ( 'NONE',  ( -19.19641293061497933, 328.8073905683720568, 14.20200298773971426 ) ) ;
#18401=CARTESIAN_POINT ( 'NONE',  ( -11.93348319268873681, 489.1823905683720568, -3.332260488124732856 ) ) ;
#18402=ORIENTED_EDGE ( 'NONE', *, *, #14073, .T. ) ;
#18403=CARTESIAN_POINT ( 'NONE',  ( -42.82802356641967378, 465.9948905601784759, -14.14213562373094746 ) ) ;
#18404=CARTESIAN_POINT ( 'NONE',  ( -25.35362745456398414, 301.0573905683720568, -16.75240474999999307 ) ) ;
#18410=CARTESIAN_POINT ( 'NONE',  ( -28.68588794268871922, 382.8698905683720000, -16.75240474999999307 ) ) ;
#18411=CARTESIAN_POINT ( 'NONE',  ( -48.68588794268871567, 441.9948905765656377, 0.000000000000000000 ) ) ;
#18412=FACE_OUTER_BOUND ( 'NONE', #2187, .T. ) ;
#18413=CARTESIAN_POINT ( 'NONE',  ( -45.43829269268871229, 433.5573905683719431, -3.332260488124726194 ) ) ;
#18414=CARTESIAN_POINT ( 'NONE',  ( -35.09675569278793006, 253.4948905683720568, -15.47720386886985544 ) ) ;
#18415=CARTESIAN_POINT ( 'NONE',  ( -22.27502019258949417, 430.7448905683720000, -15.47720386886985544 ) ) ;
#18417=( BOUNDED_CURVE ( )  B_SPLINE_CURVE ( 2, ( #10064, #8334, #16578, #1542, #14746, #13436, #13002, #4992, #6496, #1655, #6820, #11589, #14957, #29, #1765, #143, #6717 ),
 .UNSPECIFIED., .F., .T. ) 
 B_SPLINE_CURVE_WITH_KNOTS ( ( 3, 2, 2, 2, 2, 2, 2, 2, 3 ),
 ( 0.1093750000000004580, 0.1113281250000004163, 0.1132812500000003747, 0.1152343750000003331, 0.1171875000000002776, 0.1191406250000002359, 0.1210937500000001943, 0.1230468750000001527, 0.1250000000000001110 ),
 .UNSPECIFIED. ) 
 CURVE ( )  GEOMETRIC_REPRESENTATION_ITEM ( )  RATIONAL_B_SPLINE_CURVE ( ( 0.9999999999999954481, 0.9807852804032349825, 1.000000000000000000, 0.9807852804032304306, 1.000000000000000000, 0.9807852804032304306, 1.000000000000000000, 0.9807852804032304306, 1.000000000000000000, 0.9807852804032304306, 1.000000000000000000, 0.9807852804032304306, 1.000000000000000000, 0.9807852804032304306, 1.000000000000000000, 0.9807852804032293204, 1.000000000000001110 ) ) 
 REPRESENTATION_ITEM ( '' )  );
#18418=CARTESIAN_POINT ( 'NONE',  ( -42.82802356641966668, 398.4948905601784759, 14.14213562373094923 ) ) ;
#18419=CARTESIAN_POINT ( 'NONE',  ( -24.70764059509555111, 354.8073905765655809, 19.99999999999998934 ) ) ;
#18420=CARTESIAN_POINT ( 'NONE',  ( -45.64106924314017277, 276.3073905601784759, -11.32908994701042538 ) ) ;
#18421=FACE_OUTER_BOUND ( 'NONE', #4481, .T. ) ;
#18422=CARTESIAN_POINT ( 'NONE',  ( -42.88789093042843348, 334.8073905683720000, 9.489475012073734561 ) ) ;
#18424=CARTESIAN_POINT ( 'NONE',  ( -45.43829269268872650, 475.3698905683720568, 0.000000000000000000 ) ) ;
#18427=LINE ( 'NONE', #13465, #13522 ) ;
#18431=CARTESIAN_POINT ( 'NONE',  ( -11.93348319268872437, 390.6823905683720568, -3.332260488124732856 ) ) ;
#18432=CARTESIAN_POINT ( 'NONE',  ( -45.64106924314019409, 471.0573905765656377, -11.32908994701042538 ) ) ;
#18433=CARTESIAN_POINT ( 'NONE',  ( -47.16347859291446554, 526.6198905601784190, -7.653668647301793193 ) ) ;
#18434=CARTESIAN_POINT ( 'NONE',  ( -16.84014894278198682, 367.6198905683720000, 11.84573899990672530 ) ) ;
#18436=CARTESIAN_POINT ( 'NONE',  ( -28.68588794268873698, 531.3698905683720568, -16.75240474999999307 ) ) ;
#18438=CARTESIAN_POINT ( 'NONE',  ( -38.17536295476245556, 436.9323905683720000, 14.20200298773971781 ) ) ;
#18439=CARTESIAN_POINT ( 'NONE',  ( -11.93348319268874214, 528.8698905683719431, -2.051577885510841163E-15 ) ) ;
#18440=EDGE_CURVE ( 'NONE', #21369, #7041, #19335, .T. ) ;
#18441=VERTEX_POINT ( 'NONE', #11700 ) ;
#18442=CARTESIAN_POINT ( 'NONE',  ( -40.01497788969915348, 495.6823905601784759, -16.95518130045146421 ) ) ;
#18443=CARTESIAN_POINT ( 'NONE',  ( -14.48388495494901385, 487.9323905683719431, 9.489475012073732785 ) ) ;
#18445=CARTESIAN_POINT ( 'NONE',  ( -44.16309181155858710, 493.2448905683720000, -6.410867750099231266 ) ) ;
#18448=CARTESIAN_POINT ( 'NONE',  ( -14.54375231895777532, 425.7448905765656377, 14.14213562373094568 ) ) ;
#18451=CARTESIAN_POINT ( 'NONE',  ( -45.64106924314018698, 441.0573905765656946, -11.32908994701042538 ) ) ;
#18453=CARTESIAN_POINT ( 'NONE',  ( -42.83951137863823533, 204.4886979175576016, -4.967857365464206865 ) ) ;
#18454=CARTESIAN_POINT ( 'NONE',  ( -45.43829269268869808, 305.0573905683720000, -3.332260488124726194 ) ) ;
#18456=CARTESIAN_POINT ( 'NONE',  ( -32.01814843081345430, 447.5573905683720000, 16.75240474999999307 ) ) ;
#18457=LINE ( 'NONE', #3646, #3696 ) ;
#18458=CARTESIAN_POINT ( 'NONE',  ( -42.88789093042842637, 286.3073905683720000, 9.489475012073736337 ) ) ;
#18460=CARTESIAN_POINT ( 'NONE',  ( -28.68588794268870146, 269.7448905601784759, 19.99999999999999289 ) ) ;
#18461=CARTESIAN_POINT ( 'NONE',  ( -42.88789093042844769, 494.4323905683719431, -9.489475012073734561 ) ) ;
#18463=CARTESIAN_POINT ( 'NONE',  ( -38.17536295476246977, 473.8073905683720000, -14.20200298773971426 ) ) ;
#18464=CARTESIAN_POINT ( 'NONE',  ( -8.685887942688726326, 392.2448905601784759, -2.449293598294705724E-15 ) ) ;
#18465=CARTESIAN_POINT ( 'NONE',  ( -42.88789093042841927, 254.8073905683720284, 9.489475012073736337 ) ) ;
#18470=CARTESIAN_POINT ( 'NONE',  ( -35.09675569278793716, 247.2448905683720000, 15.47720386886985366 ) ) ;
#18473=CARTESIAN_POINT ( 'NONE',  ( -32.66413529028186247, 229.4323905601785043, 19.99999999999999289 ) ) ;
#18474=CARTESIAN_POINT ( 'NONE',  ( -38.17536295476244135, 275.4323905683720568, 14.20200298773971781 ) ) ;
#18475=CARTESIAN_POINT ( 'NONE',  ( -45.43829269268870519, 355.0573905683720568, -3.332260488124726194 ) ) ;
#18477=CARTESIAN_POINT ( 'NONE',  ( -45.64106924314019409, 506.3073905601784759, -11.32908994701042538 ) ) ;
#18481=CARTESIAN_POINT ( 'NONE',  ( -48.68588794268871567, 397.2448905601784759, 0.000000000000000000 ) ) ;
#18482=ORIENTED_EDGE ( 'NONE', *, *, #15061, .F. ) ;
#18485=ORIENTED_EDGE ( 'NONE', *, *, #14924, .F. ) ;
#18486=CARTESIAN_POINT ( 'NONE',  ( -11.93348319268874036, 520.0573905683719431, 3.332260488124728415 ) ) ;
#18487=CARTESIAN_POINT ( 'NONE',  ( -14.54375231895776110, 283.4948905601784759, -14.14213562373094746 ) ) ;
#18489=CARTESIAN_POINT ( 'NONE',  ( -28.68588794268870856, 317.8698905683720000, 16.75240474999999307 ) ) ;
#18491=CARTESIAN_POINT ( 'NONE',  ( -28.68588794268871567, 371.3698905683720568, -16.75240474999999307 ) ) ;
#18492=CARTESIAN_POINT ( 'NONE',  ( -28.68588794268871567, 371.3698905683720568, -16.75240474999999307 ) ) ;
#18493=CARTESIAN_POINT ( 'NONE',  ( -40.01497788969913216, 310.4323905765656377, -16.95518130045146421 ) ) ;
#18494=DIRECTION ( 'NONE',  ( 0.000000000000000000, 0.000000000000000000, 1.000000000000000000 ) ) ;
#18495=CARTESIAN_POINT ( 'NONE',  ( -44.16309181155855157, 264.4948905683720000, 6.410867750099241924 ) ) ;
#18496=CARTESIAN_POINT ( 'NONE',  ( -45.64106924314019409, 462.9323905765655809, 11.32908994701042538 ) ) ;
#18497=CARTESIAN_POINT ( 'NONE',  ( -35.09675569278795138, 413.4948905683720000, -15.47720386886985544 ) ) ;
#18499=CARTESIAN_POINT ( 'NONE',  ( -11.73070664223726389, 506.0573905765656377, 11.32908994701042005 ) ) ;
#18500=CARTESIAN_POINT ( 'NONE',  ( -11.73070664223723547, 276.0573905765655809, 11.32908994701042005 ) ) ;
#18501=UNCERTAINTY_MEASURE_WITH_UNIT (LENGTH_MEASURE( 1.000000000000000082E-05 ), #9106, 'distance_accuracy_value', 'NONE');
#18503=CARTESIAN_POINT ( 'NONE',  ( -32.01814843081344009, 327.5573905683720568, 16.75240474999999307 ) ) ;
#18504=CARTESIAN_POINT ( 'NONE',  ( -38.17536295476246977, 462.3073905683720568, -14.20200298773971426 ) ) ;
#18506=CARTESIAN_POINT ( 'NONE',  ( -14.54375231895778420, 473.4948905601785327, -14.14213562373094746 ) ) ;
#18507=CARTESIAN_POINT ( 'NONE',  ( -28.68588794268870501, 281.3698905683720000, -16.75240474999999307 ) ) ;
#18510=ORIENTED_EDGE ( 'NONE', *, *, #248, .F. ) ;
#18513=CARTESIAN_POINT ( 'NONE',  ( -44.16309181155857289, 384.7448905683720000, -6.410867750099231266 ) ) ;
#18515=CARTESIAN_POINT ( 'NONE',  ( -28.68588794268874054, 573.2448905601785327, 0.000000000000000000 ) ) ;
#18516=CARTESIAN_POINT ( 'NONE',  ( -24.70764059509555111, 384.8073905765655809, 19.99999999999998934 ) ) ;
#18517=CARTESIAN_POINT ( 'NONE',  ( -14.48388495494900674, 429.8073905683720000, -9.489475012073736337 ) ) ;
#18518=CARTESIAN_POINT ( 'NONE',  ( -38.17536295476243424, 266.9323905683720000, 14.20200298773971781 ) ) ;
#18519=CARTESIAN_POINT ( 'NONE',  ( -14.48388495494900674, 419.8073905683720000, -9.489475012073734561 ) ) ;
#18520=VECTOR ( 'NONE', #2584, 1000.000000000000000 ) ;
#18521=CARTESIAN_POINT ( 'NONE',  ( -36.33955658999051508, 363.8698905765656377, 18.47759065022572500 ) ) ;
#18523=CARTESIAN_POINT ( 'NONE',  ( -28.68588794268871212, 321.3698905683720568, -16.75240474999999307 ) ) ;
#18524=CARTESIAN_POINT ( 'NONE',  ( -42.82802356641967378, 490.7448905765656377, -14.14213562373094746 ) ) ;
#18525=CARTESIAN_POINT ( 'NONE',  ( -38.17536295476246977, 483.8073905683720000, -14.20200298773971426 ) ) ;
#18531=CARTESIAN_POINT ( 'NONE',  ( -38.17536295476245556, 396.9323905683721136, 14.20200298773971781 ) ) ;
#18533=CARTESIAN_POINT ( 'NONE',  ( -45.64106924314020119, 526.3073905601784190, -11.32908994701042715 ) ) ;
#18534=CARTESIAN_POINT ( 'NONE',  ( -28.68588794268871212, 356.3698905683720568, 16.75240474999999307 ) ) ;
#18536=ORIENTED_EDGE ( 'NONE', *, *, #2752, .F. ) ;
#18538=( BOUNDED_CURVE ( )  B_SPLINE_CURVE ( 2, ( #8385, #1482, #6654, #6763, #6545, #18342, #21376, #16738, #10116, #13381, #18233, #14690, #16520, #3318, #19639, #14903, #21267 ),
 .UNSPECIFIED., .F., .T. ) 
 B_SPLINE_CURVE_WITH_KNOTS ( ( 3, 2, 2, 2, 2, 2, 2, 2, 3 ),
 ( 0.5312500000000003331, 0.5332031250000003331, 0.5351562500000003331, 0.5371093750000003331, 0.5390625000000003331, 0.5410156250000003331, 0.5429687500000003331, 0.5449218750000003331, 0.5468750000000003331 ),
 .UNSPECIFIED. ) 
 CURVE ( )  GEOMETRIC_REPRESENTATION_ITEM ( )  RATIONAL_B_SPLINE_CURVE ( ( 0.9999999999999966693, 0.9807852804032337612, 1.000000000000000000, 0.9807852804032304306, 1.000000000000000000, 0.9807852804032304306, 1.000000000000000000, 0.9807852804032304306, 1.000000000000000000, 0.9807852804032304306, 1.000000000000000000, 0.9807852804032304306, 1.000000000000000000, 0.9807852804032304306, 1.000000000000000000, 0.9807852804032270999, 1.000000000000003331 ) ) 
 REPRESENTATION_ITEM ( '' )  );
#18539=CARTESIAN_POINT ( 'NONE',  ( -42.88789093042845479, 522.9323905683720568, -9.489475012073736337 ) ) ;
#18541=CARTESIAN_POINT ( 'NONE',  ( -8.685887942688442109, 527.3073905765654672, -3.978247347592446914 ) ) ;
#18542=CARTESIAN_POINT ( 'NONE',  ( -22.27502019258949062, 486.9948905683720568, 15.47720386886985189 ) ) ;
#18544=CARTESIAN_POINT ( 'NONE',  ( -19.19641293061499354, 487.3073905683719431, 14.20200298773971426 ) ) ;
#18546=EDGE_CURVE ( 'NONE', #15608, #19361, #16665, .T. ) ;
#18548=CARTESIAN_POINT ( 'NONE',  ( -10.20829729246299244, 416.3698905765656377, 7.653668647301790529 ) ) ;
#18549=CARTESIAN_POINT ( 'NONE',  ( -45.64106924314019409, 472.9323905765655809, 11.32908994701042538 ) ) ;
#18557=CARTESIAN_POINT ( 'NONE',  ( -45.43829269268870519, 295.3698905683720568, 0.000000000000000000 ) ) ;
#18558=EDGE_CURVE ( 'NONE', #13710, #683, #2194, .T. ) ;
#18560=CARTESIAN_POINT ( 'NONE',  ( -42.88789093042844769, 456.3073905683720000, 9.489475012073736337 ) ) ;
#18562=CARTESIAN_POINT ( 'NONE',  ( -11.93348319268871016, 270.3698905683720000, -2.051577885510841163E-15 ) ) ;
#18565=CARTESIAN_POINT ( 'NONE',  ( -40.01497788969911795, 268.8073905601784759, 16.95518130045146776 ) ) ;
#18566=CARTESIAN_POINT ( 'NONE',  ( -44.16309181155858710, 504.7448905683720000, -6.410867750099231266 ) ) ;
#18569=CARTESIAN_POINT ( 'NONE',  ( -40.53162694259545162, 464.1198905683720568, -11.84573899990672707 ) ) ;
#18571=CARTESIAN_POINT ( 'NONE',  ( -44.16309181155855867, 263.2448905683720000, -6.410867750099231266 ) ) ;
#18572=VERTEX_POINT ( 'NONE', #4001 ) ;
#18573=CARTESIAN_POINT ( 'NONE',  ( -24.70764059509554755, 334.8073905765656946, 19.99999999999998934 ) ) ;
#18575=CARTESIAN_POINT ( 'NONE',  ( -40.53162694259542320, 236.6198905683720284, 11.84573899990672885 ) ) ;
#18576=CARTESIAN_POINT ( 'NONE',  ( -40.01497788969912506, 308.8073905601784759, 16.95518130045146776 ) ) ;
#18577=CARTESIAN_POINT ( 'NONE',  ( -11.73070664223723369, 233.1823905601784475, -11.32908994701042715 ) ) ;
#18578=CARTESIAN_POINT ( 'NONE',  ( -22.27502019258947641, 270.7448905683720568, -15.47720386886985544 ) ) ;
#18579=CARTESIAN_POINT ( 'NONE',  ( -44.16309181155856578, 365.9948905683720568, 6.410867750099241924 ) ) ;
#18580=CARTESIAN_POINT ( 'NONE',  ( -42.88789093042844058, 404.8073905683721136, 9.489475012073736337 ) ) ;
#18582=CARTESIAN_POINT ( 'NONE',  ( -24.70764059509555821, 410.0573905601784759, 19.99999999999998934 ) ) ;
#18584=ORIENTED_EDGE ( 'NONE', *, *, #10920, .F. ) ;
#18588=CARTESIAN_POINT ( 'NONE',  ( -19.19641293061500420, 531.9323905683720568, -14.20200298773971603 ) ) ;
#18589=CARTESIAN_POINT ( 'NONE',  ( -11.73070664223723547, 281.3073905601784759, 11.32908994701042005 ) ) ;
#18590=CARTESIAN_POINT ( 'NONE',  ( -11.73070664223724613, 317.9323905765656377, -11.32908994701042538 ) ) ;
#18592=CARTESIAN_POINT ( 'NONE',  ( -35.09675569278794427, 317.2448905683720000, 15.47720386886985366 ) ) ;
#18594=CARTESIAN_POINT ( 'NONE',  ( -32.01814843081344719, 351.6823905683720000, -16.75240474999999307 ) ) ;
#18596=CARTESIAN_POINT ( 'NONE',  ( -35.09675569278795138, 365.7448905683720568, 15.47720386886985366 ) ) ;
#18599=CARTESIAN_POINT ( 'NONE',  ( -17.35679799567829207, 308.5573905765656377, -16.95518130045146421 ) ) ;
#18601=CARTESIAN_POINT ( 'NONE',  ( -38.17536295476244845, 272.3073905683720000, -14.20200298773971426 ) ) ;
#18602=CARTESIAN_POINT ( 'NONE',  ( -42.99843930773590017, 202.9216059526224569, 4.490902998358461851 ) ) ;
#18603=CARTESIAN_POINT ( 'NONE',  ( -25.35362745456398770, 418.1823905683720568, 16.75240474999998952 ) ) ;
#18605=CARTESIAN_POINT ( 'NONE',  ( -14.54375231895778420, 505.7448905765655809, 14.14213562373094568 ) ) ;
#18608=CARTESIAN_POINT ( 'NONE',  ( -28.68588794268870856, 327.8698905683720000, 16.75240474999999307 ) ) ;
#18609=CARTESIAN_POINT ( 'NONE',  ( -13.20868407381887089, 468.2448905683720568, 6.410867750099229490 ) ) ;
#18611=CARTESIAN_POINT ( 'NONE',  ( -10.20829729246299955, 472.8698905601784759, -7.653668647301794969 ) ) ;
#18612=CARTESIAN_POINT ( 'NONE',  ( -14.48388495494898720, 277.9323905683720000, 9.489475012073732785 ) ) ;
#18615=CARTESIAN_POINT ( 'NONE',  ( -36.33955658999051508, 339.1198905601784759, 18.47759065022572500 ) ) ;
#18616=CARTESIAN_POINT ( 'NONE',  ( -45.43829269268869808, 303.5573905683720568, -3.332260488124726194 ) ) ;
#18618=CARTESIAN_POINT ( 'NONE',  ( -16.84014894278199037, 379.1198905683720568, 11.84573899990672530 ) ) ;
#18620=CARTESIAN_POINT ( 'NONE',  ( -32.01814843081345430, 396.0573905683720568, 16.75240474999999307 ) ) ;
#18621=CARTESIAN_POINT ( 'NONE',  ( -45.43829269268869098, 265.0573905683720568, -3.332260488124726194 ) ) ;
#18622=CARTESIAN_POINT ( 'NONE',  ( -42.88789093042844058, 434.8073905683721136, 9.489475012073734561 ) ) ;
#18624=CARTESIAN_POINT ( 'NONE',  ( -21.03221929538692336, 358.8698905765656377, -18.47759065022572855 ) ) ;
#18625=DIRECTION ( 'NONE',  ( 1.191790137725560488E-16, -1.000000000000000000, 0.000000000000000000 ) ) ;
#18626=CARTESIAN_POINT ( 'NONE',  ( -13.20868407381885312, 318.2448905683720000, 6.410867750099229490 ) ) ;
#18627=CARTESIAN_POINT ( 'NONE',  ( -19.19641293061499709, 471.9323905683720568, -14.20200298773971603 ) ) ;
#18628=CARTESIAN_POINT ( 'NONE',  ( -14.54375231895777532, 435.7448905765656377, 14.14213562373094568 ) ) ;
#18630=CARTESIAN_POINT ( 'NONE',  ( -11.73070664223723014, 226.0573905765656093, 11.32908994701042005 ) ) ;
#18632=CARTESIAN_POINT ( 'NONE',  ( -13.20868407381886200, 380.9948905683720568, -6.410867750099233042 ) ) ;
#18634=CARTESIAN_POINT ( 'NONE',  ( -45.64106924314020119, 528.1823905601785327, 11.32908994701042715 ) ) ;
#18635=CARTESIAN_POINT ( 'NONE',  ( -13.20868407381885667, 338.2448905683720568, 6.410867750099229490 ) ) ;
#18637=CARTESIAN_POINT ( 'NONE',  ( -11.93348319268874214, 528.5573905683720568, 3.332260488124728415 ) ) ;
#18638=ORIENTED_EDGE ( 'NONE', *, *, #1933, .T. ) ;
#18639=CARTESIAN_POINT ( 'NONE',  ( -44.93162628806840786, 223.9102039777116602, -4.140855835305760735 ) ) ;
#18640=CARTESIAN_POINT ( 'NONE',  ( -8.685887942688539809, 312.5573905601784190, -3.978247347592740013 ) ) ;
#18641=DIRECTION ( 'NONE',  ( -1.000000000000000000, 0.000000000000000000, 0.000000000000000000 ) ) ;
#18642=CARTESIAN_POINT ( 'NONE',  ( -48.68588794268872277, 497.2448905601785327, 0.000000000000000000 ) ) ;
#18643=CARTESIAN_POINT ( 'NONE',  ( -11.93348319268873503, 478.8698905683720568, -2.051577885510841163E-15 ) ) ;
#18644=ORIENTED_EDGE ( 'NONE', *, *, #10003, .T. ) ;
#18645=CARTESIAN_POINT ( 'NONE',  ( -22.27502019258949773, 480.7448905683720568, -15.47720386886985544 ) ) ;
#18648=CARTESIAN_POINT ( 'NONE',  ( -42.82802356641966668, 420.7448905765656377, -14.14213562373094746 ) ) ;
#18657=CARTESIAN_POINT ( 'NONE',  ( -32.01814843081344009, 287.5573905683719431, 16.75240474999999307 ) ) ;
#18659=CARTESIAN_POINT ( 'NONE',  ( -13.20868407381886911, 449.7448905683720000, 6.410867750099229490 ) ) ;
#18661=( BOUNDED_SURFACE ( )  B_SPLINE_SURFACE ( 1, 2, ( 
 ( #16988, #6909, #10159, #3675, #8429, #7014, #343, #5082, #6804, #235, #10471, #18588, #10257, #14942, #13422, #18381, #20012, #16879, #5501, #15053, #11683, #1859, #7119, #3462, #20121, #447, #2168, #13744, #1963, #3570, #5189, #8751, #127, #13318, #13532, #18273, #15372, #550, #19901, #20330, #16778, #10049, #5290, #16673, #11786, #2062, #8534, #15158, #11893, #18486, #12103, #8638, #15265, #13637, #3883, #20223, #5392, #18695, #17092, #9068, #20548, #13963, #5714, #4318, #12546, #9172, #5611, #9284, #7440, #11008, #14066, #2703, #14287, #12219, #18803, #15473, #12322, #6039, #18910, #15689, #10901, #4095, #12649, #10683, #17301, #15900, #875, #17199, #17511, #3985, #19241, #4424, #2485, #8960, #2273, #8852, #10576, #7659, #20651, #20437, #767, #15583, #658, #19140, #19026, #7223, #7332, #5821, #12431, #4212, #20873, #10795, #2378, #17411, #1091, #2593, #15798, #985, #13844, #7549, #14174, #20763, #5932, #13072, #17617, #9393, #1395, #20975, #19656, #11436, #16012, #9808, #12860, #1194, #7970, #7764, #14391, #12963, #2809, #11227, #11117, #6143, #1609, #14600, #11330, #12754, #13182, #4633, #19344, #2917, #19450, #3017, #14494, #7865, #21075, #4836, #6456, #3122, #4530, #3232, #21182, #4952, #6353, #18036, #8182, #17720, #9497, #16110, #6249, #16280, #17824, #9600, #16430, #16218, #6561, #19553, #4734, #14812, #17925, #1289, #19766, #9707, #16326, #1502, #8076, #14706, #21283, #18141, #14919, #16963, #9917, #10025, #19986, #8404, #15029, #6674, #6993, #18463, #3652, #13715, #11657, #20202, #10234, #16536, #13615, #3441, #3335, #16859, #5268, #20308, #5367, #102, #16651, #6780, #8612, #6886, #7096, #13293, #10339, #318, #11972, #10135, #13400, #13506, #18249, #2041, #18358, #5055, #18569, #19878, #11551, #1721, #213, #1833, #531, #8293, #5167, #2142, #11763, #3549, #16755, #1942, #8510, #15137, #3751, #15236, #427, #20099, #11873, #8723, #15350, #3645, #7301, #18560, #11861, #12184, #20404, #5262, #13927, #15226, #3743, #524, #2346, #626, #842, #419, #4066, #15439, #734, #3851, #7085, #7191, #5360, #3958, #18659, #2035, #10330, #16952, #7408, #15550, #13814, #18456, #2134, #15340, #8715, #5579, #2453, #11963, #8603, #20191, #10650, #6985, #17061, #18770, #20515, #17270, #20299, #13707, #5471, #5684, #10227, #16850, #10440, #13606, #12290, #18876, #12069, #9034, #2244, #8822, #10546, #17167, #8926, #15657, #5790, #14249, #14139, #20615, #4598, #4389, #14357, #15760, #16182, #7621, #949, #5899, #15867, #6006, #17474, #10868, #2662, #1253, #9463, #6107, #2557, #6209, #10973, #7931, #17582, #21041, #11191, #9139, #7515, #12396, #9250, #2983, #1056, #12615, #7831, #20835, #9564, #19206, #2774, #12825, #12719, #20937, #18988, #14459, #20725, #12509, #9357, #17687, #15974, #1359, #19102, #19414, #1158, #16075, #7729, #19308, #4494, #4286, #11080, #2879, #17376, #17791, #4169, #10760, #3407, #9880, #21147, #6417, #3195, #19624, #16503, #11729, #21252, #11295, #8041, #13363, #9667, #4915, #6636, #9986, #19954, #8143, #9773, #4802, #16610, #14562, #6319, #19733, #17891, #1800, #8367, #12933, #6746, #16398, #19519, #11513, #4698, #3085, #1683, #16293, #14774, #14674, #1466, #5131, #18107, #8255, #13034, #10097, #1575, #11398, #18000, #21359, #6527, #13143, #3303, #14884, #14992, #177, #69, #13257, #18321, #19844, #1908, #5020, #3510, #16719, #11621, #18216, #283, #18531, #12262, #20170, #497, #17138, #3718, #18844, #5336, #11936, #15517, #15310, #2012, #2319, #11834, #4034, #10624, #10302, #15202, #17241, #15098, #18431, #13896, #6851, #6957, #16928, #2109, #8689, #3616, #3930, #15413, #597, #8475, #8579, #8899, #7162, #13470, #10515, #391, #20060, #5235, #10201, #3821, #16822, #7060, #13580, #13679, #20485, #20270, #2212, #5442, #12041, #18632, #10411, #17032, #8796, #13785, #20373, #5547, #12154, #702, #18741, #7271, #5657, #9434, #7590, #11162, #14219, #2852, #14434, #5757, #12367, #15627, #12479, #6184, #14110, #15838, #11048, #19072, #12795, #20695, #5868, #16053, #9219, #17345, #17660, #18955, #19387, #4572, #4255, #9112, #2424, #9006, #4138, #7802, #813, #920, #10842, #17447, #1025, #10731, #19282, #9324, #15943, #14007, #2529, #1230, #1130, #20587, #4465, #15733, #7483, #7702, #17554, #20807, #5976, #12588, #19180, #4357, #20910, #10944, #2743, #14330, #6076, #12689, #13229, #16369, #19598, #13116, #17864, #16476, #9748, #14533, #16262, #9642, #19922, #6607, #19701, #2957, #1440, #6393, #8011, #4886, #14961, #3057, #21118, #11265, #16581, #12904, #8117, #9849, #19819, #1769, #11371, #13004, #14644, #4995, #17765, #9534, #1545, #6290, #11594, #18185, #16154, #9962, #4774, #1332, #14749, #21332, #8228, #1659, #13338, #33, #21228, #3383, #6499, #18081, #7905, #17966, #8338, #148, #3169, #6721, #5101, #19495, #4673, #11484, #14857, #3275, #10067, #13552, #1983, #6928, #13654, #8659, #20141, #2080, #5411, #18294, #8769, #675, #18712, #7240, #20347, #12124, #11702, #3691, #5207, #362, #5522, #10279, #7032, #5308, #15284, #20239, #12015, #3588, #13761, #467, #18400, #11909, #8447, #18608, #18503, #3900, #3481, #10489, #3792, #15387, #15174, #2290, #11804, #567, #7135, #8871, #16690, #1879, #16898, #10384, #15489, #17004, #8554, #17111, #15072, #13868, #2185, #20456, #256, #16795, #6823, #13439, #10174, #4727, #19547, #9386, #9699, #8977, #7652, #8070, #1388, #11110, #2799, #1280, #2911, #19442, #4002, #6030, #16004, #21175, #14487, #15601, #16320, #4521, #1081, #12237, #10594, #14593, #1495, #14278, #17713, #5627, #9594, #6347, #2395, #11325, #9491, #17919, #12744, #14700, #18820, #3117, #16211, #12642, #21067, #7859, #17608, #17214, #20865, #1187, #19233, #16103, #4416, #10999, #6240, #7756, #20966, #14383, #6136, #19336, #12853, #4627, #11221, #17818, #3010, #7961, #12958, #1716, #6668, #18135, #11545, #3328, #1937, #10128, #6773, #3224, #6880, #5049, #8605, #11650, #312, #11863, #9802, #16424, #13065, #9910, #3647, #8283, #13289, #8503, #14913, #10229, #19873, #18244, #13500, #3436, #14807, #15129, #1602, #16851, #21277, #10018, #6556, #6449, #19651, #8176, #18458, #4831, #19762, #16642, #1828, #8397, #21390, #16750, #13394, #19981, #11429, #13176, #20093, #5161, #18031, #4945, #15024, #207, #11757, #3541, #2559, #2455, #3745, #7087, #10442, #12292, #10548, #10762, #10332, #14035, #3960, #10652, #13816, #17063, #17170, #15342, #13929, #7193, #11965, #13709, #20301, #17378, #4068, #2348, #421, #5473, #3853, #12071, #8928, #12398, #526, #18562, #8718, #20617, #16954, #5581, #7303, #17272, #5792, #8824, #2246, #18662, #9036, #15228, #6987, #20406, #2136, #15658, #844, #7409, #13608, #20194, #12186, #15441, #18990, #4172, #5362, #628, #18772, #15552, #736, #20517, #5686, #18878, #15762, #2776, #2664, #9141, #14564, #14359, #2881, #4288, #4701, #17584, #10870, #15869, #4391, #15976, #6008, #20837, #12618, #11193, #19416, #16077, #12511, #16184, #20939, #17893, #6109, #9567, #21149, #19104, #17476, #951, #19208, #12934, #10975, #1160, #17793, #9360, #19521, #7731, #12721, #1361, #19310, #9252, #2985, #1057, #11297, #7517, #4496, #7624, #14141, #20727, #14251, #6321, #5901, #11084, #17689, #9465, #1255, #7833, #4600, #14461, #21043, #6211, #12827, #7934, #9988, #1468, #5133, #16400, #9670, #16612, #18218, #11837, #11732, #13036, #1577, #19735, #180, #19846, #20064, #19626, #1910, #13260, #19956, #1685, #4919, #5023, #3197, #1802, #16506, #21254, #8146, #14776, #5237, #13365, #11623, #16295, #21361, #13146, #6530, #3409, #285, #9775, #6419, #18003, #8478, #4804, #14886, #8370, #18323, #15100, #18109, #11516, #3305, #16721, #8257, #6853, #9882, #3087, #13472, #8044, #6748, #71, #14994, #3513, #6639, #10100 ),
 ( #11400, #14676, #10203, #7062, #816, #8691, #10413, #5659, #13681, #7383, #15314, #500, #4036, #3825, #11938, #12264, #394, #14009, #20589, #20272, #3721, #5759, #3618, #6960, #2426, #16825, #16930, #5444, #12044, #18634, #13583, #13898, #3932, #10518, #18433, #18533, #18848, #17140, #2014, #20488, #10304, #8581, #2321, #12156, #15204, #10626, #20172, #2112, #17034, #15519, #13787, #5338, #2215, #17243, #7164, #9008, #8798, #15415, #20377, #599, #8901, #5550, #18744, #704, #7275, #15631, #1232, #7705, #18957, #4257, #1027, #17449, #14333, #9536, #19074, #9114, #5870, #11165, #7486, #2745, #4469, #7804, #17767, #5980, #7592, #2636, #14436, #12369, #14112, #4140, #17348, #21017, #7907, #15735, #10946, #10734, #16055, #6186, #921, #4574, #17556, #2959, #19183, #21121, #16156, #1334, #12798, #10845, #20912, #6078, #9221, #9326, #2854, #11050, #14535, #19389, #12482, #2531, #1132, #12691, #20697, #15841, #14222, #20809, #12590, #4360, #15947, #19284, #17662, #9437, #18188, #19497, #4675, #8120, #17969, #1548, #8231, #3279, #14752, #18085, #36, #12907, #3386, #16693, #13341, #1882, #14964, #6724, #6292, #19704, #21230, #16374, #152, #4890, #1662, #21335, #9852, #14860, #6611, #19600, #8342, #16479, #13006, #6503, #3059, #13232, #13119, #19926, #11267, #5104, #19823, #9965, #9751, #18297, #14647, #16584, #1772, #3484, #17866, #9644, #11487, #4998, #10072, #11599, #3172, #11705, #16264, #8450, #15075, #1443, #8014, #11373, #6395, #4776, #15390, #20460, #13871, #3694, #4005, #3591, #1986, #2398, #17114, #5414, #18506, #17008, #18611, #13764, #20034, #365, #10282, #15492, #8772, #10177, #10597, #20242, #678, #13657, #2188, #8662, #3795, #570, #7138, #13556, #2293, #10387, #6931, #16901, #18403, #20350, #470, #7243, #13442, #5630, #5525, #18716, #2083, #12240, #8557, #3903, #8874, #18823, #5210, #6827, #7035, #12127, #17217, #10492, #11912, #8980, #11809, #259, #15287, #12018, #16798, #5311, #15178, #20144, #9303, #14412, #7780, #19048, #19363, #18930, #17321, #17741, #11025, #20784, #12449, #10919, #12566, #7679, #13982, #15707, #4233, #9413, #2722, #4114, #4550, #14193, #10702, #791, #20565, #2828, #11138, #2505, #5951, #15604, #19259, #16029, #12343, #20994, #19161, #6159, #1003, #2933, #7351, #12772, #4441, #894, #15917, #17530, #5843, #4338, #6056, #14305, #5733, #17636, #7458, #1210, #1108, #20889, #9088, #20669, #14087, #10815, #17429, #2610, #9193, #15818, #7567, #12667, #10, #1312, #7884, #11349, #21206, #4753, #11456, #6476, #17945, #21305, #3250, #16130, #6584, #19897, #16557, #5076, #18159, #9936, #9513, #1522, #3037, #19572, #19678, #9826, #14511, #14621, #3358, #19789, #3142, #11570, #1741, #21095, #8314, #6267, #13205, #12883, #19470, #9724, #6371, #16347, #18056, #13092, #8095, #4861, #16450, #4653, #4972, #11678, #14937, #18268, #121, #6695, #11243, #14724, #9620, #1632, #13313, #8205, #14833, #17841, #16239, #1416, #7990, #12981, #5496, #442, #10155, #20116, #231, #3770, #3668, #10466, #16669, #18690, #5386, #545, #6904, #15468, #11782, #7114, #20324, #652, #1855, #10044, #10252, #18582, #7217, #10357, #15155, #13739, #8424, #13839, #11888, #15260, #7009, #8529, #13632, #15367, #16982, #2268, #17087, #13527, #20432, #6800, #5185, #5606, #12098, #8632, #337, #20218, #11992, #2163, #15048, #3566, #5285, #3877, #8746, #13417, #12212, #2058, #20008, #18377, #16772, #8846, #3458, #1959, #18481, #16874, #1087, #12645, #15577, #11002, #17406, #9389, #4207, #6139, #1190, #17613, #7655, #4090, #5927, #14169, #9063, #9167, #9279, #17505, #14387, #14283, #18906, #20869, #10678, #2698, #10789, #762, #17297, #2480, #20970, #6034, #20758, #3981, #15684, #7434, #870, #12541, #16008, #14061, #7327, #12317, #2805, #13958, #15791, #10896, #19236, #7760, #12425, #20646, #5816, #4420, #18798, #10570, #2588, #20542, #17194, #2372, #8955, #5709, #19022, #980, #7543, #19134, #4313, #15896, #19339, #6350, #6245, #12749, #18137, #17921, #6452, #7862, #8288, #21179, #14490, #19447, #7967, #19550, #9597, #3013, #16214, #14809, #1605, #19653, #16107, #19764, #3119, #99, #9703, #13179, #3331, #1285, #21072, #4527, #1391, #16533, #14596, #4730, #20423, #12960, #1718, #11327, #16323, #4949, #1498, #12857, #6558, #4630, #14916, #11114, #8073, #11224, #17717, #2914, #17821, #9913, #9494, #14703, #21279, #13068, #4833, #11433, #8178, #18033, #3229, #9804, #16427, #11548, #13903, #11944, #821, #12050, #13588, #20493, #12269, #15740, #5766, #2117, #10418, #2221, #10631, #15526, #10310, #8696, #18964, #4145, #7067, #5555, #8803, #7170, #12162, #20382, #18749, #18937, #20571, #10182, #4012, #16907, #18721, #5530, #477, #575, #7251, #8881, #16803, #10606, #10287, #17224, #20355, #10500, #1992, #15292, #2406, #8562, #5422, #15183, #369, #5317, #2088, #8668, #7043, #13662, #20249, #12023, #18615, #3801, #12134, #7144, #10393, #13768, #3909, #17012, #8778, #15499, #11142, #21100, #12777, #4555, #4120, #17536, #19054, #14201, #19370, #2728, #20894, #12571, #7684, #12672, #19265, #17434, #6164, #1114, #10823, #20790, #900, #4446, #4344, #17747, #17328, #2938, #6062, #1215, #7573, #16135, #12455, #7785, #20999, #1318, #2511, #10708, #10925, #11031, #7889, #17641, #15824, #14417, #9095, #14516, #19166, #15922, #14311, #9198, #2834, #16034, #9417, #9518, #6273, #5956, #12888, #7464, #5850, #15714, #14094, #9307, #1009, #20675, #4238, #2616, #17846, #19577, #8099, #13319, #6589, #7994, #1860, #18061, #14627, #4658, #3042, #6700, #15054, #1420, #3256, #19476, #1747, #19902, #16244, #11684, #16563, #1528, #10050, #6376, #8320, #14943, #16674, #11248, #9625, #4869, #13212, #8430, #19794, #9729, #128, #21211, #236, #6481, #9833, #16456, #3148, #8211, #9942, #4976, #18274, #3463, #14728, #6805, #12986, #4758, #11354, #5083, #1637, #16352, #14838, #15, #11575, #17951, #21310, #13098, #19684, #18166, #11462, #3363, #448, #1964, #20014, #18382, #12104, #7224, #3571, #7015, #13423, #5502, #10472, #16779, #2274, #20224, #659, #13638, #5190, #13845, #20438, #18696, #5291, #2169, #10363, #3676, #11999, #20331, #7120, #11787, #17093, #11894, #8853, #8752, #13745, #8535, #16880, #15474, #10160, #5393, #15159, #345, #18487, #6910, #10258, #13533, #2064, #8639, #16989, #18589, #15373, #20122, #15266, #3776, #551, #3884, #17917, #8395, #309, #18352, #6878, #19979, #11755, #11322, #3326, #4829, #21388, #5159, #9908, #6666, #19760, #14911, #19871, #5047, #3222, #13392, #8281, #18028, #6554, #8068, #11648, #11542, #3538, #3115, #10126, #13286, #9799, #4943, #8174, #14805, #6447, #6771, #18242, #3434, #13498, #11427, #16747, #10016, #9697, #1935, #16422, #16318, #16640, #1825, #20091, #8501, #21275, #1600, #13174, #15021, #205, #1493, #13063, #15127, #95, #14698, #16529, #18133, #19649, #1714, #9137, #9031, #7189, #8925, #2344, #12613, #20723, #5788, #17059, #15548, #20513, #731, #12394, #7619, #17164, #13812, #3956, #9248, #5577, #7406, #15758, #5897, #15865, #4064, #5682, #7299, #12507, #10438, #2242, #14032, #20402, #19100, #4284, #15437, #2659, #18873, #12182, #20612, #18768, #10543, #18986, #13925, #10648, #17267, #4167, #1054, #946, #7513, #14137, #6004, #10866, #17472, #14246, #20833, #19204, #2772, #9355, #15972, #20935, #14355, #7727, #10971, #6104, #1156, #12717, #4386, #17580, #15359, #6683, #13303, #16545, #13408, #7107, #15038, #16763, #11983, #19997, #13727, #222, #6790, #10350, #10147, #18258, #18577, #19888, #20317, #5489, #5175, #10034, #12089, #9925, #5064, #8734, #1730, #8520, #18473, #11668, #3345, #11772, #3449, #16660, #18367, #1951, #3558, #15146, #328, #5377, #13623, #10243, #1845, #16973, #6895, #8304, #13517, #3762, #540, #8413 ) ),
 .UNSPECIFIED., .F., .F., .T. ) 
 B_SPLINE_SURFACE_WITH_KNOTS ( ( 2, 2 ),
 ( 3, 2, 2, 2, 2, 2, 2, 2, 2, 2, 2, 2, 2, 2, 2, 2, 2, 2, 2, 2, 2, 2, 2, 2, 2, 2, 2, 2, 2, 2, 2, 2, 2, 2, 2, 2, 2, 2, 2, 2, 2, 2, 2, 2, 2, 2, 2, 2, 2, 2, 2, 2, 2, 2, 2, 2, 2, 2, 2, 2, 2, 2, 2, 2, 2, 2, 2, 2, 2, 2, 2, 2, 2, 2, 2, 2, 2, 2, 2, 2, 2, 2, 2, 2, 2, 2, 2, 2, 2, 2, 2, 2, 2, 2, 2, 2, 2, 2, 2, 2, 2, 2, 2, 2, 2, 2, 2, 2, 2, 2, 2, 2, 2, 2, 2, 2, 2, 2, 2, 2, 2, 2, 2, 2, 2, 2, 2, 2, 2, 2, 2, 2, 2, 2, 2, 2, 2, 2, 2, 2, 2, 2, 2, 2, 2, 2, 2, 2, 2, 2, 2, 2, 2, 2, 2, 2, 2, 2, 2, 2, 2, 2, 2, 2, 2, 2, 2, 2, 2, 2, 2, 2, 2, 2, 2, 2, 2, 2, 2, 2, 2, 2, 2, 2, 2, 2, 2, 2, 2, 2, 2, 2, 2, 2, 2, 2, 2, 2, 2, 2, 2, 2, 2, 2, 2, 2, 2, 2, 2, 2, 2, 2, 2, 2, 2, 2, 2, 2, 2, 2, 2, 2, 2, 2, 2, 2, 2, 2, 2, 2, 2, 2, 2, 2, 2, 2, 2, 2, 2, 2, 2, 2, 2, 2, 2, 2, 2, 2, 2, 2, 2, 2, 2, 2, 2, 2, 2, 2, 2, 2, 2, 2, 2, 2, 2, 2, 2, 2, 2, 2, 2, 2, 2, 2, 2, 2, 2, 2, 2, 2, 2, 2, 2, 2, 2, 2, 2, 2, 2, 2, 2, 2, 2, 2, 2, 2, 2, 2, 2, 2, 2, 2, 2, 2, 2, 2, 2, 2, 2, 2, 2, 2, 2, 2, 2, 2, 2, 2, 2, 2, 2, 2, 2, 2, 2, 2, 2, 2, 2, 2, 2, 2, 2, 2, 2, 2, 2, 2, 2, 2, 2, 2, 2, 2, 2, 2, 2, 2, 2, 2, 2, 2, 2, 2, 2, 2, 2, 2, 2, 2, 2, 2, 2, 2, 2, 2, 2, 2, 2, 2, 2, 2, 2, 2, 2, 2, 2, 2, 2, 2, 2, 2, 2, 2, 2, 2, 2, 2, 2, 2, 2, 2, 2, 2, 2, 2, 2, 2, 2, 2, 2, 2, 2, 2, 2, 2, 2, 2, 2, 2, 2, 2, 2, 2, 2, 2, 2, 2, 2, 2, 2, 2, 2, 2, 2, 2, 2, 2, 2, 2, 2, 2, 2, 2, 2, 2, 2, 2, 2, 2, 2, 2, 2, 2, 2, 2, 2, 2, 2, 2, 2, 2, 2, 2, 2, 2, 2, 2, 2, 2, 2, 2, 2, 2, 2, 2, 2, 2, 2, 2, 2, 2, 2, 2, 2, 2, 2, 2, 2, 2, 2, 2, 2, 2, 2, 2, 2, 2, 2, 2, 2, 2, 2, 2, 2, 2, 2, 2, 2, 2, 2, 2, 2, 3 ),
 ( 0.000000000000000000, 1.000000000000000000 ),
 ( 0.000000000000000000, 0.001953125000000000000, 0.003906250000000000000, 0.005859375000000000000, 0.007812500000000000000, 0.009765625000000000000, 0.01171875000000000000, 0.01367187500000000000, 0.01562500000000000000, 0.01757812500000000000, 0.01953125000000000000, 0.02148437500000000000, 0.02343750000000000000, 0.02539062500000000000, 0.02734375000000000000, 0.02929687500000000000, 0.03125000000000000000, 0.03320312500000000000, 0.03515625000000000000, 0.03710937500000000000, 0.03906250000000000000, 0.04101562500000000000, 0.04296875000000000000, 0.04492187500000000000, 0.04687500000000000000, 0.04882812500000000000, 0.05078125000000000000, 0.05273437500000000000, 0.05468750000000000000, 0.05664062500000000000, 0.05859375000000000000, 0.06054687500000000000, 0.06250000000000000000, 0.06445312500000000000, 0.06640625000000000000, 0.06835937500000000000, 0.07031250000000000000, 0.07226562500000000000, 0.07421875000000000000, 0.07617187500000000000, 0.07812500000000000000, 0.08007812500000000000, 0.08203125000000000000, 0.08398437500000000000, 0.08593750000000000000, 0.08789062500000000000, 0.08984375000000000000, 0.09179687500000000000, 0.09375000000000000000, 0.09570312500000000000, 0.09765625000000000000, 0.09960937500000000000, 0.1015625000000000000, 0.1035156250000000000, 0.1054687500000000000, 0.1074218750000000000, 0.1093750000000000000, 0.1113281250000000000, 0.1132812500000000000, 0.1152343750000000000, 0.1171875000000000000, 0.1191406250000000000, 0.1210937500000000000, 0.1230468750000000000, 0.1250000000000000000, 0.1269531250000000000, 0.1289062500000000000, 0.1308593750000000000, 0.1328125000000000000, 0.1347656250000000000, 0.1367187500000000000, 0.1386718750000000000, 0.1406250000000000000, 0.1425781250000000000, 0.1445312500000000000, 0.1464843750000000000, 0.1484375000000000000, 0.1503906250000000000, 0.1523437500000000000, 0.1542968750000000000, 0.1562500000000000000, 0.1582031250000000000, 0.1601562500000000000, 0.1621093750000000000, 0.1640625000000000000, 0.1660156250000000000, 0.1679687500000000000, 0.1699218750000000000, 0.1718750000000000000, 0.1738281250000000000, 0.1757812500000000000, 0.1777343750000000000, 0.1796875000000000000, 0.1816406250000000000, 0.1835937500000000000, 0.1855468750000000000, 0.1875000000000000000, 0.1894531250000000000, 0.1914062500000000000, 0.1933593750000000000, 0.1953125000000000000, 0.1972656250000000000, 0.1992187500000000000, 0.2011718750000000000, 0.2031250000000000000, 0.2050781250000000000, 0.2070312500000000000, 0.2089843750000000000, 0.2109375000000000000, 0.2128906250000000000, 0.2148437500000000000, 0.2167968750000000000, 0.2187500000000000000, 0.2207031250000000000, 0.2226562500000000000, 0.2246093750000000000, 0.2265625000000000000, 0.2285156250000000000, 0.2304687500000000000, 0.2324218750000000000, 0.2343750000000000000, 0.2363281250000000000, 0.2382812500000000000, 0.2402343750000000000, 0.2421875000000000000, 0.2441406250000000000, 0.2460937500000000000, 0.2480468750000000000, 0.2500000000000000000, 0.2519531250000000000, 0.2539062500000000000, 0.2558593750000000000, 0.2578125000000000000, 0.2597656250000000000, 0.2617187500000000000, 0.2636718750000000000, 0.2656250000000000000, 0.2675781250000000000, 0.2695312500000000000, 0.2714843750000000000, 0.2734375000000000000, 0.2753906250000000000, 0.2773437500000000000, 0.2792968750000000000, 0.2812500000000000000, 0.2832031250000000000, 0.2851562500000000000, 0.2871093750000000000, 0.2890625000000000000, 0.2910156250000000000, 0.2929687500000000000, 0.2949218750000000000, 0.2968750000000000000, 0.2988281250000000000, 0.3007812500000000000, 0.3027343750000000000, 0.3046875000000000000, 0.3066406250000000000, 0.3085937500000000000, 0.3105468750000000000, 0.3125000000000000000, 0.3144531250000000000, 0.3164062500000000000, 0.3183593750000000000, 0.3203125000000000000, 0.3222656250000000000, 0.3242187500000000000, 0.3261718750000000000, 0.3281250000000000000, 0.3300781250000000000, 0.3320312500000000000, 0.3339843750000000000, 0.3359375000000000000, 0.3378906250000000000, 0.3398437500000000000, 0.3417968750000000000, 0.3437500000000000000, 0.3457031250000000000, 0.3476562500000000000, 0.3496093750000000000, 0.3515625000000000000, 0.3535156250000000000, 0.3554687500000000000, 0.3574218750000000000, 0.3593750000000000000, 0.3613281250000000000, 0.3632812500000000000, 0.3652343750000000000, 0.3671875000000000000, 0.3691406250000000000, 0.3710937500000000000, 0.3730468750000000000, 0.3750000000000000000, 0.3769531250000000000, 0.3789062500000000000, 0.3808593750000000000, 0.3828125000000000000, 0.3847656250000000000, 0.3867187500000000000, 0.3886718750000000000, 0.3906250000000000000, 0.3925781250000000000, 0.3945312500000000000, 0.3964843750000000000, 0.3984375000000000000, 0.4003906250000000000, 0.4023437500000000000, 0.4042968750000000000, 0.4062500000000000000, 0.4082031250000000000, 0.4101562500000000000, 0.4121093750000000000, 0.4140625000000000000, 0.4160156250000000000, 0.4179687500000000000, 0.4199218750000000000, 0.4218750000000000000, 0.4238281250000000000, 0.4257812500000000000, 0.4277343750000000000, 0.4296875000000000000, 0.4316406250000000000, 0.4335937500000000000, 0.4355468750000000000, 0.4375000000000000000, 0.4394531250000000000, 0.4414062500000000000, 0.4433593750000000000, 0.4453125000000000000, 0.4472656250000000000, 0.4492187500000000000, 0.4511718750000000000, 0.4531250000000000000, 0.4550781250000000000, 0.4570312500000000000, 0.4589843750000000000, 0.4609375000000000000, 0.4628906250000000000, 0.4648437500000000000, 0.4667968750000000000, 0.4687500000000000000, 0.4707031250000000000, 0.4726562500000000000, 0.4746093750000000000, 0.4765625000000000000, 0.4785156250000000000, 0.4804687500000000000, 0.4824218750000000000, 0.4843750000000000000, 0.4863281250000000000, 0.4882812500000000000, 0.4902343750000000000, 0.4921875000000000000, 0.4941406250000000000, 0.4960937500000000000, 0.4980468750000000000, 0.5000000000000000000, 0.5019531250000000000, 0.5039062500000000000, 0.5058593750000000000, 0.5078125000000000000, 0.5097656250000000000, 0.5117187500000000000, 0.5136718750000000000, 0.5156250000000000000, 0.5175781250000000000, 0.5195312500000000000, 0.5214843750000000000, 0.5234375000000000000, 0.5253906250000000000, 0.5273437500000000000, 0.5292968750000000000, 0.5312500000000000000, 0.5332031250000000000, 0.5351562500000000000, 0.5371093750000000000, 0.5390625000000000000, 0.5410156250000000000, 0.5429687500000000000, 0.5449218750000000000, 0.5468750000000000000, 0.5488281250000000000, 0.5507812500000000000, 0.5527343750000000000, 0.5546875000000000000, 0.5566406250000000000, 0.5585937500000000000, 0.5605468750000000000, 0.5625000000000000000, 0.5644531250000000000, 0.5664062500000000000, 0.5683593750000000000, 0.5703125000000000000, 0.5722656250000000000, 0.5742187500000000000, 0.5761718750000000000, 0.5781250000000000000, 0.5800781250000000000, 0.5820312500000000000, 0.5839843750000000000, 0.5859375000000000000, 0.5878906250000000000, 0.5898437500000000000, 0.5917968750000000000, 0.5937500000000000000, 0.5957031250000000000, 0.5976562500000000000, 0.5996093750000000000, 0.6015625000000000000, 0.6035156250000000000, 0.6054687500000000000, 0.6074218750000000000, 0.6093750000000000000, 0.6113281250000000000, 0.6132812500000000000, 0.6152343750000000000, 0.6171875000000000000, 0.6191406250000000000, 0.6210937500000000000, 0.6230468750000000000, 0.6250000000000000000, 0.6269531250000000000, 0.6289062500000000000, 0.6308593750000000000, 0.6328125000000000000, 0.6347656250000000000, 0.6367187500000000000, 0.6386718750000000000, 0.6406250000000000000, 0.6425781250000000000, 0.6445312500000000000, 0.6464843750000000000, 0.6484375000000000000, 0.6503906250000000000, 0.6523437500000000000, 0.6542968750000000000, 0.6562500000000000000, 0.6582031250000000000, 0.6601562500000000000, 0.6621093750000000000, 0.6640625000000000000, 0.6660156250000000000, 0.6679687500000000000, 0.6699218750000000000, 0.6718750000000000000, 0.6738281250000000000, 0.6757812500000000000, 0.6777343750000000000, 0.6796875000000000000, 0.6816406250000000000, 0.6835937500000000000, 0.6855468750000000000, 0.6875000000000000000, 0.6894531250000000000, 0.6914062500000000000, 0.6933593750000000000, 0.6953125000000000000, 0.6972656250000000000, 0.6992187500000000000, 0.7011718750000000000, 0.7031250000000000000, 0.7050781250000000000, 0.7070312500000000000, 0.7089843750000000000, 0.7109375000000000000, 0.7128906250000000000, 0.7148437500000000000, 0.7167968750000000000, 0.7187500000000000000, 0.7207031250000000000, 0.7226562500000000000, 0.7246093750000000000, 0.7265625000000000000, 0.7285156250000000000, 0.7304687500000000000, 0.7324218750000000000, 0.7343750000000000000, 0.7363281250000000000, 0.7382812500000000000, 0.7402343750000000000, 0.7421875000000000000, 0.7441406250000000000, 0.7460937500000000000, 0.7480468750000000000, 0.7500000000000000000, 0.7519531250000000000, 0.7539062500000000000, 0.7558593750000000000, 0.7578125000000000000, 0.7597656250000000000, 0.7617187500000000000, 0.7636718750000000000, 0.7656250000000000000, 0.7675781250000000000, 0.7695312500000000000, 0.7714843750000000000, 0.7734375000000000000, 0.7753906250000000000, 0.7773437500000000000, 0.7792968750000000000, 0.7812500000000000000, 0.7832031250000000000, 0.7851562500000000000, 0.7871093750000000000, 0.7890625000000000000, 0.7910156250000000000, 0.7929687500000000000, 0.7949218750000000000, 0.7968750000000000000, 0.7988281250000000000, 0.8007812500000000000, 0.8027343750000000000, 0.8046875000000000000, 0.8066406250000000000, 0.8085937500000000000, 0.8105468750000000000, 0.8125000000000000000, 0.8144531250000000000, 0.8164062500000000000, 0.8183593750000000000, 0.8203125000000000000, 0.8222656250000000000, 0.8242187500000000000, 0.8261718750000000000, 0.8281250000000000000, 0.8300781250000000000, 0.8320312500000000000, 0.8339843750000000000, 0.8359375000000000000, 0.8378906250000000000, 0.8398437500000000000, 0.8417968750000000000, 0.8437500000000000000, 0.8457031250000000000, 0.8476562500000000000, 0.8496093750000000000, 0.8515625000000000000, 0.8535156250000000000, 0.8554687500000000000, 0.8574218750000000000, 0.8593750000000000000, 0.8613281250000000000, 0.8632812500000000000, 0.8652343750000000000, 0.8671875000000000000, 0.8691406250000000000, 0.8710937500000000000, 0.8730468750000000000, 0.8750000000000000000, 0.8769531250000000000, 0.8789062500000000000, 0.8808593750000000000, 0.8828125000000000000, 0.8847656250000000000, 0.8867187500000000000, 0.8886718750000000000, 0.8906250000000000000, 0.8925781250000000000, 0.8945312500000000000, 0.8964843750000000000, 0.8984375000000000000, 0.9003906250000000000, 0.9023437500000000000, 0.9042968750000000000, 0.9062500000000000000, 0.9082031250000000000, 0.9101562500000000000, 0.9121093750000000000, 0.9140625000000000000, 0.9160156250000000000, 0.9179687500000000000, 0.9199218750000000000, 0.9218750000000000000, 0.9238281250000000000, 0.9257812500000000000, 0.9277343750000000000, 0.9296875000000000000, 0.9316406250000000000, 0.9335937500000000000, 0.9355468750000000000, 0.9375000000000000000, 0.9394531250000000000, 0.9414062500000000000, 0.9433593750000000000, 0.9453125000000000000, 0.9472656250000000000, 0.9492187500000000000, 0.9511718750000000000, 0.9531250000000000000, 0.9550781250000000000, 0.9570312500000000000, 0.9589843750000000000, 0.9609375000000000000, 0.9628906250000000000, 0.9648437500000000000, 0.9667968750000000000, 0.9687500000000000000, 0.9707031250000000000, 0.9726562500000000000, 0.9746093750000000000, 0.9765625000000000000, 0.9785156250000000000, 0.9791718336226143959, 0.9889635519588405588 ),
 .UNSPECIFIED. ) 
 GEOMETRIC_REPRESENTATION_ITEM ( )  RATIONAL_B_SPLINE_SURFACE ( (
 ( 1.000000000000000000, 0.9807852804032304306, 1.000000000000000000, 0.9807852804032304306, 1.000000000000000000, 0.9807852804032304306, 1.000000000000000000, 0.9807852804032304306, 1.000000000000000000, 0.9807852804032304306, 1.000000000000000000, 0.9807852804032304306, 1.000000000000000000, 0.9807852804032304306, 1.000000000000000000, 0.9807852804032304306, 1.000000000000000000, 0.9807852804032304306, 1.000000000000000000, 0.9807852804032304306, 1.000000000000000000, 0.9807852804032304306, 1.000000000000000000, 0.9807852804032304306, 1.000000000000000000, 0.9807852804032304306, 1.000000000000000000, 0.9807852804032304306, 1.000000000000000000, 0.9807852804032304306, 1.000000000000000000, 0.9807852804032304306, 1.000000000000000000, 0.9807852804032304306, 1.000000000000000000, 0.9807852804032304306, 1.000000000000000000, 0.9807852804032304306, 1.000000000000000000, 0.9807852804032304306, 1.000000000000000000, 0.9807852804032304306, 1.000000000000000000, 0.9807852804032304306, 1.000000000000000000, 0.9807852804032304306, 1.000000000000000000, 0.9807852804032304306, 1.000000000000000000, 0.9807852804032304306, 1.000000000000000000, 0.9807852804032304306, 1.000000000000000000, 0.9807852804032304306, 1.000000000000000000, 0.9807852804032304306, 1.000000000000000000, 0.9807852804032304306, 1.000000000000000000, 0.9807852804032304306, 1.000000000000000000, 0.9807852804032304306, 1.000000000000000000, 0.9807852804032304306, 1.000000000000000000, 0.9807852804032304306, 1.000000000000000000, 0.9807852804032304306, 1.000000000000000000, 0.9807852804032304306, 1.000000000000000000, 0.9807852804032304306, 1.000000000000000000, 0.9807852804032304306, 1.000000000000000000, 0.9807852804032304306, 1.000000000000000000, 0.9807852804032304306, 1.000000000000000000, 0.9807852804032304306, 1.000000000000000000, 0.9807852804032304306, 1.000000000000000000, 0.9807852804032304306, 1.000000000000000000, 0.9807852804032304306, 1.000000000000000000, 0.9807852804032304306, 1.000000000000000000, 0.9807852804032304306, 1.000000000000000000, 0.9807852804032304306, 1.000000000000000000, 0.9807852804032304306, 1.000000000000000000, 0.9807852804032304306, 1.000000000000000000, 0.9807852804032304306, 1.000000000000000000, 0.9807852804032304306, 1.000000000000000000, 0.9807852804032304306, 1.000000000000000000, 0.9807852804032304306, 1.000000000000000000, 0.9807852804032304306, 1.000000000000000000, 0.9807852804032304306, 1.000000000000000000, 0.9807852804032304306, 1.000000000000000000, 0.9807852804032304306, 1.000000000000000000, 0.9807852804032304306, 1.000000000000000000, 0.9807852804032304306, 1.000000000000000000, 0.9807852804032304306, 1.000000000000000000, 0.9807852804032304306, 1.000000000000000000, 0.9807852804032304306, 1.000000000000000000, 0.9807852804032304306, 1.000000000000000000, 0.9807852804032304306, 1.000000000000000000, 0.9807852804032304306, 1.000000000000000000, 0.9807852804032304306, 1.000000000000000000, 0.9807852804032304306, 1.000000000000000000, 0.9807852804032304306, 1.000000000000000000, 0.9807852804032304306, 1.000000000000000000, 0.9807852804032304306, 1.000000000000000000, 0.9807852804032304306, 1.000000000000000000, 0.9807852804032304306, 1.000000000000000000, 0.9807852804032304306, 1.000000000000000000, 0.9807852804032304306, 1.000000000000000000, 0.9807852804032304306, 1.000000000000000000, 0.9807852804032304306, 1.000000000000000000, 0.9807852804032304306, 1.000000000000000000, 0.9807852804032304306, 1.000000000000000000, 0.9807852804032304306, 1.000000000000000000, 0.9807852804032304306, 1.000000000000000000, 0.9807852804032304306, 1.000000000000000000, 0.9807852804032304306, 1.000000000000000000, 0.9807852804032304306, 1.000000000000000000, 0.9807852804032304306, 1.000000000000000000, 0.9807852804032304306, 1.000000000000000000, 0.9807852804032304306, 1.000000000000000000, 0.9807852804032304306, 1.000000000000000000, 0.9807852804032304306, 1.000000000000000000, 0.9807852804032304306, 1.000000000000000000, 0.9807852804032304306, 1.000000000000000000, 0.9807852804032304306, 1.000000000000000000, 0.9807852804032304306, 1.000000000000000000, 0.9807852804032304306, 1.000000000000000000, 0.9807852804032304306, 1.000000000000000000, 0.9807852804032304306, 1.000000000000000000, 0.9807852804032304306, 1.000000000000000000, 0.9807852804032304306, 1.000000000000000000, 0.9807852804032304306, 1.000000000000000000, 0.9807852804032304306, 1.000000000000000000, 0.9807852804032304306, 1.000000000000000000, 0.9807852804032304306, 1.000000000000000000, 0.9807852804032304306, 1.000000000000000000, 0.9807852804032304306, 1.000000000000000000, 0.9807852804032304306, 1.000000000000000000, 0.9807852804032304306, 1.000000000000000000, 0.9807852804032304306, 1.000000000000000000, 0.9807852804032304306, 1.000000000000000000, 0.9807852804032304306, 1.000000000000000000, 0.9807852804032304306, 1.000000000000000000, 0.9807852804032304306, 1.000000000000000000, 0.9807852804032304306, 1.000000000000000000, 0.9807852804032304306, 1.000000000000000000, 0.9807852804032304306, 1.000000000000000000, 0.9807852804032304306, 1.000000000000000000, 0.9807852804032304306, 1.000000000000000000, 0.9807852804032304306, 1.000000000000000000, 0.9807852804032304306, 1.000000000000000000, 0.9807852804032304306, 1.000000000000000000, 0.9807852804032304306, 1.000000000000000000, 0.9807852804032304306, 1.000000000000000000, 0.9807852804032304306, 1.000000000000000000, 0.9807852804032304306, 1.000000000000000000, 0.9807852804032304306, 1.000000000000000000, 0.9807852804032304306, 1.000000000000000000, 0.9807852804032304306, 1.000000000000000000, 0.9807852804032304306, 1.000000000000000000, 0.9807852804032304306, 1.000000000000000000, 0.9807852804032304306, 1.000000000000000000, 0.9807852804032304306, 1.000000000000000000, 0.9807852804032304306, 1.000000000000000000, 0.9807852804032304306, 1.000000000000000000, 0.9807852804032304306, 1.000000000000000000, 0.9807852804032304306, 1.000000000000000000, 0.9807852804032304306, 1.000000000000000000, 0.9807852804032304306, 1.000000000000000000, 0.9807852804032304306, 1.000000000000000000, 0.9807852804032304306, 1.000000000000000000, 0.9807852804032304306, 1.000000000000000000, 0.9807852804032304306, 1.000000000000000000, 0.9807852804032304306, 1.000000000000000000, 0.9807852804032304306, 1.000000000000000000, 0.9807852804032304306, 1.000000000000000000, 0.9807852804032304306, 1.000000000000000000, 0.9807852804032304306, 1.000000000000000000, 0.9807852804032304306, 1.000000000000000000, 0.9807852804032304306, 1.000000000000000000, 0.9807852804032304306, 1.000000000000000000, 0.9807852804032304306, 1.000000000000000000, 0.9807852804032304306, 1.000000000000000000, 0.9807852804032304306, 1.000000000000000000, 0.9807852804032304306, 1.000000000000000000, 0.9807852804032304306, 1.000000000000000000, 0.9807852804032304306, 1.000000000000000000, 0.9807852804032304306, 1.000000000000000000, 0.9807852804032304306, 1.000000000000000000, 0.9807852804032304306, 1.000000000000000000, 0.9807852804032304306, 1.000000000000000000, 0.9807852804032304306, 1.000000000000000000, 0.9807852804032304306, 1.000000000000000000, 0.9807852804032304306, 1.000000000000000000, 0.9807852804032304306, 1.000000000000000000, 0.9807852804032304306, 1.000000000000000000, 0.9807852804032304306, 1.000000000000000000, 0.9807852804032304306, 1.000000000000000000, 0.9807852804032304306, 1.000000000000000000, 0.9807852804032304306, 1.000000000000000000, 0.9807852804032304306, 1.000000000000000000, 0.9807852804032304306, 1.000000000000000000, 0.9807852804032304306, 1.000000000000000000, 0.9807852804032304306, 1.000000000000000000, 0.9807852804032304306, 1.000000000000000000, 0.9807852804032304306, 1.000000000000000000, 0.9807852804032304306, 1.000000000000000000, 0.9807852804032304306, 1.000000000000000000, 0.9807852804032304306, 1.000000000000000000, 0.9807852804032304306, 1.000000000000000000, 0.9807852804032304306, 1.000000000000000000, 0.9807852804032304306, 1.000000000000000000, 0.9807852804032304306, 1.000000000000000000, 0.9807852804032304306, 1.000000000000000000, 0.9807852804032304306, 1.000000000000000000, 0.9807852804032304306, 1.000000000000000000, 0.9807852804032304306, 1.000000000000000000, 0.9807852804032304306, 1.000000000000000000, 0.9807852804032304306, 1.000000000000000000, 0.9807852804032304306, 1.000000000000000000, 0.9807852804032304306, 1.000000000000000000, 0.9807852804032304306, 1.000000000000000000, 0.9807852804032304306, 1.000000000000000000, 0.9807852804032304306, 1.000000000000000000, 0.9807852804032304306, 1.000000000000000000, 0.9807852804032304306, 1.000000000000000000, 0.9807852804032304306, 1.000000000000000000, 0.9807852804032304306, 1.000000000000000000, 0.9807852804032304306, 1.000000000000000000, 0.9807852804032304306, 1.000000000000000000, 0.9807852804032304306, 1.000000000000000000, 0.9807852804032304306, 1.000000000000000000, 0.9807852804032304306, 1.000000000000000000, 0.9807852804032304306, 1.000000000000000000, 0.9807852804032304306, 1.000000000000000000, 0.9807852804032304306, 1.000000000000000000, 0.9807852804032304306, 1.000000000000000000, 0.9807852804032304306, 1.000000000000000000, 0.9807852804032304306, 1.000000000000000000, 0.9807852804032304306, 1.000000000000000000, 0.9807852804032304306, 1.000000000000000000, 0.9807852804032304306, 1.000000000000000000, 0.9807852804032304306, 1.000000000000000000, 0.9807852804032304306, 1.000000000000000000, 0.9807852804032304306, 1.000000000000000000, 0.9807852804032304306, 1.000000000000000000, 0.9807852804032304306, 1.000000000000000000, 0.9807852804032304306, 1.000000000000000000, 0.9807852804032304306, 1.000000000000000000, 0.9807852804032304306, 1.000000000000000000, 0.9807852804032304306, 1.000000000000000000, 0.9807852804032304306, 1.000000000000000000, 0.9807852804032304306, 1.000000000000000000, 0.9807852804032304306, 1.000000000000000000, 0.9807852804032304306, 1.000000000000000000, 0.9807852804032304306, 1.000000000000000000, 0.9807852804032304306, 1.000000000000000000, 0.9807852804032304306, 1.000000000000000000, 0.9807852804032304306, 1.000000000000000000, 0.9807852804032304306, 1.000000000000000000, 0.9807852804032304306, 1.000000000000000000, 0.9807852804032304306, 1.000000000000000000, 0.9807852804032304306, 1.000000000000000000, 0.9807852804032304306, 1.000000000000000000, 0.9807852804032304306, 1.000000000000000000, 0.9807852804032304306, 1.000000000000000000, 0.9807852804032304306, 1.000000000000000000, 0.9807852804032304306, 1.000000000000000000, 0.9807852804032304306, 1.000000000000000000, 0.9807852804032304306, 1.000000000000000000, 0.9807852804032304306, 1.000000000000000000, 0.9807852804032304306, 1.000000000000000000, 0.9807852804032304306, 1.000000000000000000, 0.9807852804032304306, 1.000000000000000000, 0.9807852804032304306, 1.000000000000000000, 0.9807852804032304306, 1.000000000000000000, 0.9807852804032304306, 1.000000000000000000, 0.9807852804032304306, 1.000000000000000000, 0.9807852804032304306, 1.000000000000000000, 0.9807852804032304306, 1.000000000000000000, 0.9807852804032304306, 1.000000000000000000, 0.9807852804032304306, 1.000000000000000000, 0.9807852804032304306, 1.000000000000000000, 0.9807852804032304306, 1.000000000000000000, 0.9807852804032304306, 1.000000000000000000, 0.9807852804032304306, 1.000000000000000000, 0.9807852804032304306, 1.000000000000000000, 0.9807852804032304306, 1.000000000000000000, 0.9807852804032304306, 1.000000000000000000, 0.9807852804032304306, 1.000000000000000000, 0.9807852804032304306, 1.000000000000000000, 0.9807852804032304306, 1.000000000000000000, 0.9807852804032304306, 1.000000000000000000, 0.9807852804032304306, 1.000000000000000000, 0.9807852804032304306, 1.000000000000000000, 0.9807852804032304306, 1.000000000000000000, 0.9807852804032304306, 1.000000000000000000, 0.9807852804032304306, 1.000000000000000000, 0.9807852804032304306, 1.000000000000000000, 0.9807852804032304306, 1.000000000000000000, 0.9807852804032304306, 1.000000000000000000, 0.9807852804032304306, 1.000000000000000000, 0.9807852804032304306, 1.000000000000000000, 0.9807852804032304306, 1.000000000000000000, 0.9807852804032304306, 1.000000000000000000, 0.9807852804032304306, 1.000000000000000000, 0.9807852804032304306, 1.000000000000000000, 0.9807852804032304306, 1.000000000000000000, 0.9807852804032304306, 1.000000000000000000, 0.9807852804032304306, 1.000000000000000000, 0.9807852804032304306, 1.000000000000000000, 0.9807852804032304306, 1.000000000000000000, 0.9807852804032304306, 1.000000000000000000, 0.9807852804032304306, 1.000000000000000000, 0.9807852804032304306, 1.000000000000000000, 0.9807852804032304306, 1.000000000000000000, 0.9807852804032304306, 1.000000000000000000, 0.9807852804032304306, 1.000000000000000000, 0.9807852804032304306, 1.000000000000000000, 0.9807852804032304306, 1.000000000000000000, 0.9807852804032304306, 1.000000000000000000, 0.9807852804032304306, 1.000000000000000000, 0.9807852804032304306, 1.000000000000000000, 0.9807852804032304306, 1.000000000000000000, 0.9807852804032304306, 1.000000000000000000, 0.9807852804032304306, 1.000000000000000000, 0.9807852804032304306, 1.000000000000000000, 0.9807852804032304306, 1.000000000000000000, 0.9807852804032304306, 1.000000000000000000, 0.9807852804032304306, 1.000000000000000000, 0.9807852804032304306, 1.000000000000000000, 0.9807852804032304306, 1.000000000000000000, 0.9807852804032304306, 1.000000000000000000, 0.9807852804032304306, 1.000000000000000000, 0.9807852804032304306, 1.000000000000000000, 0.9807852804032304306, 1.000000000000000000, 0.9807852804032304306, 1.000000000000000000, 0.9807852804032304306, 1.000000000000000000, 0.9807852804032304306, 1.000000000000000000, 0.9807852804032304306, 1.000000000000000000, 0.9807852804032304306, 1.000000000000000000, 0.9807852804032304306, 1.000000000000000000, 0.9807852804032304306, 1.000000000000000000, 0.9807852804032304306, 1.000000000000000000, 0.9807852804032304306, 1.000000000000000000, 0.9807852804032304306, 1.000000000000000000, 0.9807852804032304306, 1.000000000000000000, 0.9807852804032304306, 1.000000000000000000, 0.9807852804032304306, 1.000000000000000000, 0.9807852804032304306, 1.000000000000000000, 0.9807852804032304306, 1.000000000000000000, 0.9807852804032304306, 1.000000000000000000, 0.9807852804032304306, 1.000000000000000000, 0.9807852804032304306, 1.000000000000000000, 0.9807852804032304306, 1.000000000000000000, 0.9807852804032304306, 1.000000000000000000, 0.9807852804032304306, 1.000000000000000000, 0.9807852804032304306, 1.000000000000000000, 0.9807852804032304306, 1.000000000000000000, 0.9807852804032304306, 1.000000000000000000, 0.9807852804032304306, 1.000000000000000000, 0.9807852804032304306, 1.000000000000000000, 0.9807852804032304306, 1.000000000000000000, 0.9807852804032304306, 1.000000000000000000, 0.9807852804032304306, 1.000000000000000000, 0.9807852804032304306, 1.000000000000000000, 0.9807852804032304306, 1.000000000000000000, 0.9807852804032304306, 1.000000000000000000, 0.9807852804032304306, 1.000000000000000000, 0.9807852804032304306, 1.000000000000000000, 0.9807852804032304306, 1.000000000000000000, 0.9807852804032304306, 1.000000000000000000, 0.9807852804032304306, 1.000000000000000000, 0.9807852804032304306, 1.000000000000000000, 0.9807852804032304306, 1.000000000000000000, 0.9807852804032304306, 1.000000000000000000, 0.9807852804032304306, 1.000000000000000000, 0.9807852804032304306, 1.000000000000000000, 0.9807852804032304306, 1.000000000000000000, 0.9807852804032304306, 1.000000000000000000, 0.9807852804032304306, 1.000000000000000000, 0.9807852804032304306, 1.000000000000000000, 0.9807852804032304306, 1.000000000000000000, 0.9807852804032304306, 1.000000000000000000, 0.9807852804032304306, 1.000000000000000000, 0.9807852804032304306, 1.000000000000000000, 0.9807852804032304306, 1.000000000000000000, 0.9807852804032304306, 1.000000000000000000, 0.9807852804032304306, 1.000000000000000000, 0.9807852804032304306, 1.000000000000000000, 0.9807852804032304306, 1.000000000000000000, 0.9807852804032304306, 1.000000000000000000, 0.9807852804032304306, 1.000000000000000000, 0.9807852804032304306, 1.000000000000000000, 0.9807852804032304306, 1.000000000000000000, 0.9807852804032304306, 1.000000000000000000, 0.9807852804032304306, 1.000000000000000000, 0.9807852804032304306, 1.000000000000000000, 0.9807852804032304306, 1.000000000000000000, 0.9807852804032304306, 1.000000000000000000, 0.9807852804032304306, 1.000000000000000000, 0.9807852804032304306, 1.000000000000000000, 0.9807852804032304306, 1.000000000000000000, 0.9807852804032304306, 1.000000000000000000, 0.9807852804032304306, 1.000000000000000000, 0.9807852804032304306, 1.000000000000000000, 0.9807852804032304306, 1.000000000000000000, 0.9807852804032304306, 1.000000000000000000, 0.9807852804032304306, 1.000000000000000000, 0.9807852804032304306, 1.000000000000000000, 0.9807852804032304306, 1.000000000000000000, 0.9807852804032304306, 1.000000000000000000, 0.9807852804032304306, 1.000000000000000000, 0.9807852804032304306, 1.000000000000000000, 0.9807852804032304306, 1.000000000000000000, 0.9807852804032304306, 1.000000000000000000, 0.9807852804032304306, 1.000000000000000000, 0.9807852804032304306, 1.000000000000000000, 0.9807852804032304306, 1.000000000000000000, 0.9807852804032304306, 1.000000000000000000, 0.9807852804032304306, 1.000000000000000000, 0.9807852804032304306, 1.000000000000000000, 0.9807852804032304306, 1.000000000000000000, 0.9807852804032304306, 1.000000000000000000, 0.9807852804032304306, 1.000000000000000000, 0.9807852804032304306, 1.000000000000000000, 0.9807852804032304306, 1.000000000000000000, 0.9807852804032304306, 1.000000000000000000, 0.9807852804032304306, 1.000000000000000000, 0.9807852804032304306, 1.000000000000000000, 0.9807852804032304306, 1.000000000000000000, 0.9807852804032304306, 1.000000000000000000, 0.9807852804032304306, 1.000000000000000000, 0.9807852804032304306, 1.000000000000000000, 0.9807852804032304306, 1.000000000000000000, 0.9807852804032304306, 1.000000000000000000, 0.9807852804032304306, 1.000000000000000000, 0.9807852804032304306, 1.000000000000000000, 0.9807852804032304306, 1.000000000000000000, 0.9807852804032304306, 1.000000000000000000, 0.9807852804032304306, 1.000000000000000000, 0.9807852804032304306, 1.000000000000000000, 0.9807852804032304306, 1.000000000000000000, 0.9807852804032304306, 1.000000000000000000, 0.9807852804032304306, 1.000000000000000000, 0.9807852804032304306, 1.000000000000000000, 0.9807852804032304306, 1.000000000000000000, 0.9807852804032304306, 1.000000000000000000, 0.9807852804032304306, 1.000000000000000000, 0.9807852804032304306, 1.000000000000000000, 0.9807852804032304306, 1.000000000000000000, 0.9807852804032304306, 1.000000000000000000, 0.9807852804032304306, 1.000000000000000000, 0.9807852804032304306, 1.000000000000000000, 0.9807852804032304306, 1.000000000000000000, 0.9807852804032304306, 1.000000000000000000, 0.9807852804032304306, 1.000000000000000000, 0.9807852804032304306, 1.000000000000000000, 0.9807852804032304306, 1.000000000000000000, 0.9807852804032304306, 1.000000000000000000, 0.9807852804032304306, 1.000000000000000000, 0.9807852804032304306, 1.000000000000000000, 0.9807852804032304306, 1.000000000000000000, 0.9807852804032304306, 1.000000000000000000, 0.9807852804032304306, 1.000000000000000000, 0.9807852804032304306, 1.000000000000000000, 0.9807852804032304306, 1.000000000000000000, 0.9807852804032304306, 1.000000000000000000, 0.9807852804032304306, 1.000000000000000000, 0.9807852804032304306, 1.000000000000000000, 0.9807852804032304306, 1.000000000000000000, 0.9807852804032304306, 1.000000000000000000, 0.9807852804032304306, 1.000000000000000000, 0.9807852804032304306, 1.000000000000000000, 0.9807852804032304306, 1.000000000000000000, 0.9807852804032304306, 1.000000000000000000, 0.9807852804032304306, 1.000000000000000000, 0.9807852804032304306, 1.000000000000000000, 0.9807852804032304306, 1.000000000000000000, 0.9807852804032304306, 1.000000000000000000, 0.9807852804032304306, 1.000000000000000000, 0.9807852804032304306, 1.000000000000000000, 0.9807852804032304306, 1.000000000000000000, 0.9807852804032304306, 1.000000000000000000, 0.9807852804032304306, 1.000000000000000000, 0.9807852804032304306, 1.000000000000000000, 0.9807852804032304306, 1.000000000000000000, 0.9807852804032304306, 1.000000000000000000, 0.9807852804032304306, 1.000000000000000000, 0.9807852804032304306, 1.000000000000000000, 0.9807852804032304306, 1.000000000000000000, 0.9807852804032304306, 1.000000000000000000, 0.9807852804032304306, 1.000000000000000000, 0.9807852804032304306, 1.000000000000000000, 0.9807852804032304306, 1.000000000000000000, 0.9807852804032304306, 1.000000000000000000, 0.9807852804032304306, 1.000000000000000000, 0.9807852804032304306, 1.000000000000000000, 0.9807852804032304306, 1.000000000000000000, 0.9807852804032304306, 1.000000000000000000, 0.9807852804032304306, 1.000000000000000000, 0.9807852804032304306, 1.000000000000000000, 0.9807852804032304306, 1.000000000000000000, 0.9807852804032304306, 1.000000000000000000, 0.9807852804032304306, 1.000000000000000000, 0.9807852804032304306, 1.000000000000000000, 0.9807852804032304306, 1.000000000000000000, 0.9807852804032304306, 1.000000000000000000, 0.9807852804032304306, 1.000000000000000000, 0.9807852804032304306, 1.000000000000000000, 0.9807852804032304306, 1.000000000000000000, 0.9807852804032304306, 1.000000000000000000, 0.9807852804032304306, 1.000000000000000000, 0.9807852804032304306, 1.000000000000000000, 0.9807852804032304306, 1.000000000000000000, 0.9807852804032304306, 1.000000000000000000, 0.9807852804032304306, 1.000000000000000000, 0.9807852804032304306, 1.000000000000000000, 0.9807852804032304306, 1.000000000000000000, 0.9807852804032304306, 1.000000000000000000, 0.9807852804032304306, 1.000000000000000000, 0.9807852804032304306, 1.000000000000000000, 0.9807852804032304306, 1.000000000000000000, 0.9807852804032304306, 1.000000000000000000, 0.9807852804032304306, 1.000000000000000000, 0.9807852804032304306, 1.000000000000000000, 0.9807852804032304306, 1.000000000000000000, 0.9807852804032304306, 1.000000000000000000, 0.9807852804032304306, 1.000000000000000000, 0.9807852804032304306, 1.000000000000000000, 0.9807852804032304306, 1.000000000000000000, 0.9807852804032304306, 1.000000000000000000, 0.9807852804032304306, 1.000000000000000000, 0.9807852804032304306, 1.000000000000000000, 0.9807852804032304306, 1.000000000000000000, 0.9807852804032304306, 1.000000000000000000, 0.9935442612835747589, 0.9914265054520787768, 0.9914265054520787768, 0.9914265054520787768),
 ( 1.000000000000000000, 0.9807852804032304306, 1.000000000000000000, 0.9807852804032304306, 1.000000000000000000, 0.9807852804032304306, 1.000000000000000000, 0.9807852804032304306, 1.000000000000000000, 0.9807852804032304306, 1.000000000000000000, 0.9807852804032304306, 1.000000000000000000, 0.9807852804032304306, 1.000000000000000000, 0.9807852804032304306, 1.000000000000000000, 0.9807852804032304306, 1.000000000000000000, 0.9807852804032304306, 1.000000000000000000, 0.9807852804032304306, 1.000000000000000000, 0.9807852804032304306, 1.000000000000000000, 0.9807852804032304306, 1.000000000000000000, 0.9807852804032304306, 1.000000000000000000, 0.9807852804032304306, 1.000000000000000000, 0.9807852804032304306, 1.000000000000000000, 0.9807852804032304306, 1.000000000000000000, 0.9807852804032304306, 1.000000000000000000, 0.9807852804032304306, 1.000000000000000000, 0.9807852804032304306, 1.000000000000000000, 0.9807852804032304306, 1.000000000000000000, 0.9807852804032304306, 1.000000000000000000, 0.9807852804032304306, 1.000000000000000000, 0.9807852804032304306, 1.000000000000000000, 0.9807852804032304306, 1.000000000000000000, 0.9807852804032304306, 1.000000000000000000, 0.9807852804032304306, 1.000000000000000000, 0.9807852804032304306, 1.000000000000000000, 0.9807852804032304306, 1.000000000000000000, 0.9807852804032304306, 1.000000000000000000, 0.9807852804032304306, 1.000000000000000000, 0.9807852804032304306, 1.000000000000000000, 0.9807852804032304306, 1.000000000000000000, 0.9807852804032304306, 1.000000000000000000, 0.9807852804032304306, 1.000000000000000000, 0.9807852804032304306, 1.000000000000000000, 0.9807852804032304306, 1.000000000000000000, 0.9807852804032304306, 1.000000000000000000, 0.9807852804032304306, 1.000000000000000000, 0.9807852804032304306, 1.000000000000000000, 0.9807852804032304306, 1.000000000000000000, 0.9807852804032304306, 1.000000000000000000, 0.9807852804032304306, 1.000000000000000000, 0.9807852804032304306, 1.000000000000000000, 0.9807852804032304306, 1.000000000000000000, 0.9807852804032304306, 1.000000000000000000, 0.9807852804032304306, 1.000000000000000000, 0.9807852804032304306, 1.000000000000000000, 0.9807852804032304306, 1.000000000000000000, 0.9807852804032304306, 1.000000000000000000, 0.9807852804032304306, 1.000000000000000000, 0.9807852804032304306, 1.000000000000000000, 0.9807852804032304306, 1.000000000000000000, 0.9807852804032304306, 1.000000000000000000, 0.9807852804032304306, 1.000000000000000000, 0.9807852804032304306, 1.000000000000000000, 0.9807852804032304306, 1.000000000000000000, 0.9807852804032304306, 1.000000000000000000, 0.9807852804032304306, 1.000000000000000000, 0.9807852804032304306, 1.000000000000000000, 0.9807852804032304306, 1.000000000000000000, 0.9807852804032304306, 1.000000000000000000, 0.9807852804032304306, 1.000000000000000000, 0.9807852804032304306, 1.000000000000000000, 0.9807852804032304306, 1.000000000000000000, 0.9807852804032304306, 1.000000000000000000, 0.9807852804032304306, 1.000000000000000000, 0.9807852804032304306, 1.000000000000000000, 0.9807852804032304306, 1.000000000000000000, 0.9807852804032304306, 1.000000000000000000, 0.9807852804032304306, 1.000000000000000000, 0.9807852804032304306, 1.000000000000000000, 0.9807852804032304306, 1.000000000000000000, 0.9807852804032304306, 1.000000000000000000, 0.9807852804032304306, 1.000000000000000000, 0.9807852804032304306, 1.000000000000000000, 0.9807852804032304306, 1.000000000000000000, 0.9807852804032304306, 1.000000000000000000, 0.9807852804032304306, 1.000000000000000000, 0.9807852804032304306, 1.000000000000000000, 0.9807852804032304306, 1.000000000000000000, 0.9807852804032304306, 1.000000000000000000, 0.9807852804032304306, 1.000000000000000000, 0.9807852804032304306, 1.000000000000000000, 0.9807852804032304306, 1.000000000000000000, 0.9807852804032304306, 1.000000000000000000, 0.9807852804032304306, 1.000000000000000000, 0.9807852804032304306, 1.000000000000000000, 0.9807852804032304306, 1.000000000000000000, 0.9807852804032304306, 1.000000000000000000, 0.9807852804032304306, 1.000000000000000000, 0.9807852804032304306, 1.000000000000000000, 0.9807852804032304306, 1.000000000000000000, 0.9807852804032304306, 1.000000000000000000, 0.9807852804032304306, 1.000000000000000000, 0.9807852804032304306, 1.000000000000000000, 0.9807852804032304306, 1.000000000000000000, 0.9807852804032304306, 1.000000000000000000, 0.9807852804032304306, 1.000000000000000000, 0.9807852804032304306, 1.000000000000000000, 0.9807852804032304306, 1.000000000000000000, 0.9807852804032304306, 1.000000000000000000, 0.9807852804032304306, 1.000000000000000000, 0.9807852804032304306, 1.000000000000000000, 0.9807852804032304306, 1.000000000000000000, 0.9807852804032304306, 1.000000000000000000, 0.9807852804032304306, 1.000000000000000000, 0.9807852804032304306, 1.000000000000000000, 0.9807852804032304306, 1.000000000000000000, 0.9807852804032304306, 1.000000000000000000, 0.9807852804032304306, 1.000000000000000000, 0.9807852804032304306, 1.000000000000000000, 0.9807852804032304306, 1.000000000000000000, 0.9807852804032304306, 1.000000000000000000, 0.9807852804032304306, 1.000000000000000000, 0.9807852804032304306, 1.000000000000000000, 0.9807852804032304306, 1.000000000000000000, 0.9807852804032304306, 1.000000000000000000, 0.9807852804032304306, 1.000000000000000000, 0.9807852804032304306, 1.000000000000000000, 0.9807852804032304306, 1.000000000000000000, 0.9807852804032304306, 1.000000000000000000, 0.9807852804032304306, 1.000000000000000000, 0.9807852804032304306, 1.000000000000000000, 0.9807852804032304306, 1.000000000000000000, 0.9807852804032304306, 1.000000000000000000, 0.9807852804032304306, 1.000000000000000000, 0.9807852804032304306, 1.000000000000000000, 0.9807852804032304306, 1.000000000000000000, 0.9807852804032304306, 1.000000000000000000, 0.9807852804032304306, 1.000000000000000000, 0.9807852804032304306, 1.000000000000000000, 0.9807852804032304306, 1.000000000000000000, 0.9807852804032304306, 1.000000000000000000, 0.9807852804032304306, 1.000000000000000000, 0.9807852804032304306, 1.000000000000000000, 0.9807852804032304306, 1.000000000000000000, 0.9807852804032304306, 1.000000000000000000, 0.9807852804032304306, 1.000000000000000000, 0.9807852804032304306, 1.000000000000000000, 0.9807852804032304306, 1.000000000000000000, 0.9807852804032304306, 1.000000000000000000, 0.9807852804032304306, 1.000000000000000000, 0.9807852804032304306, 1.000000000000000000, 0.9807852804032304306, 1.000000000000000000, 0.9807852804032304306, 1.000000000000000000, 0.9807852804032304306, 1.000000000000000000, 0.9807852804032304306, 1.000000000000000000, 0.9807852804032304306, 1.000000000000000000, 0.9807852804032304306, 1.000000000000000000, 0.9807852804032304306, 1.000000000000000000, 0.9807852804032304306, 1.000000000000000000, 0.9807852804032304306, 1.000000000000000000, 0.9807852804032304306, 1.000000000000000000, 0.9807852804032304306, 1.000000000000000000, 0.9807852804032304306, 1.000000000000000000, 0.9807852804032304306, 1.000000000000000000, 0.9807852804032304306, 1.000000000000000000, 0.9807852804032304306, 1.000000000000000000, 0.9807852804032304306, 1.000000000000000000, 0.9807852804032304306, 1.000000000000000000, 0.9807852804032304306, 1.000000000000000000, 0.9807852804032304306, 1.000000000000000000, 0.9807852804032304306, 1.000000000000000000, 0.9807852804032304306, 1.000000000000000000, 0.9807852804032304306, 1.000000000000000000, 0.9807852804032304306, 1.000000000000000000, 0.9807852804032304306, 1.000000000000000000, 0.9807852804032304306, 1.000000000000000000, 0.9807852804032304306, 1.000000000000000000, 0.9807852804032304306, 1.000000000000000000, 0.9807852804032304306, 1.000000000000000000, 0.9807852804032304306, 1.000000000000000000, 0.9807852804032304306, 1.000000000000000000, 0.9807852804032304306, 1.000000000000000000, 0.9807852804032304306, 1.000000000000000000, 0.9807852804032304306, 1.000000000000000000, 0.9807852804032304306, 1.000000000000000000, 0.9807852804032304306, 1.000000000000000000, 0.9807852804032304306, 1.000000000000000000, 0.9807852804032304306, 1.000000000000000000, 0.9807852804032304306, 1.000000000000000000, 0.9807852804032304306, 1.000000000000000000, 0.9807852804032304306, 1.000000000000000000, 0.9807852804032304306, 1.000000000000000000, 0.9807852804032304306, 1.000000000000000000, 0.9807852804032304306, 1.000000000000000000, 0.9807852804032304306, 1.000000000000000000, 0.9807852804032304306, 1.000000000000000000, 0.9807852804032304306, 1.000000000000000000, 0.9807852804032304306, 1.000000000000000000, 0.9807852804032304306, 1.000000000000000000, 0.9807852804032304306, 1.000000000000000000, 0.9807852804032304306, 1.000000000000000000, 0.9807852804032304306, 1.000000000000000000, 0.9807852804032304306, 1.000000000000000000, 0.9807852804032304306, 1.000000000000000000, 0.9807852804032304306, 1.000000000000000000, 0.9807852804032304306, 1.000000000000000000, 0.9807852804032304306, 1.000000000000000000, 0.9807852804032304306, 1.000000000000000000, 0.9807852804032304306, 1.000000000000000000, 0.9807852804032304306, 1.000000000000000000, 0.9807852804032304306, 1.000000000000000000, 0.9807852804032304306, 1.000000000000000000, 0.9807852804032304306, 1.000000000000000000, 0.9807852804032304306, 1.000000000000000000, 0.9807852804032304306, 1.000000000000000000, 0.9807852804032304306, 1.000000000000000000, 0.9807852804032304306, 1.000000000000000000, 0.9807852804032304306, 1.000000000000000000, 0.9807852804032304306, 1.000000000000000000, 0.9807852804032304306, 1.000000000000000000, 0.9807852804032304306, 1.000000000000000000, 0.9807852804032304306, 1.000000000000000000, 0.9807852804032304306, 1.000000000000000000, 0.9807852804032304306, 1.000000000000000000, 0.9807852804032304306, 1.000000000000000000, 0.9807852804032304306, 1.000000000000000000, 0.9807852804032304306, 1.000000000000000000, 0.9807852804032304306, 1.000000000000000000, 0.9807852804032304306, 1.000000000000000000, 0.9807852804032304306, 1.000000000000000000, 0.9807852804032304306, 1.000000000000000000, 0.9807852804032304306, 1.000000000000000000, 0.9807852804032304306, 1.000000000000000000, 0.9807852804032304306, 1.000000000000000000, 0.9807852804032304306, 1.000000000000000000, 0.9807852804032304306, 1.000000000000000000, 0.9807852804032304306, 1.000000000000000000, 0.9807852804032304306, 1.000000000000000000, 0.9807852804032304306, 1.000000000000000000, 0.9807852804032304306, 1.000000000000000000, 0.9807852804032304306, 1.000000000000000000, 0.9807852804032304306, 1.000000000000000000, 0.9807852804032304306, 1.000000000000000000, 0.9807852804032304306, 1.000000000000000000, 0.9807852804032304306, 1.000000000000000000, 0.9807852804032304306, 1.000000000000000000, 0.9807852804032304306, 1.000000000000000000, 0.9807852804032304306, 1.000000000000000000, 0.9807852804032304306, 1.000000000000000000, 0.9807852804032304306, 1.000000000000000000, 0.9807852804032304306, 1.000000000000000000, 0.9807852804032304306, 1.000000000000000000, 0.9807852804032304306, 1.000000000000000000, 0.9807852804032304306, 1.000000000000000000, 0.9807852804032304306, 1.000000000000000000, 0.9807852804032304306, 1.000000000000000000, 0.9807852804032304306, 1.000000000000000000, 0.9807852804032304306, 1.000000000000000000, 0.9807852804032304306, 1.000000000000000000, 0.9807852804032304306, 1.000000000000000000, 0.9807852804032304306, 1.000000000000000000, 0.9807852804032304306, 1.000000000000000000, 0.9807852804032304306, 1.000000000000000000, 0.9807852804032304306, 1.000000000000000000, 0.9807852804032304306, 1.000000000000000000, 0.9807852804032304306, 1.000000000000000000, 0.9807852804032304306, 1.000000000000000000, 0.9807852804032304306, 1.000000000000000000, 0.9807852804032304306, 1.000000000000000000, 0.9807852804032304306, 1.000000000000000000, 0.9807852804032304306, 1.000000000000000000, 0.9807852804032304306, 1.000000000000000000, 0.9807852804032304306, 1.000000000000000000, 0.9807852804032304306, 1.000000000000000000, 0.9807852804032304306, 1.000000000000000000, 0.9807852804032304306, 1.000000000000000000, 0.9807852804032304306, 1.000000000000000000, 0.9807852804032304306, 1.000000000000000000, 0.9807852804032304306, 1.000000000000000000, 0.9807852804032304306, 1.000000000000000000, 0.9807852804032304306, 1.000000000000000000, 0.9807852804032304306, 1.000000000000000000, 0.9807852804032304306, 1.000000000000000000, 0.9807852804032304306, 1.000000000000000000, 0.9807852804032304306, 1.000000000000000000, 0.9807852804032304306, 1.000000000000000000, 0.9807852804032304306, 1.000000000000000000, 0.9807852804032304306, 1.000000000000000000, 0.9807852804032304306, 1.000000000000000000, 0.9807852804032304306, 1.000000000000000000, 0.9807852804032304306, 1.000000000000000000, 0.9807852804032304306, 1.000000000000000000, 0.9807852804032304306, 1.000000000000000000, 0.9807852804032304306, 1.000000000000000000, 0.9807852804032304306, 1.000000000000000000, 0.9807852804032304306, 1.000000000000000000, 0.9807852804032304306, 1.000000000000000000, 0.9807852804032304306, 1.000000000000000000, 0.9807852804032304306, 1.000000000000000000, 0.9807852804032304306, 1.000000000000000000, 0.9807852804032304306, 1.000000000000000000, 0.9807852804032304306, 1.000000000000000000, 0.9807852804032304306, 1.000000000000000000, 0.9807852804032304306, 1.000000000000000000, 0.9807852804032304306, 1.000000000000000000, 0.9807852804032304306, 1.000000000000000000, 0.9807852804032304306, 1.000000000000000000, 0.9807852804032304306, 1.000000000000000000, 0.9807852804032304306, 1.000000000000000000, 0.9807852804032304306, 1.000000000000000000, 0.9807852804032304306, 1.000000000000000000, 0.9807852804032304306, 1.000000000000000000, 0.9807852804032304306, 1.000000000000000000, 0.9807852804032304306, 1.000000000000000000, 0.9807852804032304306, 1.000000000000000000, 0.9807852804032304306, 1.000000000000000000, 0.9807852804032304306, 1.000000000000000000, 0.9807852804032304306, 1.000000000000000000, 0.9807852804032304306, 1.000000000000000000, 0.9807852804032304306, 1.000000000000000000, 0.9807852804032304306, 1.000000000000000000, 0.9807852804032304306, 1.000000000000000000, 0.9807852804032304306, 1.000000000000000000, 0.9807852804032304306, 1.000000000000000000, 0.9807852804032304306, 1.000000000000000000, 0.9807852804032304306, 1.000000000000000000, 0.9807852804032304306, 1.000000000000000000, 0.9807852804032304306, 1.000000000000000000, 0.9807852804032304306, 1.000000000000000000, 0.9807852804032304306, 1.000000000000000000, 0.9807852804032304306, 1.000000000000000000, 0.9807852804032304306, 1.000000000000000000, 0.9807852804032304306, 1.000000000000000000, 0.9807852804032304306, 1.000000000000000000, 0.9807852804032304306, 1.000000000000000000, 0.9807852804032304306, 1.000000000000000000, 0.9807852804032304306, 1.000000000000000000, 0.9807852804032304306, 1.000000000000000000, 0.9807852804032304306, 1.000000000000000000, 0.9807852804032304306, 1.000000000000000000, 0.9807852804032304306, 1.000000000000000000, 0.9807852804032304306, 1.000000000000000000, 0.9807852804032304306, 1.000000000000000000, 0.9807852804032304306, 1.000000000000000000, 0.9807852804032304306, 1.000000000000000000, 0.9807852804032304306, 1.000000000000000000, 0.9807852804032304306, 1.000000000000000000, 0.9807852804032304306, 1.000000000000000000, 0.9807852804032304306, 1.000000000000000000, 0.9807852804032304306, 1.000000000000000000, 0.9807852804032304306, 1.000000000000000000, 0.9807852804032304306, 1.000000000000000000, 0.9807852804032304306, 1.000000000000000000, 0.9807852804032304306, 1.000000000000000000, 0.9807852804032304306, 1.000000000000000000, 0.9807852804032304306, 1.000000000000000000, 0.9807852804032304306, 1.000000000000000000, 0.9807852804032304306, 1.000000000000000000, 0.9807852804032304306, 1.000000000000000000, 0.9807852804032304306, 1.000000000000000000, 0.9807852804032304306, 1.000000000000000000, 0.9807852804032304306, 1.000000000000000000, 0.9807852804032304306, 1.000000000000000000, 0.9807852804032304306, 1.000000000000000000, 0.9807852804032304306, 1.000000000000000000, 0.9807852804032304306, 1.000000000000000000, 0.9807852804032304306, 1.000000000000000000, 0.9807852804032304306, 1.000000000000000000, 0.9807852804032304306, 1.000000000000000000, 0.9807852804032304306, 1.000000000000000000, 0.9807852804032304306, 1.000000000000000000, 0.9807852804032304306, 1.000000000000000000, 0.9807852804032304306, 1.000000000000000000, 0.9807852804032304306, 1.000000000000000000, 0.9807852804032304306, 1.000000000000000000, 0.9807852804032304306, 1.000000000000000000, 0.9807852804032304306, 1.000000000000000000, 0.9807852804032304306, 1.000000000000000000, 0.9807852804032304306, 1.000000000000000000, 0.9807852804032304306, 1.000000000000000000, 0.9807852804032304306, 1.000000000000000000, 0.9807852804032304306, 1.000000000000000000, 0.9807852804032304306, 1.000000000000000000, 0.9807852804032304306, 1.000000000000000000, 0.9807852804032304306, 1.000000000000000000, 0.9807852804032304306, 1.000000000000000000, 0.9807852804032304306, 1.000000000000000000, 0.9807852804032304306, 1.000000000000000000, 0.9807852804032304306, 1.000000000000000000, 0.9807852804032304306, 1.000000000000000000, 0.9807852804032304306, 1.000000000000000000, 0.9807852804032304306, 1.000000000000000000, 0.9807852804032304306, 1.000000000000000000, 0.9807852804032304306, 1.000000000000000000, 0.9807852804032304306, 1.000000000000000000, 0.9807852804032304306, 1.000000000000000000, 0.9807852804032304306, 1.000000000000000000, 0.9807852804032304306, 1.000000000000000000, 0.9807852804032304306, 1.000000000000000000, 0.9807852804032304306, 1.000000000000000000, 0.9807852804032304306, 1.000000000000000000, 0.9807852804032304306, 1.000000000000000000, 0.9807852804032304306, 1.000000000000000000, 0.9807852804032304306, 1.000000000000000000, 0.9807852804032304306, 1.000000000000000000, 0.9807852804032304306, 1.000000000000000000, 0.9807852804032304306, 1.000000000000000000, 0.9807852804032304306, 1.000000000000000000, 0.9807852804032304306, 1.000000000000000000, 0.9807852804032304306, 1.000000000000000000, 0.9807852804032304306, 1.000000000000000000, 0.9807852804032304306, 1.000000000000000000, 0.9807852804032304306, 1.000000000000000000, 0.9807852804032304306, 1.000000000000000000, 0.9807852804032304306, 1.000000000000000000, 0.9807852804032304306, 1.000000000000000000, 0.9807852804032304306, 1.000000000000000000, 0.9807852804032304306, 1.000000000000000000, 0.9807852804032304306, 1.000000000000000000, 0.9807852804032304306, 1.000000000000000000, 0.9807852804032304306, 1.000000000000000000, 0.9807852804032304306, 1.000000000000000000, 0.9807852804032304306, 1.000000000000000000, 0.9807852804032304306, 1.000000000000000000, 0.9807852804032304306, 1.000000000000000000, 0.9807852804032304306, 1.000000000000000000, 0.9807852804032304306, 1.000000000000000000, 0.9807852804032304306, 1.000000000000000000, 0.9807852804032304306, 1.000000000000000000, 0.9807852804032304306, 1.000000000000000000, 0.9807852804032304306, 1.000000000000000000, 0.9807852804032304306, 1.000000000000000000, 0.9807852804032304306, 1.000000000000000000, 0.9807852804032304306, 1.000000000000000000, 0.9807852804032304306, 1.000000000000000000, 0.9807852804032304306, 1.000000000000000000, 0.9807852804032304306, 1.000000000000000000, 0.9807852804032304306, 1.000000000000000000, 0.9807852804032304306, 1.000000000000000000, 0.9807852804032304306, 1.000000000000000000, 0.9807852804032304306, 1.000000000000000000, 0.9807852804032304306, 1.000000000000000000, 0.9807852804032304306, 1.000000000000000000, 0.9807852804032304306, 1.000000000000000000, 0.9807852804032304306, 1.000000000000000000, 0.9807852804032304306, 1.000000000000000000, 0.9807852804032304306, 1.000000000000000000, 0.9807852804032304306, 1.000000000000000000, 0.9807852804032304306, 1.000000000000000000, 0.9807852804032304306, 1.000000000000000000, 0.9807852804032304306, 1.000000000000000000, 0.9807852804032304306, 1.000000000000000000, 0.9807852804032304306, 1.000000000000000000, 0.9807852804032304306, 1.000000000000000000, 0.9807852804032304306, 1.000000000000000000, 0.9807852804032304306, 1.000000000000000000, 0.9807852804032304306, 1.000000000000000000, 0.9807852804032304306, 1.000000000000000000, 0.9807852804032304306, 1.000000000000000000, 0.9807852804032304306, 1.000000000000000000, 0.9807852804032304306, 1.000000000000000000, 0.9807852804032304306, 1.000000000000000000, 0.9807852804032304306, 1.000000000000000000, 0.9807852804032304306, 1.000000000000000000, 0.9807852804032304306, 1.000000000000000000, 0.9807852804032304306, 1.000000000000000000, 0.9807852804032304306, 1.000000000000000000, 0.9807852804032304306, 1.000000000000000000, 0.9807852804032304306, 1.000000000000000000, 0.9807852804032304306, 1.000000000000000000, 0.9807852804032304306, 1.000000000000000000, 0.9807852804032304306, 1.000000000000000000, 0.9807852804032304306, 1.000000000000000000, 0.9807852804032304306, 1.000000000000000000, 0.9807852804032304306, 1.000000000000000000, 0.9807852804032304306, 1.000000000000000000, 0.9807852804032304306, 1.000000000000000000, 0.9807852804032304306, 1.000000000000000000, 0.9807852804032304306, 1.000000000000000000, 0.9807852804032304306, 1.000000000000000000, 0.9807852804032304306, 1.000000000000000000, 0.9807852804032304306, 1.000000000000000000, 0.9807852804032304306, 1.000000000000000000, 0.9807852804032304306, 1.000000000000000000, 0.9807852804032304306, 1.000000000000000000, 0.9807852804032304306, 1.000000000000000000, 0.9807852804032304306, 1.000000000000000000, 0.9807852804032304306, 1.000000000000000000, 0.9807852804032304306, 1.000000000000000000, 0.9807852804032304306, 1.000000000000000000, 0.9807852804032304306, 1.000000000000000000, 0.9807852804032304306, 1.000000000000000000, 0.9807852804032304306, 1.000000000000000000, 0.9807852804032304306, 1.000000000000000000, 0.9807852804032304306, 1.000000000000000000, 0.9807852804032304306, 1.000000000000000000, 0.9807852804032304306, 1.000000000000000000, 0.9807852804032304306, 1.000000000000000000, 0.9807852804032304306, 1.000000000000000000, 0.9807852804032304306, 1.000000000000000000, 0.9807852804032304306, 1.000000000000000000, 0.9807852804032304306, 1.000000000000000000, 0.9807852804032304306, 1.000000000000000000, 0.9807852804032304306, 1.000000000000000000, 0.9807852804032304306, 1.000000000000000000, 0.9807852804032304306, 1.000000000000000000, 0.9807852804032304306, 1.000000000000000000, 0.9807852804032304306, 1.000000000000000000, 0.9935442612835747589, 0.9914265054520787768, 0.9914265054520787768, 0.9914265054520787768) ) ) 
 REPRESENTATION_ITEM ( '' )  SURFACE ( )  );
#18662=CARTESIAN_POINT ( 'NONE',  ( -35.09675569278793716, 267.2448905683720568, 15.47720386886985366 ) ) ;
#18666=CARTESIAN_POINT ( 'NONE',  ( -11.93348319268873503, 480.3698905683720568, -2.051577885510841163E-15 ) ) ;
#18670=DIRECTION ( 'NONE',  ( -1.000000000000000000, 0.000000000000000000, 0.000000000000000000 ) ) ;
#18671=CARTESIAN_POINT ( 'NONE',  ( -22.27502019258947286, 250.7448905683720000, -15.47720386886985544 ) ) ;
#18674=EDGE_CURVE ( 'NONE', #7167, #16774, #7455, .T. ) ;
#18675=CARTESIAN_POINT ( 'NONE',  ( -14.48388495494898898, 271.3073905683721136, -9.489475012073734561 ) ) ;
#18676=CARTESIAN_POINT ( 'NONE',  ( -36.33955658999052929, 473.8698905765656377, 18.47759065022572500 ) ) ;
#18677=CARTESIAN_POINT ( 'NONE',  ( -17.35679799567829207, 390.6823905601785327, 16.95518130045146421 ) ) ;
#18678=CARTESIAN_POINT ( 'NONE',  ( -13.20868407381884602, 239.7448905683720000, 6.410867750099229490 ) ) ;
#18680=CARTESIAN_POINT ( 'NONE',  ( -45.43829269268872650, 525.0573905683720568, -3.332260488124726194 ) ) ;
#18681=CARTESIAN_POINT ( 'NONE',  ( -10.20829729246298712, 376.3698905765656377, 7.653668647301790529 ) ) ;
#18682=CARTESIAN_POINT ( 'NONE',  ( -28.68588794268869790, 246.3698905683720000, 16.75240474999999307 ) ) ;
#18683=CARTESIAN_POINT ( 'NONE',  ( -40.53162694259543741, 364.1198905683720000, -11.84573899990672707 ) ) ;
#18687=EDGE_CURVE ( 'NONE', #19193, #1608, #7913, .T. ) ;
#18688=CARTESIAN_POINT ( 'NONE',  ( -32.01814843081345430, 396.0573905683720568, 16.75240474999999307 ) ) ;
#18690=CARTESIAN_POINT ( 'NONE',  ( -17.35679799567830628, 413.8073905601785327, -16.95518130045146421 ) ) ;
#18694=ORIENTED_EDGE ( 'NONE', *, *, #10365, .F. ) ;
#18695=CARTESIAN_POINT ( 'NONE',  ( -32.01814843081346851, 517.5573905683720568, 16.75240474999999307 ) ) ;
#18696=CARTESIAN_POINT ( 'NONE',  ( -24.70764059509554045, 290.0573905601785327, 19.99999999999998934 ) ) ;
#18700=CARTESIAN_POINT ( 'NONE',  ( -28.68588794268870856, 327.8698905683720000, 16.75240474999999307 ) ) ;
#18702=CARTESIAN_POINT ( 'NONE',  ( -25.35362745456398059, 346.6823905683720568, 16.75240474999998952 ) ) ;
#18703=CARTESIAN_POINT ( 'NONE',  ( -38.17536295476245556, 372.3073905683721136, -14.20200298773971426 ) ) ;
#18704=CARTESIAN_POINT ( 'NONE',  ( -10.20829729246297646, 287.6198905765656377, -7.653668647301794969 ) ) ;
#18706=CARTESIAN_POINT ( 'NONE',  ( -35.09675569278793716, 271.9948905683720000, -15.47720386886985544 ) ) ;
#18708=CARTESIAN_POINT ( 'NONE',  ( -28.68588794268871922, 407.8698905683720568, 16.75240474999999307 ) ) ;
#18709=CARTESIAN_POINT ( 'NONE',  ( -8.685887942688742314, 573.2448905601785327, 2.449293598294706119E-15 ) ) ;
#18710=CARTESIAN_POINT ( 'NONE',  ( -47.16347859291444422, 356.6198905601784759, -7.653668647301793193 ) ) ;
#18712=CARTESIAN_POINT ( 'NONE',  ( -42.88789093042843348, 334.4323905683720568, -9.489475012073736337 ) ) ;
#18713=CARTESIAN_POINT ( 'NONE',  ( -28.68588794268872988, 461.3698905683720000, -16.75240474999999307 ) ) ;
#18716=CARTESIAN_POINT ( 'NONE',  ( -17.35679799567830983, 463.8073905601784759, -16.95518130045146421 ) ) ;
#18717=CARTESIAN_POINT ( 'NONE',  ( -19.19641293061497933, 290.4323905683720000, -14.20200298773971603 ) ) ;
#18721=CARTESIAN_POINT ( 'NONE',  ( -48.68588794268870856, 347.2448905601784759, 0.000000000000000000 ) ) ;
#18722=( BOUNDED_CURVE ( )  B_SPLINE_CURVE ( 2, ( #837, #5572, #16661, #725, #8816, #9027, #7402, #620, #4058, #18259, #17159, #9926, #15651, #3450, #14028, #7295, #3346 ),
 .UNSPECIFIED., .F., .T. ) 
 B_SPLINE_CURVE_WITH_KNOTS ( ( 3, 2, 2, 2, 2, 2, 2, 2, 3 ),
 ( 0.8437500000000002220, 0.8457031250000002220, 0.8476562500000002220, 0.8496093750000002220, 0.8515625000000002220, 0.8535156250000002220, 0.8554687500000002220, 0.8574218750000002220, 0.8593750000000002220 ),
 .UNSPECIFIED. ) 
 CURVE ( )  GEOMETRIC_REPRESENTATION_ITEM ( )  RATIONAL_B_SPLINE_CURVE ( ( 0.9999999999999977796, 0.9807852804032326510, 1.000000000000000000, 0.9807852804032304306, 1.000000000000000000, 0.9807852804032304306, 1.000000000000000000, 0.9807852804032304306, 1.000000000000000000, 0.9807852804032304306, 1.000000000000000000, 0.9807852804032304306, 1.000000000000000000, 0.9807852804032304306, 1.000000000000000000, 0.9807852804032282101, 1.000000000000002220 ) ) 
 REPRESENTATION_ITEM ( '' )  );
#18723=CARTESIAN_POINT ( 'NONE',  ( -44.16309181155855867, 304.4948905683720568, 6.410867750099241924 ) ) ;
#18724=CARTESIAN_POINT ( 'NONE',  ( -25.35362745456398414, 378.1823905683721136, 16.75240474999998952 ) ) ;
#18725=CARTESIAN_POINT ( 'NONE',  ( -10.20829729246298712, 372.8698905601784759, -7.653668647301794969 ) ) ;
#18726=CARTESIAN_POINT ( 'NONE',  ( -28.68588794268873698, 529.4948905765655809, -19.99999999999999289 ) ) ;
#18727=CARTESIAN_POINT ( 'NONE',  ( -44.16309181155857289, 404.4948905683720000, 6.410867750099241924 ) ) ;
#18728=CARTESIAN_POINT ( 'NONE',  ( -38.17536295476244135, 253.8073905683720568, -14.20200298773971426 ) ) ;
#18731=CARTESIAN_POINT ( 'NONE',  ( -42.88789093042844058, 422.9323905683720000, -9.489475012073734561 ) ) ;
#18734=CARTESIAN_POINT ( 'NONE',  ( -32.66413529028187668, 344.1823905765656377, 19.99999999999999289 ) ) ;
#18736=CARTESIAN_POINT ( 'NONE',  ( -45.43829269268870519, 323.5573905683720000, -3.332260488124726638 ) ) ;
#18737=CARTESIAN_POINT ( 'NONE',  ( -28.68588794268872988, 482.8698905683720568, -16.75240474999999307 ) ) ;
#18739=CARTESIAN_POINT ( 'NONE',  ( -28.68588794268874054, 573.2448905601785327, 0.000000000000000000 ) ) ;
#18740=CARTESIAN_POINT ( 'NONE',  ( -36.33955658999050087, 305.3698905601784759, -18.47759065022572855 ) ) ;
#18741=CARTESIAN_POINT ( 'NONE',  ( -25.35362745456398414, 378.1823905683720568, 16.75240474999998952 ) ) ;
#18744=CARTESIAN_POINT ( 'NONE',  ( -47.16347859291446554, 517.8698905601785327, 7.653668647301805628 ) ) ;
#18745=CARTESIAN_POINT ( 'NONE',  ( -19.19641293061498644, 350.4323905683720000, -14.20200298773971603 ) ) ;
#18747=CARTESIAN_POINT ( 'NONE',  ( -42.88789093042844769, 502.9323905683720000, -9.489475012073736337 ) ) ;
#18748=ORIENTED_EDGE ( 'NONE', *, *, #14701, .T. ) ;
#18749=CARTESIAN_POINT ( 'NONE',  ( -36.33955658999051508, 349.1198905601784759, 18.47759065022572500 ) ) ;
#18750=CARTESIAN_POINT ( 'NONE',  ( -24.70764059509556176, 379.1823905765656377, -19.99999999999999289 ) ) ;
#18752=CARTESIAN_POINT ( 'NONE',  ( -48.68588794268870856, 377.2448905601784759, 0.000000000000000000 ) ) ;
#18753=FACE_OUTER_BOUND ( 'NONE', #3902, .T. ) ;
#18754=CARTESIAN_POINT ( 'NONE',  ( -32.01814843081346140, 456.0573905683720000, 16.75240474999999307 ) ) ;
#18756=CARTESIAN_POINT ( 'NONE',  ( -40.53162694259545162, 495.1198905683720000, 11.84573899990672885 ) ) ;
#18757=CARTESIAN_POINT ( 'NONE',  ( -48.68588794268872277, 487.2448905601784759, 0.000000000000000000 ) ) ;
#18759=CARTESIAN_POINT ( 'NONE',  ( -8.685887942688726326, 407.3073905765656377, -3.978247347593165895 ) ) ;
#18761=CARTESIAN_POINT ( 'NONE',  ( -48.68588794268870146, 297.2448905601784759, 0.000000000000000000 ) ) ;
#18762=CARTESIAN_POINT ( 'NONE',  ( -40.01497788969915348, 485.6823905601785327, -16.95518130045146421 ) ) ;
#18765=CARTESIAN_POINT ( 'NONE',  ( -17.35679799567830273, 433.8073905601784759, -16.95518130045146421 ) ) ;
#18767=CARTESIAN_POINT ( 'NONE',  ( -40.53162694259543031, 284.1198905683720000, -11.84573899990672707 ) ) ;
#18768=CARTESIAN_POINT ( 'NONE',  ( -48.68588794268869435, 247.2448905601785043, 0.000000000000000000 ) ) ;
#18769=CARTESIAN_POINT ( 'NONE',  ( -42.82802356641965957, 363.2448905765656377, 14.14213562373094923 ) ) ;
#18770=CARTESIAN_POINT ( 'NONE',  ( -38.17536295476246266, 443.8073905683720568, -14.20200298773971426 ) ) ;
#18771=CARTESIAN_POINT ( 'NONE',  ( -48.68588794268854514, 331.6823905765656377, -3.978247347593583783 ) ) ;
#18772=CARTESIAN_POINT ( 'NONE',  ( -19.19641293061497578, 261.9323905683720568, -14.20200298773971603 ) ) ;
#18773=VECTOR ( 'NONE', #13905, 1000.000000000000000 ) ;
#18775=CARTESIAN_POINT ( 'NONE',  ( -13.20868407381887444, 489.7448905683720568, 6.410867750099229490 ) ) ;
#18781=CARTESIAN_POINT ( 'NONE',  ( -14.48388495494898542, 249.8073905683720568, -9.489475012073736337 ) ) ;
#18784=CARTESIAN_POINT ( 'NONE',  ( -14.54375231895778420, 478.2448905765655809, -14.14213562373094746 ) ) ;
#18786=CARTESIAN_POINT ( 'NONE',  ( -24.39804996317073105, 223.9102039777117739, -18.69641520486996100 ) ) ;
#18787=CARTESIAN_POINT ( 'NONE',  ( -28.68588794268870146, 242.8698905683720568, -16.75240474999999307 ) ) ;
#18788=CARTESIAN_POINT ( 'NONE',  ( -45.43829269268872650, 515.0573905683720568, -3.332260488124726194 ) ) ;
#18790=CARTESIAN_POINT ( 'NONE',  ( -38.17536295476243424, 245.4323905683720000, 14.20200298773971781 ) ) ;
#18791=( BOUNDED_CURVE ( )  B_SPLINE_CURVE ( 2, ( #17015, #18940, #15612, #8671, #12353, #2197, #16910, #7365, #4017, #19058, #4125, #20254, #8782, #10711, #3913, #15295, #12460 ),
 .UNSPECIFIED., .F., .T. ) 
 B_SPLINE_CURVE_WITH_KNOTS ( ( 3, 2, 2, 2, 2, 2, 2, 2, 3 ),
 ( 0.7500000000000001110, 0.7519531250000001110, 0.7539062500000001110, 0.7558593750000001110, 0.7578125000000001110, 0.7597656250000001110, 0.7617187500000001110, 0.7636718750000001110, 0.7656250000000001110 ),
 .UNSPECIFIED. ) 
 CURVE ( )  GEOMETRIC_REPRESENTATION_ITEM ( )  RATIONAL_B_SPLINE_CURVE ( ( 0.9999999999999988898, 0.9807852804032315408, 1.000000000000000000, 0.9807852804032304306, 1.000000000000000000, 0.9807852804032304306, 1.000000000000000000, 0.9807852804032304306, 1.000000000000000000, 0.9807852804032304306, 1.000000000000000000, 0.9807852804032304306, 1.000000000000000000, 0.9807852804032304306, 1.000000000000000000, 0.9807852804032293204, 1.000000000000001110 ) ) 
 REPRESENTATION_ITEM ( '' )  );
#18793=CARTESIAN_POINT ( 'NONE',  ( -40.53162694259543741, 346.6198905683720000, 11.84573899990672885 ) ) ;
#18795=EDGE_CURVE ( 'NONE', #3515, #19311, #2570, .T. ) ;
#18796=CARTESIAN_POINT ( 'NONE',  ( -32.01814843081345430, 411.6823905683720568, -16.75240474999999307 ) ) ;
#18798=CARTESIAN_POINT ( 'NONE',  ( -14.54375231895776821, 380.9948905601784759, 14.14213562373094568 ) ) ;
#18799=VERTEX_POINT ( 'NONE', #17737 ) ;
#18802=VERTEX_POINT ( 'NONE', #18927 ) ;
#18803=CARTESIAN_POINT ( 'NONE',  ( -22.27502019258950128, 512.2448905683720568, -15.47720386886985544 ) ) ;
#18804=CARTESIAN_POINT ( 'NONE',  ( -43.20801099888741703, 208.4516271390267548, -3.763513762345671143 ) ) ;
#18805=VERTEX_POINT ( 'NONE', #2929 ) ;
#18806=CARTESIAN_POINT ( 'NONE',  ( -42.88789093042842637, 306.3073905683720000, 9.489475012073734561 ) ) ;
#18808=CARTESIAN_POINT ( 'NONE',  ( -35.09675569278794427, 341.9948905683720000, -15.47720386886985544 ) ) ;
#18809=CARTESIAN_POINT ( 'NONE',  ( -35.09675569278794427, 351.9948905683720000, -15.47720386886985544 ) ) ;
#18811=CARTESIAN_POINT ( 'NONE',  ( -24.70764059509554045, 284.8073905765655809, 19.99999999999998934 ) ) ;
#18812=CARTESIAN_POINT ( 'NONE',  ( -10.20829729246300310, 497.6198905765656377, -7.653668647301794969 ) ) ;
#18813=CARTESIAN_POINT ( 'NONE',  ( -44.16309181155855157, 254.4948905683720568, 6.410867750099241924 ) ) ;
#18814=CARTESIAN_POINT ( 'NONE',  ( -45.64106924314016567, 226.3073905601784759, -11.32908994701042538 ) ) ;
#18815=CARTESIAN_POINT ( 'NONE',  ( -40.53162694259544452, 404.1198905683720000, -11.84573899990672707 ) ) ;
#18816=CARTESIAN_POINT ( 'NONE',  ( -8.685887942688541585, 332.5573905601783622, -3.978247347592740013 ) ) ;
#18817=CARTESIAN_POINT ( 'NONE',  ( -24.70764059509556532, 504.8073905765656377, 19.99999999999998934 ) ) ;
#18820=CARTESIAN_POINT ( 'NONE',  ( -38.17536295476244135, 306.9323905683719431, 14.20200298773971781 ) ) ;
#18821=CARTESIAN_POINT ( 'NONE',  ( -22.27502019258949062, 466.9948905683720000, 15.47720386886985189 ) ) ;
#18823=CARTESIAN_POINT ( 'NONE',  ( -8.685887942688735208, 461.9323905601785327, 3.978247347593161010 ) ) ;
#18824=CARTESIAN_POINT ( 'NONE',  ( -40.53162694259543031, 292.6198905683720000, -11.84573899990672707 ) ) ;
#18830=CARTESIAN_POINT ( 'NONE',  ( -13.20868407381885135, 308.2448905683720000, 6.410867750099229490 ) ) ;
#18831=CARTESIAN_POINT ( 'NONE',  ( -44.16309181155857289, 374.7448905683720568, -6.410867750099231266 ) ) ;
#18833=CARTESIAN_POINT ( 'NONE',  ( -36.33955658999053639, 523.8698905765655809, 18.47759065022572500 ) ) ;
#18834=CARTESIAN_POINT ( 'NONE',  ( -40.53162694259544452, 395.1198905683720000, 11.84573899990672885 ) ) ;
#18835=CARTESIAN_POINT ( 'NONE',  ( -45.43829269268869808, 235.3698905683720284, 0.000000000000000000 ) ) ;
#18836=CARTESIAN_POINT ( 'NONE',  ( -45.43829269268871940, 424.1823905683721136, 3.332260488124734632 ) ) ;
#18837=CARTESIAN_POINT ( 'NONE',  ( -11.73070664223724613, 346.0573905765656377, 11.32908994701042005 ) ) ;
#18839=CARTESIAN_POINT ( 'NONE',  ( -42.88789093042842637, 314.8073905683721136, 9.489475012073734561 ) ) ;
#18840=CARTESIAN_POINT ( 'NONE',  ( -11.93348319268873503, 480.6823905683720000, -3.332260488124732856 ) ) ;
#18841=CARTESIAN_POINT ( 'NONE',  ( -10.20829729246300488, 516.3698905765656946, 7.653668647301790529 ) ) ;
#18844=CARTESIAN_POINT ( 'NONE',  ( -45.43829269268871229, 395.0573905683719431, -3.332260488124726194 ) ) ;
#18846=EDGE_CURVE ( 'NONE', #19418, #14194, #17837, .T. ) ;
#18848=CARTESIAN_POINT ( 'NONE',  ( -42.82802356641968089, 525.9948905601785327, -14.14213562373094746 ) ) ;
#18849=CARTESIAN_POINT ( 'NONE',  ( -42.88789093042843348, 344.8073905683719431, 9.489475012073736337 ) ) ;
#18851=CARTESIAN_POINT ( 'NONE',  ( -45.43829269268873361, 513.8698905683720568, 0.000000000000000000 ) ) ;
#18853=CARTESIAN_POINT ( 'NONE',  ( -44.33485469295106185, 223.9102039777117454, -6.015342892178036749 ) ) ;
#18855=CARTESIAN_POINT ( 'NONE',  ( -40.01497788969913216, 290.4323905765656946, -16.95518130045146421 ) ) ;
#18857=CARTESIAN_POINT ( 'NONE',  ( -45.43829269268871940, 463.5573905683720568, -3.332260488124726194 ) ) ;
#18858=ORIENTED_EDGE ( 'NONE', *, *, #11610, .F. ) ;
#18859=CARTESIAN_POINT ( 'NONE',  ( -14.48388495494901029, 477.9323905683721136, 9.489475012073731008 ) ) ;
#18862=CARTESIAN_POINT ( 'NONE',  ( -21.03221929538692692, 398.8698905765656377, -18.47759065022572855 ) ) ;
#18863=CARTESIAN_POINT ( 'NONE',  ( -21.03221929538692336, 475.1198905765656377, 18.47759065022572500 ) ) ;
#18864=CARTESIAN_POINT ( 'NONE',  ( -8.685887942688735208, 482.2448905601784759, -2.449293598294705724E-15 ) ) ;
#18866=EDGE_CURVE ( 'NONE', #2991, #16878, #7100, .T. ) ;
#18870=CARTESIAN_POINT ( 'NONE',  ( -8.685887942688708563, 242.2448905601785043, -2.449293598294705724E-15 ) ) ;
#18871=CARTESIAN_POINT ( 'NONE',  ( -28.68588794268869790, 213.9102039777116602, 0.000000000000000000 ) ) ;
#18872=CARTESIAN_POINT ( 'NONE',  ( -32.01814843081344009, 277.5573905683720000, 16.75240474999999307 ) ) ;
#18873=CARTESIAN_POINT ( 'NONE',  ( -45.64106924314017277, 248.1823905601785043, 11.32908994701042715 ) ) ;
#18875=CARTESIAN_POINT ( 'NONE',  ( -8.685887942688902186, 366.6823905765656377, 3.978247347593586447 ) ) ;
#18876=CARTESIAN_POINT ( 'NONE',  ( -11.93348319268872970, 440.0573905683720000, 3.332260488124728415 ) ) ;
#18877=CARTESIAN_POINT ( 'NONE',  ( -14.54375231895776643, 328.2448905765656377, -14.14213562373094746 ) ) ;
#18878=CARTESIAN_POINT ( 'NONE',  ( -11.93348319268870839, 260.3698905683720000, -2.051577885510841163E-15 ) ) ;
#18882=DIRECTION ( 'NONE',  ( -1.191790137725560488E-16, 1.000000000000000000, -0.000000000000000000 ) ) ;
#18884=CARTESIAN_POINT ( 'NONE',  ( -28.68588794268872988, 482.8698905683720568, -16.75240474999999307 ) ) ;
#18886=EDGE_LOOP ( 'NONE', ( #13985, #2827, #14367, #11876 ) ) ;
#18888=CARTESIAN_POINT ( 'NONE',  ( -19.19641293061497223, 250.4323905683720284, -14.20200298773971603 ) ) ;
#18892=CARTESIAN_POINT ( 'NONE',  ( -36.33955658999052218, 460.1198905765655809, -18.47759065022572855 ) ) ;
#18894=CARTESIAN_POINT ( 'NONE',  ( -45.64106924314019409, 456.3073905601785327, -11.32908994701042538 ) ) ;
#18896=CARTESIAN_POINT ( 'NONE',  ( -25.35362745456399836, 518.1823905683720568, 16.75240474999998952 ) ) ;
#18898=CARTESIAN_POINT ( 'NONE',  ( -45.43829269268869098, 254.1823905683719715, 3.332260488124734632 ) ) ;
#18899=CARTESIAN_POINT ( 'NONE',  ( -28.68588794268871212, 332.8698905683720000, -16.75240474999999307 ) ) ;
#18901=CARTESIAN_POINT ( 'NONE',  ( -8.685887942688868435, 471.9323905601783622, 3.978247347593479866 ) ) ;
#18902=CARTESIAN_POINT ( 'NONE',  ( -14.54375231895776643, 360.9948905601784759, 14.14213562373094568 ) ) ;
#18903=AXIS2_PLACEMENT_3D ( 'NONE', #8443, #20137, #358 ) ;
#18904=CARTESIAN_POINT ( 'NONE',  ( -42.88789093042844058, 392.9323905683720568, -9.489475012073736337 ) ) ;
#18905=CARTESIAN_POINT ( 'NONE',  ( -45.43829269268873361, 535.0573905683719431, -3.332260488124726638 ) ) ;
#18906=CARTESIAN_POINT ( 'NONE',  ( -21.03221929538691271, 390.3698905601785327, 18.47759065022572500 ) ) ;
#18907=CARTESIAN_POINT ( 'NONE',  ( -31.26501780185373391, 205.1437886375728965, 0.000000000000000000 ) ) ;
#18910=CARTESIAN_POINT ( 'NONE',  ( -13.20868407381887799, 510.9948905683721136, -6.410867750099233042 ) ) ;
#18911=CARTESIAN_POINT ( 'NONE',  ( -14.54375231895775933, 295.7448905765656377, 14.14213562373094568 ) ) ;
#18913=CARTESIAN_POINT ( 'NONE',  ( -19.19641293061497223, 308.8073905683721136, 14.20200298773971426 ) ) ;
#18915=CARTESIAN_POINT ( 'NONE',  ( -19.19641293061497933, 337.3073905683720568, 14.20200298773971426 ) ) ;
#18916=CARTESIAN_POINT ( 'NONE',  ( -42.88789093042843348, 342.9323905683721136, -9.489475012073734561 ) ) ;
#18918=CARTESIAN_POINT ( 'NONE',  ( -48.68588794268870146, 282.3073905765656377, 3.978247347593168115 ) ) ;
#18919=LINE ( 'NONE', #7667, #13806 ) ;
#18920=CARTESIAN_POINT ( 'NONE',  ( -42.88789093042841927, 254.8073905683720284, 9.489475012073734561 ) ) ;
#18921=CARTESIAN_POINT ( 'NONE',  ( -42.88696169552117965, 203.8418613323789543, 4.830328443944832628 ) ) ;
#18922=CARTESIAN_POINT ( 'NONE',  ( -22.27502019258947996, 398.4948905683720000, 15.47720386886985189 ) ) ;
#18924=CARTESIAN_POINT ( 'NONE',  ( -8.685887942689081598, 506.6823905765655240, 3.978247347593985683 ) ) ;
#18927=CARTESIAN_POINT ( 'NONE',  ( -8.685887942688713892, 286.9948905765656377, -2.449293598294705724E-15 ) ) ;
#18928=CARTESIAN_POINT ( 'NONE',  ( -42.88789093042844769, 462.9323905683720568, -9.489475012073736337 ) ) ;
#18929=ORIENTED_EDGE ( 'NONE', *, *, #21136, .T. ) ;
#18930=CARTESIAN_POINT ( 'NONE',  ( -32.66413529028189089, 455.0573905601785327, -19.99999999999999289 ) ) ;
#18933=CARTESIAN_POINT ( 'NONE',  ( -48.68588794268870856, 337.2448905601784759, 0.000000000000000000 ) ) ;
#18937=CARTESIAN_POINT ( 'NONE',  ( -40.01497788969913216, 348.8073905601784190, 16.95518130045146776 ) ) ;
#18938=CARTESIAN_POINT ( 'NONE',  ( -11.93348319268871727, 309.1823905683719431, -3.332260488124732856 ) ) ;
#18939=CARTESIAN_POINT ( 'NONE',  ( -13.20868407381885845, 359.7448905683720568, 6.410867750099229490 ) ) ;
#18940=CARTESIAN_POINT ( 'NONE',  ( -48.68588794268860909, 296.9323905601784759, -3.978247347593371508 ) ) ;
#18941=CARTESIAN_POINT ( 'NONE',  ( -8.685887942688742314, 526.9948905765655809, -2.449293598294705724E-15 ) ) ;
#18942=CARTESIAN_POINT ( 'NONE',  ( -38.17536295476246266, 412.3073905683720000, -14.20200298773971426 ) ) ;
#18943=CARTESIAN_POINT ( 'NONE',  ( -25.35362745456397704, 232.5573905683720568, -16.75240474999999307 ) ) ;
#18944=CARTESIAN_POINT ( 'NONE',  ( -13.20868407381886378, 408.2448905683720568, 6.410867750099229490 ) ) ;
#18948=CARTESIAN_POINT ( 'NONE',  ( -10.20829729246298356, 346.3698905765655809, 7.653668647301790529 ) ) ;
#18950=CARTESIAN_POINT ( 'NONE',  ( -48.68588794268870146, 327.2448905601785327, 0.000000000000000000 ) ) ;
#18951=CARTESIAN_POINT ( 'NONE',  ( -25.35362745456397349, 296.6823905683720568, 16.75240474999998952 ) ) ;
#18952=CARTESIAN_POINT ( 'NONE',  ( -14.48388495494900852, 459.4323905683720568, 9.489475012073732785 ) ) ;
#18955=CARTESIAN_POINT ( 'NONE',  ( -11.93348319268872260, 370.3698905683720568, -2.051577885510841163E-15 ) ) ;
#18957=CARTESIAN_POINT ( 'NONE',  ( -42.82802356641968089, 515.9948905601785327, -14.14213562373094746 ) ) ;
#18958=CARTESIAN_POINT ( 'NONE',  ( -25.35362745456397704, 336.6823905683720568, 16.75240474999998952 ) ) ;
#18962=CARTESIAN_POINT ( 'NONE',  ( -25.35362745456399836, 496.6823905683721136, 16.75240474999998952 ) ) ;
#18964=CARTESIAN_POINT ( 'NONE',  ( -10.20829729246298356, 351.6198905601784759, 7.653668647301790529 ) ) ;
#18966=CARTESIAN_POINT ( 'NONE',  ( -24.70764059509554755, 314.8073905765655809, 19.99999999999998934 ) ) ;
#18967=CARTESIAN_POINT ( 'NONE',  ( -22.27502019258949417, 422.2448905683720568, -15.47720386886985544 ) ) ;
#18969=VECTOR ( 'NONE', #12497, 1000.000000000000000 ) ;
#18971=CARTESIAN_POINT ( 'NONE',  ( -22.27502019258949062, 466.9948905683720000, 15.47720386886985189 ) ) ;
#18972=VERTEX_POINT ( 'NONE', #19119 ) ;
#18973=CARTESIAN_POINT ( 'NONE',  ( -14.48388495494901029, 469.8073905683719431, -9.489475012073734561 ) ) ;
#18975=CARTESIAN_POINT ( 'NONE',  ( -11.73070664223725501, 397.9323905765656377, -11.32908994701042715 ) ) ;
#18976=CARTESIAN_POINT ( 'NONE',  ( -40.01497788969913216, 280.4323905765655809, -16.95518130045146421 ) ) ;
#18977=CARTESIAN_POINT ( 'NONE',  ( -40.01497788969912506, 298.8073905601785327, 16.95518130045146776 ) ) ;
#18982=CARTESIAN_POINT ( 'NONE',  ( -45.64106924314016567, 238.1823905601784759, 11.32908994701042538 ) ) ;
#18983=DIRECTION ( 'NONE',  ( -1.000000000000000000, 0.000000000000000000, 0.000000000000000000 ) ) ;
#18984=( BOUNDED_CURVE ( )  B_SPLINE_CURVE ( 2, ( #19434, #19328, #7747, #17705, #2902, #16416, #12844, #9482, #17810, #15996, #13167, #12951, #6339, #8062, #4514, #1272, #7851 ),
 .UNSPECIFIED., .F., .T. ) 
 B_SPLINE_CURVE_WITH_KNOTS ( ( 3, 2, 2, 2, 2, 2, 2, 2, 3 ),
 ( 0.9062500000000001110, 0.9082031250000001110, 0.9101562500000001110, 0.9121093750000001110, 0.9140625000000001110, 0.9160156250000001110, 0.9179687500000001110, 0.9199218750000001110, 0.9218750000000001110 ),
 .UNSPECIFIED. ) 
 CURVE ( )  GEOMETRIC_REPRESENTATION_ITEM ( )  RATIONAL_B_SPLINE_CURVE ( ( 0.9999999999999988898, 0.9807852804032315408, 1.000000000000000000, 0.9807852804032304306, 1.000000000000000000, 0.9807852804032304306, 1.000000000000000000, 0.9807852804032304306, 1.000000000000000000, 0.9807852804032304306, 1.000000000000000000, 0.9807852804032304306, 1.000000000000000000, 0.9807852804032304306, 1.000000000000000000, 0.9807852804032293204, 1.000000000000001110 ) ) 
 REPRESENTATION_ITEM ( '' )  );
#18985=CARTESIAN_POINT ( 'NONE',  ( -16.84014894278197616, 279.1198905683720568, 11.84573899990672530 ) ) ;
#18986=CARTESIAN_POINT ( 'NONE',  ( -47.16347859291443001, 246.6198905601784759, -7.653668647301793193 ) ) ;
#18987=CARTESIAN_POINT ( 'NONE',  ( -32.66413529028187668, 404.1823905765656946, 19.99999999999999289 ) ) ;
#18988=CARTESIAN_POINT ( 'NONE',  ( -40.53162694259544452, 424.1198905683720000, -11.84573899990672707 ) ) ;
#18989=CARTESIAN_POINT ( 'NONE',  ( -48.68588794268873698, 573.2448905601785327, 0.000000000000000000 ) ) ;
#18990=CARTESIAN_POINT ( 'NONE',  ( -32.01814843081343298, 263.1823905683720000, -16.75240474999999307 ) ) ;
#18992=CARTESIAN_POINT ( 'NONE',  ( -45.64106924314019409, 481.0573905765655240, -11.32908994701042538 ) ) ;
#18994=CARTESIAN_POINT ( 'NONE',  ( -45.43829269268872650, 475.6823905683719431, 3.332260488124734632 ) ) ;
#18998=CARTESIAN_POINT ( 'NONE',  ( -44.16309181155855157, 234.4948905683720284, 6.410867750099241924 ) ) ;
#19000=CARTESIAN_POINT ( 'NONE',  ( -28.68588794268873698, 531.3698905683720568, -16.75240474999999307 ) ) ;
#19002=CARTESIAN_POINT ( 'NONE',  ( -32.66413529028189089, 469.8073905765656377, -19.99999999999999289 ) ) ;
#19004=CARTESIAN_POINT ( 'NONE',  ( -10.20829729246297646, 286.3698905765655809, 7.653668647301790529 ) ) ;
#19006=CARTESIAN_POINT ( 'NONE',  ( -24.70764059509556887, 454.4323905601784759, -19.99999999999999289 ) ) ;
#19009=EDGE_CURVE ( 'NONE', #18802, #3367, #15278, .T. ) ;
#19010=CARTESIAN_POINT ( 'NONE',  ( -22.27502019258950128, 512.2448905683720568, -15.47720386886985544 ) ) ;
#19012=CARTESIAN_POINT ( 'NONE',  ( -11.93348319268870661, 238.8698905683720568, -2.051577885510841163E-15 ) ) ;
#19013=CARTESIAN_POINT ( 'NONE',  ( -16.84014894278198682, 341.6198905683720000, -11.84573899990672707 ) ) ;
#19014=CARTESIAN_POINT ( 'NONE',  ( -8.685887942688735208, 472.2448905601784759, -2.449293598294705724E-15 ) ) ;
#19016=CARTESIAN_POINT ( 'NONE',  ( -36.33955658999051508, 359.1198905601785327, 18.47759065022572500 ) ) ;
#19018=CARTESIAN_POINT ( 'NONE',  ( -45.43829269268870519, 384.1823905683720000, 3.332260488124734632 ) ) ;
#19021=VECTOR ( 'NONE', #16540, 1000.000000000000000 ) ;
#19022=CARTESIAN_POINT ( 'NONE',  ( -42.82802356641965957, 378.4948905601784759, 14.14213562373094923 ) ) ;
#19024=CARTESIAN_POINT ( 'NONE',  ( -24.70764059509555821, 349.1823905765655809, -19.99999999999999289 ) ) ;
#19026=CARTESIAN_POINT ( 'NONE',  ( -28.68588794268873343, 502.8698905683719431, -16.75240474999999307 ) ) ;
#19030=CARTESIAN_POINT ( 'NONE',  ( -40.53162694259543031, 296.6198905683720000, 11.84573899990672885 ) ) ;
#19032=VERTEX_POINT ( 'NONE', #4513 ) ;
#19033=CARTESIAN_POINT ( 'NONE',  ( -13.20868407381885667, 348.2448905683720000, 6.410867750099229490 ) ) ;
#19034=CARTESIAN_POINT ( 'NONE',  ( -25.35362745456398770, 341.0573905683720568, -16.75240474999999307 ) ) ;
#19036=CARTESIAN_POINT ( 'NONE',  ( -11.73070664223724080, 277.9323905765655809, -11.32908994701042715 ) ) ;
#19038=DIRECTION ( 'NONE',  ( -1.000000000000000000, 0.000000000000000000, 0.000000000000000000 ) ) ;
#19039=CARTESIAN_POINT ( 'NONE',  ( -16.84014894278197616, 240.1198905683720284, -11.84573899990672707 ) ) ;
#19041=CARTESIAN_POINT ( 'NONE',  ( -28.68588794268871567, 387.8698905683720000, 16.75240474999999307 ) ) ;
#19046=CARTESIAN_POINT ( 'NONE',  ( -40.53162694259544452, 445.1198905683720568, 11.84573899990672885 ) ) ;
#19048=CARTESIAN_POINT ( 'NONE',  ( -40.01497788969915348, 455.6823905601785327, -16.95518130045146421 ) ) ;
#19049=VERTEX_POINT ( 'NONE', #12843 ) ;
#19052=FACE_OUTER_BOUND ( 'NONE', #4576, .T. ) ;
#19054=CARTESIAN_POINT ( 'NONE',  ( -21.03221929538691981, 334.1198905601784759, -18.47759065022572855 ) ) ;
#19056=CARTESIAN_POINT ( 'NONE',  ( -16.84014894278197971, 297.6198905683720000, 11.84573899990672530 ) ) ;
#19057=CARTESIAN_POINT ( 'NONE',  ( -19.19641293061497933, 358.8073905683720000, 14.20200298773971426 ) ) ;
#19058=CARTESIAN_POINT ( 'NONE',  ( -24.70764059509555111, 294.4323905601784190, -19.99999999999999289 ) ) ;
#19060=CARTESIAN_POINT ( 'NONE',  ( -48.68588794268872988, 522.3073905765655809, 3.978247347593168115 ) ) ;
#19061=CARTESIAN_POINT ( 'NONE',  ( -22.27502019258949417, 410.7448905683720568, -15.47720386886985544 ) ) ;
#19062=CARTESIAN_POINT ( 'NONE',  ( -19.19641293061496867, 248.8073905683720284, 14.20200298773971426 ) ) ;
#19063=CARTESIAN_POINT ( 'NONE',  ( -14.48388495494900674, 407.9323905683719431, 9.489475012073731008 ) ) ;
#19064=CARTESIAN_POINT ( 'NONE',  ( -21.03221929538692336, 348.8698905765656377, -18.47759065022572855 ) ) ;
#19065=CARTESIAN_POINT ( 'NONE',  ( -8.685887942688710339, 262.2448905601784759, -2.449293598294705724E-15 ) ) ;
#19066=CARTESIAN_POINT ( 'NONE',  ( -40.53162694259543031, 312.6198905683720000, -11.84573899990672707 ) ) ;
#19067=( NAMED_UNIT ( * ) PLANE_ANGLE_UNIT ( ) SI_UNIT ( $, .RADIAN. ) );
#19068=CARTESIAN_POINT ( 'NONE',  ( -45.43829269268871940, 465.6823905683720000, 3.332260488124734632 ) ) ;
#19069=CARTESIAN_POINT ( 'NONE',  ( -47.16347859291446554, 512.6198905765656946, 7.653668647301805628 ) ) ;
#19070=CARTESIAN_POINT ( 'NONE',  ( -8.685887942688902186, 371.9323905601784759, 3.978247347593586447 ) ) ;
#19071=CARTESIAN_POINT ( 'NONE',  ( -8.685887942688742314, 573.2448905601785327, 2.449293598294706119E-15 ) ) ;
#19072=CARTESIAN_POINT ( 'NONE',  ( -28.68588794268871567, 372.8698905683720000, -16.75240474999999307 ) ) ;
#19073=CARTESIAN_POINT ( 'NONE',  ( -25.35362745456399836, 496.6823905683721136, 16.75240474999998952 ) ) ;
#19074=CARTESIAN_POINT ( 'NONE',  ( -21.03221929538694113, 514.1198905601785327, -18.47759065022572855 ) ) ;
#19075=CARTESIAN_POINT ( 'NONE',  ( -28.68588794268871567, 351.3698905683720568, -16.75240474999999307 ) ) ;
#19076=ADVANCED_FACE ( 'NONE', ( #4302 ), #7530, .T. ) ;
#19078=CARTESIAN_POINT ( 'NONE',  ( -35.09675569278797269, 505.7448905683720000, 15.47720386886985366 ) ) ;
#19079=ORIENTED_EDGE ( 'NONE', *, *, #17553, .F. ) ;
#19080=CARTESIAN_POINT ( 'NONE',  ( -21.03221929538690560, 315.1198905765656377, 18.47759065022572500 ) ) ;
#19081=CARTESIAN_POINT ( 'NONE',  ( -28.68588794268872277, 422.8698905683720568, -16.75240474999999307 ) ) ;
#19084=CARTESIAN_POINT ( 'NONE',  ( -40.53162694259545162, 462.6198905683720000, -11.84573899990672707 ) ) ;
#19086=ORIENTED_EDGE ( 'NONE', *, *, #4146, .T. ) ;
#19087=CARTESIAN_POINT ( 'NONE',  ( -38.17536295476246977, 472.3073905683720568, -14.20200298773971426 ) ) ;
#19088=CARTESIAN_POINT ( 'NONE',  ( -24.70764059509553334, 250.0573905601785043, 19.99999999999998934 ) ) ;
#19089=CARTESIAN_POINT ( 'NONE',  ( -36.33955658999052218, 393.8698905765656377, 18.47759065022572500 ) ) ;
#19090=CARTESIAN_POINT ( 'NONE',  ( -8.685887942688712116, 282.2448905601784759, -2.449293598294705724E-15 ) ) ;
#19096=CARTESIAN_POINT ( 'NONE',  ( -10.20829729246297291, 241.6198905601784759, 7.653668647301790529 ) ) ;
#19099=CARTESIAN_POINT ( 'NONE',  ( -32.01814843081343298, 273.1823905683720568, -16.75240474999999307 ) ) ;
#19100=CARTESIAN_POINT ( 'NONE',  ( -32.66413529028186247, 249.4323905601784475, 19.99999999999999289 ) ) ;
#19102=CARTESIAN_POINT ( 'NONE',  ( -16.84014894278199748, 421.6198905683720000, -11.84573899990672707 ) ) ;
#19104=CARTESIAN_POINT ( 'NONE',  ( -16.84014894278197616, 251.6198905683720284, -11.84573899990672707 ) ) ;
#19105=ADVANCED_FACE ( 'NONE', ( #15884 ), #9266, .T. ) ;
#19108=CARTESIAN_POINT ( 'NONE',  ( -36.33955658999052218, 480.1198905765656377, -18.47759065022572855 ) ) ;
#19109=ORIENTED_EDGE ( 'NONE', *, *, #10920, .T. ) ;
#19110=CARTESIAN_POINT ( 'NONE',  ( -40.53162694259545162, 484.1198905683720000, -11.84573899990672707 ) ) ;
#19112=CYLINDRICAL_SURFACE ( 'NONE', #20397, 19.99999999999999645 ) ;
#19113=CARTESIAN_POINT ( 'NONE',  ( -25.35362745456396638, 246.6823905683720284, 16.75240474999998952 ) ) ;
#19114=ORIENTED_EDGE ( 'NONE', *, *, #20396, .F. ) ;
#19115=CARTESIAN_POINT ( 'NONE',  ( -11.93348319268874036, 519.1823905683720568, -3.332260488124732856 ) ) ;
#19117=CARTESIAN_POINT ( 'NONE',  ( -21.03221929538693402, 458.8698905765656377, -18.47759065022572855 ) ) ;
#19119=CARTESIAN_POINT ( 'NONE',  ( -8.685887942688713892, 292.2448905601784759, -2.449293598294705724E-15 ) ) ;
#19120=CARTESIAN_POINT ( 'NONE',  ( -27.59433460082644274, 223.9102039777117170, -18.70402771398575226 ) ) ;
#19121=CARTESIAN_POINT ( 'NONE',  ( -22.27502019258945865, 228.4948905683720284, 15.47720386886985189 ) ) ;
#19122=( BOUNDED_CURVE ( )  B_SPLINE_CURVE ( 2, ( #16009, #1191, #12961, #7761, #14388, #20972, #6140, #12751, #11115, #19551, #17923, #9169, #5557, #3230, #12052, #10023, #1500 ),
 .UNSPECIFIED., .F., .T. ) 
 B_SPLINE_CURVE_WITH_KNOTS ( ( 3, 2, 2, 2, 2, 2, 2, 2, 3 ),
 ( 0.9375000000000001110, 0.9394531250000001110, 0.9414062500000001110, 0.9433593750000001110, 0.9453125000000001110, 0.9472656250000001110, 0.9492187500000001110, 0.9511718750000001110, 0.9531250000000001110 ),
 .UNSPECIFIED. ) 
 CURVE ( )  GEOMETRIC_REPRESENTATION_ITEM ( )  RATIONAL_B_SPLINE_CURVE ( ( 0.9999999999999988898, 0.9807852804032315408, 1.000000000000000000, 0.9807852804032304306, 1.000000000000000000, 0.9807852804032304306, 1.000000000000000000, 0.9807852804032304306, 1.000000000000000000, 0.9807852804032304306, 1.000000000000000000, 0.9807852804032304306, 1.000000000000000000, 0.9807852804032304306, 1.000000000000000000, 0.9807852804032293204, 1.000000000000001110 ) ) 
 REPRESENTATION_ITEM ( '' )  );
#19123=CARTESIAN_POINT ( 'NONE',  ( -22.27502019258949417, 518.4948905683719431, 15.47720386886985189 ) ) ;
#19124=CARTESIAN_POINT ( 'NONE',  ( -48.68588794268873698, 573.2448905601785327, 0.000000000000000000 ) ) ;
#19125=CARTESIAN_POINT ( 'NONE',  ( -45.43829269268869808, 223.8698905683720284, 0.000000000000000000 ) ) ;
#19126=CARTESIAN_POINT ( 'NONE',  ( -32.01814843081344719, 333.1823905683720000, -16.75240474999999307 ) ) ;
#19128=CARTESIAN_POINT ( 'NONE',  ( -24.70764059509556176, 470.0573905601784759, 19.99999999999998934 ) ) ;
#19129=CARTESIAN_POINT ( 'NONE',  ( -48.68588794268870146, 271.9948905765656377, 0.000000000000000000 ) ) ;
#19131=CARTESIAN_POINT ( 'NONE',  ( -11.93348319268872260, 379.1823905683721136, -3.332260488124732856 ) ) ;
#19132=CARTESIAN_POINT ( 'NONE',  ( -48.68588794268870146, 321.9948905765655809, 0.000000000000000000 ) ) ;
#19134=CARTESIAN_POINT ( 'NONE',  ( -48.68588794268870856, 377.5573905601785327, 3.978247347593168115 ) ) ;
#19138=VERTEX_POINT ( 'NONE', #5805 ) ;
#19139=ORIENTED_EDGE ( 'NONE', *, *, #4537, .T. ) ;
#19140=CARTESIAN_POINT ( 'NONE',  ( -32.01814843081346140, 503.1823905683721136, -16.75240474999999307 ) ) ;
#19142=CARTESIAN_POINT ( 'NONE',  ( -8.685887942688715668, 296.9948905765655809, -2.449293598294705724E-15 ) ) ;
#19144=CARTESIAN_POINT ( 'NONE',  ( -35.09675569278794427, 297.2448905683720000, 15.47720386886985366 ) ) ;
#19146=CARTESIAN_POINT ( 'NONE',  ( -19.19641293061497933, 327.3073905683720568, 14.20200298773971426 ) ) ;
#19147=CARTESIAN_POINT ( 'NONE',  ( -14.48388495494899608, 347.9323905683720568, 9.489475012073731008 ) ) ;
#19150=CARTESIAN_POINT ( 'NONE',  ( -14.54375231895775755, 258.2448905765656377, -14.14213562373094746 ) ) ;
#19151=CARTESIAN_POINT ( 'NONE',  ( -48.68588794268872277, 501.9948905765656377, 0.000000000000000000 ) ) ;
#19152=CARTESIAN_POINT ( 'NONE',  ( -11.93348319268870661, 249.1823905683720568, -3.332260488124732856 ) ) ;
#19153=CARTESIAN_POINT ( 'NONE',  ( -32.66413529028185536, 225.0573905601784759, -19.99999999999999289 ) ) ;
#19154=CARTESIAN_POINT ( 'NONE',  ( -38.17536295476245556, 406.9323905683719431, 14.20200298773971781 ) ) ;
#19155=ADVANCED_FACE ( 'NONE', ( #13384 ), #21378, .T. ) ;
#19158=CARTESIAN_POINT ( 'NONE',  ( -14.54375231895775578, 243.4948905601784759, -14.14213562373094746 ) ) ;
#19159=CARTESIAN_POINT ( 'NONE',  ( -13.20868407381887089, 449.4948905683720568, -6.410867750099233042 ) ) ;
#19161=CARTESIAN_POINT ( 'NONE',  ( -42.82802356641966668, 445.9948905601784759, -14.14213562373094746 ) ) ;
#19162=EDGE_CURVE ( 'NONE', #13267, #19049, #14585, .T. ) ;
#19166=CARTESIAN_POINT ( 'NONE',  ( -8.685887942688717445, 322.2448905601784759, -2.449293598294705724E-15 ) ) ;
#19167=CARTESIAN_POINT ( 'NONE',  ( -25.35362745456398059, 358.1823905683720000, 16.75240474999998952 ) ) ;
#19169=CARTESIAN_POINT ( 'NONE',  ( -48.68588794268872277, 501.6823905765655809, -3.978247347593158345 ) ) ;
#19170=CARTESIAN_POINT ( 'NONE',  ( -13.20868407381886200, 379.4948905683720000, -6.410867750099233042 ) ) ;
#19171=CARTESIAN_POINT ( 'NONE',  ( -38.17536295476243424, 236.9323905683720000, 14.20200298773971781 ) ) ;
#19172=CARTESIAN_POINT ( 'NONE',  ( -32.01814843081344719, 401.6823905683720000, -16.75240474999999307 ) ) ;
#19173=CARTESIAN_POINT ( 'NONE',  ( -8.685887942688719221, 336.6823905765656377, 3.978247347593161010 ) ) ;
#19174=CARTESIAN_POINT ( 'NONE',  ( -8.685887942688539809, 322.5573905601784190, -3.978247347592740013 ) ) ;
#19175=CARTESIAN_POINT ( 'NONE',  ( -38.17536295476244845, 312.3073905683720568, -14.20200298773971426 ) ) ;
#19176=CARTESIAN_POINT ( 'NONE',  ( -19.19641293061499354, 451.9323905683720568, -14.20200298773971603 ) ) ;
#19177=CARTESIAN_POINT ( 'NONE',  ( -45.64106924314019409, 458.1823905601784190, 11.32908994701042538 ) ) ;
#19180=CARTESIAN_POINT ( 'NONE',  ( -11.93348319268872260, 360.6823905683720568, -3.332260488124732856 ) ) ;
#19181=CARTESIAN_POINT ( 'NONE',  ( -32.01814843081346851, 506.0573905683719431, 16.75240474999999307 ) ) ;
#19183=CARTESIAN_POINT ( 'NONE',  ( -36.33955658999052218, 505.3698905601784190, -18.47759065022572855 ) ) ;
#19184=CARTESIAN_POINT ( 'NONE',  ( -40.53162694259543031, 325.1198905683720568, 11.84573899990672885 ) ) ;
#19186=CARTESIAN_POINT ( 'NONE',  ( -40.53162694259545162, 495.1198905683720000, 11.84573899990672885 ) ) ;
#19187=ORIENTED_EDGE ( 'NONE', *, *, #15407, .F. ) ;
#19189=CARTESIAN_POINT ( 'NONE',  ( -44.16309181155857289, 425.9948905683720568, 6.410867750099241924 ) ) ;
#19192=CARTESIAN_POINT ( 'NONE',  ( -19.19641293061499354, 460.4323905683721136, -14.20200298773971603 ) ) ;
#19193=VERTEX_POINT ( 'NONE', #3214 ) ;
#19194=CARTESIAN_POINT ( 'NONE',  ( -40.53162694259545162, 475.1198905683720000, 11.84573899990672885 ) ) ;
#19195=CARTESIAN_POINT ( 'NONE',  ( -10.20829729246297291, 246.3698905765656093, 7.653668647301790529 ) ) ;
#19196=CARTESIAN_POINT ( 'NONE',  ( -48.68588794268871567, 411.9948905765656377, 0.000000000000000000 ) ) ;
#19197=CARTESIAN_POINT ( 'NONE',  ( -21.03221929538691271, 278.8698905765656377, -18.47759065022572855 ) ) ;
#19199=CARTESIAN_POINT ( 'NONE',  ( -10.20829729246299600, 437.6198905765656377, -7.653668647301794969 ) ) ;
#19203=CARTESIAN_POINT ( 'NONE',  ( -45.56270947133124594, 223.9102039777115749, 4.062575975128698502 ) ) ;
#19204=CARTESIAN_POINT ( 'NONE',  ( -8.685887942688708563, 242.2448905601785043, -2.449293598294705724E-15 ) ) ;
#19205=FACE_OUTER_BOUND ( 'NONE', #2457, .T. ) ;
#19206=CARTESIAN_POINT ( 'NONE',  ( -45.43829269268871229, 425.6823905683720568, 3.332260488124734632 ) ) ;
#19207=CARTESIAN_POINT ( 'NONE',  ( -10.20829729246298712, 382.8698905601784759, -7.653668647301794969 ) ) ;
#19208=CARTESIAN_POINT ( 'NONE',  ( -11.93348319268870839, 250.6823905683720852, -3.332260488124732856 ) ) ;
#19211=FACE_OUTER_BOUND ( 'NONE', #17873, .T. ) ;
#19212=ORIENTED_EDGE ( 'NONE', *, *, #16923, .T. ) ;
#19213=CARTESIAN_POINT ( 'NONE',  ( -14.48388495494901029, 471.3073905683720568, -9.489475012073734561 ) ) ;
#19217=CARTESIAN_POINT ( 'NONE',  ( -32.01814843081343298, 236.0573905683720284, 16.75240474999999307 ) ) ;
#19219=CARTESIAN_POINT ( 'NONE',  ( -44.16309181155859420, 533.2448905683719431, -6.410867750099231266 ) ) ;
#19222=CARTESIAN_POINT ( 'NONE',  ( -10.20829729246299955, 467.6198905765656377, -7.653668647301794969 ) ) ;
#19224=CARTESIAN_POINT ( 'NONE',  ( -42.82802356641965247, 283.2448905765656377, 14.14213562373094923 ) ) ;
#19225=CARTESIAN_POINT ( 'NONE',  ( -28.49465132804630940, 223.9102039777116602, -18.60448546972727257 ) ) ;
#19227=EDGE_CURVE ( 'NONE', #18805, #4636, #8273, .T. ) ;
#19229=CARTESIAN_POINT ( 'NONE',  ( -19.19641293061496867, 237.3073905683720284, 14.20200298773971426 ) ) ;
#19230=CARTESIAN_POINT ( 'NONE',  ( -13.20868407381885490, 329.7448905683720568, 6.410867750099229490 ) ) ;
#19232=DIRECTION ( 'NONE',  ( -1.191790137725560488E-16, 1.000000000000000000, -0.000000000000000000 ) ) ;
#19233=CARTESIAN_POINT ( 'NONE',  ( -38.17536295476244845, 303.8073905683720000, -14.20200298773971426 ) ) ;
#19234=CARTESIAN_POINT ( 'NONE',  ( -19.19641293061498999, 390.4323905683720568, -14.20200298773971603 ) ) ;
#19235=CARTESIAN_POINT ( 'NONE',  ( -19.19641293061500065, 528.8073905683720568, 14.20200298773971426 ) ) ;
#19236=CARTESIAN_POINT ( 'NONE',  ( -10.20829729246298712, 382.8698905601784759, -7.653668647301794969 ) ) ;
#19239=VERTEX_POINT ( 'NONE', #6547 ) ;
#19241=CARTESIAN_POINT ( 'NONE',  ( -35.09675569278797269, 507.2448905683719431, 15.47720386886985366 ) ) ;
#19242=CARTESIAN_POINT ( 'NONE',  ( -11.73070664223723902, 296.0573905765655809, 11.32908994701042005 ) ) ;
#19244=( BOUNDED_CURVE ( )  B_SPLINE_CURVE ( 2, ( #1246, #9455, #20713, #21031, #20603, #18976, #19406, #12709, #7608, #14127, #19197, #14238, #9343, #15646, #17365, #5887, #11070 ),
 .UNSPECIFIED., .F., .T. ) 
 B_SPLINE_CURVE_WITH_KNOTS ( ( 3, 2, 2, 2, 2, 2, 2, 2, 3 ),
 ( 0.7812500000000001110, 0.7832031250000001110, 0.7851562500000001110, 0.7871093750000001110, 0.7890625000000002220, 0.7910156250000002220, 0.7929687500000002220, 0.7949218750000002220, 0.7968750000000002220 ),
 .UNSPECIFIED. ) 
 CURVE ( )  GEOMETRIC_REPRESENTATION_ITEM ( )  RATIONAL_B_SPLINE_CURVE ( ( 0.9999999999999988898, 0.9807852804032315408, 1.000000000000000000, 0.9807852804032304306, 1.000000000000000000, 0.9807852804032304306, 1.000000000000000000, 0.9807852804032304306, 1.000000000000000000, 0.9807852804032304306, 1.000000000000000000, 0.9807852804032304306, 1.000000000000000000, 0.9807852804032304306, 1.000000000000000000, 0.9807852804032282101, 1.000000000000002220 ) ) 
 REPRESENTATION_ITEM ( '' )  );
#19245=CARTESIAN_POINT ( 'NONE',  ( -42.88789093042842637, 296.3073905683720000, 9.489475012073734561 ) ) ;
#19246=CARTESIAN_POINT ( 'NONE',  ( -44.16309181155856578, 323.2448905683720000, -6.410867750099231266 ) ) ;
#19248=CARTESIAN_POINT ( 'NONE',  ( -40.01497788969913216, 270.4323905765655809, -16.95518130045146421 ) ) ;
#19249=CARTESIAN_POINT ( 'NONE',  ( -47.16347859291445133, 396.6198905601784759, -7.653668647301793193 ) ) ;
#19250=CARTESIAN_POINT ( 'NONE',  ( -28.68588794268870146, 241.3698905683720568, -16.75240474999999307 ) ) ;
#19251=CARTESIAN_POINT ( 'NONE',  ( -42.88789093042844058, 396.3073905683719431, 9.489475012073736337 ) ) ;
#19252=CIRCLE ( 'NONE', #17869, 20.00000000000000000 ) ;
#19253=CYLINDRICAL_SURFACE ( 'NONE', #4405, 19.99999999999999645 ) ;
#19256=CARTESIAN_POINT ( 'NONE',  ( -21.03221929538694113, 508.8698905765656377, -18.47759065022572855 ) ) ;
#19257=CARTESIAN_POINT ( 'NONE',  ( -35.09675569278795138, 441.9948905683720568, -15.47720386886985544 ) ) ;
#19258=ORIENTED_EDGE ( 'NONE', *, *, #992, .T. ) ;
#19259=CARTESIAN_POINT ( 'NONE',  ( -48.68588794268871567, 447.2448905601785327, 0.000000000000000000 ) ) ;
#19263=ORIENTED_EDGE ( 'NONE', *, *, #14132, .T. ) ;
#19265=CARTESIAN_POINT ( 'NONE',  ( -10.20829729246298179, 331.6198905601784759, 7.653668647301790529 ) ) ;
#19267=EDGE_CURVE ( 'NONE', #15984, #13902, #20186, .T. ) ;
#19268=CARTESIAN_POINT ( 'NONE',  ( -32.01814843081344719, 367.5573905683721136, 16.75240474999999307 ) ) ;
#19270=CARTESIAN_POINT ( 'NONE',  ( -48.68588794268872277, 501.9948905765656377, 0.000000000000000000 ) ) ;
#19271=CARTESIAN_POINT ( 'NONE',  ( -16.84014894278199392, 390.1198905683720000, -11.84573899990672707 ) ) ;
#19272=CARTESIAN_POINT ( 'NONE',  ( -28.68588794268870146, 242.8698905683720568, -16.75240474999999307 ) ) ;
#19273=CARTESIAN_POINT ( 'NONE',  ( -16.84014894278199037, 397.6198905683720568, 11.84573899990672530 ) ) ;
#19274=CARTESIAN_POINT ( 'NONE',  ( -8.685887942688717445, 326.6823905765656377, 3.978247347593161010 ) ) ;
#19276=CARTESIAN_POINT ( 'NONE',  ( -11.93348319268871549, 308.8698905683720000, -2.051577885510841163E-15 ) ) ;
#19277=CARTESIAN_POINT ( 'NONE',  ( -38.17536295476246266, 466.9323905683720568, 14.20200298773971781 ) ) ;
#19279=CARTESIAN_POINT ( 'NONE',  ( -32.66413529028188378, 459.4323905601785327, 19.99999999999999289 ) ) ;
#19280=CARTESIAN_POINT ( 'NONE',  ( -48.68588794268870856, 367.2448905601784759, 0.000000000000000000 ) ) ;
#19282=CARTESIAN_POINT ( 'NONE',  ( -45.43829269268870519, 365.6823905683720568, 3.332260488124734632 ) ) ;
#19283=CARTESIAN_POINT ( 'NONE',  ( -35.09675569278797269, 505.7448905683720000, 15.47720386886985366 ) ) ;
#19284=CARTESIAN_POINT ( 'NONE',  ( -48.68588794268872277, 497.5573905601785327, 3.978247347593168115 ) ) ;
#19285=CARTESIAN_POINT ( 'NONE',  ( -32.01814843081344009, 326.0573905683720000, 16.75240474999999307 ) ) ;
#19287=CARTESIAN_POINT ( 'NONE',  ( -32.66413529028185536, 259.4323905601784190, 19.99999999999999289 ) ) ;
#19291=CARTESIAN_POINT ( 'NONE',  ( -16.84014894278199392, 419.1198905683720000, 11.84573899990672530 ) ) ;
#19294=CARTESIAN_POINT ( 'NONE',  ( -22.27502019258949773, 450.7448905683720000, -15.47720386886985544 ) ) ;
#19295=B_SPLINE_CURVE_WITH_KNOTS ( 'NONE', 3,
 ( #14267, #8942, #14049, #17183, #4410, #18786, #10991, #10777, #967, #19120, #19225, #640, #14157, #12634, #7531, #15456, #9050, #6024, #17394, #17600, #8836, #5697, #7206, #3970 ),
 .UNSPECIFIED., .F., .F.,
 ( 4, 2, 2, 2, 2, 2, 2, 2, 2, 2, 2, 4 ),
 ( 0.000000000000000000, 0.002718680586849495009, 0.005437361173698990018, 0.006796701467123738606, 0.008156041760548486327, 0.01087472234739798004, 0.01223406264082271995, 0.01359340293424745640, 0.01631208352109693796, 0.01903076410794641779, 0.02039010440137115424, 0.02174944469479589415 ),
 .UNSPECIFIED. ) ;
#19297=CARTESIAN_POINT ( 'NONE',  ( -16.84014894278200103, 460.1198905683720568, -11.84573899990672707 ) ) ;
#19300=CARTESIAN_POINT ( 'NONE',  ( -45.64106924314018698, 381.0573905765656377, -11.32908994701042715 ) ) ;
#19302=CARTESIAN_POINT ( 'NONE',  ( -45.64106924314017988, 371.0573905765656946, -11.32908994701042538 ) ) ;
#19303=LINE ( 'NONE', #20715, #6000 ) ;
#19307=CARTESIAN_POINT ( 'NONE',  ( -42.82802356641965957, 345.9948905601784759, -14.14213562373094746 ) ) ;
#19308=CARTESIAN_POINT ( 'NONE',  ( -11.93348319268872793, 420.0573905683720000, 3.332260488124728415 ) ) ;
#19310=CARTESIAN_POINT ( 'NONE',  ( -32.01814843081343298, 247.5573905683720000, 16.75240474999999307 ) ) ;
#19311=VERTEX_POINT ( 'NONE', #10431 ) ;
#19312=CARTESIAN_POINT ( 'NONE',  ( -36.33955658999052218, 423.8698905765655809, 18.47759065022572500 ) ) ;
#19313=ORIENTED_EDGE ( 'NONE', *, *, #15061, .T. ) ;
#19314=CARTESIAN_POINT ( 'NONE',  ( -38.17536295476246977, 463.8073905683720000, -14.20200298773971426 ) ) ;
#19315=CARTESIAN_POINT ( 'NONE',  ( -10.20829729246297291, 236.3698905765656093, 7.653668647301790529 ) ) ;
#19319=CARTESIAN_POINT ( 'NONE',  ( -11.93348319268870661, 229.1823905683720284, -3.332260488124732856 ) ) ;
#19321=CARTESIAN_POINT ( 'NONE',  ( -19.19641293061500065, 527.3073905683720568, 14.20200298773971426 ) ) ;
#19324=CARTESIAN_POINT ( 'NONE',  ( -14.54375231895778242, 458.2448905765656377, -14.14213562373094746 ) ) ;
#19327=DIRECTION ( 'NONE',  ( -1.191790137725560488E-16, 1.000000000000000000, -0.000000000000000000 ) ) ;
#19328=CARTESIAN_POINT ( 'NONE',  ( -48.68588794268860198, 241.6823905765656093, -3.978247347593371508 ) ) ;
#19330=CARTESIAN_POINT ( 'NONE',  ( -8.685887942688703234, 223.9102039777117454, 1.614530918564491380 ) ) ;
#19331=CARTESIAN_POINT ( 'NONE',  ( -44.16309181155855157, 234.4948905683720284, 6.410867750099241924 ) ) ;
#19332=CARTESIAN_POINT ( 'NONE',  ( -11.93348319268871727, 320.0573905683720000, 3.332260488124728415 ) ) ;
#19333=CARTESIAN_POINT ( 'NONE',  ( -14.54375231895778064, 443.4948905601784759, -14.14213562373094746 ) ) ;
#19335=B_SPLINE_CURVE_WITH_KNOTS ( 'NONE', 1,
 ( #3273, #9848 ),
 .UNSPECIFIED., .F., .F.,
 ( 2, 2 ),
 ( 0.000000000000000000, 1.000000000000000000 ),
 .UNSPECIFIED. ) ;
#19336=CARTESIAN_POINT ( 'NONE',  ( -13.20868407381885312, 300.9948905683720568, -6.410867750099233042 ) ) ;
#19337=CARTESIAN_POINT ( 'NONE',  ( -14.48388495494900141, 387.9323905683720000, 9.489475012073732785 ) ) ;
#19338=CARTESIAN_POINT ( 'NONE',  ( -28.68588794268873698, 532.8698905683719431, -16.75240474999999307 ) ) ;
#19339=CARTESIAN_POINT ( 'NONE',  ( -47.16347859291444422, 376.6198905601784759, -7.653668647301793193 ) ) ;
#19340=ADVANCED_FACE ( 'NONE', ( #15220 ), #20291, .T. ) ;
#19341=CARTESIAN_POINT ( 'NONE',  ( -45.64106924314018698, 406.3073905601785327, -11.32908994701042538 ) ) ;
#19344=CARTESIAN_POINT ( 'NONE',  ( -16.84014894278200103, 489.1198905683720000, 11.84573899990672530 ) ) ;
#19346=EDGE_LOOP ( 'NONE', ( #16875, #18004, #21339, #7308 ) ) ;
#19347=CARTESIAN_POINT ( 'NONE',  ( -35.09675569278793716, 293.4948905683720000, -15.47720386886985544 ) ) ;
#19348=CARTESIAN_POINT ( 'NONE',  ( -45.43829269268869808, 323.5573905683720000, -3.332260488124726194 ) ) ;
#19349=CARTESIAN_POINT ( 'NONE',  ( -48.68588794268869435, 262.3073905765655809, 3.978247347593168115 ) ) ;
#19353=CARTESIAN_POINT ( 'NONE',  ( -19.19641293061498999, 381.9323905683720568, -14.20200298773971603 ) ) ;
#19354=EDGE_CURVE ( 'NONE', #19427, #21369, #12091, .T. ) ;
#19358=CARTESIAN_POINT ( 'NONE',  ( -45.64106924314020119, 511.0573905765657514, -11.32908994701042538 ) ) ;
#19359=CARTESIAN_POINT ( 'NONE',  ( -28.68588794268872277, 446.3698905683720000, 16.75240474999999307 ) ) ;
#19361=VERTEX_POINT ( 'NONE', #13489 ) ;
#19362=( BOUNDED_CURVE ( )  B_SPLINE_CURVE ( 2, ( #5385, #3666, #16873, #15046, #119, #6693, #5283, #5495, #7113, #13738, #441, #3564, #9934, #13524, #2057, #15153, #8630 ),
 .UNSPECIFIED., .F., .T. ) 
 B_SPLINE_CURVE_WITH_KNOTS ( ( 3, 2, 2, 2, 2, 2, 2, 2, 3 ),
 ( 0.07812500000000043021, 0.08007812500000038858, 0.08203125000000034694, 0.08398437500000030531, 0.08593750000000024980, 0.08789062500000020817, 0.08984375000000016653, 0.09179687500000012490, 0.09375000000000008327 ),
 .UNSPECIFIED. ) 
 CURVE ( )  GEOMETRIC_REPRESENTATION_ITEM ( )  RATIONAL_B_SPLINE_CURVE ( ( 0.9999999999999957812, 0.9807852804032346494, 1.000000000000000000, 0.9807852804032304306, 1.000000000000000000, 0.9807852804032304306, 1.000000000000000000, 0.9807852804032304306, 1.000000000000000000, 0.9807852804032304306, 1.000000000000000000, 0.9807852804032304306, 1.000000000000000000, 0.9807852804032304306, 1.000000000000000000, 0.9807852804032296534, 1.000000000000000888 ) ) 
 REPRESENTATION_ITEM ( '' )  );
#19363=CARTESIAN_POINT ( 'NONE',  ( -36.33955658999052218, 455.3698905601784759, -18.47759065022572855 ) ) ;
#19368=ORIENTED_EDGE ( 'NONE', *, *, #19009, .F. ) ;
#19369=CARTESIAN_POINT ( 'NONE',  ( -11.73070664223724613, 356.0573905765655809, 11.32908994701042005 ) ) ;
#19370=CARTESIAN_POINT ( 'NONE',  ( -14.54375231895776643, 333.4948905601784759, -14.14213562373094746 ) ) ;
#19371=CARTESIAN_POINT ( 'NONE',  ( -45.20498122175430922, 223.9102039777117739, -2.861862797699382011 ) ) ;
#19372=CARTESIAN_POINT ( 'NONE',  ( -38.17536295476245556, 363.8073905683720000, -14.20200298773971426 ) ) ;
#19375=CARTESIAN_POINT ( 'NONE',  ( -47.16347859291446554, 511.3698905765655809, -7.653668647301793193 ) ) ;
#19376=CARTESIAN_POINT ( 'NONE',  ( -42.88789093042843348, 384.8073905683720000, 9.489475012073736337 ) ) ;
#19377=CARTESIAN_POINT ( 'NONE',  ( -22.27502019258946930, 222.2448905683720568, -15.47720386886985544 ) ) ;
#19378=CARTESIAN_POINT ( 'NONE',  ( -44.16309181155857289, 383.2448905683720000, -6.410867750099231266 ) ) ;
#19379=CARTESIAN_POINT ( 'NONE',  ( -24.70764059509555821, 319.1823905765655809, -19.99999999999999289 ) ) ;
#19380=CARTESIAN_POINT ( 'NONE',  ( -17.35679799567830273, 423.8073905601785327, -16.95518130045146421 ) ) ;
#19381=CARTESIAN_POINT ( 'NONE',  ( -22.27502019258946930, 286.9948905683720000, 15.47720386886985189 ) ) ;
#19382=CARTESIAN_POINT ( 'NONE',  ( -44.16309181155858710, 454.7448905683720568, -6.410867750099231266 ) ) ;
#19383=CARTESIAN_POINT ( 'NONE',  ( -21.03221929538691981, 460.3698905601784759, 18.47759065022572500 ) ) ;
#19386=CIRCLE ( 'NONE', #758, 15.00000000000000000 ) ;
#19387=CARTESIAN_POINT ( 'NONE',  ( -11.93348319268872260, 370.0573905683719431, 3.332260488124728415 ) ) ;
#19388=CARTESIAN_POINT ( 'NONE',  ( -25.35362745456399836, 506.6823905683720568, 16.75240474999998952 ) ) ;
#19389=CARTESIAN_POINT ( 'NONE',  ( -11.73070664223726389, 501.3073905601785327, 11.32908994701042005 ) ) ;
#19390=CARTESIAN_POINT ( 'NONE',  ( -44.16309181155857289, 333.2448905683720568, -6.410867750099231266 ) ) ;
#19391=ORIENTED_EDGE ( 'NONE', *, *, #5373, .F. ) ;
#19392=CARTESIAN_POINT ( 'NONE',  ( -17.35679799567827786, 260.6823905601785327, 16.95518130045146421 ) ) ;
#19393=ORIENTED_EDGE ( 'NONE', *, *, #7494, .F. ) ;
#19395=CARTESIAN_POINT ( 'NONE',  ( -8.685887942688742314, 573.2448905601785327, 2.449293598294706119E-15 ) ) ;
#19396=EDGE_CURVE ( 'NONE', #1687, #17091, #11537, .T. ) ;
#19397=CARTESIAN_POINT ( 'NONE',  ( -32.01814843081344719, 427.5573905683720568, 16.75240474999999307 ) ) ;
#19398=CARTESIAN_POINT ( 'NONE',  ( -48.68588794268871567, 391.9948905765656377, 0.000000000000000000 ) ) ;
#19399=CARTESIAN_POINT ( 'NONE',  ( -28.68588794268874054, 573.2448905601785327, 0.000000000000000000 ) ) ;
#19400=CARTESIAN_POINT ( 'NONE',  ( -32.01814843081346140, 451.6823905683720568, -16.75240474999999307 ) ) ;
#19401=ORIENTED_EDGE ( 'NONE', *, *, #5957, .F. ) ;
#19402=CARTESIAN_POINT ( 'NONE',  ( -25.35362745456400546, 471.0573905683721136, -16.75240474999999307 ) ) ;
#19405=CARTESIAN_POINT ( 'NONE',  ( -14.54375231895777176, 378.2448905765656377, -14.14213562373094746 ) ) ;
#19406=CARTESIAN_POINT ( 'NONE',  ( -36.33955658999050087, 280.1198905765656377, -18.47759065022572855 ) ) ;
#19408=CARTESIAN_POINT ( 'NONE',  ( -11.73070664223724968, 367.9323905765655809, -11.32908994701042538 ) ) ;
#19410=CARTESIAN_POINT ( 'NONE',  ( -45.64106924314016567, 252.9323905765656377, 11.32908994701042538 ) ) ;
#19413=CARTESIAN_POINT ( 'NONE',  ( -11.73070664223724791, 343.1823905601785327, -11.32908994701042538 ) ) ;
#19414=CARTESIAN_POINT ( 'NONE',  ( -14.48388495494900496, 421.3073905683720000, -9.489475012073736337 ) ) ;
#19416=CARTESIAN_POINT ( 'NONE',  ( -42.88789093042841927, 254.4323905683720284, -9.489475012073736337 ) ) ;
#19418=VERTEX_POINT ( 'NONE', #4055 ) ;
#19421=CARTESIAN_POINT ( 'NONE',  ( -25.35362745456399125, 458.1823905683719431, 16.75240474999998952 ) ) ;
#19423=CARTESIAN_POINT ( 'NONE',  ( -42.82802356641964536, 220.7448905765656093, -14.14213562373094746 ) ) ;
#19425=CARTESIAN_POINT ( 'NONE',  ( -42.88446638378037790, 206.4484180351193174, 4.837872587287140647 ) ) ;
#19426=CARTESIAN_POINT ( 'NONE',  ( -16.84014894278201169, 531.6198905683720568, -11.84573899990672707 ) ) ;
#19427=VERTEX_POINT ( 'NONE', #10643 ) ;
#19430=CARTESIAN_POINT ( 'NONE',  ( -11.73070664223725501, 436.0573905765656377, 11.32908994701042005 ) ) ;
#19432=CARTESIAN_POINT ( 'NONE',  ( -47.16347859291444422, 347.8698905601784759, 7.653668647301805628 ) ) ;
#19434=CARTESIAN_POINT ( 'NONE',  ( -48.68588794268869435, 241.9948905765656377, 0.000000000000000000 ) ) ;
#19435=CARTESIAN_POINT ( 'NONE',  ( -48.68588794268870146, 271.9948905765656377, 0.000000000000000000 ) ) ;
#19439=CARTESIAN_POINT ( 'NONE',  ( -13.20868407381885490, 320.9948905683720568, -6.410867750099233042 ) ) ;
#19440=CARTESIAN_POINT ( 'NONE',  ( -42.82802356641964536, 235.9948905601784759, -14.14213562373094746 ) ) ;
#19442=CARTESIAN_POINT ( 'NONE',  ( -44.16309181155856578, 314.7448905683720000, -6.410867750099231266 ) ) ;
#19443=CARTESIAN_POINT ( 'NONE',  ( -32.01814843081344719, 371.6823905683720000, -16.75240474999999307 ) ) ;
#19444=EDGE_CURVE ( 'NONE', #21047, #14199, #9877, .T. ) ;
#19445=CARTESIAN_POINT ( 'NONE',  ( -38.17536295476247687, 533.8073905683720568, -14.20200298773971426 ) ) ;
#19447=CARTESIAN_POINT ( 'NONE',  ( -11.73070664223725146, 373.1823905601784759, -11.32908994701042715 ) ) ;
#19448=CARTESIAN_POINT ( 'NONE',  ( -28.68588794268871922, 404.7448905601784759, -19.99999999999999289 ) ) ;
#19449=ORIENTED_EDGE ( 'NONE', *, *, #13664, .F. ) ;
#19450=CARTESIAN_POINT ( 'NONE',  ( -22.27502019258949062, 488.4948905683720568, 15.47720386886985189 ) ) ;
#19451=CYLINDRICAL_SURFACE ( 'NONE', #11445, 19.99999999999999645 ) ;
#19452=CARTESIAN_POINT ( 'NONE',  ( -16.84014894278197971, 287.6198905683720000, 11.84573899990672530 ) ) ;
#19454=CARTESIAN_POINT ( 'NONE',  ( -11.93348319268871016, 280.0573905683720568, 3.332260488124728859 ) ) ;
#19455=CARTESIAN_POINT ( 'NONE',  ( -28.68588794268870856, 316.3698905683720568, 16.75240474999999307 ) ) ;
#19456=CARTESIAN_POINT ( 'NONE',  ( -25.35362745456398059, 262.5573905683720000, -16.75240474999999307 ) ) ;
#19458=CARTESIAN_POINT ( 'NONE',  ( -40.01497788969911795, 263.5573905765656377, 16.95518130045146776 ) ) ;
#19460=CARTESIAN_POINT ( 'NONE',  ( -11.93348319268870661, 228.5573905683720568, 3.332260488124728859 ) ) ;
#19462=CARTESIAN_POINT ( 'NONE',  ( -25.35362745456399125, 372.5573905683720568, -16.75240474999999307 ) ) ;
#19467=CARTESIAN_POINT ( 'NONE',  ( -16.84014894278199748, 437.6198905683720000, 11.84573899990672530 ) ) ;
#19470=CARTESIAN_POINT ( 'NONE',  ( -36.33955658999051508, 425.3698905601784759, -18.47759065022572855 ) ) ;
#19476=CARTESIAN_POINT ( 'NONE',  ( -11.73070664223723902, 311.3073905601784759, 11.32908994701042005 ) ) ;
#19480=CARTESIAN_POINT ( 'NONE',  ( -16.84014894278198682, 341.6198905683720000, -11.84573899990672707 ) ) ;
#19481=CARTESIAN_POINT ( 'NONE',  ( -28.68588794268873343, 499.4948905765656377, -19.99999999999999289 ) ) ;
#19482=CARTESIAN_POINT ( 'NONE',  ( -16.84014894278199037, 377.6198905683720568, 11.84573899990672530 ) ) ;
#19484=CARTESIAN_POINT ( 'NONE',  ( -35.09675569278795138, 385.7448905683720000, 15.47720386886985366 ) ) ;
#19485=CARTESIAN_POINT ( 'NONE',  ( -10.20829729246298001, 316.3698905765656377, 7.653668647301790529 ) ) ;
#19486=CARTESIAN_POINT ( 'NONE',  ( -10.20829729246299244, 422.8698905601784759, -7.653668647301794969 ) ) ;
#19487=CARTESIAN_POINT ( 'NONE',  ( -19.19641293061497578, 290.4323905683720568, -14.20200298773971603 ) ) ;
#19489=CARTESIAN_POINT ( 'NONE',  ( -45.43829269268871940, 445.3698905683720000, 0.000000000000000000 ) ) ;
#19491=CARTESIAN_POINT ( 'NONE',  ( -24.70764059509554755, 284.4323905601784759, -19.99999999999999289 ) ) ;
#19492=CARTESIAN_POINT ( 'NONE',  ( -8.685887942688724550, 372.2448905601784759, -2.449293598294705724E-15 ) ) ;
#19495=CARTESIAN_POINT ( 'NONE',  ( -13.20868407381885667, 339.7448905683720568, 6.410867750099229490 ) ) ;
#19496=CARTESIAN_POINT ( 'NONE',  ( -44.16309181155857999, 504.4948905683720568, 6.410867750099241924 ) ) ;
#19497=CARTESIAN_POINT ( 'NONE',  ( -45.64106924314020119, 496.3073905601784759, -11.32908994701042715 ) ) ;
#19498=CARTESIAN_POINT ( 'NONE',  ( -25.35362745456397704, 316.6823905683720000, 16.75240474999998952 ) ) ;
#19500=CARTESIAN_POINT ( 'NONE',  ( -24.70764059509553334, 260.0573905601784759, 19.99999999999998934 ) ) ;
#19503=CARTESIAN_POINT ( 'NONE',  ( -32.01814843081344719, 403.1823905683720000, -16.75240474999999307 ) ) ;
#19504=CARTESIAN_POINT ( 'NONE',  ( -31.26501780185373391, 205.1437886375728965, 0.000000000000000000 ) ) ;
#19506=CARTESIAN_POINT ( 'NONE',  ( -19.19641293061499354, 440.4323905683720000, -14.20200298773971603 ) ) ;
#19507=CARTESIAN_POINT ( 'NONE',  ( -42.88789093042844769, 452.9323905683721136, -9.489475012073734561 ) ) ;
#19509=CARTESIAN_POINT ( 'NONE',  ( -10.20829729246299067, 412.8698905601784759, -7.653668647301794969 ) ) ;
#19510=CARTESIAN_POINT ( 'NONE',  ( -21.03221929538691271, 385.1198905765656377, 18.47759065022572500 ) ) ;
#19515=CARTESIAN_POINT ( 'NONE',  ( -40.53162694259545162, 496.6198905683720000, 11.84573899990672885 ) ) ;
#19517=CARTESIAN_POINT ( 'NONE',  ( -13.68588794268869790, 213.9102039777116602, 1.836970198721029589E-15 ) ) ;
#19518=CARTESIAN_POINT ( 'NONE',  ( -40.01497788969913927, 345.6823905601784759, -16.95518130045146421 ) ) ;
#19519=CARTESIAN_POINT ( 'NONE',  ( -28.68588794268871922, 407.8698905683720568, 16.75240474999999307 ) ) ;
#19521=CARTESIAN_POINT ( 'NONE',  ( -19.19641293061496867, 248.8073905683720284, 14.20200298773971426 ) ) ;
#19523=VERTEX_POINT ( 'NONE', #14129 ) ;
#19526=CARTESIAN_POINT ( 'NONE',  ( -45.43829269268872650, 455.0573905683720000, -3.332260488124726638 ) ) ;
#19527=CARTESIAN_POINT ( 'NONE',  ( -42.82802356641964536, 233.2448905765656093, 14.14213562373094923 ) ) ;
#19530=CARTESIAN_POINT ( 'NONE',  ( -43.37409492154782242, 209.1153864038857648, 3.054836571872670881 ) ) ;
#19531=CARTESIAN_POINT ( 'NONE',  ( -14.48388495494901740, 529.4323905683720568, 9.489475012073732785 ) ) ;
#19534=CARTESIAN_POINT ( 'NONE',  ( -45.43829269268872650, 504.1823905683721136, 3.332260488124734632 ) ) ;
#19537=CARTESIAN_POINT ( 'NONE',  ( -28.68588794268872277, 444.4948905765655809, 19.99999999999999289 ) ) ;
#19538=CARTESIAN_POINT ( 'NONE',  ( -47.16347859291443712, 301.3698905765655809, -7.653668647301793193 ) ) ;
#19539=CARTESIAN_POINT ( 'NONE',  ( -16.84014894278198327, 337.6198905683720000, 11.84573899990672530 ) ) ;
#19542=CARTESIAN_POINT ( 'NONE',  ( -48.68588794268879383, 287.5573905601784759, 3.978247347592954952 ) ) ;
#19543=CARTESIAN_POINT ( 'NONE',  ( -38.17536295476243424, 225.4323905683720000, 14.20200298773971781 ) ) ;
#19544=CARTESIAN_POINT ( 'NONE',  ( -40.53162694259543031, 326.6198905683720568, 11.84573899990672885 ) ) ;
#19545=EDGE_CURVE ( 'NONE', #19877, #19032, #19303, .T. ) ;
#19547=CARTESIAN_POINT ( 'NONE',  ( -25.35362745456397704, 318.1823905683720568, 16.75240474999998952 ) ) ;
#19548=CARTESIAN_POINT ( 'NONE',  ( -38.17536295476246977, 516.9323905683720568, 14.20200298773971781 ) ) ;
#19549=( BOUNDED_CURVE ( )  B_SPLINE_CURVE ( 2, ( #20614, #15549, #5578, #17060, #15438, #5683, #732, #625, #9249, #18987, #4065, #10649, #17375, #4168, #12289, #17268, #2452 ),
 .UNSPECIFIED., .F., .T. ) 
 B_SPLINE_CURVE_WITH_KNOTS ( ( 3, 2, 2, 2, 2, 2, 2, 2, 3 ),
 ( 0.3906250000000001665, 0.3925781250000001665, 0.3945312500000001665, 0.3964843750000001665, 0.3984375000000001665, 0.4003906250000001665, 0.4023437500000001665, 0.4042968750000001665, 0.4062500000000001665 ),
 .UNSPECIFIED. ) 
 CURVE ( )  GEOMETRIC_REPRESENTATION_ITEM ( )  RATIONAL_B_SPLINE_CURVE ( ( 0.9999999999999983347, 0.9807852804032320959, 1.000000000000000000, 0.9807852804032304306, 1.000000000000000000, 0.9807852804032304306, 1.000000000000000000, 0.9807852804032304306, 1.000000000000000000, 0.9807852804032304306, 1.000000000000000000, 0.9807852804032304306, 1.000000000000000000, 0.9807852804032304306, 1.000000000000000000, 0.9807852804032287652, 1.000000000000001554 ) ) 
 REPRESENTATION_ITEM ( '' )  );
#19550=CARTESIAN_POINT ( 'NONE',  ( -8.685887942688722774, 372.5573905601784759, -3.978247347593165895 ) ) ;
#19551=CARTESIAN_POINT ( 'NONE',  ( -24.70764059509554755, 229.1823905765656377, -19.99999999999999289 ) ) ;
#19553=CARTESIAN_POINT ( 'NONE',  ( -11.93348319268873503, 480.6823905683720000, -3.332260488124732856 ) ) ;
#19554=CARTESIAN_POINT ( 'NONE',  ( -28.68588794268874054, 573.2448905601785327, 0.000000000000000000 ) ) ;
#19555=CARTESIAN_POINT ( 'NONE',  ( -11.93348319268871371, 279.1823905683720000, -3.332260488124732856 ) ) ;
#19557=CARTESIAN_POINT ( 'NONE',  ( -14.48388495494898720, 279.4323905683720568, 9.489475012073731008 ) ) ;
#19559=CARTESIAN_POINT ( 'NONE',  ( -44.16309181155855867, 314.4948905683720000, 6.410867750099241924 ) ) ;
#19560=CARTESIAN_POINT ( 'NONE',  ( -8.685887942688712116, 266.6823905765655809, 3.978247347593161010 ) ) ;
#19562=CARTESIAN_POINT ( 'NONE',  ( -45.43829269268869808, 233.5573905683720568, -3.332260488124726638 ) ) ;
#19563=CARTESIAN_POINT ( 'NONE',  ( -28.68588794268871567, 372.8698905683720000, -16.75240474999999307 ) ) ;
#19566=CARTESIAN_POINT ( 'NONE',  ( -10.20829729246297468, 261.6198905601784759, 7.653668647301790529 ) ) ;
#19569=CARTESIAN_POINT ( 'NONE',  ( -45.43829269268871229, 424.1823905683721136, 3.332260488124734632 ) ) ;
#19572=CARTESIAN_POINT ( 'NONE',  ( -24.70764059509555821, 430.0573905601785327, 19.99999999999998934 ) ) ;
#19577=CARTESIAN_POINT ( 'NONE',  ( -40.01497788969913216, 315.6823905601785327, -16.95518130045146421 ) ) ;
#19580=CARTESIAN_POINT ( 'NONE',  ( -14.48388495494899608, 349.4323905683720000, 9.489475012073731008 ) ) ;
#19582=CARTESIAN_POINT ( 'NONE',  ( -8.685887942688740537, 506.6823905765656377, 3.978247347593161010 ) ) ;
#19583=CARTESIAN_POINT ( 'NONE',  ( -11.93348319268872437, 388.5573905683720000, 3.332260488124728415 ) ) ;
#19585=CARTESIAN_POINT ( 'NONE',  ( -22.27502019258947996, 386.9948905683720568, 15.47720386886985189 ) ) ;
#19587=CARTESIAN_POINT ( 'NONE',  ( -42.82802356641965247, 323.2448905765656377, 14.14213562373094923 ) ) ;
#19588=DIRECTION ( 'NONE',  ( -1.000000000000000000, 0.000000000000000000, 0.000000000000000000 ) ) ;
#19590=CARTESIAN_POINT ( 'NONE',  ( -25.35362745456396993, 276.6823905683720000, 16.75240474999998952 ) ) ;
#19591=CARTESIAN_POINT ( 'NONE',  ( -45.43829269268871229, 445.0573905683720000, -3.332260488124726194 ) ) ;
#19598=CARTESIAN_POINT ( 'NONE',  ( -32.01814843081344719, 357.5573905683720000, 16.75240474999999307 ) ) ;
#19599=CARTESIAN_POINT ( 'NONE',  ( -35.09675569278796559, 475.7448905683720568, 15.47720386886985366 ) ) ;
#19600=CARTESIAN_POINT ( 'NONE',  ( -48.68588794268872277, 487.5573905601784759, 3.978247347593168115 ) ) ;
#19601=CARTESIAN_POINT ( 'NONE',  ( -22.27502019258947286, 326.9948905683720000, 15.47720386886985189 ) ) ;
#19602=VERTEX_POINT ( 'NONE', #15752 ) ;
#19603=CARTESIAN_POINT ( 'NONE',  ( -42.82802356641964536, 258.4948905601784759, 14.14213562373094923 ) ) ;
#19605=ORIENTED_EDGE ( 'NONE', *, *, #11610, .T. ) ;
#19608=CARTESIAN_POINT ( 'NONE',  ( -13.20868407381886378, 409.7448905683720000, 6.410867750099229490 ) ) ;
#19610=CARTESIAN_POINT ( 'NONE',  ( -40.53162694259544452, 442.6198905683720568, -11.84573899990672707 ) ) ;
#19611=CARTESIAN_POINT ( 'NONE',  ( -22.27502019258948707, 446.9948905683720000, 15.47720386886985189 ) ) ;
#19614=CARTESIAN_POINT ( 'NONE',  ( -21.03221929538692692, 388.8698905765656377, -18.47759065022572855 ) ) ;
#19616=CARTESIAN_POINT ( 'NONE',  ( -28.68588794268870501, 264.7448905601784759, -19.99999999999999289 ) ) ;
#19618=CARTESIAN_POINT ( 'NONE',  ( -21.03221929538689849, 255.1198905765656377, 18.47759065022572500 ) ) ;
#19619=CARTESIAN_POINT ( 'NONE',  ( -25.35362745456399480, 488.1823905683720568, 16.75240474999998952 ) ) ;
#19623=ADVANCED_FACE ( 'NONE', ( #2444 ), #7721, .T. ) ;
#19624=CARTESIAN_POINT ( 'NONE',  ( -45.43829269268871229, 415.6823905683721136, 3.332260488124734632 ) ) ;
#19626=CARTESIAN_POINT ( 'NONE',  ( -45.43829269268869808, 235.3698905683720284, 0.000000000000000000 ) ) ;
#19628=CARTESIAN_POINT ( 'NONE',  ( -32.66413529028187668, 424.1823905765656377, 19.99999999999999289 ) ) ;
#19630=CARTESIAN_POINT ( 'NONE',  ( -40.53162694259545162, 454.1198905683720568, -11.84573899990672707 ) ) ;
#19631=CARTESIAN_POINT ( 'NONE',  ( -36.33955658999049376, 230.1198905765656093, -18.47759065022572855 ) ) ;
#19632=ORIENTED_EDGE ( 'NONE', *, *, #20470, .T. ) ;
#19633=LINE ( 'NONE', #8052, #7254 ) ;
#19634=CARTESIAN_POINT ( 'NONE',  ( -19.19641293061500065, 528.8073905683719431, 14.20200298773971426 ) ) ;
#19636=CARTESIAN_POINT ( 'NONE',  ( -44.16309181155858710, 514.4948905683720568, 6.410867750099241924 ) ) ;
#19638=CARTESIAN_POINT ( 'NONE',  ( -48.68588794268872277, 452.3073905765656377, 3.978247347593168115 ) ) ;
#19639=CARTESIAN_POINT ( 'NONE',  ( -10.20829729246298534, 357.6198905765656377, -7.653668647301794969 ) ) ;
#19640=CARTESIAN_POINT ( 'NONE',  ( -21.03221929538690915, 248.8698905765656093, -18.47759065022572855 ) ) ;
#19646=CARTESIAN_POINT ( 'NONE',  ( -17.15890915289496732, 223.9102039777116318, -16.43681639555801510 ) ) ;
#19647=CARTESIAN_POINT ( 'NONE',  ( -11.93348319268871549, 310.3698905683720568, -2.051577885510841163E-15 ) ) ;
#19648=DIRECTION ( 'NONE',  ( 1.191790137725560488E-16, -1.000000000000000000, 0.000000000000000000 ) ) ;
#19649=CARTESIAN_POINT ( 'NONE',  ( -28.68588794268869790, 259.7448905601784759, 19.99999999999999289 ) ) ;
#19651=CARTESIAN_POINT ( 'NONE',  ( -38.17536295476244135, 286.9323905683720000, 14.20200298773971781 ) ) ;
#19652=CARTESIAN_POINT ( 'NONE',  ( -45.43829269268873361, 525.6823905683720568, 3.332260488124734632 ) ) ;
#19653=CARTESIAN_POINT ( 'NONE',  ( -17.35679799567829207, 370.6823905601784759, 16.95518130045146421 ) ) ;
#19654=CARTESIAN_POINT ( 'NONE',  ( -48.68588794268853803, 316.9323905601784759, -3.978247347593583783 ) ) ;
#19656=CARTESIAN_POINT ( 'NONE',  ( -45.43829269268872650, 495.3698905683720568, 0.000000000000000000 ) ) ;
#19657=DIRECTION ( 'NONE',  ( -1.191790137725560488E-16, 1.000000000000000000, -0.000000000000000000 ) ) ;
#19658=CARTESIAN_POINT ( 'NONE',  ( -38.17536295476244135, 285.4323905683720568, 14.20200298773971781 ) ) ;
#19662=CARTESIAN_POINT ( 'NONE',  ( -42.88789093042842637, 276.3073905683720000, 9.489475012073734561 ) ) ;
#19663=VECTOR ( 'NONE', #13020, 1000.000000000000000 ) ;
#19664=CARTESIAN_POINT ( 'NONE',  ( -22.27502019258947996, 310.7448905683720000, -15.47720386886985544 ) ) ;
#19665=CARTESIAN_POINT ( 'NONE',  ( -32.01814843081343298, 257.5573905683720000, 16.75240474999999307 ) ) ;
#19666=CARTESIAN_POINT ( 'NONE',  ( -24.70764059509554755, 239.1823905765656093, -19.99999999999999289 ) ) ;
#19668=LINE ( 'NONE', #21392, #2008 ) ;
#19669=CARTESIAN_POINT ( 'NONE',  ( -45.43829269268870519, 375.6823905683720000, 3.332260488124734632 ) ) ;
#19671=CARTESIAN_POINT ( 'NONE',  ( -11.73070664223723547, 281.3073905601785327, 11.32908994701042005 ) ) ;
#19673=( BOUNDED_CURVE ( )  B_SPLINE_CURVE ( 2, ( #2013, #13581, #178, #18432, #9881, #1909, #3196, #4803, #16504, #11399, #8476, #18001, #6747, #1684, #13144, #9774, #16399 ),
 .UNSPECIFIED., .F., .T. ) 
 B_SPLINE_CURVE_WITH_KNOTS ( ( 3, 2, 2, 2, 2, 2, 2, 2, 3 ),
 ( 0.1875000000000001665, 0.1894531250000001665, 0.1914062500000001665, 0.1933593750000001665, 0.1953125000000001665, 0.1972656250000001665, 0.1992187500000001665, 0.2011718750000001665, 0.2031250000000001665 ),
 .UNSPECIFIED. ) 
 CURVE ( )  GEOMETRIC_REPRESENTATION_ITEM ( )  RATIONAL_B_SPLINE_CURVE ( ( 0.9999999999999983347, 0.9807852804032320959, 1.000000000000000000, 0.9807852804032304306, 1.000000000000000000, 0.9807852804032304306, 1.000000000000000000, 0.9807852804032304306, 1.000000000000000000, 0.9807852804032304306, 1.000000000000000000, 0.9807852804032304306, 1.000000000000000000, 0.9807852804032304306, 1.000000000000000000, 0.9807852804032287652, 1.000000000000001554 ) ) 
 REPRESENTATION_ITEM ( '' )  );
#19674=CARTESIAN_POINT ( 'NONE',  ( -8.685887942688534480, 267.3073905765655240, -3.978247347592740013 ) ) ;
#19675=CARTESIAN_POINT ( 'NONE',  ( -19.19641293061498999, 430.4323905683720000, -14.20200298773971603 ) ) ;
#19678=CARTESIAN_POINT ( 'NONE',  ( -28.68588794268871922, 429.7448905601785327, 19.99999999999999289 ) ) ;
#19681=ORIENTED_EDGE ( 'NONE', *, *, #13058, .F. ) ;
#19684=CARTESIAN_POINT ( 'NONE',  ( -48.68588794268870146, 297.2448905601784759, 0.000000000000000000 ) ) ;
#19685=DIRECTION ( 'NONE',  ( 1.191790137725560488E-16, -1.000000000000000000, 0.000000000000000000 ) ) ;
#19686=CARTESIAN_POINT ( 'NONE',  ( -28.68588794268871212, 347.8698905683720568, 16.75240474999999307 ) ) ;
#19687=CARTESIAN_POINT ( 'NONE',  ( -24.70764059509556532, 484.8073905765656946, 19.99999999999998934 ) ) ;
#19688=CARTESIAN_POINT ( 'NONE',  ( -45.43829269268871229, 373.8698905683720000, 0.000000000000000000 ) ) ;
#19690=CARTESIAN_POINT ( 'NONE',  ( -28.68588794268871922, 381.3698905683720568, -16.75240474999999307 ) ) ;
#19691=CARTESIAN_POINT ( 'NONE',  ( -40.01497788969912506, 323.5573905765655809, 16.95518130045146776 ) ) ;
#19692=CARTESIAN_POINT ( 'NONE',  ( -28.68588794268872277, 424.7448905601784759, -19.99999999999999289 ) ) ;
#19693=CARTESIAN_POINT ( 'NONE',  ( -16.84014894278198327, 290.1198905683720568, -11.84573899990672707 ) ) ;
#19694=CARTESIAN_POINT ( 'NONE',  ( -14.54375231895777532, 440.9948905601784759, 14.14213562373094568 ) ) ;
#19695=CARTESIAN_POINT ( 'NONE',  ( -42.88789093042844058, 446.3073905683720000, 9.489475012073736337 ) ) ;
#19699=DIRECTION ( 'NONE',  ( -1.191790137725560488E-16, 1.000000000000000000, -0.000000000000000000 ) ) ;
#19701=CARTESIAN_POINT ( 'NONE',  ( -42.88789093042843348, 354.4323905683720568, -9.489475012073736337 ) ) ;
#19702=CARTESIAN_POINT ( 'NONE',  ( -28.68588794268873343, 491.3698905683720568, -16.75240474999999307 ) ) ;
#19704=CARTESIAN_POINT ( 'NONE',  ( -17.35679799567830628, 490.6823905601784759, 16.95518130045146421 ) ) ;
#19705=CARTESIAN_POINT ( 'NONE',  ( -14.48388495494899075, 307.9323905683720000, 9.489475012073732785 ) ) ;
#19709=CARTESIAN_POINT ( 'NONE',  ( -28.68588794268869790, 259.7448905601784759, 19.99999999999999289 ) ) ;
#19714=CARTESIAN_POINT ( 'NONE',  ( -38.17536295476246266, 403.8073905683721136, -14.20200298773971426 ) ) ;
#19715=CYLINDRICAL_SURFACE ( 'NONE', #14208, 19.99999999999999645 ) ;
#19716=DIRECTION ( 'NONE',  ( -1.191790137725560488E-16, 1.000000000000000000, -0.000000000000000000 ) ) ;
#19717=CARTESIAN_POINT ( 'NONE',  ( -42.88789093042844058, 444.8073905683720568, 9.489475012073736337 ) ) ;
#19718=CARTESIAN_POINT ( 'NONE',  ( -28.68588794268872633, 451.3698905683720000, -16.75240474999999307 ) ) ;
#19722=CARTESIAN_POINT ( 'NONE',  ( -14.54375231895777354, 388.2448905765655809, -14.14213562373094746 ) ) ;
#19725=CARTESIAN_POINT ( 'NONE',  ( -40.01497788969914637, 430.4323905765655809, -16.95518130045146421 ) ) ;
#19727=CARTESIAN_POINT ( 'NONE',  ( -42.88789093042845479, 506.3073905683720568, 9.489475012073736337 ) ) ;
#19729=CYLINDRICAL_SURFACE ( 'NONE', #12680, 19.99999999999999645 ) ;
#19730=CARTESIAN_POINT ( 'NONE',  ( -17.35679799567830628, 463.8073905601784190, -16.95518130045146421 ) ) ;
#19731=CARTESIAN_POINT ( 'NONE',  ( -42.82802356641968089, 518.4948905601785327, 14.14213562373094923 ) ) ;
#19733=CARTESIAN_POINT ( 'NONE',  ( -11.93348319268872615, 410.0573905683720000, 3.332260488124728415 ) ) ;
#19735=CARTESIAN_POINT ( 'NONE',  ( -40.53162694259542320, 236.6198905683720284, 11.84573899990672885 ) ) ;
#19736=ORIENTED_EDGE ( 'NONE', *, *, #2411, .T. ) ;
#19739=CARTESIAN_POINT ( 'NONE',  ( -25.35362745456400191, 452.5573905683720568, -16.75240474999999307 ) ) ;
#19740=CARTESIAN_POINT ( 'NONE',  ( -14.54375231895775045, 225.7448905765656093, 14.14213562373094568 ) ) ;
#19743=CARTESIAN_POINT ( 'NONE',  ( -48.68588794268875120, 522.3073905765655809, 3.978247347593114824 ) ) ;
#19744=CARTESIAN_POINT ( 'NONE',  ( -21.25395633610896695, 220.6412455016266279, -15.05426537146665389 ) ) ;
#19745=ORIENTED_EDGE ( 'NONE', *, *, #19396, .T. ) ;
#19746=CARTESIAN_POINT ( 'NONE',  ( -32.01814843081345430, 501.6823905683720568, -16.75240474999999307 ) ) ;
#19748=EDGE_CURVE ( 'NONE', #15635, #15821, #16532, .T. ) ;
#19749=CARTESIAN_POINT ( 'NONE',  ( -48.68588794268871567, 442.3073905765656377, 3.978247347593168115 ) ) ;
#19751=CARTESIAN_POINT ( 'NONE',  ( -36.33955658999050797, 329.1198905601784759, 18.47759065022572500 ) ) ;
#19756=CARTESIAN_POINT ( 'NONE',  ( -8.685887942688738761, 496.9948905765655809, -2.449293598294705724E-15 ) ) ;
#19757=CARTESIAN_POINT ( 'NONE',  ( -13.20868407381885312, 319.7448905683720000, 6.410867750099229490 ) ) ;
#19759=CARTESIAN_POINT ( 'NONE',  ( -48.68588794268860198, 236.9323905601785043, -3.978247347593371508 ) ) ;
#19760=CARTESIAN_POINT ( 'NONE',  ( -28.68588794268870501, 274.7448905601784759, -19.99999999999999289 ) ) ;
#19761=DIRECTION ( 'NONE',  ( -1.191790137725560488E-16, 1.000000000000000000, -0.000000000000000000 ) ) ;
#19762=CARTESIAN_POINT ( 'NONE',  ( -45.43829269268869808, 285.6823905683720000, 3.332260488124734632 ) ) ;
#19763=CARTESIAN_POINT ( 'NONE',  ( -35.09675569278795848, 503.4948905683720568, -15.47720386886985544 ) ) ;
#19764=CARTESIAN_POINT ( 'NONE',  ( -24.70764059509555111, 370.0573905601783622, 19.99999999999998934 ) ) ;
#19766=CARTESIAN_POINT ( 'NONE',  ( -16.84014894278200103, 479.1198905683720000, 11.84573899990672530 ) ) ;
#19768=CARTESIAN_POINT ( 'NONE',  ( -40.53162694259543031, 275.1198905683720568, 11.84573899990672885 ) ) ;
#19770=ORIENTED_EDGE ( 'NONE', *, *, #4862, .T. ) ;
#19771=FACE_OUTER_BOUND ( 'NONE', #20841, .T. ) ;
#19772=CARTESIAN_POINT ( 'NONE',  ( -35.09675569278794427, 287.2448905683720000, 15.47720386886985366 ) ) ;
#19773=CARTESIAN_POINT ( 'NONE',  ( -42.88789093042841927, 254.4323905683720284, -9.489475012073734561 ) ) ;
#19774=CARTESIAN_POINT ( 'NONE',  ( -48.68588794268869435, 251.9948905765656093, 0.000000000000000000 ) ) ;
#19775=CARTESIAN_POINT ( 'NONE',  ( -8.685887942688742314, 573.2448905601785327, 2.449293598294706119E-15 ) ) ;
#19777=CARTESIAN_POINT ( 'NONE',  ( -42.88789093042841927, 264.8073905683721136, 9.489475012073736337 ) ) ;
#19778=CARTESIAN_POINT ( 'NONE',  ( -11.93348319268872260, 380.0573905683721136, 3.332260488124728415 ) ) ;
#19779=FACE_OUTER_BOUND ( 'NONE', #6431, .T. ) ;
#19780=CARTESIAN_POINT ( 'NONE',  ( -10.20829729246299777, 457.6198905765656377, -7.653668647301794969 ) ) ;
#19786=CARTESIAN_POINT ( 'NONE',  ( -44.16309181155857999, 413.2448905683720568, -6.410867750099231266 ) ) ;
#19789=CARTESIAN_POINT ( 'NONE',  ( -45.64106924314019409, 428.1823905601784759, 11.32908994701042715 ) ) ;
#19790=ORIENTED_EDGE ( 'NONE', *, *, #9878, .F. ) ;
#19793=CARTESIAN_POINT ( 'NONE',  ( -48.68588794268880093, 352.3073905765656377, 3.978247347592954952 ) ) ;
#19794=CARTESIAN_POINT ( 'NONE',  ( -42.82802356641965247, 305.9948905601784759, -14.14213562373094746 ) ) ;
#19797=CIRCLE ( 'NONE', #12554, 5.000000000000001776 ) ;
#19798=CARTESIAN_POINT ( 'NONE',  ( -38.17536295476245556, 353.8073905683720568, -14.20200298773971426 ) ) ;
#19800=CARTESIAN_POINT ( 'NONE',  ( -14.54375231895778597, 488.2448905765656377, -14.14213562373094746 ) ) ;
#19801=CARTESIAN_POINT ( 'NONE',  ( -32.01814843081344719, 361.6823905683720568, -16.75240474999999307 ) ) ;
#19805=CARTESIAN_POINT ( 'NONE',  ( -40.53162694259543741, 382.6198905683720568, -11.84573899990672707 ) ) ;
#19807=CARTESIAN_POINT ( 'NONE',  ( -11.73070664223723902, 306.0573905765655809, 11.32908994701042005 ) ) ;
#19809=CARTESIAN_POINT ( 'NONE',  ( -44.16309181155855867, 294.4948905683720000, 6.410867750099241924 ) ) ;
#19810=DIRECTION ( 'NONE',  ( -1.000000000000000000, 0.000000000000000000, 0.000000000000000000 ) ) ;
#19811=( BOUNDED_CURVE ( )  B_SPLINE_CURVE ( 2, ( #6366, #12975, #19566, #12695, #16058, #19392, #21233, #19500, #19709, #19287, #1551, #12910, #19603, #1337, #4577, #4679, #2857 ),
 .UNSPECIFIED., .F., .T. ) 
 B_SPLINE_CURVE_WITH_KNOTS ( ( 3, 2, 2, 2, 2, 2, 2, 2, 3 ),
 ( 0.8593750000000002220, 0.8613281250000002220, 0.8632812500000002220, 0.8652343750000002220, 0.8671875000000002220, 0.8691406250000002220, 0.8710937500000002220, 0.8730468750000002220, 0.8750000000000002220 ),
 .UNSPECIFIED. ) 
 CURVE ( )  GEOMETRIC_REPRESENTATION_ITEM ( )  RATIONAL_B_SPLINE_CURVE ( ( 0.9999999999999977796, 0.9807852804032326510, 1.000000000000000000, 0.9807852804032304306, 1.000000000000000000, 0.9807852804032304306, 1.000000000000000000, 0.9807852804032304306, 1.000000000000000000, 0.9807852804032304306, 1.000000000000000000, 0.9807852804032304306, 1.000000000000000000, 0.9807852804032304306, 1.000000000000000000, 0.9807852804032282101, 1.000000000000002220 ) ) 
 REPRESENTATION_ITEM ( '' )  );
#19812=CARTESIAN_POINT ( 'NONE',  ( -28.68588794268872277, 437.8698905683720568, 16.75240474999999307 ) ) ;
#19814=CARTESIAN_POINT ( 'NONE',  ( -14.54375231895778775, 513.4948905601785327, -14.14213562373094746 ) ) ;
#19818=VECTOR ( 'NONE', #14254, 1000.000000000000000 ) ;
#19819=CARTESIAN_POINT ( 'NONE',  ( -11.93348319268872260, 350.0573905683720000, 3.332260488124728415 ) ) ;
#19820=CARTESIAN_POINT ( 'NONE',  ( -28.68588794268872633, 476.3698905683720568, 16.75240474999999307 ) ) ;
#19821=AXIS2_PLACEMENT_3D ( 'NONE', #21194, #12441, #12871 ) ;
#19823=CARTESIAN_POINT ( 'NONE',  ( -21.03221929538693757, 484.1198905601785327, -18.47759065022572855 ) ) ;
#19824=CARTESIAN_POINT ( 'NONE',  ( -45.43829269268870519, 293.8698905683720568, 0.000000000000000000 ) ) ;
#19829=CARTESIAN_POINT ( 'NONE',  ( -45.43829269268871940, 395.6823905683719431, 3.332260488124734632 ) ) ;
#19830=DIRECTION ( 'NONE',  ( -1.000000000000000000, 0.000000000000000000, 0.000000000000000000 ) ) ;
#19832=CARTESIAN_POINT ( 'NONE',  ( -45.43829269268871229, 434.1823905683720568, 3.332260488124734632 ) ) ;
#19833=CARTESIAN_POINT ( 'NONE',  ( -38.17536295476245556, 445.4323905683720000, 14.20200298773971781 ) ) ;
#19834=CARTESIAN_POINT ( 'NONE',  ( -48.68588794268873698, 573.2448905601785327, 0.000000000000000000 ) ) ;
#19835=CARTESIAN_POINT ( 'NONE',  ( -10.20829729246298712, 367.6198905765656377, -7.653668647301794969 ) ) ;
#19841=CARTESIAN_POINT ( 'NONE',  ( -38.17536295476246977, 506.9323905683720568, 14.20200298773971781 ) ) ;
#19844=CARTESIAN_POINT ( 'NONE',  ( -14.48388495494900496, 399.4323905683720568, 9.489475012073732785 ) ) ;
#19846=CARTESIAN_POINT ( 'NONE',  ( -44.16309181155855157, 235.9948905683720284, 6.410867750099241924 ) ) ;
#19847=CARTESIAN_POINT ( 'NONE',  ( -38.17536295476245556, 372.3073905683721136, -14.20200298773971426 ) ) ;
#19849=CARTESIAN_POINT ( 'NONE',  ( -42.88789093042845479, 532.9323905683720568, -9.489475012073736337 ) ) ;
#19851=CARTESIAN_POINT ( 'NONE',  ( -13.20868407381887089, 450.9948905683720000, -6.410867750099233042 ) ) ;
#19852=CARTESIAN_POINT ( 'NONE',  ( -14.48388495494901740, 517.9323905683720568, 9.489475012073732785 ) ) ;
#19854=CARTESIAN_POINT ( 'NONE',  ( -28.68588794268871922, 429.7448905601785327, 19.99999999999999289 ) ) ;
#19855=CARTESIAN_POINT ( 'NONE',  ( -35.09675569278796559, 485.7448905683720568, 15.47720386886985366 ) ) ;
#19857=CARTESIAN_POINT ( 'NONE',  ( -13.20868407381887621, 498.2448905683720000, 6.410867750099229490 ) ) ;
#19860=CARTESIAN_POINT ( 'NONE',  ( -47.16347859291445843, 452.6198905765656377, 7.653668647301805628 ) ) ;
#19861=CARTESIAN_POINT ( 'NONE',  ( -42.82802356641965247, 300.7448905765656377, -14.14213562373094746 ) ) ;
#19862=CARTESIAN_POINT ( 'NONE',  ( -28.68588794268870146, 249.4948905765656093, -19.99999999999999289 ) ) ;
#19863=DIRECTION ( 'NONE',  ( -1.000000000000000000, 0.000000000000000000, 0.000000000000000000 ) ) ;
#19866=CARTESIAN_POINT ( 'NONE',  ( -48.68588794268871567, 437.2448905601785327, 0.000000000000000000 ) ) ;
#19869=CARTESIAN_POINT ( 'NONE',  ( -42.88789093042842637, 306.3073905683719431, 9.489475012073736337 ) ) ;
#19870=CARTESIAN_POINT ( 'NONE',  ( -40.01497788969915348, 528.8073905601785327, 16.95518130045146776 ) ) ;
#19871=CARTESIAN_POINT ( 'NONE',  ( -21.03221929538691271, 274.1198905601784759, -18.47759065022572855 ) ) ;
#19872=CARTESIAN_POINT ( 'NONE',  ( -24.70764059509555466, 414.8073905765656946, 19.99999999999998934 ) ) ;
#19873=CARTESIAN_POINT ( 'NONE',  ( -11.93348319268871371, 290.6823905683721136, -3.332260488124732856 ) ) ;
#19875=CARTESIAN_POINT ( 'NONE',  ( -28.68588794268872988, 507.8698905683720568, 16.75240474999999307 ) ) ;
#19877=VERTEX_POINT ( 'NONE', #6714 ) ;
#19878=CARTESIAN_POINT ( 'NONE',  ( -38.17536295476246977, 463.8073905683720000, -14.20200298773971426 ) ) ;
#19880=CARTESIAN_POINT ( 'NONE',  ( -28.68588794268870501, 271.3698905683720000, -16.75240474999999307 ) ) ;
#19884=CARTESIAN_POINT ( 'NONE',  ( -22.27502019258947641, 272.2448905683720568, -15.47720386886985544 ) ) ;
#19885=CARTESIAN_POINT ( 'NONE',  ( -35.09675569278793716, 257.2448905683720000, 15.47720386886985366 ) ) ;
#19886=CARTESIAN_POINT ( 'NONE',  ( -24.70764059509554755, 249.1823905765656093, -19.99999999999999289 ) ) ;
#19888=CARTESIAN_POINT ( 'NONE',  ( -10.20829729246297113, 232.8698905601784759, -7.653668647301794969 ) ) ;
#19890=CARTESIAN_POINT ( 'NONE',  ( -28.68588794268870146, 276.3698905683720000, 16.75240474999999307 ) ) ;
#19891=CARTESIAN_POINT ( 'NONE',  ( -38.17536295476245556, 363.8073905683720568, -14.20200298773971426 ) ) ;
#19892=CARTESIAN_POINT ( 'NONE',  ( -21.03221929538690205, 280.3698905601784759, 18.47759065022572500 ) ) ;
#19894=CARTESIAN_POINT ( 'NONE',  ( -25.35362745456398770, 426.6823905683720568, 16.75240474999998952 ) ) ;
#19897=CARTESIAN_POINT ( 'NONE',  ( -8.685887942688729879, 432.5573905601785327, -3.978247347593165895 ) ) ;
#19901=CARTESIAN_POINT ( 'NONE',  ( -35.09675569278796559, 523.4948905683720568, -15.47720386886985544 ) ) ;
#19902=CARTESIAN_POINT ( 'NONE',  ( -17.35679799567828496, 310.6823905601784759, 16.95518130045146421 ) ) ;
#19904=CARTESIAN_POINT ( 'NONE',  ( -35.09675569278795138, 347.2448905683720000, 15.47720386886985366 ) ) ;
#19905=ORIENTED_EDGE ( 'NONE', *, *, #13998, .T. ) ;
#19906=CARTESIAN_POINT ( 'NONE',  ( -32.66413529028189089, 479.8073905765655809, -19.99999999999999289 ) ) ;
#19907=CARTESIAN_POINT ( 'NONE',  ( -16.84014894278199037, 360.1198905683720000, -11.84573899990672707 ) ) ;
#19908=CARTESIAN_POINT ( 'NONE',  ( -45.43829269268871229, 363.8698905683720000, 0.000000000000000000 ) ) ;
#19910=CARTESIAN_POINT ( 'NONE',  ( -42.82802356641965247, 300.7448905765656377, -14.14213562373094746 ) ) ;
#19912=CARTESIAN_POINT ( 'NONE',  ( -25.35362745456398059, 271.0573905683719431, -16.75240474999999307 ) ) ;
#19914=CARTESIAN_POINT ( 'NONE',  ( -22.27502019258949773, 442.2448905683720000, -15.47720386886985544 ) ) ;
#19919=CARTESIAN_POINT ( 'NONE',  ( -28.68588794268874054, 573.2448905601785327, 0.000000000000000000 ) ) ;
#19922=CARTESIAN_POINT ( 'NONE',  ( -45.43829269268870519, 355.0573905683720568, -3.332260488124726194 ) ) ;
#19923=CARTESIAN_POINT ( 'NONE',  ( -42.88789093042844769, 482.9323905683720568, -9.489475012073736337 ) ) ;
#19924=ADVANCED_FACE ( 'NONE', ( #11586 ), #16467, .T. ) ;
#19926=CARTESIAN_POINT ( 'NONE',  ( -32.66413529028189089, 485.0573905601785327, -19.99999999999999289 ) ) ;
#19927=CARTESIAN_POINT ( 'NONE',  ( -32.01814843081344009, 301.6823905683720568, -16.75240474999999307 ) ) ;
#19931=EDGE_LOOP ( 'NONE', ( #9969, #13640, #2061, #4534, #8408 ) ) ;
#19933=CARTESIAN_POINT ( 'NONE',  ( -19.19641293061498999, 411.9323905683720000, -14.20200298773971603 ) ) ;
#19934=CARTESIAN_POINT ( 'NONE',  ( -48.68588794268872277, 477.2448905601784759, 0.000000000000000000 ) ) ;
#19935=CARTESIAN_POINT ( 'NONE',  ( -10.20829729246298889, 386.3698905765656377, 7.653668647301790529 ) ) ;
#19936=CARTESIAN_POINT ( 'NONE',  ( -11.93348319268872793, 419.1823905683720000, -3.332260488124732856 ) ) ;
#19937=CARTESIAN_POINT ( 'NONE',  ( -28.68588794268870146, 252.8698905683720000, -16.75240474999999307 ) ) ;
#19938=CARTESIAN_POINT ( 'NONE',  ( -35.09675569278795848, 445.7448905683720000, 15.47720386886985366 ) ) ;
#19939=( BOUNDED_CURVE ( )  B_SPLINE_CURVE ( 2, ( #2223, #19654, #14917, #1607, #8074, #15421, #3120, #3333, #13794, #6454, #6778, #16324, #8291, #13070, #20280, #18640, #14704 ),
 .UNSPECIFIED., .F., .T. ) 
 B_SPLINE_CURVE_WITH_KNOTS ( ( 3, 2, 2, 2, 2, 2, 2, 2, 3 ),
 ( 0.6875000000000002220, 0.6894531250000002220, 0.6914062500000002220, 0.6933593750000002220, 0.6953125000000002220, 0.6972656250000002220, 0.6992187500000002220, 0.7011718750000002220, 0.7031250000000002220 ),
 .UNSPECIFIED. ) 
 CURVE ( )  GEOMETRIC_REPRESENTATION_ITEM ( )  RATIONAL_B_SPLINE_CURVE ( ( 0.9999999999999977796, 0.9807852804032326510, 1.000000000000000000, 0.9807852804032304306, 1.000000000000000000, 0.9807852804032304306, 1.000000000000000000, 0.9807852804032304306, 1.000000000000000000, 0.9807852804032304306, 1.000000000000000000, 0.9807852804032304306, 1.000000000000000000, 0.9807852804032304306, 1.000000000000000000, 0.9807852804032282101, 1.000000000000002220 ) ) 
 REPRESENTATION_ITEM ( '' )  );
#19942=CARTESIAN_POINT ( 'NONE',  ( -17.35679799567829207, 365.4323905765656377, 16.95518130045146421 ) ) ;
#19946=CARTESIAN_POINT ( 'NONE',  ( -48.68588794268863040, 491.6823905765656946, -3.978247347593371508 ) ) ;
#19947=CARTESIAN_POINT ( 'NONE',  ( -44.16309181155858710, 504.7448905683720000, -6.410867750099231266 ) ) ;
#19948=VECTOR ( 'NONE', #6950, 1000.000000000000000 ) ;
#19950=LINE ( 'NONE', #8473, #12426 ) ;
#19951=CARTESIAN_POINT ( 'NONE',  ( -47.16347859291445133, 417.8698905601784759, 7.653668647301805628 ) ) ;
#19954=CARTESIAN_POINT ( 'NONE',  ( -22.27502019258949417, 412.2448905683720568, -15.47720386886985544 ) ) ;
#19956=CARTESIAN_POINT ( 'NONE',  ( -42.88789093042841927, 234.4323905683720284, -9.489475012073736337 ) ) ;
#19957=CARTESIAN_POINT ( 'NONE',  ( -11.93348319268872260, 368.5573905683720568, 3.332260488124728415 ) ) ;
#19959=CARTESIAN_POINT ( 'NONE',  ( -44.16309181155859420, 523.2448905683719431, -6.410867750099231266 ) ) ;
#19960=ORIENTED_EDGE ( 'NONE', *, *, #10736, .T. ) ;
#19961=CARTESIAN_POINT ( 'NONE',  ( -19.19641293061498999, 438.8073905683720000, 14.20200298773971426 ) ) ;
#19962=CARTESIAN_POINT ( 'NONE',  ( -11.93348319268874214, 529.1823905683719431, -3.332260488124732856 ) ) ;
#19963=ORIENTED_EDGE ( 'NONE', *, *, #11546, .T. ) ;
#19964=CARTESIAN_POINT ( 'NONE',  ( -10.20829729246299422, 431.6198905601785327, 7.653668647301790529 ) ) ;
#19965=CARTESIAN_POINT ( 'NONE',  ( -35.09675569278795848, 481.9948905683720000, -15.47720386886985544 ) ) ;
#19967=CARTESIAN_POINT ( 'NONE',  ( -28.68588794268872988, 496.3698905683720568, 16.75240474999999307 ) ) ;
#19969=CARTESIAN_POINT ( 'NONE',  ( -11.73070664223725856, 427.9323905765656377, -11.32908994701042715 ) ) ;
#19972=CARTESIAN_POINT ( 'NONE',  ( -48.68588794268887909, 452.3073905765655809, 3.978247347592742678 ) ) ;
#19976=CARTESIAN_POINT ( 'NONE',  ( -8.685887942688713892, 223.9102039777116886, 2.449293598294704541E-15 ) ) ;
#19977=CARTESIAN_POINT ( 'NONE',  ( -45.43829269268869808, 295.0573905683720000, -3.332260488124726194 ) ) ;
#19978=CARTESIAN_POINT ( 'NONE',  ( -11.73070664223726745, 531.3073905601785327, 11.32908994701042005 ) ) ;
#19979=CARTESIAN_POINT ( 'NONE',  ( -48.68588794268870146, 277.5573905601784190, 3.978247347593168115 ) ) ;
#19981=CARTESIAN_POINT ( 'NONE',  ( -35.09675569278793716, 283.4948905683720000, -15.47720386886985544 ) ) ;
#19982=ADVANCED_FACE ( 'NONE', ( #8222 ), #14851, .T. ) ;
#19984=CARTESIAN_POINT ( 'NONE',  ( -11.93348319268873858, 510.0573905683719431, 3.332260488124728859 ) ) ;
#19985=ORIENTED_EDGE ( 'NONE', *, *, #7877, .T. ) ;
#19986=CARTESIAN_POINT ( 'NONE',  ( -45.43829269268872650, 475.3698905683720568, 0.000000000000000000 ) ) ;
#19988=CARTESIAN_POINT ( 'NONE',  ( -40.01497788969914637, 410.4323905765655809, -16.95518130045146421 ) ) ;
#19989=CARTESIAN_POINT ( 'NONE',  ( -35.09675569278793006, 261.9948905683720000, -15.47720386886985544 ) ) ;
#19993=CARTESIAN_POINT ( 'NONE',  ( -14.48388495494898720, 269.4323905683720568, 9.489475012073731008 ) ) ;
#19994=CARTESIAN_POINT ( 'NONE',  ( -16.84014894278197616, 241.6198905683720284, -11.84573899990672707 ) ) ;
#19995=CARTESIAN_POINT ( 'NONE',  ( -48.68588794268869435, 241.6823905765655809, -3.978247347593158345 ) ) ;
#19996=CARTESIAN_POINT ( 'NONE',  ( -48.68588794268870146, 307.2448905601784759, 0.000000000000000000 ) ) ;
#19997=CARTESIAN_POINT ( 'NONE',  ( -36.33955658999049376, 235.3698905601784759, -18.47759065022572855 ) ) ;
#19998=CARTESIAN_POINT ( 'NONE',  ( -42.88789093042842637, 274.8073905683720000, 9.489475012073736337 ) ) ;
#19999=CARTESIAN_POINT ( 'NONE',  ( -14.48388495494899608, 349.4323905683720000, 9.489475012073732785 ) ) ;
#20005=CARTESIAN_POINT ( 'NONE',  ( -42.88789093042844058, 424.8073905683720000, 9.489475012073736337 ) ) ;
#20007=VERTEX_POINT ( 'NONE', #9953 ) ;
#20008=CARTESIAN_POINT ( 'NONE',  ( -36.33955658999052218, 399.1198905601784759, 18.47759065022572500 ) ) ;
#20010=EDGE_LOOP ( 'NONE', ( #10253, #17620, #19109, #7681 ) ) ;
#20012=CARTESIAN_POINT ( 'NONE',  ( -11.93348319268874214, 530.3698905683720568, -2.051577885510841163E-15 ) ) ;
#20014=CARTESIAN_POINT ( 'NONE',  ( -36.33955658999050087, 295.3698905601784759, -18.47759065022572855 ) ) ;
#20017=CARTESIAN_POINT ( 'NONE',  ( -13.20868407381885312, 319.7448905683720000, 6.410867750099229490 ) ) ;
#20018=CARTESIAN_POINT ( 'NONE',  ( -25.35362745456399125, 361.0573905683720000, -16.75240474999999307 ) ) ;
#20019=CARTESIAN_POINT ( 'NONE',  ( -42.88789093042843348, 372.9323905683720568, -9.489475012073734561 ) ) ;
#20021=EDGE_CURVE ( 'NONE', #16325, #18084, #12094, .T. ) ;
#20022=CARTESIAN_POINT ( 'NONE',  ( -32.66413529028186957, 304.1823905765656377, 19.99999999999999289 ) ) ;
#20023=CARTESIAN_POINT ( 'NONE',  ( -43.68588794268869435, 200.1437886375728965, -2.037320803886357560E-15 ) ) ;
#20024=CARTESIAN_POINT ( 'NONE',  ( -22.27502019258947641, 260.7448905683720000, -15.47720386886985544 ) ) ;
#20025=CARTESIAN_POINT ( 'NONE',  ( -48.68588794268880804, 437.5573905601785327, 3.978247347592954952 ) ) ;
#20026=CARTESIAN_POINT ( 'NONE',  ( -22.27502019258949417, 422.2448905683720568, -15.47720386886985544 ) ) ;
#20028=CARTESIAN_POINT ( 'NONE',  ( -48.68588794268867304, 516.9323905601784190, -3.978247347593264927 ) ) ;
#20031=EDGE_CURVE ( 'NONE', #4181, #14447, #6979, .T. ) ;
#20032=CARTESIAN_POINT ( 'NONE',  ( -22.27502019258949062, 486.9948905683720568, 15.47720386886985189 ) ) ;
#20034=CARTESIAN_POINT ( 'NONE',  ( -8.685887942688735208, 472.2448905601784759, -2.449293598294705724E-15 ) ) ;
#20035=CARTESIAN_POINT ( 'NONE',  ( -44.16309181155856578, 313.2448905683720000, -6.410867750099231266 ) ) ;
#20039=CARTESIAN_POINT ( 'NONE',  ( -28.68588794268874054, 573.2448905601785327, 0.000000000000000000 ) ) ;
#20040=CARTESIAN_POINT ( 'NONE',  ( -11.93348319268872437, 390.0573905683720568, 3.332260488124728859 ) ) ;
#20043=CARTESIAN_POINT ( 'NONE',  ( -40.53162694259544452, 432.6198905683720000, -11.84573899990672707 ) ) ;
#20044=CARTESIAN_POINT ( 'NONE',  ( -14.48388495494898720, 261.3073905683720568, -9.489475012073736337 ) ) ;
#20046=CARTESIAN_POINT ( 'NONE',  ( -35.09675569278795138, 431.9948905683720568, -15.47720386886985544 ) ) ;
#20050=CARTESIAN_POINT ( 'NONE',  ( -17.35679799567829207, 355.4323905765655809, 16.95518130045146421 ) ) ;
#20052=CARTESIAN_POINT ( 'NONE',  ( -28.68588794268874054, 573.2448905601785327, 0.000000000000000000 ) ) ;
#20053=CARTESIAN_POINT ( 'NONE',  ( -25.35362745456397704, 326.6823905683720568, 16.75240474999998952 ) ) ;
#20055=CARTESIAN_POINT ( 'NONE',  ( -14.48388495494901029, 479.4323905683720568, 9.489475012073732785 ) ) ;
#20059=CARTESIAN_POINT ( 'NONE',  ( -17.35679799567829562, 420.6823905601784190, 16.95518130045146421 ) ) ;
#20060=CARTESIAN_POINT ( 'NONE',  ( -45.43829269268870519, 385.0573905683720000, -3.332260488124726194 ) ) ;
#20064=CARTESIAN_POINT ( 'NONE',  ( -45.43829269268869098, 235.6823905683720284, 3.332260488124734632 ) ) ;
#20065=CARTESIAN_POINT ( 'NONE',  ( -28.68588794268871567, 361.3698905683720568, -16.75240474999999307 ) ) ;
#20067=ORIENTED_EDGE ( 'NONE', *, *, #4137, .T. ) ;
#20068=CARTESIAN_POINT ( 'NONE',  ( -14.48388495494901917, 529.8073905683720568, -9.489475012073736337 ) ) ;
#20070=CARTESIAN_POINT ( 'NONE',  ( -32.01814843081344719, 443.1823905683720568, -16.75240474999999307 ) ) ;
#20071=CARTESIAN_POINT ( 'NONE',  ( -32.01814843081346851, 526.0573905683720568, 16.75240474999999307 ) ) ;
#20074=CARTESIAN_POINT ( 'NONE',  ( -47.16347859291445133, 427.8698905601784759, 7.653668647301805628 ) ) ;
#20075=CARTESIAN_POINT ( 'NONE',  ( -19.19641293061499709, 480.4323905683720568, -14.20200298773971603 ) ) ;
#20077=CARTESIAN_POINT ( 'NONE',  ( -13.20868407381887621, 489.4948905683720568, -6.410867750099233042 ) ) ;
#20080=CARTESIAN_POINT ( 'NONE',  ( -14.54375231895777887, 428.2448905765656377, -14.14213562373094746 ) ) ;
#20084=DIRECTION ( 'NONE',  ( 1.000000000000000000, 1.191790137725560488E-16, 0.000000000000000000 ) ) ;
#20085=APPLICATION_CONTEXT ( 'automotive_design' ) ;
#20088=CARTESIAN_POINT ( 'NONE',  ( -42.87299489053027912, 204.0036020648173292, -4.871053504435129078 ) ) ;
#20089=CARTESIAN_POINT ( 'NONE',  ( -42.88789093042842637, 304.4323905683720000, -9.489475012073736337 ) ) ;
#20091=CARTESIAN_POINT ( 'NONE',  ( -21.03221929538691271, 264.1198905601784759, -18.47759065022572855 ) ) ;
#20092=CARTESIAN_POINT ( 'NONE',  ( -31.26501780185373391, 205.1437886375728965, 5.000000000000001776 ) ) ;
#20093=CARTESIAN_POINT ( 'NONE',  ( -25.35362745456398059, 282.5573905683720568, -16.75240474999999307 ) ) ;
#20096=AXIS2_PLACEMENT_3D ( 'NONE', #14517, #21101, #4659 ) ;
#20097=CARTESIAN_POINT ( 'NONE',  ( -19.19641293061499709, 508.8073905683720000, 14.20200298773971426 ) ) ;
#20098=ORIENTED_EDGE ( 'NONE', *, *, #5468, .T. ) ;
#20099=CARTESIAN_POINT ( 'NONE',  ( -25.35362745456399125, 458.1823905683720000, 16.75240474999998952 ) ) ;
#20100=CYLINDRICAL_SURFACE ( 'NONE', #8290, 19.99999999999999645 ) ;
#20101=CARTESIAN_POINT ( 'NONE',  ( -28.68588794268870501, 261.3698905683720000, -16.75240474999999307 ) ) ;
#20104=CARTESIAN_POINT ( 'NONE',  ( -16.84014894278197971, 271.6198905683720568, -11.84573899990672707 ) ) ;
#20105=CARTESIAN_POINT ( 'NONE',  ( -25.35362745456396638, 238.1823905683720852, 16.75240474999998952 ) ) ;
#20106=CARTESIAN_POINT ( 'NONE',  ( -8.685887942688893304, 311.9323905601784190, 3.978247347593586447 ) ) ;
#20108=CARTESIAN_POINT ( 'NONE',  ( -28.68588794268870501, 261.3698905683720000, -16.75240474999999307 ) ) ;
#20109=AXIS2_PLACEMENT_3D ( 'NONE', #11644, #8498, #3738 ) ;
#20110=CARTESIAN_POINT ( 'NONE',  ( -22.27502019258948707, 352.2448905683720000, -15.47720386886985544 ) ) ;
#20111=CARTESIAN_POINT ( 'NONE',  ( -10.20829729246300310, 502.8698905601784759, -7.653668647301794969 ) ) ;
#20112=EDGE_CURVE ( 'NONE', #11812, #9678, #11010, .T. ) ;
#20113=CARTESIAN_POINT ( 'NONE',  ( -38.17536295476246266, 412.3073905683720000, -14.20200298773971426 ) ) ;
#20114=CARTESIAN_POINT ( 'NONE',  ( -40.01497788969913927, 340.4323905765656946, -16.95518130045146421 ) ) ;
#20116=CARTESIAN_POINT ( 'NONE',  ( -40.01497788969914637, 415.6823905601785327, -16.95518130045146421 ) ) ;
#20117=ORIENTED_EDGE ( 'NONE', *, *, #13954, .T. ) ;
#20121=CARTESIAN_POINT ( 'NONE',  ( -28.68588794268873343, 527.8698905683720568, 16.75240474999999307 ) ) ;
#20122=CARTESIAN_POINT ( 'NONE',  ( -17.35679799567828141, 280.6823905601784190, 16.95518130045146421 ) ) ;
#20123=CARTESIAN_POINT ( 'NONE',  ( -43.67243589781771362, 210.1033101532991338, -0.6559853996653195463 ) ) ;
#20126=CARTESIAN_POINT ( 'NONE',  ( -22.27502019258948351, 332.2448905683720568, -15.47720386886985544 ) ) ;
#20128=CARTESIAN_POINT ( 'NONE',  ( -19.19641293061498288, 367.3073905683720000, 14.20200298773971426 ) ) ;
#20129=CARTESIAN_POINT ( 'NONE',  ( -42.88789093042843348, 362.9323905683720568, -9.489475012073734561 ) ) ;
#20131=CARTESIAN_POINT ( 'NONE',  ( -45.64106924314017988, 311.0573905765656377, -11.32908994701042715 ) ) ;
#20133=CARTESIAN_POINT ( 'NONE',  ( -28.68588794268870501, 261.3698905683720000, -16.75240474999999307 ) ) ;
#20136=CARTESIAN_POINT ( 'NONE',  ( -16.84014894278199748, 421.6198905683720000, -11.84573899990672707 ) ) ;
#20137=DIRECTION ( 'NONE',  ( -1.191790137725560488E-16, 1.000000000000000000, -0.000000000000000000 ) ) ;
#20138=CARTESIAN_POINT ( 'NONE',  ( -17.35679799567829562, 353.8073905601785327, -16.95518130045146421 ) ) ;
#20139=CARTESIAN_POINT ( 'NONE',  ( -47.16347859291443712, 272.6198905765655809, 7.653668647301805628 ) ) ;
#20140=CARTESIAN_POINT ( 'NONE',  ( -32.66413529028187668, 409.4323905601784759, 19.99999999999999289 ) ) ;
#20141=CARTESIAN_POINT ( 'NONE',  ( -42.88789093042843348, 336.3073905683720568, 9.489475012073736337 ) ) ;
#20142=CARTESIAN_POINT ( 'NONE',  ( -28.68588794268872277, 456.3698905683720000, 16.75240474999999307 ) ) ;
#20144=CARTESIAN_POINT ( 'NONE',  ( -48.68588794268872277, 456.9323905601784190, -3.978247347593158345 ) ) ;
#20145=CARTESIAN_POINT ( 'NONE',  ( -28.68588794268870856, 301.3698905683720568, -16.75240474999999307 ) ) ;
#20149=CYLINDRICAL_SURFACE ( 'NONE', #13984, 19.99999999999999645 ) ;
#20151=CARTESIAN_POINT ( 'NONE',  ( -14.48388495494899963, 379.4323905683720568, 9.489475012073731008 ) ) ;
#20154=CARTESIAN_POINT ( 'NONE',  ( -35.09675569278795848, 425.7448905683720000, 15.47720386886985366 ) ) ;
#20155=CARTESIAN_POINT ( 'NONE',  ( -11.93348319268871194, 270.0573905683719431, 3.332260488124728415 ) ) ;
#20156=CARTESIAN_POINT ( 'NONE',  ( -38.17536295476245556, 425.4323905683719431, 14.20200298773971781 ) ) ;
#20160=CARTESIAN_POINT ( 'NONE',  ( -24.70764059509555111, 364.8073905765656377, 19.99999999999998934 ) ) ;
#20161=CARTESIAN_POINT ( 'NONE',  ( -24.70764059509554755, 274.4323905601784759, -19.99999999999999289 ) ) ;
#20162=CARTESIAN_POINT ( 'NONE',  ( -44.16309181155856578, 323.2448905683720000, -6.410867750099231266 ) ) ;
#20163=CARTESIAN_POINT ( 'NONE',  ( -45.43829269268873361, 533.8698905683720568, 0.000000000000000000 ) ) ;
#20164=CARTESIAN_POINT ( 'NONE',  ( -28.68588794268872633, 477.8698905683720568, 16.75240474999999307 ) ) ;
#20166=CARTESIAN_POINT ( 'NONE',  ( -24.70764059509555821, 434.8073905765656377, 19.99999999999998934 ) ) ;
#20170=CARTESIAN_POINT ( 'NONE',  ( -42.88789093042844058, 396.3073905683719431, 9.489475012073736337 ) ) ;
#20171=DIRECTION ( 'NONE',  ( -1.191790137725560488E-16, 1.000000000000000000, -0.000000000000000000 ) ) ;
#20172=CARTESIAN_POINT ( 'NONE',  ( -10.20829729246300488, 522.8698905601785327, -7.653668647301794969 ) ) ;
#20173=CARTESIAN_POINT ( 'NONE',  ( -11.93348319268872260, 359.1823905683720000, -3.332260488124732856 ) ) ;
#20175=CARTESIAN_POINT ( 'NONE',  ( -22.27502019258950483, 520.7448905683720568, -15.47720386886985544 ) ) ;
#20177=CARTESIAN_POINT ( 'NONE',  ( -45.43829269268872650, 524.1823905683720568, 3.332260488124734632 ) ) ;
#20178=ORIENTED_EDGE ( 'NONE', *, *, #15327, .T. ) ;
#20179=CARTESIAN_POINT ( 'NONE',  ( -14.48388495494901029, 477.9323905683721136, 9.489475012073732785 ) ) ;
#20181=CARTESIAN_POINT ( 'NONE',  ( -45.43829269268872650, 483.8698905683720568, 0.000000000000000000 ) ) ;
#20183=CARTESIAN_POINT ( 'NONE',  ( -14.54375231895777709, 418.2448905765655809, -14.14213562373094746 ) ) ;
#20184=CARTESIAN_POINT ( 'NONE',  ( -28.68588794268872633, 474.4948905765656377, 19.99999999999999289 ) ) ;
#20186=LINE ( 'NONE', #2128, #16021 ) ;
#20189=CARTESIAN_POINT ( 'NONE',  ( -28.68588794268870501, 297.8698905683720000, 16.75240474999999307 ) ) ;
#20190=CARTESIAN_POINT ( 'NONE',  ( -47.16347859291446554, 527.8698905601784190, 7.653668647301805628 ) ) ;
#20191=CARTESIAN_POINT ( 'NONE',  ( -45.43829269268871229, 445.0573905683720000, -3.332260488124726194 ) ) ;
#20193=( BOUNDED_CURVE ( )  B_SPLINE_CURVE ( 2, ( #8239, #5320, #14869, #8349, #14973, #13347, #799, #17228, #5534, #13992, #688, #12139, #12249, #7255, #18725, #8991, #903 ),
 .UNSPECIFIED., .F., .T. ) 
 B_SPLINE_CURVE_WITH_KNOTS ( ( 3, 2, 2, 2, 2, 2, 2, 2, 3 ),
 ( 0.5000000000000002220, 0.5019531250000002220, 0.5039062500000002220, 0.5058593750000002220, 0.5078125000000002220, 0.5097656250000002220, 0.5117187500000002220, 0.5136718750000002220, 0.5156250000000002220 ),
 .UNSPECIFIED. ) 
 CURVE ( )  GEOMETRIC_REPRESENTATION_ITEM ( )  RATIONAL_B_SPLINE_CURVE ( ( 0.9999999999999977796, 0.9807852804032326510, 1.000000000000000000, 0.9807852804032304306, 1.000000000000000000, 0.9807852804032304306, 1.000000000000000000, 0.9807852804032304306, 1.000000000000000000, 0.9807852804032304306, 1.000000000000000000, 0.9807852804032304306, 1.000000000000000000, 0.9807852804032304306, 1.000000000000000000, 0.9807852804032282101, 1.000000000000002220 ) ) 
 REPRESENTATION_ITEM ( '' )  );
#20194=CARTESIAN_POINT ( 'NONE',  ( -40.53162694259542320, 264.1198905683720568, -11.84573899990672707 ) ) ;
#20195=EDGE_CURVE ( 'NONE', #13560, #13932, #10010, .T. ) ;
#20198=CARTESIAN_POINT ( 'NONE',  ( -22.27502019258949417, 498.4948905683720568, 15.47720386886985189 ) ) ;
#20199=ADVANCED_FACE ( 'NONE', ( #14610 ), #7670, .T. ) ;
#20201=VERTEX_POINT ( 'NONE', #12763 ) ;
#20202=CARTESIAN_POINT ( 'NONE',  ( -25.35362745456400546, 472.5573905683720568, -16.75240474999999307 ) ) ;
#20204=CARTESIAN_POINT ( 'NONE',  ( -40.53162694259542320, 255.1198905683720284, 11.84573899990672885 ) ) ;
#20206=LINE ( 'NONE', #217, #4533 ) ;
#20207=CARTESIAN_POINT ( 'NONE',  ( -25.35362745456396993, 268.1823905683720000, 16.75240474999998952 ) ) ;
#20208=CARTESIAN_POINT ( 'NONE',  ( -11.73070664223724968, 391.3073905601784759, 11.32908994701042005 ) ) ;
#20209=CARTESIAN_POINT ( 'NONE',  ( -25.35362745456396638, 248.1823905683720568, 16.75240474999998952 ) ) ;
#20211=CARTESIAN_POINT ( 'NONE',  ( -14.54375231895775933, 310.9948905601784759, 14.14213562373094568 ) ) ;
#20213=CARTESIAN_POINT ( 'NONE',  ( -45.43829269268869808, 273.5573905683720000, -3.332260488124726194 ) ) ;
#20214=CARTESIAN_POINT ( 'NONE',  ( -32.01814843081344719, 353.1823905683720568, -16.75240474999999307 ) ) ;
#20216=CARTESIAN_POINT ( 'NONE',  ( -22.27502019258949417, 410.7448905683720568, -15.47720386886985544 ) ) ;
#20218=CARTESIAN_POINT ( 'NONE',  ( -8.685887942688726326, 402.5573905601784190, -3.978247347593165895 ) ) ;
#20219=ORIENTED_EDGE ( 'NONE', *, *, #3878, .F. ) ;
#20220=DIRECTION ( 'NONE',  ( -1.191790137725560488E-16, 1.000000000000000000, -0.000000000000000000 ) ) ;
#20223=CARTESIAN_POINT ( 'NONE',  ( -25.35362745456399836, 518.1823905683720568, 16.75240474999998952 ) ) ;
#20224=CARTESIAN_POINT ( 'NONE',  ( -8.685887942688713892, 291.9323905601784759, 3.978247347593161010 ) ) ;
#20225=CARTESIAN_POINT ( 'NONE',  ( -36.33955658999050087, 320.1198905765656377, -18.47759065022572855 ) ) ;
#20226=ORIENTED_EDGE ( 'NONE', *, *, #17994, .T. ) ;
#20227=CARTESIAN_POINT ( 'NONE',  ( -11.93348319268871727, 330.0573905683720000, 3.332260488124728859 ) ) ;
#20228=EDGE_LOOP ( 'NONE', ( #1004, #9786, #17065, #8094 ) ) ;
#20229=CARTESIAN_POINT ( 'NONE',  ( -16.84014894278198327, 337.6198905683720000, 11.84573899990672530 ) ) ;
#20230=CARTESIAN_POINT ( 'NONE',  ( -14.48388495494899963, 367.9323905683720000, 9.489475012073731008 ) ) ;
#20231=CARTESIAN_POINT ( 'NONE',  ( -8.685887942688715668, 306.6823905765655809, 3.978247347593161010 ) ) ;
#20233=CARTESIAN_POINT ( 'NONE',  ( -35.09675569278794427, 275.7448905683720568, 15.47720386886985366 ) ) ;
#20234=CARTESIAN_POINT ( 'NONE',  ( -43.68588794268869435, 200.1437886375728397, 0.3328713742805498588 ) ) ;
#20235=CARTESIAN_POINT ( 'NONE',  ( -19.19641293061498999, 411.9323905683720000, -14.20200298773971603 ) ) ;
#20239=CARTESIAN_POINT ( 'NONE',  ( -11.93348319268871727, 330.3698905683720000, -2.051577885510841163E-15 ) ) ;
#20240=CARTESIAN_POINT ( 'NONE',  ( -38.17536295476246266, 465.4323905683720000, 14.20200298773971781 ) ) ;
#20241=ORIENTED_EDGE ( 'NONE', *, *, #19009, .T. ) ;
#20242=CARTESIAN_POINT ( 'NONE',  ( -24.70764059509556532, 470.0573905601784759, 19.99999999999998934 ) ) ;
#20243=CARTESIAN_POINT ( 'NONE',  ( -45.43829269268869808, 284.1823905683720568, 3.332260488124734632 ) ) ;
#20244=EDGE_CURVE ( 'NONE', #13932, #6110, #19295, .T. ) ;
#20246=CARTESIAN_POINT ( 'NONE',  ( -35.86044580198795018, 223.9104597372275123, 18.66884633871304899 ) ) ;
#20248=CYLINDRICAL_SURFACE ( 'NONE', #3946, 19.99999999999999645 ) ;
#20249=CARTESIAN_POINT ( 'NONE',  ( -28.68588794268870856, 339.7448905601784759, 19.99999999999999289 ) ) ;
#20250=( BOUNDED_CURVE ( )  B_SPLINE_CURVE ( 2, ( #10006, #11747, #8386, #21377, #11533, #9899, #16521, #10117, #19862, #11640, #19640, #13488, #21268, #301, #11853, #88, #13052 ),
 .UNSPECIFIED., .F., .T. ) 
 B_SPLINE_CURVE_WITH_KNOTS ( ( 3, 2, 2, 2, 2, 2, 2, 2, 3 ),
 ( 0.8750000000000002220, 0.8769531250000002220, 0.8789062500000002220, 0.8808593750000002220, 0.8828125000000002220, 0.8847656250000002220, 0.8867187500000002220, 0.8886718750000002220, 0.8906250000000002220 ),
 .UNSPECIFIED. ) 
 CURVE ( )  GEOMETRIC_REPRESENTATION_ITEM ( )  RATIONAL_B_SPLINE_CURVE ( ( 0.9999999999999977796, 0.9807852804032326510, 1.000000000000000000, 0.9807852804032304306, 1.000000000000000000, 0.9807852804032304306, 1.000000000000000000, 0.9807852804032304306, 1.000000000000000000, 0.9807852804032304306, 1.000000000000000000, 0.9807852804032304306, 1.000000000000000000, 0.9807852804032304306, 1.000000000000000000, 0.9807852804032282101, 1.000000000000002220 ) ) 
 REPRESENTATION_ITEM ( '' )  );
#20251=CARTESIAN_POINT ( 'NONE',  ( -40.53162694259543031, 295.1198905683720000, 11.84573899990672885 ) ) ;
#20252=CARTESIAN_POINT ( 'NONE',  ( -13.20868407381886023, 379.7448905683720000, 6.410867750099229490 ) ) ;
#20254=CARTESIAN_POINT ( 'NONE',  ( -17.35679799567828852, 293.8073905601784759, -16.95518130045146421 ) ) ;
#20257=CARTESIAN_POINT ( 'NONE',  ( -16.84014894278199392, 417.6198905683720000, 11.84573899990672530 ) ) ;
#20258=CARTESIAN_POINT ( 'NONE',  ( -16.84014894278197971, 261.6198905683720568, -11.84573899990672707 ) ) ;
#20259=CARTESIAN_POINT ( 'NONE',  ( -25.35362745456399836, 421.0573905683720000, -16.75240474999999307 ) ) ;
#20260=VECTOR ( 'NONE', #3433, 1000.000000000000000 ) ;
#20261=CARTESIAN_POINT ( 'NONE',  ( -36.33955658999050797, 360.1198905765656377, -18.47759065022572855 ) ) ;
#20262=CARTESIAN_POINT ( 'NONE',  ( -47.16347859291443712, 276.6198905601784759, -7.653668647301793193 ) ) ;
#20263=CARTESIAN_POINT ( 'NONE',  ( -11.93348319268871549, 319.1823905683720568, -3.332260488124732856 ) ) ;
#20264=CARTESIAN_POINT ( 'NONE',  ( -40.53162694259545162, 474.1198905683720568, -11.84573899990672707 ) ) ;
#20268=CARTESIAN_POINT ( 'NONE',  ( -11.73070664223724258, 303.1823905601784190, -11.32908994701042538 ) ) ;
#20270=CARTESIAN_POINT ( 'NONE',  ( -22.27502019258949062, 382.2448905683720000, -15.47720386886985544 ) ) ;
#20272=CARTESIAN_POINT ( 'NONE',  ( -11.73070664223726745, 531.3073905601785327, 11.32908994701042005 ) ) ;
#20273=CARTESIAN_POINT ( 'NONE',  ( -42.88789093042843348, 352.9323905683721136, -9.489475012073736337 ) ) ;
#20274=EDGE_CURVE ( 'NONE', #7137, #15902, #9315, .T. ) ;
#20277=CARTESIAN_POINT ( 'NONE',  ( -40.53162694259545873, 522.6198905683720568, -11.84573899990672707 ) ) ;
#20280=CARTESIAN_POINT ( 'NONE',  ( -10.20829729246298001, 312.8698905601784759, -7.653668647301794969 ) ) ;
#20282=CARTESIAN_POINT ( 'NONE',  ( -8.685887942688742314, 526.9948905765655809, -2.449293598294705724E-15 ) ) ;
#20283=CARTESIAN_POINT ( 'NONE',  ( -42.88789093042844769, 474.8073905683720000, 9.489475012073736337 ) ) ;
#20285=CARTESIAN_POINT ( 'NONE',  ( -40.53162694259545162, 482.6198905683720000, -11.84573899990672707 ) ) ;
#20288=CARTESIAN_POINT ( 'NONE',  ( -40.01497788969914637, 420.4323905765655809, -16.95518130045146421 ) ) ;
#20291=PLANE ( 'NONE',  #2894 ) ;
#20292=CYLINDRICAL_SURFACE ( 'NONE', #20814, 19.99999999999999645 ) ;
#20295=CARTESIAN_POINT ( 'NONE',  ( -28.68588794268872277, 434.7448905601784759, -19.99999999999999289 ) ) ;
#20297=CARTESIAN_POINT ( 'NONE',  ( -13.20868407381885135, 290.9948905683720000, -6.410867750099233042 ) ) ;
#20299=CARTESIAN_POINT ( 'NONE',  ( -28.68588794268872633, 442.8698905683720568, -16.75240474999999307 ) ) ;
#20301=CARTESIAN_POINT ( 'NONE',  ( -38.17536295476244845, 273.8073905683720000, -14.20200298773971426 ) ) ;
#20305=CARTESIAN_POINT ( 'NONE',  ( -11.73070664223727100, 533.1823905601784190, -11.32908994701042538 ) ) ;
#20306=CARTESIAN_POINT ( 'NONE',  ( -11.93348319268873681, 490.3698905683720568, -2.051577885510841163E-15 ) ) ;
#20307=ORIENTED_EDGE ( 'NONE', *, *, #9439, .T. ) ;
#20308=CARTESIAN_POINT ( 'NONE',  ( -11.93348319268873503, 470.0573905683720568, 3.332260488124728415 ) ) ;
#20309=CARTESIAN_POINT ( 'NONE',  ( -48.68588794268871567, 411.9948905765656377, 0.000000000000000000 ) ) ;
#20310=CARTESIAN_POINT ( 'NONE',  ( -28.68588794268870146, 251.3698905683720000, -16.75240474999999307 ) ) ;
#20313=CARTESIAN_POINT ( 'NONE',  ( -28.68588794268872633, 474.4948905765656377, 19.99999999999999289 ) ) ;
#20315=CARTESIAN_POINT ( 'NONE',  ( -42.88789093042841927, 244.4323905683720284, -9.489475012073734561 ) ) ;
#20316=CARTESIAN_POINT ( 'NONE',  ( -24.70764059509556532, 419.1823905765655809, -19.99999999999999289 ) ) ;
#20317=CARTESIAN_POINT ( 'NONE',  ( -8.685887942688706786, 232.5573905601785043, -3.978247347593165895 ) ) ;
#20318=CARTESIAN_POINT ( 'NONE',  ( -22.27502019258947286, 250.7448905683720000, -15.47720386886985544 ) ) ;
#20319=CARTESIAN_POINT ( 'NONE',  ( -11.93348319268872082, 360.3698905683720568, -2.051577885510841163E-15 ) ) ;
#20321=CARTESIAN_POINT ( 'NONE',  ( -22.27502019258947996, 396.9948905683720568, 15.47720386886985189 ) ) ;
#20324=CARTESIAN_POINT ( 'NONE',  ( -10.20829729246299067, 411.6198905601784759, 7.653668647301790529 ) ) ;
#20330=CARTESIAN_POINT ( 'NONE',  ( -32.01814843081346851, 523.1823905683720568, -16.75240474999999307 ) ) ;
#20331=CARTESIAN_POINT ( 'NONE',  ( -45.64106924314017988, 288.1823905601785327, 11.32908994701042715 ) ) ;
#20334=CARTESIAN_POINT ( 'NONE',  ( -32.01814843081344719, 333.1823905683719431, -16.75240474999999307 ) ) ;
#20336=CARTESIAN_POINT ( 'NONE',  ( -28.68588794268871567, 351.3698905683720568, -16.75240474999999307 ) ) ;
#20337=CARTESIAN_POINT ( 'NONE',  ( -28.68588794268871212, 356.3698905683720568, 16.75240474999999307 ) ) ;
#20338=CARTESIAN_POINT ( 'NONE',  ( -48.68588794268870146, 291.9948905765656377, 0.000000000000000000 ) ) ;
#20340=CARTESIAN_POINT ( 'NONE',  ( -16.84014894278197971, 270.1198905683720568, -11.84573899990672707 ) ) ;
#20342=CARTESIAN_POINT ( 'NONE',  ( -22.27502019258948351, 408.4948905683720000, 15.47720386886985189 ) ) ;
#20344=CARTESIAN_POINT ( 'NONE',  ( -8.685887942688735208, 548.2448905601784190, 2.449293598294706513E-15 ) ) ;
#20346=CARTESIAN_POINT ( 'NONE',  ( -40.01497788969913927, 408.8073905601784759, 16.95518130045146776 ) ) ;
#20347=CARTESIAN_POINT ( 'NONE',  ( -38.17536295476245556, 333.8073905683720000, -14.20200298773971426 ) ) ;
#20348=CARTESIAN_POINT ( 'NONE',  ( -44.16309181155857999, 464.4948905683720000, 6.410867750099241924 ) ) ;
#20350=CARTESIAN_POINT ( 'NONE',  ( -40.01497788969915348, 465.6823905601785327, -16.95518130045146421 ) ) ;
#20351=CARTESIAN_POINT ( 'NONE',  ( -38.17536295476244135, 285.4323905683720568, 14.20200298773971781 ) ) ;
#20352=ORIENTED_EDGE ( 'NONE', *, *, #14073, .F. ) ;
#20355=CARTESIAN_POINT ( 'NONE',  ( -21.03221929538691981, 344.1198905601784759, -18.47759065022572855 ) ) ;
#20356=CARTESIAN_POINT ( 'NONE',  ( -35.09675569278794427, 295.7448905683720568, 15.47720386886985366 ) ) ;
#20358=CARTESIAN_POINT ( 'NONE',  ( -42.88789093042843348, 374.4323905683720000, -9.489475012073734561 ) ) ;
#20359=CARTESIAN_POINT ( 'NONE',  ( -28.68588794268869435, 229.7448905601785043, 19.99999999999999289 ) ) ;
#20360=CARTESIAN_POINT ( 'NONE',  ( -42.82802356641968089, 530.7448905765656946, -14.14213562373094746 ) ) ;
#20361=CARTESIAN_POINT ( 'NONE',  ( -13.20868407381886556, 399.4948905683720000, -6.410867750099233042 ) ) ;
#20362=CARTESIAN_POINT ( 'NONE',  ( -25.35362745456396638, 258.1823905683720000, 16.75240474999998952 ) ) ;
#20363=CARTESIAN_POINT ( 'NONE',  ( -11.93348319268872970, 428.8698905683720568, -2.051577885510841163E-15 ) ) ;
#20365=CARTESIAN_POINT ( 'NONE',  ( -32.66413529028187668, 339.8073905765656377, -19.99999999999999289 ) ) ;
#20367=CARTESIAN_POINT ( 'NONE',  ( -40.53162694259543031, 325.1198905683720568, 11.84573899990672885 ) ) ;
#20368=CARTESIAN_POINT ( 'NONE',  ( -28.68588794268872988, 472.8698905683720568, -16.75240474999999307 ) ) ;
#20369=CARTESIAN_POINT ( 'NONE',  ( -17.35679799567829917, 435.4323905765656377, 16.95518130045146421 ) ) ;
#20371=CYLINDRICAL_SURFACE ( 'NONE', #14737, 19.99999999999999645 ) ;
#20373=CARTESIAN_POINT ( 'NONE',  ( -14.48388495494899963, 379.4323905683721136, 9.489475012073732785 ) ) ;
#20376=( BOUNDED_CURVE ( )  B_SPLINE_CURVE ( 2, ( #17368, #10432, #15861, #3951, #7611, #20716, #3845, #20606, #7293, #20395, #17054, #8815, #13918, #2339, #15432, #2655, #5781 ),
 .UNSPECIFIED., .F., .T. ) 
 B_SPLINE_CURVE_WITH_KNOTS ( ( 3, 2, 2, 2, 2, 2, 2, 2, 3 ),
 ( 0.1406250000000001388, 0.1425781250000001388, 0.1445312500000001388, 0.1464843750000001388, 0.1484375000000001388, 0.1503906250000001388, 0.1523437500000001388, 0.1542968750000001388, 0.1562500000000001388 ),
 .UNSPECIFIED. ) 
 CURVE ( )  GEOMETRIC_REPRESENTATION_ITEM ( )  RATIONAL_B_SPLINE_CURVE ( ( 0.9999999999999986677, 0.9807852804032317628, 1.000000000000000000, 0.9807852804032304306, 1.000000000000000000, 0.9807852804032304306, 1.000000000000000000, 0.9807852804032304306, 1.000000000000000000, 0.9807852804032304306, 1.000000000000000000, 0.9807852804032304306, 1.000000000000000000, 0.9807852804032304306, 1.000000000000000000, 0.9807852804032290983, 1.000000000000001332 ) ) 
 REPRESENTATION_ITEM ( '' )  );
#20377=CARTESIAN_POINT ( 'NONE',  ( -36.33955658999053639, 519.1198905601785327, 18.47759065022572500 ) ) ;
#20378=CARTESIAN_POINT ( 'NONE',  ( -45.43829269268870519, 353.5573905683721136, -3.332260488124726194 ) ) ;
#20379=ORIENTED_EDGE ( 'NONE', *, *, #388, .T. ) ;
#20380=CARTESIAN_POINT ( 'NONE',  ( -19.19641293061499709, 497.3073905683720568, 14.20200298773971426 ) ) ;
#20382=CARTESIAN_POINT ( 'NONE',  ( -32.66413529028187668, 349.4323905601785327, 19.99999999999999289 ) ) ;
#20387=CARTESIAN_POINT ( 'NONE',  ( -28.68588794268872988, 461.3698905683720000, -16.75240474999999307 ) ) ;
#20389=CARTESIAN_POINT ( 'NONE',  ( -44.16309181155857999, 494.4948905683720568, 6.410867750099241924 ) ) ;
#20390=CARTESIAN_POINT ( 'NONE',  ( -8.685887942688708563, 246.9948905765656093, -2.449293598294705724E-15 ) ) ;
#20391=CARTESIAN_POINT ( 'NONE',  ( -47.16347859291445133, 432.6198905765656377, 7.653668647301805628 ) ) ;
#20392=CARTESIAN_POINT ( 'NONE',  ( -8.685887942688735208, 476.9948905765656377, -2.449293598294705724E-15 ) ) ;
#20393=FACE_OUTER_BOUND ( 'NONE', #6696, .T. ) ;
#20395=CARTESIAN_POINT ( 'NONE',  ( -32.66413529028188378, 484.1823905765656946, 19.99999999999999289 ) ) ;
#20396=EDGE_CURVE ( 'NONE', #19138, #9067, #18984, .T. ) ;
#20397=AXIS2_PLACEMENT_3D ( 'NONE', #10554, #5691, #15665 ) ;
#20399=CARTESIAN_POINT ( 'NONE',  ( -24.70764059509556532, 434.4323905601785327, -19.99999999999999289 ) ) ;
#20401=CARTESIAN_POINT ( 'NONE',  ( -14.48388495494898720, 279.4323905683720568, 9.489475012073732785 ) ) ;
#20402=CARTESIAN_POINT ( 'NONE',  ( -28.68588794268869790, 249.7448905601784475, 19.99999999999999289 ) ) ;
#20404=CARTESIAN_POINT ( 'NONE',  ( -45.43829269268872650, 455.3698905683720000, 0.000000000000000000 ) ) ;
#20405=CARTESIAN_POINT ( 'NONE',  ( -47.16347859291445133, 401.3698905765656377, -7.653668647301793193 ) ) ;
#20406=CARTESIAN_POINT ( 'NONE',  ( -44.16309181155855157, 265.9948905683720000, 6.410867750099241924 ) ) ;
#20410=CARTESIAN_POINT ( 'NONE',  ( -45.43829269268872650, 475.0573905683720000, -3.332260488124726638 ) ) ;
#20414=EDGE_LOOP ( 'NONE', ( #3039, #9466, #4097, #15321 ) ) ;
#20415=CARTESIAN_POINT ( 'NONE',  ( -48.68588794268871567, 401.9948905765656377, 0.000000000000000000 ) ) ;
#20416=CARTESIAN_POINT ( 'NONE',  ( -45.43829269268869808, 253.8698905683720000, 0.000000000000000000 ) ) ;
#20417=ORIENTED_EDGE ( 'NONE', *, *, #6166, .T. ) ;
#20418=FACE_OUTER_BOUND ( 'NONE', #10467, .T. ) ;
#20419=CARTESIAN_POINT ( 'NONE',  ( -48.68588794268872277, 481.6823905765656377, -3.978247347593158345 ) ) ;
#20421=CARTESIAN_POINT ( 'NONE',  ( -11.93348319268870661, 240.6823905683720284, -3.332260488124732856 ) ) ;
#20423=CARTESIAN_POINT ( 'NONE',  ( -42.82802356641965957, 365.9948905601784759, -14.14213562373094746 ) ) ;
#20424=CARTESIAN_POINT ( 'NONE',  ( -28.68588794268872988, 517.8698905683720568, 16.75240474999999307 ) ) ;
#20425=CARTESIAN_POINT ( 'NONE',  ( -47.16347859291444422, 372.6198905765655809, 7.653668647301805628 ) ) ;
#20426=CARTESIAN_POINT ( 'NONE',  ( -22.27502019258946220, 246.9948905683720284, 15.47720386886985189 ) ) ;
#20427=CARTESIAN_POINT ( 'NONE',  ( -40.53162694259543741, 334.1198905683720568, -11.84573899990672707 ) ) ;
#20428=CARTESIAN_POINT ( 'NONE',  ( -24.70764059509554755, 320.0573905601784759, 19.99999999999998934 ) ) ;
#20430=CARTESIAN_POINT ( 'NONE',  ( -35.09675569278795848, 405.7448905683720568, 15.47720386886985366 ) ) ;
#20432=CARTESIAN_POINT ( 'NONE',  ( -28.68588794268871922, 404.7448905601784759, -19.99999999999999289 ) ) ;
#20433=ORIENTED_EDGE ( 'NONE', *, *, #16475, .F. ) ;
#20434=DIRECTION ( 'NONE',  ( -1.000000000000000000, 0.000000000000000000, 0.000000000000000000 ) ) ;
#20436=ORIENTED_EDGE ( 'NONE', *, *, #1969, .F. ) ;
#20437=CARTESIAN_POINT ( 'NONE',  ( -42.88789093042844769, 504.4323905683721136, -9.489475012073736337 ) ) ;
#20438=CARTESIAN_POINT ( 'NONE',  ( -21.03221929538690205, 290.3698905601784759, 18.47759065022572500 ) ) ;
#20439=CARTESIAN_POINT ( 'NONE',  ( -43.04742826731176564, 207.6584868706943041, -4.333760535973599559 ) ) ;
#20441=CARTESIAN_POINT ( 'NONE',  ( -19.19641293061497933, 331.9323905683720000, -14.20200298773971603 ) ) ;
#20444=CARTESIAN_POINT ( 'NONE',  ( -45.43829269268870519, 353.5573905683721136, -3.332260488124726194 ) ) ;
#20445=CARTESIAN_POINT ( 'NONE',  ( -14.48388495494899786, 349.8073905683720000, -9.489475012073734561 ) ) ;
#20446=CARTESIAN_POINT ( 'NONE',  ( -8.685887942688713892, 286.6823905765656377, 3.978247347593161010 ) ) ;
#20447=CARTESIAN_POINT ( 'NONE',  ( -48.68588794268865882, 501.6823905765654672, -3.978247347593317773 ) ) ;
#20448=CARTESIAN_POINT ( 'NONE',  ( -35.09675569278793006, 251.9948905683720568, -15.47720386886985544 ) ) ;
#20451=CARTESIAN_POINT ( 'NONE',  ( -16.84014894278199748, 411.6198905683720568, -11.84573899990672707 ) ) ;
#20453=CARTESIAN_POINT ( 'NONE',  ( -45.64106924314017988, 356.3073905601785896, -11.32908994701042538 ) ) ;
#20455=CARTESIAN_POINT ( 'NONE',  ( -42.82802356641966668, 408.4948905601784759, 14.14213562373094923 ) ) ;
#20456=CARTESIAN_POINT ( 'NONE',  ( -11.93348319268871549, 320.3698905683720568, -2.051577885510841163E-15 ) ) ;
#20457=CARTESIAN_POINT ( 'NONE',  ( -42.88789093042844769, 454.8073905683720000, 9.489475012073736337 ) ) ;
#20458=ORIENTED_EDGE ( 'NONE', *, *, #21380, .F. ) ;
#20460=CARTESIAN_POINT ( 'NONE',  ( -45.64106924314020119, 476.3073905601785327, -11.32908994701042715 ) ) ;
#20461=CARTESIAN_POINT ( 'NONE',  ( -14.48388495494899075, 279.8073905683720000, -9.489475012073736337 ) ) ;
#20462=EDGE_CURVE ( 'NONE', #683, #16932, #3215, .T. ) ;
#20465=CARTESIAN_POINT ( 'NONE',  ( -22.27502019258949773, 452.2448905683720000, -15.47720386886985544 ) ) ;
#20469=CARTESIAN_POINT ( 'NONE',  ( -25.35362745456397349, 306.6823905683720000, 16.75240474999998952 ) ) ;
#20470=EDGE_CURVE ( 'NONE', #2640, #8642, #14583, .T. ) ;
#20471=CARTESIAN_POINT ( 'NONE',  ( -19.19641293061498288, 378.8073905683721136, 14.20200298773971426 ) ) ;
#20472=CARTESIAN_POINT ( 'NONE',  ( -8.685887942688795604, 231.9323905601784759, 3.978247347593374172 ) ) ;
#20473=CARTESIAN_POINT ( 'NONE',  ( -21.03221929538692692, 515.1198905765656946, 18.47759065022572500 ) ) ;
#20474=CARTESIAN_POINT ( 'NONE',  ( -11.93348319268872615, 399.1823905683720568, -3.332260488124732856 ) ) ;
#20475=CARTESIAN_POINT ( 'NONE',  ( -22.27502019258946220, 248.4948905683720284, 15.47720386886985189 ) ) ;
#20476=CARTESIAN_POINT ( 'NONE',  ( -11.93348319268872970, 428.5573905683720568, 3.332260488124728859 ) ) ;
#20477=CARTESIAN_POINT ( 'NONE',  ( -14.54375231895776466, 335.7448905765655809, 14.14213562373094568 ) ) ;
#20479=CARTESIAN_POINT ( 'NONE',  ( -19.19641293061497223, 307.3073905683720000, 14.20200298773971426 ) ) ;
#20480=CARTESIAN_POINT ( 'NONE',  ( -40.53162694259545162, 476.6198905683720000, 11.84573899990672885 ) ) ;
#20485=CARTESIAN_POINT ( 'NONE',  ( -25.35362745456399480, 382.5573905683720568, -16.75240474999999307 ) ) ;
#20488=CARTESIAN_POINT ( 'NONE',  ( -32.66413529028189799, 525.0573905601784190, -19.99999999999999289 ) ) ;
#20489=CARTESIAN_POINT ( 'NONE',  ( -22.27502019258948351, 340.7448905683720568, -15.47720386886985544 ) ) ;
#20491=CARTESIAN_POINT ( 'NONE',  ( -42.88789093042845479, 504.8073905683720568, 9.489475012073736337 ) ) ;
#20493=CARTESIAN_POINT ( 'NONE',  ( -32.66413529028187668, 355.0573905601785327, -19.99999999999999289 ) ) ;
#20494=CARTESIAN_POINT ( 'NONE',  ( -11.73070664223724968, 377.9323905765656946, -11.32908994701042538 ) ) ;
#20497=DIRECTION ( 'NONE',  ( -1.191790137725560488E-16, 1.000000000000000000, -0.000000000000000000 ) ) ;
#20498=CARTESIAN_POINT ( 'NONE',  ( -16.84014894278200103, 467.6198905683720000, 11.84573899990672530 ) ) ;
#20500=CARTESIAN_POINT ( 'NONE',  ( -11.93348319268873503, 478.8698905683720568, -2.051577885510841163E-15 ) ) ;
#20501=CARTESIAN_POINT ( 'NONE',  ( -36.33955658999050087, 243.8698905765656093, 18.47759065022572500 ) ) ;
#20503=CARTESIAN_POINT ( 'NONE',  ( -28.68588794268871922, 399.4948905765656377, -19.99999999999999289 ) ) ;
#20505=CARTESIAN_POINT ( 'NONE',  ( -47.16347859291443712, 297.8698905601784759, 7.653668647301805628 ) ) ;
#20506=CARTESIAN_POINT ( 'NONE',  ( -11.73070664223726389, 483.1823905601784190, -11.32908994701042538 ) ) ;
#20509=CARTESIAN_POINT ( 'NONE',  ( -28.68588794268874054, 573.2448905601785327, 0.000000000000000000 ) ) ;
#20511=( BOUNDED_CURVE ( )  B_SPLINE_CURVE ( 2, ( #17797, #2987, #16080, #16402, #6422, #13038, #1688, #21046, #8150, #19628, #19312, #1579, #12830, #6112, #4807, #14678, #8259 ),
 .UNSPECIFIED., .F., .T. ) 
 B_SPLINE_CURVE_WITH_KNOTS ( ( 3, 2, 2, 2, 2, 2, 2, 2, 3 ),
 ( 0.3281250000000001110, 0.3300781250000001110, 0.3320312500000001110, 0.3339843750000001110, 0.3359375000000001110, 0.3378906250000001110, 0.3398437500000001110, 0.3417968750000001110, 0.3437500000000001110 ),
 .UNSPECIFIED. ) 
 CURVE ( )  GEOMETRIC_REPRESENTATION_ITEM ( )  RATIONAL_B_SPLINE_CURVE ( ( 0.9999999999999988898, 0.9807852804032315408, 1.000000000000000000, 0.9807852804032304306, 1.000000000000000000, 0.9807852804032304306, 1.000000000000000000, 0.9807852804032304306, 1.000000000000000000, 0.9807852804032304306, 1.000000000000000000, 0.9807852804032304306, 1.000000000000000000, 0.9807852804032304306, 1.000000000000000000, 0.9807852804032293204, 1.000000000000001110 ) ) 
 REPRESENTATION_ITEM ( '' )  );
#20512=CARTESIAN_POINT ( 'NONE',  ( -42.88789093042842637, 276.3073905683720568, 9.489475012073736337 ) ) ;
#20513=CARTESIAN_POINT ( 'NONE',  ( -42.82802356641964536, 255.9948905601784759, -14.14213562373094746 ) ) ;
#20515=CARTESIAN_POINT ( 'NONE',  ( -35.09675569278795138, 443.4948905683720568, -15.47720386886985544 ) ) ;
#20517=CARTESIAN_POINT ( 'NONE',  ( -13.20868407381884779, 260.9948905683720568, -6.410867750099233042 ) ) ;
#20520=CARTESIAN_POINT ( 'NONE',  ( -28.68588794268874054, 573.2448905601785327, 0.000000000000000000 ) ) ;
#20522=CARTESIAN_POINT ( 'NONE',  ( -35.09675569278795848, 483.4948905683720000, -15.47720386886985544 ) ) ;
#20527=CARTESIAN_POINT ( 'NONE',  ( -44.16309181155855867, 233.2448905683720000, -6.410867750099231266 ) ) ;
#20528=VERTEX_POINT ( 'NONE', #11749 ) ;
#20530=CARTESIAN_POINT ( 'NONE',  ( -28.68588794268872988, 459.4948905765656377, -19.99999999999999289 ) ) ;
#20532=CARTESIAN_POINT ( 'NONE',  ( -25.35362745456397704, 232.5573905683720568, -16.75240474999999307 ) ) ;
#20533=CARTESIAN_POINT ( 'NONE',  ( -38.17536295476247687, 513.8073905683720568, -14.20200298773971426 ) ) ;
#20535=CARTESIAN_POINT ( 'NONE',  ( -35.09675569278793716, 245.7448905683720000, 15.47720386886985366 ) ) ;
#20537=CARTESIAN_POINT ( 'NONE',  ( -42.88789093042843348, 344.4323905683720000, -9.489475012073736337 ) ) ;
#20540=CARTESIAN_POINT ( 'NONE',  ( -48.68588794268870146, 301.9948905765655809, 0.000000000000000000 ) ) ;
#20541=CARTESIAN_POINT ( 'NONE',  ( -42.88789093042843348, 384.8073905683720000, 9.489475012073736337 ) ) ;
#20542=CARTESIAN_POINT ( 'NONE',  ( -24.70764059509555466, 380.0573905601785327, 19.99999999999998934 ) ) ;
#20545=CARTESIAN_POINT ( 'NONE',  ( -10.20829729246298356, 347.6198905765656377, -7.653668647301794969 ) ) ;
#20548=CARTESIAN_POINT ( 'NONE',  ( -40.53162694259545873, 516.6198905683720568, 11.84573899990672885 ) ) ;
#20549=CARTESIAN_POINT ( 'NONE',  ( -47.16347859291443712, 292.6198905765656377, 7.653668647301805628 ) ) ;
#20551=CARTESIAN_POINT ( 'NONE',  ( -16.84014894278198327, 301.6198905683720000, -11.84573899990672707 ) ) ;
#20552=ORIENTED_EDGE ( 'NONE', *, *, #19396, .F. ) ;
#20553=CARTESIAN_POINT ( 'NONE',  ( -38.17536295476245556, 352.3073905683720000, -14.20200298773971426 ) ) ;
#20554=CARTESIAN_POINT ( 'NONE',  ( -16.84014894278198682, 347.6198905683720000, 11.84573899990672530 ) ) ;
#20555=CARTESIAN_POINT ( 'NONE',  ( -8.685887942688713892, 286.9948905765656377, -2.449293598294705724E-15 ) ) ;
#20557=CARTESIAN_POINT ( 'NONE',  ( -14.48388495494898542, 249.8073905683720284, -9.489475012073734561 ) ) ;
#20558=CARTESIAN_POINT ( 'NONE',  ( -43.64324723180578047, 200.2731091681331179, 1.141620385913097779 ) ) ;
#20559=CARTESIAN_POINT ( 'NONE',  ( -25.35362745456399480, 392.5573905683720000, -16.75240474999999307 ) ) ;
#20561=CARTESIAN_POINT ( 'NONE',  ( -32.66413529028189089, 509.8073905765655240, -19.99999999999999289 ) ) ;
#20563=CARTESIAN_POINT ( 'NONE',  ( -25.35362745456400191, 461.0573905683721136, -16.75240474999999307 ) ) ;
#20564=EDGE_LOOP ( 'NONE', ( #8513, #4365, #6111, #15525 ) ) ;
#20565=CARTESIAN_POINT ( 'NONE',  ( -36.33955658999052218, 449.1198905601784759, 18.47759065022572500 ) ) ;
#20566=CARTESIAN_POINT ( 'NONE',  ( -11.93348319268871194, 278.5573905683720000, 3.332260488124728415 ) ) ;
#20571=CARTESIAN_POINT ( 'NONE',  ( -42.82802356641965957, 348.4948905601785327, 14.14213562373094923 ) ) ;
#20572=CARTESIAN_POINT ( 'NONE',  ( -11.93348319268871371, 298.8698905683720000, -2.051577885510841163E-15 ) ) ;
#20573=CARTESIAN_POINT ( 'NONE',  ( -19.19641293061498288, 371.9323905683720568, -14.20200298773971603 ) ) ;
#20575=CARTESIAN_POINT ( 'NONE',  ( -36.33955658999053639, 513.8698905765655809, 18.47759065022572500 ) ) ;
#20576=CARTESIAN_POINT ( 'NONE',  ( -25.35362745456398770, 406.6823905683720000, 16.75240474999998952 ) ) ;
#20577=CARTESIAN_POINT ( 'NONE',  ( -14.48388495494898365, 249.4323905683720000, 9.489475012073732785 ) ) ;
#20578=CARTESIAN_POINT ( 'NONE',  ( -19.19641293061498999, 410.4323905683720568, -14.20200298773971603 ) ) ;
#20579=CARTESIAN_POINT ( 'NONE',  ( -42.82802356641965957, 353.2448905765656377, 14.14213562373094923 ) ) ;
#20581=CARTESIAN_POINT ( 'NONE',  ( -22.27502019258947996, 310.7448905683720000, -15.47720386886985544 ) ) ;
#20582=CARTESIAN_POINT ( 'NONE',  ( -32.01814843081346140, 457.5573905683720000, 16.75240474999999307 ) ) ;
#20583=CARTESIAN_POINT ( 'NONE',  ( -17.35679799567830628, 515.4323905765656946, 16.95518130045146421 ) ) ;
#20587=CARTESIAN_POINT ( 'NONE',  ( -35.09675569278794427, 363.4948905683720568, -15.47720386886985544 ) ) ;
#20589=CARTESIAN_POINT ( 'NONE',  ( -10.20829729246300666, 531.6198905601785327, 7.653668647301790529 ) ) ;
#20590=CARTESIAN_POINT ( 'NONE',  ( -32.01814843081344719, 341.6823905683720000, -16.75240474999999307 ) ) ;
#20592=CARTESIAN_POINT ( 'NONE',  ( -32.01814843081346140, 501.6823905683720568, -16.75240474999999307 ) ) ;
#20594=CARTESIAN_POINT ( 'NONE',  ( -14.54375231895777176, 378.2448905765656377, -14.14213562373094746 ) ) ;
#20598=CARTESIAN_POINT ( 'NONE',  ( -25.35362745456400546, 471.0573905683720568, -16.75240474999999307 ) ) ;
#20600=CARTESIAN_POINT ( 'NONE',  ( -44.16309181155858710, 473.2448905683720568, -6.410867750099231266 ) ) ;
#20601=LINE ( 'NONE', #4270, #18969 ) ;
#20602=CARTESIAN_POINT ( 'NONE',  ( -36.33955658999052218, 403.8698905765656377, 18.47759065022572500 ) ) ;
#20603=CARTESIAN_POINT ( 'NONE',  ( -42.82802356641965247, 280.7448905765655809, -14.14213562373094746 ) ) ;
#20604=CARTESIAN_POINT ( 'NONE',  ( -10.20829729246297823, 301.6198905601784759, 7.653668647301790529 ) ) ;
#20606=CARTESIAN_POINT ( 'NONE',  ( -24.70764059509556176, 484.8073905765656946, 19.99999999999998934 ) ) ;
#20611=CARTESIAN_POINT ( 'NONE',  ( -35.09675569278794427, 277.2448905683720568, 15.47720386886985366 ) ) ;
#20612=CARTESIAN_POINT ( 'NONE',  ( -48.68588794268869435, 247.5573905601785043, 3.978247347593168115 ) ) ;
#20614=CARTESIAN_POINT ( 'NONE',  ( -8.685887942688726326, 406.9948905765656377, -2.449293598294705724E-15 ) ) ;
#20615=CARTESIAN_POINT ( 'NONE',  ( -42.88789093042844058, 436.3073905683720568, 9.489475012073736337 ) ) ;
#20617=CARTESIAN_POINT ( 'NONE',  ( -13.20868407381884779, 269.7448905683720568, 6.410867750099229490 ) ) ;
#20621=CARTESIAN_POINT ( 'NONE',  ( -45.43829269268872650, 475.3698905683720568, 0.000000000000000000 ) ) ;
#20622=VECTOR ( 'NONE', #11862, 1000.000000000000000 ) ;
#20624=CARTESIAN_POINT ( 'NONE',  ( -11.73070664223726745, 526.0573905765656946, 11.32908994701042005 ) ) ;
#20625=CARTESIAN_POINT ( 'NONE',  ( -13.20868407381884602, 248.2448905683720000, 6.410867750099229490 ) ) ;
#20626=ORIENTED_EDGE ( 'NONE', *, *, #9004, .F. ) ;
#20629=CARTESIAN_POINT ( 'NONE',  ( -48.68588794268872277, 472.3073905765656377, 3.978247347593168115 ) ) ;
#20633=CARTESIAN_POINT ( 'NONE',  ( -40.53162694259542320, 224.1198905683720000, -11.84573899990672707 ) ) ;
#20634=( BOUNDED_CURVE ( )  B_SPLINE_CURVE ( 2, ( #15356, #13943, #7205, #20208, #7421, #18677, #10347, #537, #13724, #10559, #2361, #10455, #15455, #2257, #4079, #17075, #8941 ),
 .UNSPECIFIED., .F., .T. ) 
 B_SPLINE_CURVE_WITH_KNOTS ( ( 3, 2, 2, 2, 2, 2, 2, 2, 3 ),
 ( 0.4531250000000002220, 0.4550781250000002220, 0.4570312500000002220, 0.4589843750000002220, 0.4609375000000002220, 0.4628906250000002220, 0.4648437500000002220, 0.4667968750000002220, 0.4687500000000002220 ),
 .UNSPECIFIED. ) 
 CURVE ( )  GEOMETRIC_REPRESENTATION_ITEM ( )  RATIONAL_B_SPLINE_CURVE ( ( 0.9999999999999977796, 0.9807852804032326510, 1.000000000000000000, 0.9807852804032304306, 1.000000000000000000, 0.9807852804032304306, 1.000000000000000000, 0.9807852804032304306, 1.000000000000000000, 0.9807852804032304306, 1.000000000000000000, 0.9807852804032304306, 1.000000000000000000, 0.9807852804032304306, 1.000000000000000000, 0.9807852804032282101, 1.000000000000002220 ) ) 
 REPRESENTATION_ITEM ( '' )  );
#20635=CARTESIAN_POINT ( 'NONE',  ( -35.09675569278796559, 523.4948905683720568, -15.47720386886985544 ) ) ;
#20637=CARTESIAN_POINT ( 'NONE',  ( -11.93348319268870839, 239.1823905683720284, -3.332260488124732856 ) ) ;
#20638=CARTESIAN_POINT ( 'NONE',  ( -22.27502019258947286, 328.4948905683720568, 15.47720386886985189 ) ) ;
#20641=CARTESIAN_POINT ( 'NONE',  ( -42.82802356641965247, 303.2448905765656377, 14.14213562373094923 ) ) ;
#20643=CARTESIAN_POINT ( 'NONE',  ( -11.93348319268872437, 388.8698905683720000, -2.051577885510841163E-15 ) ) ;
#20645=CARTESIAN_POINT ( 'NONE',  ( -40.01497788969912506, 323.5573905765655809, 16.95518130045146776 ) ) ;
#20646=CARTESIAN_POINT ( 'NONE',  ( -8.685887942688722774, 381.9323905601784759, 3.978247347593161010 ) ) ;
#20648=CARTESIAN_POINT ( 'NONE',  ( -48.68588794268871567, 407.2448905601784759, 0.000000000000000000 ) ) ;
#20651=CARTESIAN_POINT ( 'NONE',  ( -44.16309181155858710, 504.7448905683720000, -6.410867750099231266 ) ) ;
#20654=CARTESIAN_POINT ( 'NONE',  ( -25.35362745456397349, 298.1823905683720000, 16.75240474999998952 ) ) ;
#20656=CARTESIAN_POINT ( 'NONE',  ( -25.35362745456398770, 341.0573905683720000, -16.75240474999999307 ) ) ;
#20657=CARTESIAN_POINT ( 'NONE',  ( -32.01814843081344719, 341.6823905683720000, -16.75240474999999307 ) ) ;
#20658=CARTESIAN_POINT ( 'NONE',  ( -36.33955658999050087, 280.1198905765656377, -18.47759065022572855 ) ) ;
#20659=CARTESIAN_POINT ( 'NONE',  ( -36.33955658999051508, 395.3698905601785327, -18.47759065022572855 ) ) ;
#20660=CARTESIAN_POINT ( 'NONE',  ( -28.68588794268869790, 246.3698905683720000, 16.75240474999999307 ) ) ;
#20662=CARTESIAN_POINT ( 'NONE',  ( -19.19641293061498999, 391.9323905683720000, -14.20200298773971603 ) ) ;
#20666=CARTESIAN_POINT ( 'NONE',  ( -17.35679799567828141, 243.8073905601784759, -16.95518130045146421 ) ) ;
#20667=CARTESIAN_POINT ( 'NONE',  ( -42.88789093042844058, 442.9323905683721136, -9.489475012073736337 ) ) ;
#20668=EDGE_LOOP ( 'NONE', ( #3836, #3565, #17280, #14286 ) ) ;
#20669=CARTESIAN_POINT ( 'NONE',  ( -32.66413529028188378, 439.4323905601785327, 19.99999999999999289 ) ) ;
#20675=CARTESIAN_POINT ( 'NONE',  ( -48.68588794268870146, 316.9323905601784759, -3.978247347593158345 ) ) ;
#20676=CARTESIAN_POINT ( 'NONE',  ( -11.93348319268871549, 298.5573905683720000, 3.332260488124728415 ) ) ;
#20678=CARTESIAN_POINT ( 'NONE',  ( -44.16309181155857289, 364.7448905683720568, -6.410867750099231266 ) ) ;
#20680=CARTESIAN_POINT ( 'NONE',  ( -36.33955658999052929, 530.1198905765655809, -18.47759065022572855 ) ) ;
#20681=CARTESIAN_POINT ( 'NONE',  ( -45.43829269268871229, 404.1823905683720568, 3.332260488124734632 ) ) ;
#20682=CARTESIAN_POINT ( 'NONE',  ( -25.35362745456396638, 238.1823905683720852, 16.75240474999998952 ) ) ;
#20683=CARTESIAN_POINT ( 'NONE',  ( -45.43829269268871940, 403.8698905683720000, 0.000000000000000000 ) ) ;
#20686=CARTESIAN_POINT ( 'NONE',  ( -10.20829729246298356, 347.6198905765656377, -7.653668647301794969 ) ) ;
#20687=CARTESIAN_POINT ( 'NONE',  ( -11.73070664223724613, 323.1823905601784190, -11.32908994701042538 ) ) ;
#20688=CARTESIAN_POINT ( 'NONE',  ( -38.17536295476244135, 315.4323905683720000, 14.20200298773971781 ) ) ;
#20690=CARTESIAN_POINT ( 'NONE',  ( -25.35362745456400191, 462.5573905683720000, -16.75240474999999307 ) ) ;
#20692=CARTESIAN_POINT ( 'NONE',  ( -17.35679799567829917, 460.6823905601785327, 16.95518130045146421 ) ) ;
#20695=CARTESIAN_POINT ( 'NONE',  ( -22.27502019258948707, 372.2448905683720000, -15.47720386886985544 ) ) ;
#20696=CARTESIAN_POINT ( 'NONE',  ( -40.53162694259545162, 502.6198905683720568, -11.84573899990672707 ) ) ;
#20697=CARTESIAN_POINT ( 'NONE',  ( -28.68588794268872988, 499.7448905601785327, 19.99999999999999289 ) ) ;
#20698=CARTESIAN_POINT ( 'NONE',  ( -40.53162694259543741, 342.6198905683720000, -11.84573899990672707 ) ) ;
#20701=CARTESIAN_POINT ( 'NONE',  ( -32.01814843081346140, 496.0573905683720568, 16.75240474999999307 ) ) ;
#20703=LINE ( 'NONE', #12489, #18773 ) ;
#20704=CARTESIAN_POINT ( 'NONE',  ( -45.43829269268871940, 425.6823905683720568, 3.332260488124734632 ) ) ;
#20705=CARTESIAN_POINT ( 'NONE',  ( -48.68588794268870856, 331.9948905765656377, 0.000000000000000000 ) ) ;
#20708=CARTESIAN_POINT ( 'NONE',  ( -11.93348319268873325, 458.8698905683720000, -2.051577885510841163E-15 ) ) ;
#20710=CARTESIAN_POINT ( 'NONE',  ( -25.35362745456399480, 466.6823905683720000, 16.75240474999998952 ) ) ;
#20711=CARTESIAN_POINT ( 'NONE',  ( -42.82802356641964536, 248.4948905601784759, 14.14213562373094923 ) ) ;
#20712=CARTESIAN_POINT ( 'NONE',  ( -8.685887942688726326, 396.6823905765656946, 3.978247347593161010 ) ) ;
#20713=CARTESIAN_POINT ( 'NONE',  ( -47.16347859291443712, 281.3698905765656377, -7.653668647301793193 ) ) ;
#20714=CARTESIAN_POINT ( 'NONE',  ( -8.685887942688724550, 366.9948905765655809, -2.449293598294705724E-15 ) ) ;
#20715=CARTESIAN_POINT ( 'NONE',  ( -8.685887942688742314, 573.2448905601785327, 2.449293598294706119E-15 ) ) ;
#20716=CARTESIAN_POINT ( 'NONE',  ( -17.35679799567830273, 485.4323905765656946, 16.95518130045146421 ) ) ;
#20719=CARTESIAN_POINT ( 'NONE',  ( -10.20829729246299244, 421.6198905601785327, 7.653668647301790529 ) ) ;
#20721=CARTESIAN_POINT ( 'NONE',  ( -13.20868407381884779, 279.7448905683720568, 6.410867750099229490 ) ) ;
#20723=CARTESIAN_POINT ( 'NONE',  ( -48.68588794268869435, 257.2448905601784759, 0.000000000000000000 ) ) ;
#20725=CARTESIAN_POINT ( 'NONE',  ( -35.09675569278795138, 423.4948905683720568, -15.47720386886985544 ) ) ;
#20726=DIRECTION ( 'NONE',  ( -1.191790137725560488E-16, 1.000000000000000000, -0.000000000000000000 ) ) ;
#20727=CARTESIAN_POINT ( 'NONE',  ( -44.16309181155855867, 244.7448905683720000, -6.410867750099231266 ) ) ;
#20730=LINE ( 'NONE', #14363, #8754 ) ;
#20731=ORIENTED_EDGE ( 'NONE', *, *, #1759, .F. ) ;
#20732=CARTESIAN_POINT ( 'NONE',  ( -11.93348319268873503, 480.6823905683720568, -3.332260488124732856 ) ) ;
#20734=VERTEX_POINT ( 'NONE', #3531 ) ;
#20735=CARTESIAN_POINT ( 'NONE',  ( -42.82802356641965957, 365.9948905601784759, -14.14213562373094746 ) ) ;
#20736=CARTESIAN_POINT ( 'NONE',  ( -35.09675569278793716, 235.7448905683720000, 15.47720386886985366 ) ) ;
#20737=ORIENTED_EDGE ( 'NONE', *, *, #16367, .T. ) ;
#20738=CARTESIAN_POINT ( 'NONE',  ( -22.27502019258950483, 520.7448905683720568, -15.47720386886985544 ) ) ;
#20739=DIRECTION ( 'NONE',  ( -1.191790137725560488E-16, 1.000000000000000000, -0.000000000000000000 ) ) ;
#20741=CARTESIAN_POINT ( 'NONE',  ( -45.64106924314020119, 461.0573905765656377, -11.32908994701042715 ) ) ;
#20745=CARTESIAN_POINT ( 'NONE',  ( -32.01814843081346851, 517.5573905683720568, 16.75240474999999307 ) ) ;
#20747=CARTESIAN_POINT ( 'NONE',  ( -42.88789093042841927, 254.8073905683720284, 9.489475012073736337 ) ) ;
#20748=CARTESIAN_POINT ( 'NONE',  ( -35.09675569278794427, 333.4948905683720568, -15.47720386886985544 ) ) ;
#20750=CARTESIAN_POINT ( 'NONE',  ( -48.68588794268887909, 467.5573905601785327, 3.978247347592795524 ) ) ;
#20751=VECTOR ( 'NONE', #382, 1000.000000000000000 ) ;
#20752=CARTESIAN_POINT ( 'NONE',  ( -8.685887942688717445, 306.9948905765655809, -2.449293598294705724E-15 ) ) ;
#20754=CARTESIAN_POINT ( 'NONE',  ( -22.27502019258949062, 390.7448905683720000, -15.47720386886985544 ) ) ;
#20756=FACE_OUTER_BOUND ( 'NONE', #7937, .T. ) ;
#20758=CARTESIAN_POINT ( 'NONE',  ( -48.68588794268870856, 387.2448905601784759, 0.000000000000000000 ) ) ;
#20759=ORIENTED_EDGE ( 'NONE', *, *, #7140, .T. ) ;
#20761=EDGE_LOOP ( 'NONE', ( #17306, #16238, #9192, #14897 ) ) ;
#20763=CARTESIAN_POINT ( 'NONE',  ( -32.01814843081346140, 497.5573905683720568, 16.75240474999999307 ) ) ;
#20764=CARTESIAN_POINT ( 'NONE',  ( -10.20829729246297823, 296.3698905765655809, 7.653668647301790529 ) ) ;
#20766=( BOUNDED_CURVE ( )  B_SPLINE_CURVE ( 2, ( #16696, #5314, #11915, #1885, #2085, #5418, #13986, #12131, #10496, #10819, #3798, #4008, #17117, #681, #5846, #10602, #18933 ),
 .UNSPECIFIED., .F., .T. ) 
 B_SPLINE_CURVE_WITH_KNOTS ( ( 3, 2, 2, 2, 2, 2, 2, 2, 3 ),
 ( 0.6093750000000002220, 0.6113281250000002220, 0.6132812500000002220, 0.6152343750000002220, 0.6171875000000002220, 0.6191406250000002220, 0.6210937500000002220, 0.6230468750000002220, 0.6250000000000002220 ),
 .UNSPECIFIED. ) 
 CURVE ( )  GEOMETRIC_REPRESENTATION_ITEM ( )  RATIONAL_B_SPLINE_CURVE ( ( 0.9999999999999977796, 0.9807852804032326510, 1.000000000000000000, 0.9807852804032304306, 1.000000000000000000, 0.9807852804032304306, 1.000000000000000000, 0.9807852804032304306, 1.000000000000000000, 0.9807852804032304306, 1.000000000000000000, 0.9807852804032304306, 1.000000000000000000, 0.9807852804032304306, 1.000000000000000000, 0.9807852804032282101, 1.000000000000002220 ) ) 
 REPRESENTATION_ITEM ( '' )  );
#20767=CARTESIAN_POINT ( 'NONE',  ( -28.68588794268870501, 307.8698905683720000, 16.75240474999999307 ) ) ;
#20768=CARTESIAN_POINT ( 'NONE',  ( -16.84014894278200813, 501.6198905683720000, -11.84573899990672707 ) ) ;
#20770=CARTESIAN_POINT ( 'NONE',  ( -45.43829269268870519, 334.1823905683720000, 3.332260488124734632 ) ) ;
#20771=CARTESIAN_POINT ( 'NONE',  ( -45.43829269268871229, 343.8698905683720000, 0.000000000000000000 ) ) ;
#20772=CARTESIAN_POINT ( 'NONE',  ( -11.73070664223723547, 276.0573905765656377, 11.32908994701042005 ) ) ;
#20774=DIRECTION ( 'NONE',  ( -1.191790137725560488E-16, 1.000000000000000000, -0.000000000000000000 ) ) ;
#20776=CARTESIAN_POINT ( 'NONE',  ( -19.19641293061496512, 237.3073905683720284, 14.20200298773971426 ) ) ;
#20778=CARTESIAN_POINT ( 'NONE',  ( -44.16309181155857289, 395.9948905683720568, 6.410867750099241924 ) ) ;
#20781=CARTESIAN_POINT ( 'NONE',  ( -45.64106924314016567, 246.3073905601784759, -11.32908994701042538 ) ) ;
#20782=CARTESIAN_POINT ( 'NONE',  ( -44.16309181155857999, 443.2448905683720000, -6.410867750099231266 ) ) ;
#20784=CARTESIAN_POINT ( 'NONE',  ( -17.35679799567830983, 453.8073905601784759, -16.95518130045146421 ) ) ;
#20790=CARTESIAN_POINT ( 'NONE',  ( -24.70764059509554755, 330.0573905601785327, 19.99999999999998934 ) ) ;
#20791=ADVANCED_FACE ( 'NONE', ( #11855 ), #20292, .T. ) ;
#20792=CARTESIAN_POINT ( 'NONE',  ( -32.01814843081344719, 363.1823905683720568, -16.75240474999999307 ) ) ;
#20793=CARTESIAN_POINT ( 'NONE',  ( -47.16347859291443001, 227.8698905601784759, 7.653668647301805628 ) ) ;
#20794=CARTESIAN_POINT ( 'NONE',  ( -14.54375231895778597, 515.7448905765655809, 14.14213562373094568 ) ) ;
#20795=CARTESIAN_POINT ( 'NONE',  ( -28.68588794268871567, 396.3698905683720000, 16.75240474999999307 ) ) ;
#20796=CARTESIAN_POINT ( 'NONE',  ( -11.93348319268870661, 240.3698905683720568, -2.051577885510841163E-15 ) ) ;
#20797=CARTESIAN_POINT ( 'NONE',  ( -13.20868407381886556, 399.4948905683720000, -6.410867750099233042 ) ) ;
#20798=CARTESIAN_POINT ( 'NONE',  ( -24.70764059509555111, 344.8073905765656377, 19.99999999999998934 ) ) ;
#20799=CARTESIAN_POINT ( 'NONE',  ( -40.01497788969913216, 325.6823905601784759, -16.95518130045146421 ) ) ;
#20800=CARTESIAN_POINT ( 'NONE',  ( -35.09675569278793716, 311.9948905683720568, -15.47720386886985544 ) ) ;
#20801=CARTESIAN_POINT ( 'NONE',  ( -28.68588794268872988, 462.8698905683720000, -16.75240474999999307 ) ) ;
#20807=CARTESIAN_POINT ( 'NONE',  ( -16.84014894278199037, 361.6198905683720000, -11.84573899990672707 ) ) ;
#20808=CARTESIAN_POINT ( 'NONE',  ( -35.09675569278795848, 501.9948905683720000, -15.47720386886985544 ) ) ;
#20809=CARTESIAN_POINT ( 'NONE',  ( -40.01497788969914637, 498.8073905601784759, 16.95518130045146776 ) ) ;
#20810=CARTESIAN_POINT ( 'NONE',  ( -16.84014894278198682, 330.1198905683720568, -11.84573899990672707 ) ) ;
#20812=CARTESIAN_POINT ( 'NONE',  ( -22.27502019258950128, 500.7448905683720000, -15.47720386886985544 ) ) ;
#20814=AXIS2_PLACEMENT_3D ( 'NONE', #10119, #16741, #15120 ) ;
#20815=CARTESIAN_POINT ( 'NONE',  ( -8.685887942688893304, 316.6823905765655809, 3.978247347593586447 ) ) ;
#20817=CARTESIAN_POINT ( 'NONE',  ( -11.93348319268872793, 420.3698905683720568, -2.051577885510841163E-15 ) ) ;
#20818=CARTESIAN_POINT ( 'NONE',  ( -11.73070664223724968, 396.0573905765655809, 11.32908994701042005 ) ) ;
#20820=CARTESIAN_POINT ( 'NONE',  ( -13.20868407381887266, 459.4948905683720568, -6.410867750099233042 ) ) ;
#20823=CARTESIAN_POINT ( 'NONE',  ( -22.27502019258948707, 456.9948905683720000, 15.47720386886985189 ) ) ;
#20824=CARTESIAN_POINT ( 'NONE',  ( -8.685887942688708563, 242.2448905601785043, -2.449293598294705724E-15 ) ) ;
#20825=CARTESIAN_POINT ( 'NONE',  ( -10.20829729246299067, 407.6198905765656377, -7.653668647301794969 ) ) ;
#20831=CARTESIAN_POINT ( 'NONE',  ( -17.35679799567829207, 343.8073905601785327, -16.95518130045146421 ) ) ;
#20833=CARTESIAN_POINT ( 'NONE',  ( -8.685887942688708563, 242.5573905601784759, -3.978247347593165895 ) ) ;
#20835=CARTESIAN_POINT ( 'NONE',  ( -42.88789093042844058, 426.3073905683720568, 9.489475012073736337 ) ) ;
#20837=CARTESIAN_POINT ( 'NONE',  ( -45.43829269268869808, 255.3698905683720000, 0.000000000000000000 ) ) ;
#20839=ORIENTED_EDGE ( 'NONE', *, *, #19162, .F. ) ;
#20840=DIRECTION ( 'NONE',  ( -1.191790137725560488E-16, 1.000000000000000000, 0.000000000000000000 ) ) ;
#20841=EDGE_LOOP ( 'NONE', ( #17693, #19632, #12911 ) ) ;
#20842=CARTESIAN_POINT ( 'NONE',  ( -14.48388495494901029, 469.4323905683720568, 9.489475012073731008 ) ) ;
#20844=EDGE_LOOP ( 'NONE', ( #18510, #10205 ) ) ;
#20846=CARTESIAN_POINT ( 'NONE',  ( -38.17536295476243424, 245.4323905683720000, 14.20200298773971781 ) ) ;
#20849=CARTESIAN_POINT ( 'NONE',  ( -25.35362745456399836, 516.6823905683720568, 16.75240474999998952 ) ) ;
#20851=CARTESIAN_POINT ( 'NONE',  ( -14.54375231895777887, 455.7448905765656377, 14.14213562373094568 ) ) ;
#20854=CARTESIAN_POINT ( 'NONE',  ( -28.68588794268872633, 454.7448905601784759, -19.99999999999999289 ) ) ;
#20855=CARTESIAN_POINT ( 'NONE',  ( -22.27502019258947286, 232.2448905683720000, -15.47720386886985544 ) ) ;
#20857=CARTESIAN_POINT ( 'NONE',  ( -32.01814843081343298, 226.0573905683720568, 16.75240474999999307 ) ) ;
#20858=CARTESIAN_POINT ( 'NONE',  ( -38.17536295476245556, 333.8073905683720000, -14.20200298773971426 ) ) ;
#20860=AXIS2_PLACEMENT_3D ( 'NONE', #20520, #18882, #4394 ) ;
#20861=CARTESIAN_POINT ( 'NONE',  ( -10.20829729246299777, 471.6198905601784759, 7.653668647301790529 ) ) ;
#20862=LINE ( 'NONE', #12641, #9896 ) ;
#20865=CARTESIAN_POINT ( 'NONE',  ( -42.88789093042842637, 304.4323905683720000, -9.489475012073736337 ) ) ;
#20867=CARTESIAN_POINT ( 'NONE',  ( -16.84014894278199392, 390.1198905683720000, -11.84573899990672707 ) ) ;
#20869=CARTESIAN_POINT ( 'NONE',  ( -24.70764059509555466, 390.0573905601784759, 19.99999999999998934 ) ) ;
#20871=VERTEX_POINT ( 'NONE', #13805 ) ;
#20873=CARTESIAN_POINT ( 'NONE',  ( -13.20868407381887799, 500.9948905683721136, -6.410867750099233042 ) ) ;
#20874=DIRECTION ( 'NONE',  ( -1.191790137725560488E-16, 1.000000000000000000, -0.000000000000000000 ) ) ;
#20876=EDGE_CURVE ( 'NONE', #14922, #13587, #20376, .T. ) ;
#20877=CARTESIAN_POINT ( 'NONE',  ( -45.43829269268870519, 305.6823905683720000, 3.332260488124734632 ) ) ;
#20878=CARTESIAN_POINT ( 'NONE',  ( -32.01814843081344009, 326.0573905683720000, 16.75240474999999307 ) ) ;
#20879=AXIS2_PLACEMENT_3D ( 'NONE', #11492, #14969, #18090 ) ;
#20880=CARTESIAN_POINT ( 'NONE',  ( -8.685887942688712116, 267.3073905765655809, -3.978247347593165895 ) ) ;
#20881=CARTESIAN_POINT ( 'NONE',  ( -22.27502019258946220, 236.9948905683720284, 15.47720386886985189 ) ) ;
#20882=CARTESIAN_POINT ( 'NONE',  ( -45.43829269268871229, 405.6823905683720568, 3.332260488124734632 ) ) ;
#20885=CARTESIAN_POINT ( 'NONE',  ( -8.685887942688708563, 242.2448905601785043, -2.449293598294705724E-15 ) ) ;
#20886=CARTESIAN_POINT ( 'NONE',  ( -38.17536295476245556, 435.4323905683720568, 14.20200298773971781 ) ) ;
#20887=ORIENTED_EDGE ( 'NONE', *, *, #12205, .T. ) ;
#20888=( BOUNDED_CURVE ( )  B_SPLINE_CURVE ( 2, ( #8945, #14160, #18681, #17078, #2472, #643, #5920, #12529, #2261, #10889, #13947, #8839, #9053, #7209, #20425, #14052, #3868 ),
 .UNSPECIFIED., .F., .T. ) 
 B_SPLINE_CURVE_WITH_KNOTS ( ( 3, 2, 2, 2, 2, 2, 2, 2, 3 ),
 ( 0.4843750000000002220, 0.4863281250000002220, 0.4882812500000002220, 0.4902343750000002220, 0.4921875000000002220, 0.4941406250000002220, 0.4960937500000002220, 0.4980468750000002220, 0.5000000000000002220 ),
 .UNSPECIFIED. ) 
 CURVE ( )  GEOMETRIC_REPRESENTATION_ITEM ( )  RATIONAL_B_SPLINE_CURVE ( ( 0.9999999999999977796, 0.9807852804032326510, 1.000000000000000000, 0.9807852804032304306, 1.000000000000000000, 0.9807852804032304306, 1.000000000000000000, 0.9807852804032304306, 1.000000000000000000, 0.9807852804032304306, 1.000000000000000000, 0.9807852804032304306, 1.000000000000000000, 0.9807852804032304306, 1.000000000000000000, 0.9807852804032282101, 1.000000000000002220 ) ) 
 REPRESENTATION_ITEM ( '' )  );
#20889=CARTESIAN_POINT ( 'NONE',  ( -24.70764059509556176, 440.0573905601785327, 19.99999999999998934 ) ) ;
#20890=ORIENTED_EDGE ( 'NONE', *, *, #21136, .F. ) ;
#20894=CARTESIAN_POINT ( 'NONE',  ( -10.20829729246298179, 332.8698905601785327, -7.653668647301794969 ) ) ;
#20895=CARTESIAN_POINT ( 'NONE',  ( -13.20868407381886200, 370.9948905683720568, -6.410867750099233042 ) ) ;
#20897=CARTESIAN_POINT ( 'NONE',  ( -47.16347859291446554, 512.6198905765656946, 7.653668647301805628 ) ) ;
#20898=CARTESIAN_POINT ( 'NONE',  ( -25.35362745456399480, 381.0573905683719431, -16.75240474999999307 ) ) ;
#20899=CARTESIAN_POINT ( 'NONE',  ( -25.35362745456397704, 242.5573905683720000, -16.75240474999999307 ) ) ;
#20900=CARTESIAN_POINT ( 'NONE',  ( -11.93348319268872615, 398.5573905683720568, 3.332260488124728859 ) ) ;
#20901=CARTESIAN_POINT ( 'NONE',  ( -28.68588794268871212, 319.4948905765656377, -19.99999999999999289 ) ) ;
#20903=CARTESIAN_POINT ( 'NONE',  ( -25.35362745456397349, 306.6823905683720000, 16.75240474999998952 ) ) ;
#20905=CARTESIAN_POINT ( 'NONE',  ( -13.20868407381886911, 449.7448905683720000, 6.410867750099229490 ) ) ;
#20907=CARTESIAN_POINT ( 'NONE',  ( -42.82802356641965957, 368.4948905601784759, 14.14213562373094923 ) ) ;
#20910=CARTESIAN_POINT ( 'NONE',  ( -11.93348319268872260, 360.0573905683719431, 3.332260488124728415 ) ) ;
#20911=CARTESIAN_POINT ( 'NONE',  ( -14.48388495494901562, 497.9323905683720568, 9.489475012073732785 ) ) ;
#20912=CARTESIAN_POINT ( 'NONE',  ( -14.54375231895778775, 503.4948905601784759, -14.14213562373094746 ) ) ;
#20913=CARTESIAN_POINT ( 'NONE',  ( -11.93348319268871904, 328.5573905683720568, 3.332260488124728415 ) ) ;
#20914=ORIENTED_EDGE ( 'NONE', *, *, #557, .T. ) ;
#20919=CARTESIAN_POINT ( 'NONE',  ( -19.19641293061498644, 428.8073905683720000, 14.20200298773971426 ) ) ;
#20920=CARTESIAN_POINT ( 'NONE',  ( -8.685887942688911068, 446.6823905765656377, 3.978247347593586447 ) ) ;
#20922=CARTESIAN_POINT ( 'NONE',  ( -38.17536295476246266, 442.3073905683721136, -14.20200298773971426 ) ) ;
#20924=CARTESIAN_POINT ( 'NONE',  ( -35.09675569278795848, 461.9948905683720000, -15.47720386886985544 ) ) ;
#20925=CARTESIAN_POINT ( 'NONE',  ( -8.685887942688594876, 412.5573905601785896, -3.978247347592846594 ) ) ;
#20926=CARTESIAN_POINT ( 'NONE',  ( -40.01497788969914637, 410.4323905765656377, -16.95518130045146421 ) ) ;
#20931=CARTESIAN_POINT ( 'NONE',  ( -48.68588794268871567, 421.9948905765656377, 0.000000000000000000 ) ) ;
#20932=CARTESIAN_POINT ( 'NONE',  ( -28.68588794268870146, 254.7448905601784475, -19.99999999999999289 ) ) ;
#20935=CARTESIAN_POINT ( 'NONE',  ( -14.54375231895775222, 240.9948905601784759, 14.14213562373094568 ) ) ;
#20937=CARTESIAN_POINT ( 'NONE',  ( -42.88789093042844058, 424.4323905683720568, -9.489475012073736337 ) ) ;
#20938=CARTESIAN_POINT ( 'NONE',  ( -17.35679799567829917, 383.8073905601784190, -16.95518130045146421 ) ) ;
#20939=CARTESIAN_POINT ( 'NONE',  ( -32.01814843081343298, 253.1823905683720568, -16.75240474999999307 ) ) ;
#20944=CARTESIAN_POINT ( 'NONE',  ( -14.48388495494901029, 459.4323905683721136, 9.489475012073731008 ) ) ;
#20945=CARTESIAN_POINT ( 'NONE',  ( -32.66413529028186247, 224.1823905765656377, 19.99999999999999289 ) ) ;
#20948=CARTESIAN_POINT ( 'NONE',  ( -42.88789093042841927, 242.9323905683720284, -9.489475012073736337 ) ) ;
#20954=CARTESIAN_POINT ( 'NONE',  ( -8.685887942688736985, 467.3073905765656946, -3.978247347593165895 ) ) ;
#20956=CARTESIAN_POINT ( 'NONE',  ( -32.66413529028186247, 284.1823905765656377, 19.99999999999999289 ) ) ;
#20960=CARTESIAN_POINT ( 'NONE',  ( -9.656732250201606860, 223.9102039777117170, 6.363799471863218926 ) ) ;
#20961=CARTESIAN_POINT ( 'NONE',  ( -42.88789093042841927, 224.8073905683720284, 9.489475012073736337 ) ) ;
#20962=CARTESIAN_POINT ( 'NONE',  ( -19.19641293061497933, 311.9323905683720568, -14.20200298773971603 ) ) ;
#20963=ADVANCED_FACE ( 'NONE', ( #10644 ), #17262, .T. ) ;
#20964=DIRECTION ( 'NONE',  ( 1.000000000000000000, 1.191790137725560488E-16, 0.000000000000000000 ) ) ;
#20966=CARTESIAN_POINT ( 'NONE',  ( -19.19641293061497933, 301.9323905683720000, -14.20200298773971603 ) ) ;
#20968=CARTESIAN_POINT ( 'NONE',  ( -16.84014894278199037, 377.6198905683720568, 11.84573899990672530 ) ) ;
#20969=CARTESIAN_POINT ( 'NONE',  ( -16.84014894278200813, 529.1198905683720568, 11.84573899990672530 ) ) ;
#20970=CARTESIAN_POINT ( 'NONE',  ( -47.16347859291444422, 387.8698905601784759, 7.653668647301805628 ) ) ;
#20972=CARTESIAN_POINT ( 'NONE',  ( -40.01497788969912506, 230.4323905765656093, -16.95518130045146421 ) ) ;
#20975=CARTESIAN_POINT ( 'NONE',  ( -45.43829269268871940, 495.6823905683720568, 3.332260488124734632 ) ) ;
#20978=CARTESIAN_POINT ( 'NONE',  ( -40.53162694259543031, 294.1198905683720568, -11.84573899990672707 ) ) ;
#20979=CARTESIAN_POINT ( 'NONE',  ( -35.09675569278794427, 331.9948905683720000, -15.47720386886985544 ) ) ;
#20980=CARTESIAN_POINT ( 'NONE',  ( -21.03221929538690205, 265.1198905765655809, 18.47759065022572500 ) ) ;
#20981=DIRECTION ( 'NONE',  ( -1.000000000000000000, 0.000000000000000000, 0.000000000000000000 ) ) ;
#20982=CARTESIAN_POINT ( 'NONE',  ( -42.88789093042841927, 234.8073905683720284, 9.489475012073734561 ) ) ;
#20983=CARTESIAN_POINT ( 'NONE',  ( -32.01814843081345430, 403.1823905683720000, -16.75240474999999307 ) ) ;
#20985=FACE_OUTER_BOUND ( 'NONE', #2351, .T. ) ;
#20989=CARTESIAN_POINT ( 'NONE',  ( -8.685887942688738761, 506.9948905765655240, -2.449293598294705724E-15 ) ) ;
#20991=CARTESIAN_POINT ( 'NONE',  ( -19.19641293061499354, 450.4323905683720000, -14.20200298773971603 ) ) ;
#20992=CYLINDRICAL_SURFACE ( 'NONE', #9801, 19.99999999999999645 ) ;
#20994=CARTESIAN_POINT ( 'NONE',  ( -45.64106924314019409, 446.3073905601784759, -11.32908994701042715 ) ) ;
#20999=CARTESIAN_POINT ( 'NONE',  ( -42.82802356641965247, 325.9948905601784759, -14.14213562373094746 ) ) ;
#21001=CARTESIAN_POINT ( 'NONE',  ( -40.53162694259543741, 354.1198905683720568, -11.84573899990672707 ) ) ;
#21003=CARTESIAN_POINT ( 'NONE',  ( -28.68588794268872988, 494.4948905765656377, 19.99999999999999289 ) ) ;
#21004=CARTESIAN_POINT ( 'NONE',  ( -38.17536295476246266, 392.3073905683720568, -14.20200298773971426 ) ) ;
#21005=CARTESIAN_POINT ( 'NONE',  ( -13.20868407381884424, 229.7448905683720568, 6.410867750099229490 ) ) ;
#21006=CARTESIAN_POINT ( 'NONE',  ( -19.19641293061498644, 407.3073905683719431, 14.20200298773971426 ) ) ;
#21007=CARTESIAN_POINT ( 'NONE',  ( -48.68588794268870146, 322.3073905765656377, 3.978247347593168115 ) ) ;
#21009=CARTESIAN_POINT ( 'NONE',  ( -32.01814843081344009, 296.0573905683720000, 16.75240474999999307 ) ) ;
#21011=CARTESIAN_POINT ( 'NONE',  ( -19.19641293061499354, 461.9323905683720568, -14.20200298773971603 ) ) ;
#21012=LINE ( 'NONE', #10727, #17855 ) ;
#21014=CYLINDRICAL_SURFACE ( 'NONE', #3664, 19.99999999999999645 ) ;
#21015=( BOUNDED_CURVE ( )  B_SPLINE_CURVE ( 2, ( #10289, #20472, #8886, #2090, #7046, #13666, #12026, #580, #20359, #15502, #5641, #1613, #11555, #10826, #20793, #6170, #1725 ),
 .UNSPECIFIED., .F., .T. ) 
 B_SPLINE_CURVE_WITH_KNOTS ( ( 3, 2, 2, 2, 2, 2, 2, 2, 3 ),
 ( 0.9531250000000001110, 0.9550781250000001110, 0.9570312500000001110, 0.9589843750000001110, 0.9609375000000001110, 0.9628906250000001110, 0.9648437500000001110, 0.9667968750000001110, 0.9687500000000001110 ),
 .UNSPECIFIED. ) 
 CURVE ( )  GEOMETRIC_REPRESENTATION_ITEM ( )  RATIONAL_B_SPLINE_CURVE ( ( 0.9999999999999988898, 0.9807852804032315408, 1.000000000000000000, 0.9807852804032304306, 1.000000000000000000, 0.9807852804032304306, 1.000000000000000000, 0.9807852804032304306, 1.000000000000000000, 0.9807852804032304306, 1.000000000000000000, 0.9807852804032304306, 1.000000000000000000, 0.9807852804032304306, 1.000000000000000000, 0.9807852804032293204, 1.000000000000001110 ) ) 
 REPRESENTATION_ITEM ( '' )  );
#21016=CARTESIAN_POINT ( 'NONE',  ( -45.43829269268872650, 493.8698905683720568, 0.000000000000000000 ) ) ;
#21017=CARTESIAN_POINT ( 'NONE',  ( -40.01497788969915348, 508.8073905601784190, 16.95518130045146776 ) ) ;
#21018=CARTESIAN_POINT ( 'NONE',  ( -22.27502019258948351, 330.7448905683720568, -15.47720386886985544 ) ) ;
#21020=CARTESIAN_POINT ( 'NONE',  ( -11.73070664223726922, 523.1823905601784190, -11.32908994701042538 ) ) ;
#21021=ORIENTED_EDGE ( 'NONE', *, *, #20274, .F. ) ;
#21024=CARTESIAN_POINT ( 'NONE',  ( -45.43829269268871940, 425.0573905683720568, -3.332260488124726638 ) ) ;
#21025=FACE_OUTER_BOUND ( 'NONE', #19931, .T. ) ;
#21026=CARTESIAN_POINT ( 'NONE',  ( -42.88789093042844058, 442.9323905683721136, -9.489475012073736337 ) ) ;
#21028=CARTESIAN_POINT ( 'NONE',  ( -45.43829269268872650, 473.8698905683720568, 0.000000000000000000 ) ) ;
#21030=CARTESIAN_POINT ( 'NONE',  ( -32.66413529028187668, 374.1823905765655809, 19.99999999999999289 ) ) ;
#21031=CARTESIAN_POINT ( 'NONE',  ( -45.64106924314017277, 281.0573905765656377, -11.32908994701042538 ) ) ;
#21035=VECTOR ( 'NONE', #18054, 1000.000000000000000 ) ;
#21039=CARTESIAN_POINT ( 'NONE',  ( -44.87387987751963436, 223.9102039777115465, 7.648793815183834610 ) ) ;
#21041=CARTESIAN_POINT ( 'NONE',  ( -14.48388495494900496, 429.4323905683720000, 9.489475012073732785 ) ) ;
#21042=DIRECTION ( 'NONE',  ( -1.191790137725560488E-16, 1.000000000000000000, -0.000000000000000000 ) ) ;
#21043=CARTESIAN_POINT ( 'NONE',  ( -14.48388495494898542, 241.3073905683720852, -9.489475012073736337 ) ) ;
#21046=CARTESIAN_POINT ( 'NONE',  ( -24.70764059509555466, 424.8073905765656377, 19.99999999999998934 ) ) ;
#21047=VERTEX_POINT ( 'NONE', #9346 ) ;
#21048=CARTESIAN_POINT ( 'NONE',  ( -44.16309181155857999, 465.9948905683720000, 6.410867750099241924 ) ) ;
#21049=CARTESIAN_POINT ( 'NONE',  ( -45.64106924314017277, 231.0573905765656093, -11.32908994701042715 ) ) ;
#21050=ORIENTED_EDGE ( 'NONE', *, *, #8218, .F. ) ;
#21051=CARTESIAN_POINT ( 'NONE',  ( -43.15102588740143119, 208.1950015687324651, 3.974285180378254179 ) ) ;
#21052=CARTESIAN_POINT ( 'NONE',  ( -42.88789093042841927, 222.9323905683720284, -9.489475012073736337 ) ) ;
#21053=EDGE_LOOP ( 'NONE', ( #20436, #506, #17843, #2374 ) ) ;
#21054=CARTESIAN_POINT ( 'NONE',  ( -13.20868407381888154, 529.4948905683720568, -6.410867750099233042 ) ) ;
#21056=VECTOR ( 'NONE', #16119, 1000.000000000000000 ) ;
#21058=CARTESIAN_POINT ( 'NONE',  ( -32.66413529028188378, 434.1823905765656377, 19.99999999999999289 ) ) ;
#21059=CARTESIAN_POINT ( 'NONE',  ( -17.35679799567828852, 350.6823905601785327, 16.95518130045146421 ) ) ;
#21060=CARTESIAN_POINT ( 'NONE',  ( -40.01497788969912506, 283.5573905765656377, 16.95518130045146776 ) ) ;
#21063=CARTESIAN_POINT ( 'NONE',  ( -20.29731878304196968, 220.5357918889952771, -14.50086109035067317 ) ) ;
#21064=CARTESIAN_POINT ( 'NONE',  ( -22.27502019258947996, 312.2448905683720000, -15.47720386886985544 ) ) ;
#21067=CARTESIAN_POINT ( 'NONE',  ( -45.43829269268869808, 305.6823905683719431, 3.332260488124734632 ) ) ;
#21069=CARTESIAN_POINT ( 'NONE',  ( -32.01814843081344719, 361.6823905683720568, -16.75240474999999307 ) ) ;
#21070=CARTESIAN_POINT ( 'NONE',  ( -19.19641293061499709, 518.8073905683719431, 14.20200298773971426 ) ) ;
#21071=( BOUNDED_CURVE ( )  B_SPLINE_CURVE ( 2, ( #1254, #7832, #16183, #7622, #1360, #7932, #6320, #6958, #8144, #8368, #6852, #11514, #21360, #18217, #6528, #284, #16720 ),
 .UNSPECIFIED., .F., .T. ) 
 B_SPLINE_CURVE_WITH_KNOTS ( ( 3, 2, 2, 2, 2, 2, 2, 2, 3 ),
 ( 0.8281250000000002220, 0.8300781250000002220, 0.8320312500000002220, 0.8339843750000002220, 0.8359375000000002220, 0.8378906250000002220, 0.8398437500000002220, 0.8417968750000002220, 0.8437500000000002220 ),
 .UNSPECIFIED. ) 
 CURVE ( )  GEOMETRIC_REPRESENTATION_ITEM ( )  RATIONAL_B_SPLINE_CURVE ( ( 0.9999999999999977796, 0.9807852804032326510, 1.000000000000000000, 0.9807852804032304306, 1.000000000000000000, 0.9807852804032304306, 1.000000000000000000, 0.9807852804032304306, 1.000000000000000000, 0.9807852804032304306, 1.000000000000000000, 0.9807852804032304306, 1.000000000000000000, 0.9807852804032304306, 1.000000000000000000, 0.9807852804032282101, 1.000000000000002220 ) ) 
 REPRESENTATION_ITEM ( '' )  );
#21072=CARTESIAN_POINT ( 'NONE',  ( -47.16347859291444422, 367.8698905601784759, 7.653668647301805628 ) ) ;
#21075=CARTESIAN_POINT ( 'NONE',  ( -35.09675569278796559, 487.2448905683720000, 15.47720386886985366 ) ) ;
#21076=FACE_OUTER_BOUND ( 'NONE', #10766, .T. ) ;
#21077=CARTESIAN_POINT ( 'NONE',  ( -11.93348319268871016, 278.8698905683720000, -2.051577885510841163E-15 ) ) ;
#21081=CARTESIAN_POINT ( 'NONE',  ( -42.88789093042842637, 284.4323905683720568, -9.489475012073734561 ) ) ;
#21082=CARTESIAN_POINT ( 'NONE',  ( -22.27502019258947286, 316.9948905683720568, 15.47720386886985189 ) ) ;
#21083=CARTESIAN_POINT ( 'NONE',  ( -11.73070664223723369, 256.0573905765656377, 11.32908994701042005 ) ) ;
#21084=CARTESIAN_POINT ( 'NONE',  ( -8.685887942688735208, 472.2448905601784759, -2.449293598294705724E-15 ) ) ;
#21085=CARTESIAN_POINT ( 'NONE',  ( -38.17536295476243424, 225.4323905683720000, 14.20200298773971781 ) ) ;
#21086=CARTESIAN_POINT ( 'NONE',  ( -38.17536295476245556, 373.8073905683720000, -14.20200298773971426 ) ) ;
#21091=CARTESIAN_POINT ( 'NONE',  ( -14.48388495494900852, 439.8073905683721136, -9.489475012073736337 ) ) ;
#21095=CARTESIAN_POINT ( 'NONE',  ( -48.68588794268871567, 426.9323905601784759, -3.978247347593158345 ) ) ;
#21096=ORIENTED_EDGE ( 'NONE', *, *, #19545, .F. ) ;
#21100=CARTESIAN_POINT ( 'NONE',  ( -40.01497788969913927, 335.6823905601784759, -16.95518130045146421 ) ) ;
#21101=DIRECTION ( 'NONE',  ( -1.191790137725560488E-16, 1.000000000000000000, -0.000000000000000000 ) ) ;
#21102=CARTESIAN_POINT ( 'NONE',  ( -25.35362745456398770, 342.5573905683721136, -16.75240474999999307 ) ) ;
#21105=CARTESIAN_POINT ( 'NONE',  ( -40.01497788969915348, 503.5573905765656946, 16.95518130045146776 ) ) ;
#21106=CARTESIAN_POINT ( 'NONE',  ( -32.01814843081345430, 391.6823905683720568, -16.75240474999999307 ) ) ;
#21109=CARTESIAN_POINT ( 'NONE',  ( -16.84014894278199392, 380.1198905683720568, -11.84573899990672707 ) ) ;
#21110=CARTESIAN_POINT ( 'NONE',  ( -14.54375231895776466, 318.2448905765656377, -14.14213562373094746 ) ) ;
#21111=CYLINDRICAL_SURFACE ( 'NONE', #8609, 15.00000000000000000 ) ;
#21112=CARTESIAN_POINT ( 'NONE',  ( -45.43829269268870519, 293.5573905683720568, -3.332260488124726638 ) ) ;
#21113=CARTESIAN_POINT ( 'NONE',  ( -38.17536295476246266, 433.8073905683720568, -14.20200298773971426 ) ) ;
#21114=CARTESIAN_POINT ( 'NONE',  ( -8.685887942688712116, 282.2448905601784759, -2.449293598294705724E-15 ) ) ;
#21115=CARTESIAN_POINT ( 'NONE',  ( -45.64106924314017988, 368.1823905601785327, 11.32908994701042538 ) ) ;
#21116=CYLINDRICAL_SURFACE ( 'NONE', #5383, 19.99999999999999645 ) ;
#21118=CARTESIAN_POINT ( 'NONE',  ( -19.19641293061498644, 351.9323905683720568, -14.20200298773971603 ) ) ;
#21119=CARTESIAN_POINT ( 'NONE',  ( -45.43829269268872650, 503.8698905683720568, 0.000000000000000000 ) ) ;
#21121=CARTESIAN_POINT ( 'NONE',  ( -32.66413529028189089, 505.0573905601784759, -19.99999999999999289 ) ) ;
#21122=CARTESIAN_POINT ( 'NONE',  ( -14.48388495494899253, 317.9323905683720000, 9.489475012073732785 ) ) ;
#21128=CARTESIAN_POINT ( 'NONE',  ( -14.48388495494900674, 401.3073905683720000, -9.489475012073734561 ) ) ;
#21129=CARTESIAN_POINT ( 'NONE',  ( -14.54375231895775222, 235.7448905765656093, 14.14213562373094568 ) ) ;
#21131=CARTESIAN_POINT ( 'NONE',  ( -32.01814843081345430, 446.0573905683720568, 16.75240474999999307 ) ) ;
#21133=CARTESIAN_POINT ( 'NONE',  ( -40.53162694259545162, 455.1198905683720568, 11.84573899990672885 ) ) ;
#21136=EDGE_CURVE ( 'NONE', #4636, #18799, #13756, .T. ) ;
#21137=CARTESIAN_POINT ( 'NONE',  ( -40.01497788969914637, 390.4323905765655809, -16.95518130045146421 ) ) ;
#21143=CARTESIAN_POINT ( 'NONE',  ( -14.48388495494901562, 491.3073905683720000, -9.489475012073736337 ) ) ;
#21146=CARTESIAN_POINT ( 'NONE',  ( -39.58131762249983154, 223.9102039777117170, 16.01692832265988642 ) ) ;
#21147=CARTESIAN_POINT ( 'NONE',  ( -40.53162694259544452, 416.6198905683720000, 11.84573899990672885 ) ) ;
#21148=CARTESIAN_POINT ( 'NONE',  ( -24.70764059509556176, 384.4323905601784190, -19.99999999999999289 ) ) ;
#21149=CARTESIAN_POINT ( 'NONE',  ( -19.19641293061497223, 251.9323905683720284, -14.20200298773971603 ) ) ;
#21151=EDGE_LOOP ( 'NONE', ( #9019, #12321, #20737, #10580 ) ) ;
#21152=CYLINDRICAL_SURFACE ( 'NONE', #16204, 19.99999999999999645 ) ;
#21154=CARTESIAN_POINT ( 'NONE',  ( -22.27502019258949062, 468.4948905683720000, 15.47720386886985189 ) ) ;
#21155=AXIS2_PLACEMENT_3D ( 'NONE', #13989, #12671, #1008 ) ;
#21156=CARTESIAN_POINT ( 'NONE',  ( -21.03221929538690915, 228.8698905765655809, -18.47759065022572855 ) ) ;
#21158=CARTESIAN_POINT ( 'NONE',  ( -13.20868407381887977, 529.7448905683720568, 6.410867750099229490 ) ) ;
#21159=ORIENTED_EDGE ( 'NONE', *, *, #7140, .F. ) ;
#21160=CARTESIAN_POINT ( 'NONE',  ( -25.35362745456401257, 531.0573905683719431, -16.75240474999999307 ) ) ;
#21161=DIRECTION ( 'NONE',  ( -1.000000000000000000, 0.000000000000000000, 0.000000000000000000 ) ) ;
#21162=CARTESIAN_POINT ( 'NONE',  ( -8.685887942688731655, 447.3073905765656377, -3.978247347593165895 ) ) ;
#21165=CARTESIAN_POINT ( 'NONE',  ( -11.93348319268872260, 339.1823905683720000, -3.332260488124732856 ) ) ;
#21166=CARTESIAN_POINT ( 'NONE',  ( -32.66413529028188378, 454.1823905765656377, 19.99999999999999289 ) ) ;
#21168=CARTESIAN_POINT ( 'NONE',  ( -8.685887942688802710, 291.9323905601784759, 3.978247347593374172 ) ) ;
#21172=CARTESIAN_POINT ( 'NONE',  ( -45.43829269268870519, 315.3698905683720568, 0.000000000000000000 ) ) ;
#21173=CARTESIAN_POINT ( 'NONE',  ( -10.20829729246299600, 442.8698905601784759, -7.653668647301794969 ) ) ;
#21175=CARTESIAN_POINT ( 'NONE',  ( -35.09675569278793716, 313.4948905683720000, -15.47720386886985544 ) ) ;
#21177=CARTESIAN_POINT ( 'NONE',  ( -45.43829269268873361, 515.6823905683720568, 3.332260488124734632 ) ) ;
#21179=CARTESIAN_POINT ( 'NONE',  ( -17.35679799567829917, 373.8073905601784759, -16.95518130045146421 ) ) ;
#21182=CARTESIAN_POINT ( 'NONE',  ( -45.43829269268872650, 485.3698905683720568, 0.000000000000000000 ) ) ;
#21184=CARTESIAN_POINT ( 'NONE',  ( -45.43829269268869808, 274.1823905683720000, 3.332260488124734632 ) ) ;
#21186=CARTESIAN_POINT ( 'NONE',  ( -28.68588794268870501, 282.8698905683720568, -16.75240474999999307 ) ) ;
#21187=CARTESIAN_POINT ( 'NONE',  ( -38.17536295476245556, 332.3073905683720000, -14.20200298773971426 ) ) ;
#21188=CARTESIAN_POINT ( 'NONE',  ( -11.93348319268870839, 260.6823905683720000, -3.332260488124732856 ) ) ;
#21189=ADVANCED_FACE ( 'NONE', ( #16285 ), #1460, .T. ) ;
#21190=AXIS2_PLACEMENT_3D ( 'NONE', #2270, #20220, #20434 ) ;
#21191=CARTESIAN_POINT ( 'NONE',  ( -40.01497788969912506, 260.4323905765656377, -16.95518130045146421 ) ) ;
#21193=CARTESIAN_POINT ( 'NONE',  ( -35.09675569278793716, 225.7448905683720568, 15.47720386886985366 ) ) ;
#21194=CARTESIAN_POINT ( 'NONE',  ( -28.68588794268874054, 573.2448905601785327, 0.000000000000000000 ) ) ;
#21196=CARTESIAN_POINT ( 'NONE',  ( -19.19641293061498288, 368.8073905683720000, 14.20200298773971426 ) ) ;
#21200=CARTESIAN_POINT ( 'NONE',  ( -21.03221929538691271, 268.8698905765656377, -18.47759065022572855 ) ) ;
#21203=CARTESIAN_POINT ( 'NONE',  ( -16.84014894278199748, 430.1198905683720000, -11.84573899990672707 ) ) ;
#21206=CARTESIAN_POINT ( 'NONE',  ( -36.33955658999051508, 435.3698905601784759, -18.47759065022572855 ) ) ;
#21211=CARTESIAN_POINT ( 'NONE',  ( -32.66413529028186957, 305.0573905601784759, -19.99999999999999289 ) ) ;
#21214=CARTESIAN_POINT ( 'NONE',  ( -25.35362745456397704, 338.1823905683720000, 16.75240474999998952 ) ) ;
#21215=CARTESIAN_POINT ( 'NONE',  ( -48.68588794268872988, 512.3073905765655809, 3.978247347593168115 ) ) ;
#21216=CARTESIAN_POINT ( 'NONE',  ( -40.53162694259543741, 375.1198905683720000, 11.84573899990672885 ) ) ;
#21217=CARTESIAN_POINT ( 'NONE',  ( -28.68588794268869435, 227.8698905683720284, 16.75240474999999307 ) ) ;
#21218=CARTESIAN_POINT ( 'NONE',  ( -16.84014894278199392, 390.1198905683720000, -11.84573899990672707 ) ) ;
#21220=CARTESIAN_POINT ( 'NONE',  ( -21.03221929538690560, 325.1198905765655809, 18.47759065022572500 ) ) ;
#21222=CARTESIAN_POINT ( 'NONE',  ( -40.53162694259543031, 285.1198905683720568, 11.84573899990672885 ) ) ;
#21224=CARTESIAN_POINT ( 'NONE',  ( -16.84014894278200103, 441.6198905683720568, -11.84573899990672707 ) ) ;
#21225=CARTESIAN_POINT ( 'NONE',  ( -32.66413529028186247, 285.0573905601784759, -19.99999999999999289 ) ) ;
#21228=CARTESIAN_POINT ( 'NONE',  ( -32.01814843081344719, 343.1823905683721136, -16.75240474999999307 ) ) ;
#21229=CARTESIAN_POINT ( 'NONE',  ( -16.84014894278200103, 477.6198905683720000, 11.84573899990672530 ) ) ;
#21230=CARTESIAN_POINT ( 'NONE',  ( -21.03221929538692336, 490.3698905601784759, 18.47759065022572500 ) ) ;
#21231=CARTESIAN_POINT ( 'NONE',  ( -45.43829269268869808, 314.1823905683720000, 3.332260488124734632 ) ) ;
#21233=CARTESIAN_POINT ( 'NONE',  ( -21.03221929538689849, 260.3698905601785327, 18.47759065022572500 ) ) ;
#21236=CARTESIAN_POINT ( 'NONE',  ( -22.27502019258947996, 398.4948905683720000, 15.47720386886985189 ) ) ;
#21237=CARTESIAN_POINT ( 'NONE',  ( -47.16347859291443001, 232.6198905765656377, 7.653668647301805628 ) ) ;
#21239=CARTESIAN_POINT ( 'NONE',  ( -32.01814843081345430, 441.6823905683721136, -16.75240474999999307 ) ) ;
#21240=CARTESIAN_POINT ( 'NONE',  ( -45.43829269268871940, 444.1823905683719431, 3.332260488124734632 ) ) ;
#21243=CARTESIAN_POINT ( 'NONE',  ( -8.685887942688722774, 377.3073905765656946, -3.978247347593165895 ) ) ;
#21245=CARTESIAN_POINT ( 'NONE',  ( -17.35679799567829917, 388.5573905765656377, -16.95518130045146421 ) ) ;
#21247=CARTESIAN_POINT ( 'NONE',  ( -17.35679799567827786, 255.4323905765656377, 16.95518130045146421 ) ) ;
#21248=CARTESIAN_POINT ( 'NONE',  ( -14.48388495494901740, 501.3073905683720568, -9.489475012073736337 ) ) ;
#21251=CARTESIAN_POINT ( 'NONE',  ( -17.35679799567830628, 520.6823905601785327, 16.95518130045146421 ) ) ;
#21252=CARTESIAN_POINT ( 'NONE',  ( -44.16309181155857999, 414.7448905683720568, -6.410867750099231266 ) ) ;
#21253=CARTESIAN_POINT ( 'NONE',  ( -28.68588794268874054, 573.2448905601785327, 0.000000000000000000 ) ) ;
#21254=CARTESIAN_POINT ( 'NONE',  ( -22.27502019258947286, 232.2448905683720000, -15.47720386886985544 ) ) ;
#21255=EDGE_CURVE ( 'NONE', #15902, #13267, #11615, .T. ) ;
#21257=ORIENTED_EDGE ( 'NONE', *, *, #18023, .T. ) ;
#21258=CARTESIAN_POINT ( 'NONE',  ( -38.17536295476246977, 473.8073905683720000, -14.20200298773971426 ) ) ;
#21259=CARTESIAN_POINT ( 'NONE',  ( -44.16309181155859420, 533.2448905683719431, -6.410867750099231266 ) ) ;
#21260=ORIENTED_EDGE ( 'NONE', *, *, #17633, .F. ) ;
#21262=CARTESIAN_POINT ( 'NONE',  ( -40.53162694259542320, 225.1198905683720000, 11.84573899990672885 ) ) ;
#21263=EDGE_LOOP ( 'NONE', ( #10705, #19770, #20887, #8236 ) ) ;
#21264=CARTESIAN_POINT ( 'NONE',  ( -45.43829269268873361, 514.1823905683720568, 3.332260488124734632 ) ) ;
#21266=CARTESIAN_POINT ( 'NONE',  ( -11.73070664223726034, 437.9323905765655809, -11.32908994701042715 ) ) ;
#21267=CARTESIAN_POINT ( 'NONE',  ( -8.685887942688722774, 356.9948905765655809, -2.449293598294705724E-15 ) ) ;
#21268=CARTESIAN_POINT ( 'NONE',  ( -14.54375231895775755, 248.2448905765656377, -14.14213562373094746 ) ) ;
#21271=CARTESIAN_POINT ( 'NONE',  ( -45.64106924314017277, 288.1823905601785327, 11.32908994701042538 ) ) ;
#21272=CARTESIAN_POINT ( 'NONE',  ( -19.19641293061496512, 227.3073905683720000, 14.20200298773971426 ) ) ;
#21273=CARTESIAN_POINT ( 'NONE',  ( -42.88789093042842637, 326.3073905683721136, 9.489475012073736337 ) ) ;
#21274=CARTESIAN_POINT ( 'NONE',  ( -32.66413529028187668, 445.0573905601784759, -19.99999999999999289 ) ) ;
#21275=CARTESIAN_POINT ( 'NONE',  ( -14.54375231895775755, 263.4948905601784759, -14.14213562373094746 ) ) ;
#21277=CARTESIAN_POINT ( 'NONE',  ( -25.35362745456397349, 288.1823905683720000, 16.75240474999998952 ) ) ;
#21278=CARTESIAN_POINT ( 'NONE',  ( -42.88789093042845479, 526.3073905683720568, 9.489475012073734561 ) ) ;
#21279=CARTESIAN_POINT ( 'NONE',  ( -28.68588794268871212, 359.7448905601784759, 19.99999999999999289 ) ) ;
#21283=CARTESIAN_POINT ( 'NONE',  ( -35.09675569278796559, 477.2448905683720568, 15.47720386886985366 ) ) ;
#21285=CARTESIAN_POINT ( 'NONE',  ( -14.48388495494899075, 279.8073905683720000, -9.489475012073736337 ) ) ;
#21286=ORIENTED_EDGE ( 'NONE', *, *, #20876, .F. ) ;
#21287=CARTESIAN_POINT ( 'NONE',  ( -14.48388495494899075, 281.3073905683720000, -9.489475012073734561 ) ) ;
#21289=CARTESIAN_POINT ( 'NONE',  ( -28.68588794268870856, 311.3698905683720568, -16.75240474999999307 ) ) ;
#21290=CARTESIAN_POINT ( 'NONE',  ( -36.33955658999050087, 253.8698905765656093, 18.47759065022572500 ) ) ;
#21292=CARTESIAN_POINT ( 'NONE',  ( -13.20868407381884602, 229.4948905683720284, -6.410867750099233042 ) ) ;
#21294=CARTESIAN_POINT ( 'NONE',  ( -38.17536295476245556, 383.8073905683720568, -14.20200298773971426 ) ) ;
#21299=DIRECTION ( 'NONE',  ( -1.191790137725560488E-16, 1.000000000000000000, -0.000000000000000000 ) ) ;
#21301=CARTESIAN_POINT ( 'NONE',  ( -25.35362745456399836, 421.0573905683720000, -16.75240474999999307 ) ) ;
#21305=CARTESIAN_POINT ( 'NONE',  ( -17.35679799567830628, 433.8073905601784759, -16.95518130045146421 ) ) ;
#21309=CARTESIAN_POINT ( 'NONE',  ( -14.54375231895776643, 355.7448905765655809, 14.14213562373094568 ) ) ;
#21310=CARTESIAN_POINT ( 'NONE',  ( -47.16347859291443712, 297.8698905601784759, 7.653668647301805628 ) ) ;
#21312=CARTESIAN_POINT ( 'NONE',  ( -11.93348319268871904, 340.3698905683720000, -2.051577885510841163E-15 ) ) ;
#21313=AXIS2_PLACEMENT_3D ( 'NONE', #2443, #15647, #833 ) ;
#21314=CARTESIAN_POINT ( 'NONE',  ( -47.16347859291445843, 481.3698905765655809, -7.653668647301793193 ) ) ;
#21315=CARTESIAN_POINT ( 'NONE',  ( -44.16309181155856578, 374.4948905683720000, 6.410867750099241924 ) ) ;
#21316=CARTESIAN_POINT ( 'NONE',  ( -19.19641293061496512, 228.8073905683720284, 14.20200298773971426 ) ) ;
#21317=CARTESIAN_POINT ( 'NONE',  ( -32.01814843081344719, 391.6823905683720568, -16.75240474999999307 ) ) ;
#21320=CARTESIAN_POINT ( 'NONE',  ( -21.03221929538690560, 315.1198905765656377, 18.47759065022572500 ) ) ;
#21321=CARTESIAN_POINT ( 'NONE',  ( -24.70764059509556532, 424.4323905601785327, -19.99999999999999289 ) ) ;
#21322=CARTESIAN_POINT ( 'NONE',  ( -13.20868407381884779, 278.2448905683720568, 6.410867750099229490 ) ) ;
#21326=CARTESIAN_POINT ( 'NONE',  ( -19.19641293061498999, 431.9323905683719431, -14.20200298773971603 ) ) ;
#21328=CARTESIAN_POINT ( 'NONE',  ( -11.73070664223726745, 513.1823905601785327, -11.32908994701042538 ) ) ;
#21330=CARTESIAN_POINT ( 'NONE',  ( -48.68588794268877251, 447.5573905601785327, 3.978247347593061978 ) ) ;
#21332=CARTESIAN_POINT ( 'NONE',  ( -44.16309181155857289, 344.7448905683720568, -6.410867750099231266 ) ) ;
#21333=CARTESIAN_POINT ( 'NONE',  ( -35.09675569278796559, 485.7448905683720568, 15.47720386886985366 ) ) ;
#21335=CARTESIAN_POINT ( 'NONE',  ( -40.01497788969914637, 488.8073905601784759, 16.95518130045146776 ) ) ;
#21336=CARTESIAN_POINT ( 'NONE',  ( -44.16309181155855867, 304.4948905683720568, 6.410867750099241924 ) ) ;
#21339=ORIENTED_EDGE ( 'NONE', *, *, #19267, .T. ) ;
#21342=ORIENTED_EDGE ( 'NONE', *, *, #20031, .F. ) ;
#21343=CARTESIAN_POINT ( 'NONE',  ( -40.53162694259544452, 404.1198905683720000, -11.84573899990672707 ) ) ;
#21344=CARTESIAN_POINT ( 'NONE',  ( -48.68588794268885778, 477.5573905601784759, 3.978247347592849259 ) ) ;
#21345=DIRECTION ( 'NONE',  ( -1.000000000000000000, 0.000000000000000000, 0.000000000000000000 ) ) ;
#21346=CARTESIAN_POINT ( 'NONE',  ( -35.09675569278795848, 445.7448905683720000, 15.47720386886985366 ) ) ;
#21347=CARTESIAN_POINT ( 'NONE',  ( -16.84014894278200103, 440.1198905683720568, -11.84573899990672707 ) ) ;
#21348=CARTESIAN_POINT ( 'NONE',  ( -32.66413529028187668, 415.0573905601784759, -19.99999999999999289 ) ) ;
#21349=EDGE_CURVE ( 'NONE', #5796, #13961, #13573, .T. ) ;
#21350=CARTESIAN_POINT ( 'NONE',  ( -11.73070664223725146, 386.0573905765656946, 11.32908994701042005 ) ) ;
#21352=CARTESIAN_POINT ( 'NONE',  ( -28.68588794268874054, 573.2448905601785327, 0.000000000000000000 ) ) ;
#21354=CARTESIAN_POINT ( 'NONE',  ( -10.20829729246300133, 487.6198905765656377, -7.653668647301794969 ) ) ;
#21355=CARTESIAN_POINT ( 'NONE',  ( -32.01814843081346140, 487.5573905683720568, 16.75240474999999307 ) ) ;
#21358=LINE ( 'NONE', #3509, #408 ) ;
#21359=CARTESIAN_POINT ( 'NONE',  ( -25.35362745456399480, 402.5573905683720000, -16.75240474999999307 ) ) ;
#21360=CARTESIAN_POINT ( 'NONE',  ( -42.82802356641964536, 263.2448905765656377, 14.14213562373094923 ) ) ;
#21361=CARTESIAN_POINT ( 'NONE',  ( -11.93348319268870661, 230.0573905683720284, 3.332260488124728415 ) ) ;
#21365=VERTEX_POINT ( 'NONE', #6952 ) ;
#21366=CARTESIAN_POINT ( 'NONE',  ( -45.43829269268871940, 445.0573905683720000, -3.332260488124726638 ) ) ;
#21367=CARTESIAN_POINT ( 'NONE',  ( -17.35679799567827786, 235.4323905765656093, 16.95518130045146421 ) ) ;
#21369=VERTEX_POINT ( 'NONE', #20163 ) ;
#21371=CARTESIAN_POINT ( 'NONE',  ( -14.48388495494898187, 227.9323905683720000, 9.489475012073732785 ) ) ;
#21373=CARTESIAN_POINT ( 'NONE',  ( -38.17536295476246977, 502.3073905683720568, -14.20200298773971426 ) ) ;
#21375=CARTESIAN_POINT ( 'NONE',  ( -8.685887942688729879, 436.9948905765656377, -2.449293598294705724E-15 ) ) ;
#21376=CARTESIAN_POINT ( 'NONE',  ( -36.33955658999050797, 360.1198905765656377, -18.47759065022572855 ) ) ;
#21377=CARTESIAN_POINT ( 'NONE',  ( -45.64106924314016567, 251.0573905765656093, -11.32908994701042538 ) ) ;
#21378=CYLINDRICAL_SURFACE ( 'NONE', #12559, 19.99999999999999645 ) ;
#21380=EDGE_CURVE ( 'NONE', #15268, #14922, #15150, .T. ) ;
#21381=CARTESIAN_POINT ( 'NONE',  ( -10.20829729246297646, 291.6198905601784759, 7.653668647301790529 ) ) ;
#21384=CARTESIAN_POINT ( 'NONE',  ( -14.80883852731595596, 223.9102039777117170, 14.49255704181644866 ) ) ;
#21385=LINE ( 'NONE', #18025, #5566 ) ;
#21386=CARTESIAN_POINT ( 'NONE',  ( -45.43829269268869808, 315.6823905683720000, 3.332260488124734632 ) ) ;
#21387=PLANE ( 'NONE',  #11274 ) ;
#21388=CARTESIAN_POINT ( 'NONE',  ( -42.82802356641965247, 275.9948905601785327, -14.14213562373094746 ) ) ;
#21390=CARTESIAN_POINT ( 'NONE',  ( -42.88789093042842637, 284.4323905683720000, -9.489475012073736337 ) ) ;
#21392=CARTESIAN_POINT ( 'NONE',  ( -48.68588794268873698, 573.2448905601785327, 0.000000000000000000 ) ) ;
#21436=COLOUR_RGB('Black',0.12,0.14,0.17);
#21437=FILL_AREA_STYLE_COLOUR('',#21436);
#21438=FILL_AREA_STYLE('',(#21437));
#21439=SURFACE_STYLE_FILL_AREA(#21438);
#21440=SURFACE_SIDE_STYLE('',(#21439));
#21441=SURFACE_STYLE_USAGE(.BOTH.,#21440);
#21442=PRESENTATION_STYLE_ASSIGNMENT((#21441));
ENDSEC;
END-ISO-10303-21;
